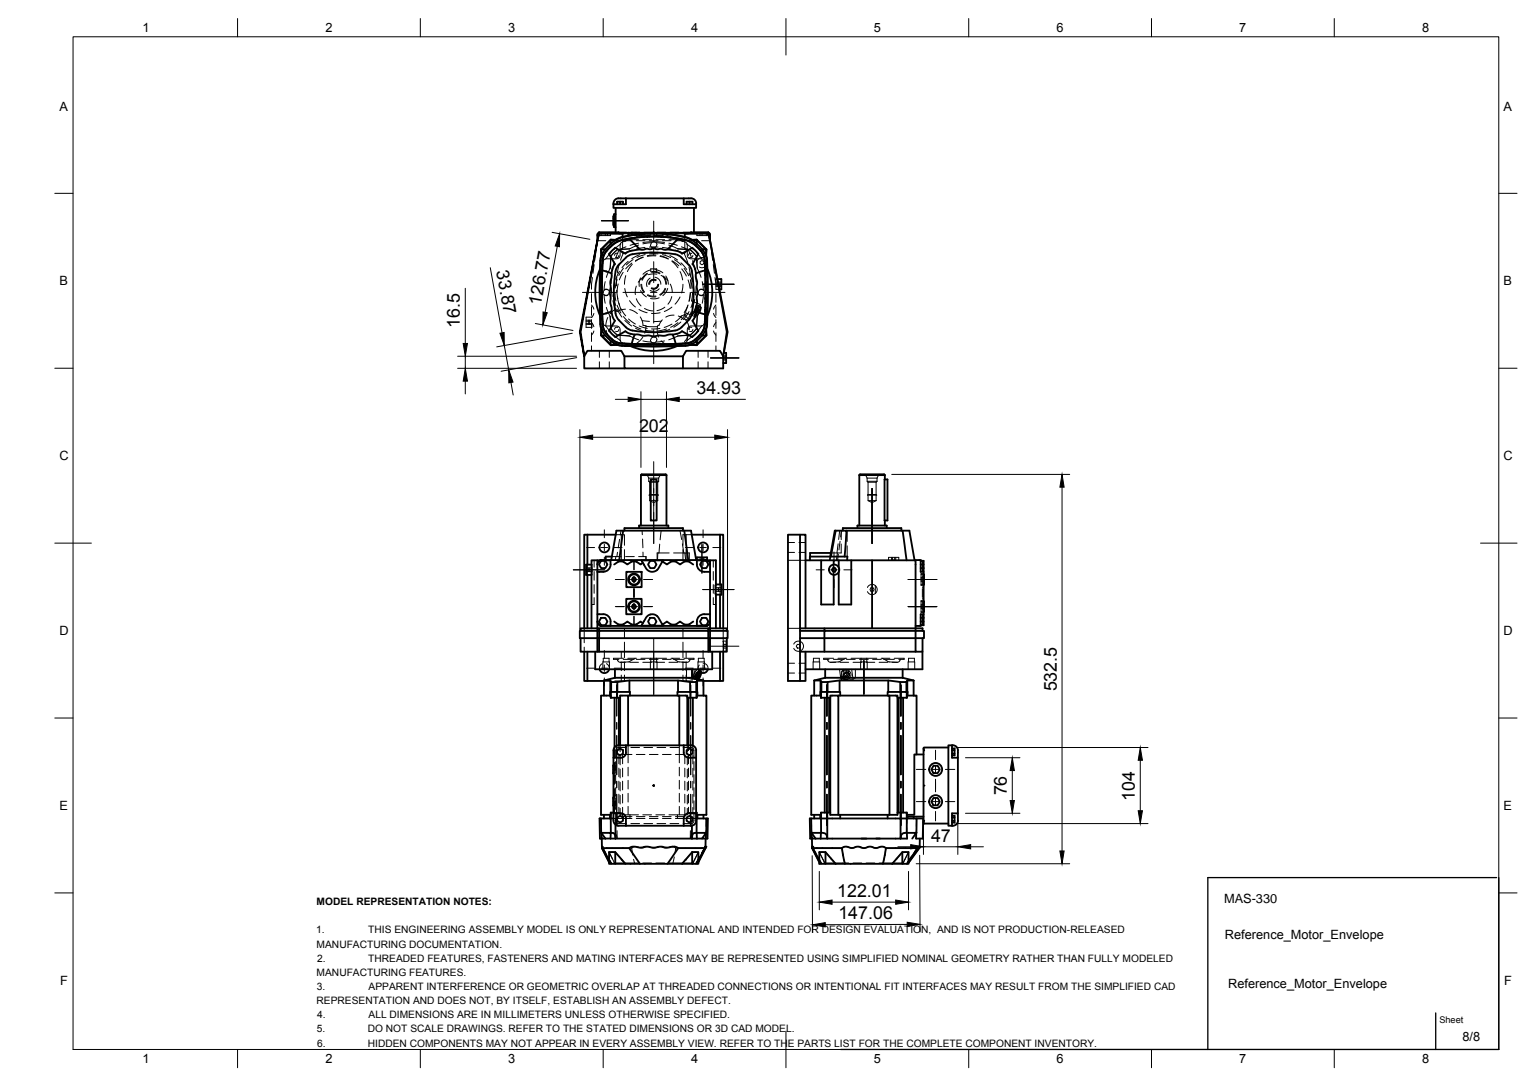
ISO-10303-21;
HEADER;
/* Generated by software containing ST-Developer
 * from STEP Tools, Inc. (www.steptools.com) 
 */

FILE_DESCRIPTION(
/* description */ ('STEP AP214'),
/* implementation_level */ '2;1');

FILE_NAME(
/* name */ 'Reference_Motor_Envelope.step',
/* time_stamp */ '2026-10-12T14:05:15-07:00',
/* author */ (''),
/* organization */ (''),
/* preprocessor_version */ 'ST-DEVELOPER v20.2',
/* originating_system */ 'Autodesk Translation Framework v15.15.0.0',
/* authorisation */ '');

FILE_SCHEMA (('AUTOMOTIVE_DESIGN { 1 0 10303 214 3 1 1 }'));
ENDSEC;

DATA;
#10=MECHANICAL_DESIGN_GEOMETRIC_PRESENTATION_REPRESENTATION('',(#288),#39959);
#95=SPHERICAL_SURFACE('',#19264,20.3600000000001);
#96=SPHERICAL_SURFACE('',#19265,20.3600000000002);
#97=(
BOUNDED_CURVE()
B_SPLINE_CURVE(3,(#30732,#30733,#30734,#30735),.UNSPECIFIED.,.F.,.F.)
B_SPLINE_CURVE_WITH_KNOTS((4,4),(-1.,-3.7852598383457E-5),.UNSPECIFIED.)
CURVE()
GEOMETRIC_REPRESENTATION_ITEM()
RATIONAL_B_SPLINE_CURVE((1.,0.978516928803385,0.978516115613319,0.999997560429802))
REPRESENTATION_ITEM('')
);
#98=(
BOUNDED_CURVE()
B_SPLINE_CURVE(3,(#30762,#30763,#30764,#30765),.UNSPECIFIED.,.F.,.F.)
B_SPLINE_CURVE_WITH_KNOTS((4,4),(-1.,0.),.UNSPECIFIED.)
CURVE()
GEOMETRIC_REPRESENTATION_ITEM()
RATIONAL_B_SPLINE_CURVE((1.,0.998672257010864,0.998672257010864,1.))
REPRESENTATION_ITEM('')
);
#99=(
BOUNDED_CURVE()
B_SPLINE_CURVE(2,(#31270,#31271,#31272),.UNSPECIFIED.,.F.,.F.)
B_SPLINE_CURVE_WITH_KNOTS((3,3),(-7.67019091974518,-5.57466309126419),
 .UNSPECIFIED.)
CURVE()
GEOMETRIC_REPRESENTATION_ITEM()
RATIONAL_B_SPLINE_CURVE((1.51474535125471,1.4769886104751,1.42144161629559))
REPRESENTATION_ITEM('')
);
#100=(
BOUNDED_CURVE()
B_SPLINE_CURVE(2,(#31276,#31277,#31278),.UNSPECIFIED.,.F.,.F.)
B_SPLINE_CURVE_WITH_KNOTS((3,3),(-18.6605106590412,-16.5649828305604),
 .UNSPECIFIED.)
CURVE()
GEOMETRIC_REPRESENTATION_ITEM()
RATIONAL_B_SPLINE_CURVE((1.4214416162955,1.476988610475,1.51474535125461))
REPRESENTATION_ITEM('')
);
#101=(
BOUNDED_CURVE()
B_SPLINE_CURVE(2,(#31282,#31283,#31284),.UNSPECIFIED.,.F.,.F.)
B_SPLINE_CURVE_WITH_KNOTS((3,3),(-7.6701909197441,-5.57466309126325),
 .UNSPECIFIED.)
CURVE()
GEOMETRIC_REPRESENTATION_ITEM()
RATIONAL_B_SPLINE_CURVE((1.51474535125461,1.47698861047501,1.4214416162955))
REPRESENTATION_ITEM('')
);
#102=(
BOUNDED_CURVE()
B_SPLINE_CURVE(2,(#31288,#31289,#31290),.UNSPECIFIED.,.F.,.F.)
B_SPLINE_CURVE_WITH_KNOTS((3,3),(-18.660510659043,-16.564982830562),
 .UNSPECIFIED.)
CURVE()
GEOMETRIC_REPRESENTATION_ITEM()
RATIONAL_B_SPLINE_CURVE((1.42144161629558,1.47698861047509,1.5147453512547))
REPRESENTATION_ITEM('')
);
#103=(
BOUNDED_CURVE()
B_SPLINE_CURVE(2,(#31295,#31296,#31297),.UNSPECIFIED.,.F.,.F.)
B_SPLINE_CURVE_WITH_KNOTS((3,3),(0.289788647925159,0.47130189078059),
 .UNSPECIFIED.)
CURVE()
GEOMETRIC_REPRESENTATION_ITEM()
RATIONAL_B_SPLINE_CURVE((1.27594103621743,1.36080572125034,1.44372227312264))
REPRESENTATION_ITEM('')
);
#104=(
BOUNDED_CURVE()
B_SPLINE_CURVE(2,(#31299,#31300,#31301),.UNSPECIFIED.,.F.,.F.)
B_SPLINE_CURVE_WITH_KNOTS((3,3),(4.49748593074956,6.56746087072966),
 .UNSPECIFIED.)
CURVE()
GEOMETRIC_REPRESENTATION_ITEM()
RATIONAL_B_SPLINE_CURVE((1.14470058445899,1.15519608505713,1.14470058445899))
REPRESENTATION_ITEM('')
);
#105=(
BOUNDED_CURVE()
B_SPLINE_CURVE(2,(#31302,#31303,#31304),.UNSPECIFIED.,.F.,.F.)
B_SPLINE_CURVE_WITH_KNOTS((3,3),(0.289788647925165,0.4713018907806),
 .UNSPECIFIED.)
CURVE()
GEOMETRIC_REPRESENTATION_ITEM()
RATIONAL_B_SPLINE_CURVE((1.27594103621742,1.36080572125034,1.44372227312264))
REPRESENTATION_ITEM('')
);
#106=(
BOUNDED_CURVE()
B_SPLINE_CURVE(2,(#31308,#31309,#31310),.UNSPECIFIED.,.F.,.F.)
B_SPLINE_CURVE_WITH_KNOTS((3,3),(16.5649828305673,18.6605106590487),
 .UNSPECIFIED.)
CURVE()
GEOMETRIC_REPRESENTATION_ITEM()
RATIONAL_B_SPLINE_CURVE((1.514745351255,1.47698861047538,1.42144161629586))
REPRESENTATION_ITEM('')
);
#107=(
BOUNDED_CURVE()
B_SPLINE_CURVE(2,(#31314,#31315,#31316),.UNSPECIFIED.,.F.,.F.)
B_SPLINE_CURVE_WITH_KNOTS((3,3),(5.57466309126757,7.67019091974901),
 .UNSPECIFIED.)
CURVE()
GEOMETRIC_REPRESENTATION_ITEM()
RATIONAL_B_SPLINE_CURVE((1.4214416162959,1.47698861047542,1.51474535125504))
REPRESENTATION_ITEM('')
);
#108=(
BOUNDED_CURVE()
B_SPLINE_CURVE(2,(#31320,#31321,#31322),.UNSPECIFIED.,.F.,.F.)
B_SPLINE_CURVE_WITH_KNOTS((3,3),(16.5649828305679,18.6605106590493),
 .UNSPECIFIED.)
CURVE()
GEOMETRIC_REPRESENTATION_ITEM()
RATIONAL_B_SPLINE_CURVE((1.51474535125504,1.47698861047542,1.4214416162959))
REPRESENTATION_ITEM('')
);
#109=(
BOUNDED_CURVE()
B_SPLINE_CURVE(2,(#31325,#31326,#31327),.UNSPECIFIED.,.F.,.F.)
B_SPLINE_CURVE_WITH_KNOTS((3,3),(5.5746630912673,7.67019091974871),
 .UNSPECIFIED.)
CURVE()
GEOMETRIC_REPRESENTATION_ITEM()
RATIONAL_B_SPLINE_CURVE((1.42144161629587,1.47698861047539,1.514745351255))
REPRESENTATION_ITEM('')
);
#110=(
BOUNDED_CURVE()
B_SPLINE_CURVE(2,(#32616,#32617,#32618),.UNSPECIFIED.,.F.,.F.)
B_SPLINE_CURVE_WITH_KNOTS((3,3),(-33.3299544599618,-31.4526565385171),
 .UNSPECIFIED.)
CURVE()
GEOMETRIC_REPRESENTATION_ITEM()
RATIONAL_B_SPLINE_CURVE((1.20098306198357,1.20314118954088,1.20441859364838))
REPRESENTATION_ITEM('')
);
#111=(
BOUNDED_CURVE()
B_SPLINE_CURVE(3,(#32734,#32735,#32736,#32737),.UNSPECIFIED.,.F.,.F.)
B_SPLINE_CURVE_WITH_KNOTS((4,4),(0.,1.),.UNSPECIFIED.)
CURVE()
GEOMETRIC_REPRESENTATION_ITEM()
RATIONAL_B_SPLINE_CURVE((0.996955268533354,0.975234645152216,0.976249555641098,
1.))
REPRESENTATION_ITEM('')
);
#112=(
BOUNDED_CURVE()
B_SPLINE_CURVE(3,(#32739,#32740,#32741,#32742),.UNSPECIFIED.,.F.,.F.)
B_SPLINE_CURVE_WITH_KNOTS((4,4),(0.,1.),.UNSPECIFIED.)
CURVE()
GEOMETRIC_REPRESENTATION_ITEM()
RATIONAL_B_SPLINE_CURVE((1.,0.976245441159908,0.975234294192269,0.996966559097083))
REPRESENTATION_ITEM('')
);
#125=ORIENTED_CLOSED_SHELL('',*,#18265,.F.);
#126=ORIENTED_CLOSED_SHELL('',*,#18266,.F.);
#127=ORIENTED_CLOSED_SHELL('',*,#18267,.F.);
#128=ORIENTED_CLOSED_SHELL('',*,#18268,.F.);
#129=CONICAL_SURFACE('',#18879,28.6682517601201,1.23062314824616);
#130=CONICAL_SURFACE('',#18880,50.,0.475882249660419);
#131=CONICAL_SURFACE('',#18882,32.793965079916,0.986624506004945);
#132=CONICAL_SURFACE('',#18883,45.3097394023382,1.52321322351791);
#133=CONICAL_SURFACE('',#18886,0.857142857149273,0.197395559849881);
#134=CONICAL_SURFACE('',#18890,0.999999999925894,0.463647609000806);
#135=CONICAL_SURFACE('',#18893,0.499999999966139,0.463647608692697);
#136=CONICAL_SURFACE('',#18930,107.1412427187,0.174532925199605);
#137=CONICAL_SURFACE('',#18993,76.5,1.3264502315157);
#138=CONICAL_SURFACE('',#19016,6.99999999990287,0.785398163411024);
#139=CONICAL_SURFACE('',#19043,17.4625,0.785398163397448);
#140=CONICAL_SURFACE('',#19069,945.,0.0174532925199452);
#141=CONICAL_SURFACE('',#19072,6.75000000001091,0.785398163397448);
#142=CONICAL_SURFACE('',#19078,942.,0.0174532925199432);
#143=CONICAL_SURFACE('',#19090,6.34999999994079,0.785398163364011);
#144=CONICAL_SURFACE('',#19099,5.4999999998131,1.10714871774448);
#145=CONICAL_SURFACE('',#19291,96.9819619535671,1.14717901504738);
#146=CONICAL_SURFACE('',#19315,22.3000008196592,0.0174532925199444);
#147=CONICAL_SURFACE('',#19317,86.00000081803,0.0174532925199416);
#148=CONICAL_SURFACE('',#19319,22.3000010500621,0.0174532925199414);
#149=CONICAL_SURFACE('',#19321,942.000001054498,0.0174532925199525);
#150=CONICAL_SURFACE('',#19323,22.3000013536827,0.0174532925199416);
#151=CONICAL_SURFACE('',#19325,86.0000013640202,0.0174532925199415);
#152=CONICAL_SURFACE('',#19327,22.3000017511903,0.0174532925199381);
#153=CONICAL_SURFACE('',#19329,22.3000017511903,0.0174532925199378);
#154=CONICAL_SURFACE('',#19331,86.0000013640202,0.0174532925199428);
#155=CONICAL_SURFACE('',#19333,32.8000013531573,0.0174532925199434);
#156=CONICAL_SURFACE('',#19335,200.000000812291,0.0174532925199407);
#157=CONICAL_SURFACE('',#19337,32.8000008122913,0.0174532925199388);
#158=CONICAL_SURFACE('',#19339,86.0000008122913,0.0174532925199416);
#159=CONICAL_SURFACE('',#19341,22.3000008122913,0.0174532925199454);
#160=CONICAL_SURFACE('',#19343,941.999999061101,0.017453292519947);
#161=CONICAL_SURFACE('',#19389,25.2657032643209,0.0174532925199449);
#162=CONICAL_SURFACE('',#19394,25.2657032643207,0.0174532925199417);
#163=CONICAL_SURFACE('',#19396,945.,0.0174532925199452);
#164=CONICAL_SURFACE('',#19398,25.2657032643207,0.0174532925199417);
#165=CONICAL_SURFACE('',#19403,25.2657032643145,0.0174532925199406);
#166=CONICAL_SURFACE('',#19405,25.2657032643204,0.0174532925199395);
#167=CONICAL_SURFACE('',#19410,34.9999999991313,0.0174532925199434);
#168=CONICAL_SURFACE('',#19412,180.,0.017453292519941);
#169=CONICAL_SURFACE('',#19414,34.9999999991315,0.0174532925199386);
#170=CONICAL_SURFACE('',#19419,25.2657032643206,0.0174532925199426);
#171=CONICAL_SURFACE('',#19421,945.,0.0174532925199372);
#172=CONICAL_SURFACE('',#19904,107.1412427187,0.174532925199605);
#173=CONICAL_SURFACE('',#19906,107.1412427187,0.174532925199605);
#174=CONICAL_SURFACE('',#19908,107.1412427187,0.174532925199605);
#175=CONICAL_SURFACE('',#19910,107.1412427187,0.174532925199605);
#183=BREP_WITH_VOIDS('Body1',#18269,(#125,#126,#127,#128));
#188=(
BOUNDED_SURFACE()
B_SPLINE_SURFACE(3,1,((#30722,#30723),(#30724,#30725),(#30726,#30727),(#30728,
#30729)),.UNSPECIFIED.,.F.,.F.,.F.)
B_SPLINE_SURFACE_WITH_KNOTS((4,4),(2,2),(0.,1.),(0.,1.),.UNSPECIFIED.)
GEOMETRIC_REPRESENTATION_ITEM()
RATIONAL_B_SPLINE_SURFACE(((1.,1.),(0.978516115582536,0.975189339715083),
(0.978516115582536,0.975189339715083),(1.,1.)))
REPRESENTATION_ITEM('')
SURFACE()
);
#189=(
BOUNDED_SURFACE()
B_SPLINE_SURFACE(3,1,((#30753,#30754),(#30755,#30756),(#30757,#30758),(#30759,
#30760)),.UNSPECIFIED.,.F.,.F.,.F.)
B_SPLINE_SURFACE_WITH_KNOTS((4,4),(2,2),(0.,1.),(0.,0.740226077012362),
 .UNSPECIFIED.)
GEOMETRIC_REPRESENTATION_ITEM()
RATIONAL_B_SPLINE_SURFACE(((1.,1.),(0.998672257010864,0.999507458473034),
(0.998672257010864,0.999507458473034),(1.,1.)))
REPRESENTATION_ITEM('')
SURFACE()
);
#190=(
BOUNDED_SURFACE()
B_SPLINE_SURFACE(3,1,((#31681,#31682),(#31683,#31684),(#31685,#31686),(#31687,
#31688)),.UNSPECIFIED.,.F.,.F.,.F.)
B_SPLINE_SURFACE_WITH_KNOTS((4,4),(2,2),(0.,1.),(-0.000822310060064629,
0.),.UNSPECIFIED.)
GEOMETRIC_REPRESENTATION_ITEM()
RATIONAL_B_SPLINE_SURFACE(((1.,1.),(0.962057791684876,0.962057791684876),
(0.962057791684876,0.962057791684876),(1.,1.)))
REPRESENTATION_ITEM('')
SURFACE()
);
#191=(
BOUNDED_SURFACE()
B_SPLINE_SURFACE(3,1,((#31700,#31701),(#31702,#31703),(#31704,#31705),(#31706,
#31707)),.UNSPECIFIED.,.F.,.F.,.F.)
B_SPLINE_SURFACE_WITH_KNOTS((4,4),(2,2),(0.,1.),(-0.000910780085741153,
0.),.UNSPECIFIED.)
GEOMETRIC_REPRESENTATION_ITEM()
RATIONAL_B_SPLINE_SURFACE(((1.,1.),(0.962057791684877,0.962057791684877),
(0.962057791684877,0.962057791684877),(1.,1.)))
REPRESENTATION_ITEM('')
SURFACE()
);
#192=(
BOUNDED_SURFACE()
B_SPLINE_SURFACE(3,1,((#31721,#31722),(#31723,#31724),(#31725,#31726),(#31727,
#31728)),.UNSPECIFIED.,.F.,.F.,.F.)
B_SPLINE_SURFACE_WITH_KNOTS((4,4),(2,2),(0.,1.),(0.,1.),.UNSPECIFIED.)
GEOMETRIC_REPRESENTATION_ITEM()
RATIONAL_B_SPLINE_SURFACE(((1.,1.),(0.962057791684877,0.975189339715083),
(0.962057791684877,0.975189339715083),(1.,1.)))
REPRESENTATION_ITEM('')
SURFACE()
);
#193=(
BOUNDED_SURFACE()
B_SPLINE_SURFACE(3,1,((#31772,#31773,#31774),(#31775,#31776,#31777),(#31778,
#31779,#31780),(#31781,#31782,#31783)),.UNSPECIFIED.,.F.,.F.,.F.)
B_SPLINE_SURFACE_WITH_KNOTS((4,4),(2,1,2),(0.633064943864098,0.634076354292062),
(-0.000184246289843766,0.,1.),.UNSPECIFIED.)
GEOMETRIC_REPRESENTATION_ITEM()
RATIONAL_B_SPLINE_SURFACE(((0.791557642220831,0.791557642220831,0.816814678743125),
(0.791557642220831,0.791557642220831,0.816814678743125),(0.791557642220831,
0.791557642220831,0.816814678743125),(0.791557642220831,0.791557642220831,
0.816814678743125)))
REPRESENTATION_ITEM('')
SURFACE()
);
#194=(
BOUNDED_SURFACE()
B_SPLINE_SURFACE(3,1,((#31793,#31794),(#31795,#31796),(#31797,#31798),(#31799,
#31800)),.UNSPECIFIED.,.F.,.F.,.F.)
B_SPLINE_SURFACE_WITH_KNOTS((4,4),(2,2),(0.,0.365923647633872),(0.,1.),
 .UNSPECIFIED.)
GEOMETRIC_REPRESENTATION_ITEM()
RATIONAL_B_SPLINE_SURFACE(((1.,1.),(0.89042205119026,0.903699651216535),
(0.820941265109217,0.84263787732833),(0.791557641756873,0.816814678335385)))
REPRESENTATION_ITEM('')
SURFACE()
);
#195=(
BOUNDED_SURFACE()
B_SPLINE_SURFACE(3,1,((#31831,#31832),(#31833,#31834),(#31835,#31836),(#31837,
#31838)),.UNSPECIFIED.,.F.,.F.,.F.)
B_SPLINE_SURFACE_WITH_KNOTS((4,4),(2,2),(0.,1.),(-0.000981925268428012,
0.),.UNSPECIFIED.)
GEOMETRIC_REPRESENTATION_ITEM()
RATIONAL_B_SPLINE_SURFACE(((1.,1.),(0.96205779168488,0.96205779168488),
(0.96205779168488,0.96205779168488),(1.,1.)))
REPRESENTATION_ITEM('')
SURFACE()
);
#196=(
BOUNDED_SURFACE()
B_SPLINE_SURFACE(3,1,((#31853,#31854),(#31855,#31856),(#31857,#31858),(#31859,
#31860)),.UNSPECIFIED.,.F.,.F.,.F.)
B_SPLINE_SURFACE_WITH_KNOTS((4,4),(2,2),(0.,1.),(0.,1.),.UNSPECIFIED.)
GEOMETRIC_REPRESENTATION_ITEM()
RATIONAL_B_SPLINE_SURFACE(((1.,1.),(0.96205779168488,0.975189339715083),
(0.96205779168488,0.975189339715083),(1.,1.)))
REPRESENTATION_ITEM('')
SURFACE()
);
#197=(
BOUNDED_SURFACE()
B_SPLINE_SURFACE(3,1,((#31906,#31907),(#31908,#31909),(#31910,#31911),(#31912,
#31913)),.UNSPECIFIED.,.F.,.F.,.F.)
B_SPLINE_SURFACE_WITH_KNOTS((4,4),(2,2),(0.,1.),(-0.000863309921543448,
0.),.UNSPECIFIED.)
GEOMETRIC_REPRESENTATION_ITEM()
RATIONAL_B_SPLINE_SURFACE(((1.,1.),(0.96207291357299,0.96207291357299),
(0.96207291357299,0.96207291357299),(1.,1.)))
REPRESENTATION_ITEM('')
SURFACE()
);
#198=(
BOUNDED_SURFACE()
B_SPLINE_SURFACE(3,1,((#31927,#31928),(#31929,#31930),(#31931,#31932),(#31933,
#31934)),.UNSPECIFIED.,.F.,.F.,.F.)
B_SPLINE_SURFACE_WITH_KNOTS((4,4),(2,2),(0.,1.),(0.,1.),.UNSPECIFIED.)
GEOMETRIC_REPRESENTATION_ITEM()
RATIONAL_B_SPLINE_SURFACE(((1.,1.),(0.96207291357299,0.975189339715083),
(0.96207291357299,0.975189339715083),(1.,1.)))
REPRESENTATION_ITEM('')
SURFACE()
);
#199=(
BOUNDED_SURFACE()
B_SPLINE_SURFACE(3,1,((#31980,#31981),(#31982,#31983),(#31984,#31985),(#31986,
#31987)),.UNSPECIFIED.,.F.,.F.,.F.)
B_SPLINE_SURFACE_WITH_KNOTS((4,4),(2,2),(0.,1.),(-0.000880114866331669,
0.),.UNSPECIFIED.)
GEOMETRIC_REPRESENTATION_ITEM()
RATIONAL_B_SPLINE_SURFACE(((1.,1.),(0.962072913572991,0.962072913572991),
(0.962072913572991,0.962072913572991),(1.,1.)))
REPRESENTATION_ITEM('')
SURFACE()
);
#200=(
BOUNDED_SURFACE()
B_SPLINE_SURFACE(3,1,((#32001,#32002),(#32003,#32004),(#32005,#32006),(#32007,
#32008)),.UNSPECIFIED.,.F.,.F.,.F.)
B_SPLINE_SURFACE_WITH_KNOTS((4,4),(2,2),(0.,1.),(-0.000751572727532702,
0.),.UNSPECIFIED.)
GEOMETRIC_REPRESENTATION_ITEM()
RATIONAL_B_SPLINE_SURFACE(((1.,1.),(0.962057791684879,0.962057791684879),
(0.962057791684879,0.962057791684879),(1.,1.)))
REPRESENTATION_ITEM('')
SURFACE()
);
#201=(
BOUNDED_SURFACE()
B_SPLINE_SURFACE(3,1,((#32916,#32917),(#32918,#32919),(#32920,#32921),(#32922,
#32923)),.UNSPECIFIED.,.F.,.F.,.F.)
B_SPLINE_SURFACE_WITH_KNOTS((4,4),(2,2),(0.,1.),(0.,1.),.UNSPECIFIED.)
GEOMETRIC_REPRESENTATION_ITEM()
RATIONAL_B_SPLINE_SURFACE(((1.,1.),(0.962057791684879,0.975189339715082),
(0.962057791684879,0.975189339715082),(1.,1.)))
REPRESENTATION_ITEM('')
SURFACE()
);
#202=(
BOUNDED_SURFACE()
B_SPLINE_SURFACE(3,1,((#32926,#32927,#32928,#32929),(#32930,#32931,#32932,
#32933),(#32934,#32935,#32936,#32937),(#32938,#32939,#32940,#32941),(#32942,
#32943,#32944,#32945),(#32946,#32947,#32948,#32949),(#32950,#32951,#32952,
#32953),(#32954,#32955,#32956,#32957),(#32958,#32959,#32960,#32961),(#32962,
#32963,#32964,#32965)),.UNSPECIFIED.,.F.,.F.,.F.)
B_SPLINE_SURFACE_WITH_KNOTS((4,3,3,4),(2,1,1,2),(-0.000662388520973799,
0.,1.,1.00066238358002),(-0.00076018000588443,0.,0.676109671237994,0.676144257435705),
 .UNSPECIFIED.)
GEOMETRIC_REPRESENTATION_ITEM()
RATIONAL_B_SPLINE_SURFACE(((1.,1.,1.,1.),(1.,1.,1.,1.),(1.,1.,1.,1.),(1.,
1.,1.,1.),(0.998736553042339,0.998736553042339,0.999455940415833,0.999455940415833),
(0.998736553042339,0.998736553042339,0.999455940415833,0.999455940415833),
(1.,1.,1.,1.),(1.,1.,1.,1.),(1.,1.,1.,1.),(1.,1.,1.,1.)))
REPRESENTATION_ITEM('')
SURFACE()
);
#203=(
BOUNDED_SURFACE()
B_SPLINE_SURFACE(3,1,((#32993,#32994),(#32995,#32996),(#32997,#32998),(#32999,
#33000)),.UNSPECIFIED.,.F.,.F.,.F.)
B_SPLINE_SURFACE_WITH_KNOTS((4,4),(2,2),(0.,1.),(0.,1.),.UNSPECIFIED.)
GEOMETRIC_REPRESENTATION_ITEM()
RATIONAL_B_SPLINE_SURFACE(((1.,1.),(0.962072913572991,0.975189339715083),
(0.962072913572991,0.975189339715083),(1.,1.)))
REPRESENTATION_ITEM('')
SURFACE()
);
#204=(
BOUNDED_SURFACE()
B_SPLINE_SURFACE(3,1,((#33002,#33003,#33004,#33005),(#33006,#33007,#33008,
#33009),(#33010,#33011,#33012,#33013),(#33014,#33015,#33016,#33017)),
 .UNSPECIFIED.,.F.,.F.,.F.)
B_SPLINE_SURFACE_WITH_KNOTS((4,4),(2,1,1,2),(0.847974360952231,1.),(-0.000384803530329693,
0.,1.,1.001),.UNSPECIFIED.)
GEOMETRIC_REPRESENTATION_ITEM()
RATIONAL_B_SPLINE_SURFACE(((0.9997286731407,0.9997286731407,0.99414139959028,
0.99414139959028),(0.999802900849163,0.999802900849163,0.995744154600748,
0.995744154600748),(0.999893343135597,0.999893343135597,0.997697021403988,
0.997697021403988),(1.,1.,1.,1.)))
REPRESENTATION_ITEM('')
SURFACE()
);
#205=(
BOUNDED_SURFACE()
B_SPLINE_SURFACE(3,1,((#33043,#33044),(#33045,#33046),(#33047,#33048),(#33049,
#33050)),.UNSPECIFIED.,.F.,.F.,.F.)
B_SPLINE_SURFACE_WITH_KNOTS((4,4),(2,2),(0.,0.366201644461032),(0.,1.),
 .UNSPECIFIED.)
GEOMETRIC_REPRESENTATION_ITEM()
RATIONAL_B_SPLINE_SURFACE(((1.,1.),(0.890338803435454,0.903626490622545),
(0.820835717386409,0.842545118861594),(0.791490741852866,0.816755884717148)))
REPRESENTATION_ITEM('')
SURFACE()
);
#206=(
BOUNDED_SURFACE()
B_SPLINE_SURFACE(3,1,((#33065,#33066),(#33067,#33068),(#33069,#33070),(#33071,
#33072)),.UNSPECIFIED.,.F.,.F.,.F.)
B_SPLINE_SURFACE_WITH_KNOTS((4,4),(2,2),(0.,1.),(0.,0.966511290545803),
 .UNSPECIFIED.)
GEOMETRIC_REPRESENTATION_ITEM()
RATIONAL_B_SPLINE_SURFACE(((1.,1.),(0.969175395688119,0.979164837438946),
(0.969175395688119,0.979164837438946),(1.,1.)))
REPRESENTATION_ITEM('')
SURFACE()
);
#207=(
BOUNDED_SURFACE()
B_SPLINE_SURFACE(3,1,((#33093,#33094),(#33095,#33096),(#33097,#33098),(#33099,
#33100)),.UNSPECIFIED.,.F.,.F.,.F.)
B_SPLINE_SURFACE_WITH_KNOTS((4,4),(2,2),(0.,1.),(0.,1.),.UNSPECIFIED.)
GEOMETRIC_REPRESENTATION_ITEM()
RATIONAL_B_SPLINE_SURFACE(((1.,1.),(0.97852393395982,0.98163056167315),
(0.97852393395982,0.98163056167315),(1.,1.)))
REPRESENTATION_ITEM('')
SURFACE()
);
#208=(
BOUNDED_SURFACE()
B_SPLINE_SURFACE(3,1,((#33115,#33116),(#33117,#33118),(#33119,#33120),(#33121,
#33122)),.UNSPECIFIED.,.F.,.F.,.F.)
B_SPLINE_SURFACE_WITH_KNOTS((4,4),(2,2),(0.,1.),(0.,0.960625757105633),
 .UNSPECIFIED.)
GEOMETRIC_REPRESENTATION_ITEM()
RATIONAL_B_SPLINE_SURFACE(((1.,1.),(0.969713710620478,0.979821031654969),
(0.969713710620478,0.979821031654969),(1.,1.)))
REPRESENTATION_ITEM('')
SURFACE()
);
#209=(
BOUNDED_SURFACE()
B_SPLINE_SURFACE(3,1,((#33145,#33146),(#33147,#33148),(#33149,#33150),(#33151,
#33152)),.UNSPECIFIED.,.F.,.F.,.F.)
B_SPLINE_SURFACE_WITH_KNOTS((4,4),(2,2),(0.,1.),(0.,1.),.UNSPECIFIED.)
GEOMETRIC_REPRESENTATION_ITEM()
RATIONAL_B_SPLINE_SURFACE(((1.,1.),(0.978523933959819,0.981630561673153),
(0.978523933959819,0.981630561673153),(1.,1.)))
REPRESENTATION_ITEM('')
SURFACE()
);
#210=(
BOUNDED_SURFACE()
B_SPLINE_SURFACE(3,1,((#33167,#33168),(#33169,#33170),(#33171,#33172),(#33173,
#33174)),.UNSPECIFIED.,.F.,.F.,.F.)
B_SPLINE_SURFACE_WITH_KNOTS((4,4),(2,2),(0.,1.),(0.,0.966511290545776),
 .UNSPECIFIED.)
GEOMETRIC_REPRESENTATION_ITEM()
RATIONAL_B_SPLINE_SURFACE(((1.,1.),(0.969175395688119,0.979164837438949),
(0.969175395688119,0.979164837438949),(1.,1.)))
REPRESENTATION_ITEM('')
SURFACE()
);
#211=(
BOUNDED_SURFACE()
B_SPLINE_SURFACE(3,1,((#33197,#33198),(#33199,#33200),(#33201,#33202),(#33203,
#33204)),.UNSPECIFIED.,.F.,.F.,.F.)
B_SPLINE_SURFACE_WITH_KNOTS((4,4),(2,2),(0.633798356768784,1.),(0.,1.),
 .UNSPECIFIED.)
GEOMETRIC_REPRESENTATION_ITEM()
RATIONAL_B_SPLINE_SURFACE(((0.791490742148516,0.816755884976974),(0.820835717853236,
0.842545119271855),(0.890338803803731,0.903626490946197),(1.,1.)))
REPRESENTATION_ITEM('')
SURFACE()
);
#212=(
BOUNDED_SURFACE()
B_SPLINE_SURFACE(3,1,((#33226,#33227,#33228,#33229),(#33230,#33231,#33232,
#33233),(#33234,#33235,#33236,#33237),(#33238,#33239,#33240,#33241)),
 .UNSPECIFIED.,.F.,.F.,.F.)
B_SPLINE_SURFACE_WITH_KNOTS((4,4),(2,1,1,2),(0.,0.152025639047805),(-0.000385633117440705,
0.,1.,1.001),.UNSPECIFIED.)
GEOMETRIC_REPRESENTATION_ITEM()
RATIONAL_B_SPLINE_SURFACE(((1.,1.,1.,1.),(0.999893343135597,0.999893343135597,
0.997697021403987,0.997697021403987),(0.999802900849163,0.999802900849163,
0.995744154600747,0.995744154600747),(0.9997286731407,0.9997286731407,0.994141399590279,
0.994141399590279)))
REPRESENTATION_ITEM('')
SURFACE()
);
#213=(
BOUNDED_SURFACE()
B_SPLINE_SURFACE(3,1,((#33248,#33249),(#33250,#33251),(#33252,#33253),(#33254,
#33255)),.UNSPECIFIED.,.F.,.F.,.F.)
B_SPLINE_SURFACE_WITH_KNOTS((4,4),(2,2),(0.,1.),(1.,1.00115361672614),
 .UNSPECIFIED.)
GEOMETRIC_REPRESENTATION_ITEM()
RATIONAL_B_SPLINE_SURFACE(((1.,1.),(0.975189339715083,0.975189339715083),
(0.975189339715083,0.975189339715083),(1.,1.)))
REPRESENTATION_ITEM('')
SURFACE()
);
#214=(
BOUNDED_SURFACE()
B_SPLINE_SURFACE(3,1,((#33256,#33257,#33258,#33259),(#33260,#33261,#33262,
#33263),(#33264,#33265,#33266,#33267),(#33268,#33269,#33270,#33271),(#33272,
#33273,#33274,#33275),(#33276,#33277,#33278,#33279),(#33280,#33281,#33282,
#33283),(#33284,#33285,#33286,#33287),(#33288,#33289,#33290,#33291),(#33292,
#33293,#33294,#33295)),.UNSPECIFIED.,.F.,.F.,.F.)
B_SPLINE_SURFACE_WITH_KNOTS((4,3,3,4),(2,1,1,2),(-0.000651766775030853,
0.,1.,1.00065175575688),(-0.000817120226221179,0.,0.676109671237986,0.676119671237986),
 .UNSPECIFIED.)
GEOMETRIC_REPRESENTATION_ITEM()
RATIONAL_B_SPLINE_SURFACE(((1.,1.,1.,1.),(1.,1.,1.,1.),(1.,1.,1.,1.),(1.,
1.,1.,1.),(0.998736553042339,0.998736553042339,0.999455940415833,0.999455940415833),
(0.998736553042339,0.998736553042339,0.999455940415833,0.999455940415833),
(1.,1.,1.,1.),(1.,1.,1.,1.),(1.,1.,1.,1.),(1.,1.,1.,1.)))
REPRESENTATION_ITEM('')
SURFACE()
);
#215=(
BOUNDED_SURFACE()
B_SPLINE_SURFACE(3,1,((#33318,#33319),(#33320,#33321),(#33322,#33323),(#33324,
#33325)),.UNSPECIFIED.,.F.,.F.,.F.)
B_SPLINE_SURFACE_WITH_KNOTS((4,4),(2,2),(0.,1.),(1.,1.00127139915746),
 .UNSPECIFIED.)
GEOMETRIC_REPRESENTATION_ITEM()
RATIONAL_B_SPLINE_SURFACE(((1.,1.),(0.975189339715083,0.975189339715083),
(0.975189339715083,0.975189339715083),(1.,1.)))
REPRESENTATION_ITEM('')
SURFACE()
);
#216=(
BOUNDED_SURFACE()
B_SPLINE_SURFACE(3,1,((#33333,#33334,#33335,#33336),(#33337,#33338,#33339,
#33340),(#33341,#33342,#33343,#33344),(#33345,#33346,#33347,#33348),(#33349,
#33350,#33351,#33352),(#33353,#33354,#33355,#33356),(#33357,#33358,#33359,
#33360)),.UNSPECIFIED.,.F.,.F.,.F.)
B_SPLINE_SURFACE_WITH_KNOTS((4,3,4),(2,1,1,2),(0.,0.15224442477612,0.152293862972879),
(-0.000531337228447352,0.,1.,1.001),.UNSPECIFIED.)
GEOMETRIC_REPRESENTATION_ITEM()
RATIONAL_B_SPLINE_SURFACE(((1.,1.,1.,1.),(0.999893154836255,0.999893154836255,
0.997693707102185,0.997693707102186),(0.999802576253004,0.999802576253004,
0.995738534439964,0.995738534439964),(0.999728264250248,0.999728264250248,
0.994134482013335,0.994134482013335),(0.999728264250248,0.999728264250248,
0.994134482013335,0.994134482013335),(0.999728264250248,0.999728264250248,
0.994134482013335,0.994134482013335),(0.999728264250248,0.999728264250248,
0.994134482013335,0.994134482013335)))
REPRESENTATION_ITEM('')
SURFACE()
);
#217=(
BOUNDED_SURFACE()
B_SPLINE_SURFACE(3,1,((#33373,#33374,#33375,#33376),(#33377,#33378,#33379,
#33380),(#33381,#33382,#33383,#33384),(#33385,#33386,#33387,#33388)),
 .UNSPECIFIED.,.F.,.F.,.F.)
B_SPLINE_SURFACE_WITH_KNOTS((4,4),(2,1,1,2),(0.847755575223898,1.),(-0.000531332476382396,
0.,1.,1.001),.UNSPECIFIED.)
GEOMETRIC_REPRESENTATION_ITEM()
RATIONAL_B_SPLINE_SURFACE(((0.999728264250248,0.999728264250248,0.994134482013336,
0.994134482013336),(0.999802576253004,0.999802576253004,0.995738534439964,
0.995738534439964),(0.999893154836255,0.999893154836255,0.997693707102186,
0.997693707102186),(1.,1.,1.,1.)))
REPRESENTATION_ITEM('')
SURFACE()
);
#218=(
BOUNDED_SURFACE()
B_SPLINE_SURFACE(3,1,((#33391,#33392,#33393,#33394),(#33395,#33396,#33397,
#33398),(#33399,#33400,#33401,#33402),(#33403,#33404,#33405,#33406)),
 .UNSPECIFIED.,.F.,.F.,.F.)
B_SPLINE_SURFACE_WITH_KNOTS((4,4),(2,1,1,2),(0.365923647633872,0.36753176510902),
(-0.000355481502485282,0.,1.,1.0002958898079),.UNSPECIFIED.)
GEOMETRIC_REPRESENTATION_ITEM()
RATIONAL_B_SPLINE_SURFACE(((0.791557641756873,0.791557641756873,0.816814678335385,
0.816814678335385),(0.791557641756873,0.791557641756873,0.816814678335385,
0.816814678335385),(0.791557641756873,0.791557641756873,0.816814678335385,
0.816814678335385),(0.791557641756873,0.791557641756873,0.816814678335385,
0.816814678335385)))
REPRESENTATION_ITEM('')
SURFACE()
);
#219=(
BOUNDED_SURFACE()
B_SPLINE_SURFACE(3,1,((#33407,#33408),(#33409,#33410),(#33411,#33412),(#33413,
#33414)),.UNSPECIFIED.,.F.,.F.,.F.)
B_SPLINE_SURFACE_WITH_KNOTS((4,4),(2,2),(0.,1.),(0.,0.966044174191949),
 .UNSPECIFIED.)
GEOMETRIC_REPRESENTATION_ITEM()
RATIONAL_B_SPLINE_SURFACE(((1.,1.),(0.969175395688119,0.979160009526791),
(0.969175395688119,0.979160009526791),(1.,1.)))
REPRESENTATION_ITEM('')
SURFACE()
);
#220=(
BOUNDED_SURFACE()
B_SPLINE_SURFACE(3,1,((#33423,#33424),(#33425,#33426),(#33427,#33428),(#33429,
#33430)),.UNSPECIFIED.,.F.,.F.,.F.)
B_SPLINE_SURFACE_WITH_KNOTS((4,4),(2,2),(0.,1.),(0.,1.),.UNSPECIFIED.)
GEOMETRIC_REPRESENTATION_ITEM()
RATIONAL_B_SPLINE_SURFACE(((1.,1.),(0.97852393395982,0.98163056167315),
(0.97852393395982,0.98163056167315),(1.,1.)))
REPRESENTATION_ITEM('')
SURFACE()
);
#221=(
BOUNDED_SURFACE()
B_SPLINE_SURFACE(3,1,((#33432,#33433),(#33434,#33435),(#33436,#33437),(#33438,
#33439)),.UNSPECIFIED.,.F.,.F.,.F.)
B_SPLINE_SURFACE_WITH_KNOTS((4,4),(2,2),(0.,1.),(0.,0.960122375136112),
 .UNSPECIFIED.)
GEOMETRIC_REPRESENTATION_ITEM()
RATIONAL_B_SPLINE_SURFACE(((1.,1.),(0.969713710620478,0.979815735270679),
(0.969713710620478,0.979815735270679),(1.,1.)))
REPRESENTATION_ITEM('')
SURFACE()
);
#222=(
BOUNDED_SURFACE()
B_SPLINE_SURFACE(3,1,((#33448,#33449),(#33450,#33451),(#33452,#33453),(#33454,
#33455)),.UNSPECIFIED.,.F.,.F.,.F.)
B_SPLINE_SURFACE_WITH_KNOTS((4,4),(2,2),(0.,1.),(0.,1.),.UNSPECIFIED.)
GEOMETRIC_REPRESENTATION_ITEM()
RATIONAL_B_SPLINE_SURFACE(((1.,1.),(0.978523933959819,0.981630561673153),
(0.978523933959819,0.981630561673153),(1.,1.)))
REPRESENTATION_ITEM('')
SURFACE()
);
#223=(
BOUNDED_SURFACE()
B_SPLINE_SURFACE(3,1,((#33457,#33458),(#33459,#33460),(#33461,#33462),(#33463,
#33464)),.UNSPECIFIED.,.F.,.F.,.F.)
B_SPLINE_SURFACE_WITH_KNOTS((4,4),(2,2),(0.,1.),(0.,0.966044174191933),
 .UNSPECIFIED.)
GEOMETRIC_REPRESENTATION_ITEM()
RATIONAL_B_SPLINE_SURFACE(((1.,1.),(0.969175395688119,0.979160009526794),
(0.969175395688119,0.979160009526794),(1.,1.)))
REPRESENTATION_ITEM('')
SURFACE()
);
#224=(
BOUNDED_SURFACE()
B_SPLINE_SURFACE(3,1,((#33466,#33467),(#33468,#33469),(#33470,#33471),(#33472,
#33473)),.UNSPECIFIED.,.F.,.F.,.F.)
B_SPLINE_SURFACE_WITH_KNOTS((4,4),(2,2),(0.634076354292062,1.),(0.,1.),
 .UNSPECIFIED.)
GEOMETRIC_REPRESENTATION_ITEM()
RATIONAL_B_SPLINE_SURFACE(((0.791557642220831,0.816814678743125),(0.820941265840603,
0.842637877971094),(0.890422051766993,0.903699651723386),(1.,1.)))
REPRESENTATION_ITEM('')
SURFACE()
);
#225=(
BOUNDED_SURFACE()
B_SPLINE_SURFACE(3,1,((#33474,#33475),(#33476,#33477),(#33478,#33479),(#33480,
#33481)),.UNSPECIFIED.,.F.,.F.,.F.)
B_SPLINE_SURFACE_WITH_KNOTS((4,4),(2,2),(0.,1.),(1.,1.00115971095081),
 .UNSPECIFIED.)
GEOMETRIC_REPRESENTATION_ITEM()
RATIONAL_B_SPLINE_SURFACE(((1.,1.),(0.975189339715083,0.975189339715083),
(0.975189339715083,0.975189339715083),(1.,1.)))
REPRESENTATION_ITEM('')
SURFACE()
);
#226=(
BOUNDED_SURFACE()
B_SPLINE_SURFACE(3,1,((#33482,#33483),(#33484,#33485),(#33486,#33487),(#33488,
#33489),(#33490,#33491),(#33492,#33493),(#33494,#33495),(#33496,#33497),
(#33498,#33499),(#33500,#33501)),.UNSPECIFIED.,.F.,.F.,.F.)
B_SPLINE_SURFACE_WITH_KNOTS((4,3,3,4),(2,2),(-0.000658266375657395,0.,1.,
1.00065830337858),(-0.000823662838273568,0.),.UNSPECIFIED.)
GEOMETRIC_REPRESENTATION_ITEM()
RATIONAL_B_SPLINE_SURFACE(((1.,1.),(1.,1.),(1.,1.),(1.,1.),(0.998672257010864,
0.998672257010864),(0.998672257010864,0.998672257010864),(1.,1.),(1.,1.),
(1.,1.),(1.,1.)))
REPRESENTATION_ITEM('')
SURFACE()
);
#227=(
BOUNDED_SURFACE()
B_SPLINE_SURFACE(3,1,((#33526,#33527),(#33528,#33529),(#33530,#33531),(#33532,
#33533)),.UNSPECIFIED.,.F.,.F.,.F.)
B_SPLINE_SURFACE_WITH_KNOTS((4,4),(2,2),(0.,1.),(-0.000998381213712629,
0.),.UNSPECIFIED.)
GEOMETRIC_REPRESENTATION_ITEM()
RATIONAL_B_SPLINE_SURFACE(((1.,1.),(0.978516115582536,0.978516115582536),
(0.978516115582536,0.978516115582536),(1.,1.)))
REPRESENTATION_ITEM('')
SURFACE()
);
#228=(
BOUNDED_SURFACE()
B_SPLINE_SURFACE(3,1,((#34127,#34128,#34129,#34130),(#34131,#34132,#34133,
#34134),(#34135,#34136,#34137,#34138),(#34139,#34140,#34141,#34142),(#34143,
#34144,#34145,#34146),(#34147,#34148,#34149,#34150),(#34151,#34152,#34153,
#34154),(#34155,#34156,#34157,#34158),(#34159,#34160,#34161,#34162),(#34163,
#34164,#34165,#34166)),.UNSPECIFIED.,.F.,.F.,.F.)
B_SPLINE_SURFACE_WITH_KNOTS((4,3,3,4),(2,1,1,2),(-0.001,0.,0.205321724422313,
0.206321724412313),(-0.000396813100233054,0.,1.,1.001),.UNSPECIFIED.)
GEOMETRIC_REPRESENTATION_ITEM()
RATIONAL_B_SPLINE_SURFACE(((1.,1.,1.,1.),(1.,1.,1.,1.),(1.,1.,1.,1.),(1.,
1.,1.,1.),(0.996948890458759,0.996948890458759,0.996889659273247,0.996889659273247),
(0.994524239989928,0.994524239989928,0.994417939068052,0.994417939068052),
(0.992726048593505,0.992726048593505,0.992584839384415,0.992584839384415),
(0.992726048593505,0.992726048593505,0.992584839384415,0.992584839384415),
(0.992726048593505,0.992726048593505,0.992584839384415,0.992584839384415),
(0.992726048593505,0.992726048593505,0.992584839384415,0.992584839384415)))
REPRESENTATION_ITEM('')
SURFACE()
);
#229=(
BOUNDED_SURFACE()
B_SPLINE_SURFACE(3,1,((#35952,#35953),(#35954,#35955),(#35956,#35957),(#35958,
#35959),(#35960,#35961),(#35962,#35963),(#35964,#35965)),.UNSPECIFIED.,
 .F.,.F.,.F.)
B_SPLINE_SURFACE_WITH_KNOTS((4,3,4),(2,2),(0.,1.,1.00008671004856),(0.,
0.740226077012249),.UNSPECIFIED.)
GEOMETRIC_REPRESENTATION_ITEM()
RATIONAL_B_SPLINE_SURFACE(((1.,1.),(0.998672257010864,0.999507458473034),
(0.998672257010864,0.999507458473034),(1.,1.),(1.,1.),(1.,1.),(1.,1.)))
REPRESENTATION_ITEM('')
SURFACE()
);
#230=(
BOUNDED_SURFACE()
B_SPLINE_SURFACE(3,1,((#35978,#35979),(#35980,#35981),(#35982,#35983),(#35984,
#35985)),.UNSPECIFIED.,.F.,.F.,.F.)
B_SPLINE_SURFACE_WITH_KNOTS((4,4),(2,2),(0.,1.),(0.,1.),.UNSPECIFIED.)
GEOMETRIC_REPRESENTATION_ITEM()
RATIONAL_B_SPLINE_SURFACE(((1.,1.),(0.962057791684876,0.975189339715083),
(0.962057791684876,0.975189339715083),(1.,1.)))
REPRESENTATION_ITEM('')
SURFACE()
);
#231=(
BOUNDED_SURFACE()
B_SPLINE_SURFACE(3,1,((#35998,#35999,#36000,#36001),(#36002,#36003,#36004,
#36005),(#36006,#36007,#36008,#36009),(#36010,#36011,#36012,#36013)),
 .UNSPECIFIED.,.F.,.F.,.F.)
B_SPLINE_SURFACE_WITH_KNOTS((4,4),(2,1,1,2),(0.,0.152244424776119),(-0.000281365801619608,
0.,1.,1.001),.UNSPECIFIED.)
GEOMETRIC_REPRESENTATION_ITEM()
RATIONAL_B_SPLINE_SURFACE(((1.,1.,1.,1.),(0.999893154836255,0.999893154836255,
0.997693707102186,0.997693707102186),(0.999802576253004,0.999802576253004,
0.995738534439964,0.995738534439964),(0.999728264250248,0.999728264250248,
0.994134482013336,0.994134482013336)))
REPRESENTATION_ITEM('')
SURFACE()
);
#232=(
BOUNDED_SURFACE()
B_SPLINE_SURFACE(3,1,((#36027,#36028,#36029,#36030),(#36031,#36032,#36033,
#36034),(#36035,#36036,#36037,#36038),(#36039,#36040,#36041,#36042)),
 .UNSPECIFIED.,.F.,.F.,.F.)
B_SPLINE_SURFACE_WITH_KNOTS((4,4),(2,1,1,2),(0.847755575223896,1.),(-0.000269810410367957,
0.,1.,1.001),.UNSPECIFIED.)
GEOMETRIC_REPRESENTATION_ITEM()
RATIONAL_B_SPLINE_SURFACE(((0.999728264250248,0.999728264250248,0.994134482013336,
0.994134482013336),(0.999802576253004,0.999802576253004,0.995738534439964,
0.995738534439964),(0.999893154836255,0.999893154836255,0.997693707102186,
0.997693707102186),(1.,1.,1.,1.)))
REPRESENTATION_ITEM('')
SURFACE()
);
#233=(
BOUNDED_SURFACE()
B_SPLINE_SURFACE(3,1,((#36063,#36064),(#36065,#36066),(#36067,#36068),(#36069,
#36070)),.UNSPECIFIED.,.F.,.F.,.F.)
B_SPLINE_SURFACE_WITH_KNOTS((4,4),(2,2),(0.,0.365923648059291),(0.,1.),
 .UNSPECIFIED.)
GEOMETRIC_REPRESENTATION_ITEM()
RATIONAL_B_SPLINE_SURFACE(((1.,1.),(0.890422051062866,0.903699651104578),
(0.820941264947662,0.842637877186351),(0.79155764165439,0.816814678245319)))
REPRESENTATION_ITEM('')
SURFACE()
);
#234=(
BOUNDED_SURFACE()
B_SPLINE_SURFACE(3,1,((#36085,#36086),(#36087,#36088),(#36089,#36090),(#36091,
#36092)),.UNSPECIFIED.,.F.,.F.,.F.)
B_SPLINE_SURFACE_WITH_KNOTS((4,4),(2,2),(0.,1.),(0.,0.966044174191948),
 .UNSPECIFIED.)
GEOMETRIC_REPRESENTATION_ITEM()
RATIONAL_B_SPLINE_SURFACE(((1.,1.),(0.969175395688119,0.979160009526791),
(0.969175395688119,0.979160009526791),(1.,1.)))
REPRESENTATION_ITEM('')
SURFACE()
);
#235=(
BOUNDED_SURFACE()
B_SPLINE_SURFACE(3,1,((#36115,#36116),(#36117,#36118),(#36119,#36120),(#36121,
#36122)),.UNSPECIFIED.,.F.,.F.,.F.)
B_SPLINE_SURFACE_WITH_KNOTS((4,4),(2,2),(0.,1.),(0.,1.),.UNSPECIFIED.)
GEOMETRIC_REPRESENTATION_ITEM()
RATIONAL_B_SPLINE_SURFACE(((1.,1.),(0.97852393395982,0.98163056167315),
(0.97852393395982,0.98163056167315),(1.,1.)))
REPRESENTATION_ITEM('')
SURFACE()
);
#236=(
BOUNDED_SURFACE()
B_SPLINE_SURFACE(3,1,((#36137,#36138),(#36139,#36140),(#36141,#36142),(#36143,
#36144)),.UNSPECIFIED.,.F.,.F.,.F.)
B_SPLINE_SURFACE_WITH_KNOTS((4,4),(2,2),(0.,1.),(0.,0.960122375136112),
 .UNSPECIFIED.)
GEOMETRIC_REPRESENTATION_ITEM()
RATIONAL_B_SPLINE_SURFACE(((1.,1.),(0.969713710620478,0.979815735270679),
(0.969713710620478,0.979815735270679),(1.,1.)))
REPRESENTATION_ITEM('')
SURFACE()
);
#237=(
BOUNDED_SURFACE()
B_SPLINE_SURFACE(3,1,((#36167,#36168),(#36169,#36170),(#36171,#36172),(#36173,
#36174)),.UNSPECIFIED.,.F.,.F.,.F.)
B_SPLINE_SURFACE_WITH_KNOTS((4,4),(2,2),(0.,1.),(0.,1.),.UNSPECIFIED.)
GEOMETRIC_REPRESENTATION_ITEM()
RATIONAL_B_SPLINE_SURFACE(((1.,1.),(0.978523933959819,0.981630561673153),
(0.978523933959819,0.981630561673153),(1.,1.)))
REPRESENTATION_ITEM('')
SURFACE()
);
#238=(
BOUNDED_SURFACE()
B_SPLINE_SURFACE(3,1,((#36189,#36190),(#36191,#36192),(#36193,#36194),(#36195,
#36196)),.UNSPECIFIED.,.F.,.F.,.F.)
B_SPLINE_SURFACE_WITH_KNOTS((4,4),(2,2),(0.,1.),(0.,0.966044174191938),
 .UNSPECIFIED.)
GEOMETRIC_REPRESENTATION_ITEM()
RATIONAL_B_SPLINE_SURFACE(((1.,1.),(0.969175395688119,0.979160009526794),
(0.969175395688119,0.979160009526794),(1.,1.)))
REPRESENTATION_ITEM('')
SURFACE()
);
#239=(
BOUNDED_SURFACE()
B_SPLINE_SURFACE(3,1,((#36209,#36210),(#36211,#36212),(#36213,#36214),(#36215,
#36216)),.UNSPECIFIED.,.F.,.F.,.F.)
B_SPLINE_SURFACE_WITH_KNOTS((4,4),(2,2),(0.634076354292045,1.),(0.,1.),
 .UNSPECIFIED.)
GEOMETRIC_REPRESENTATION_ITEM()
RATIONAL_B_SPLINE_SURFACE(((0.791557642220827,0.816814678743122),(0.820941265840597,
0.842637877971089),(0.890422051766988,0.903699651723381),(1.,1.)))
REPRESENTATION_ITEM('')
SURFACE()
);
#240=(
BOUNDED_SURFACE()
B_SPLINE_SURFACE(3,2,((#38724,#38725,#38726),(#38727,#38728,#38729),(#38730,
#38731,#38732),(#38733,#38734,#38735),(#38736,#38737,#38738),(#38739,#38740,
#38741)),.UNSPECIFIED.,.F.,.F.,.F.)
B_SPLINE_SURFACE_WITH_KNOTS((4,2,4),(3,3),(7.24208658159082,7.54803410778265,
7.85398163397448),(0.,1.),.UNSPECIFIED.)
GEOMETRIC_REPRESENTATION_ITEM()
RATIONAL_B_SPLINE_SURFACE(((1.,0.913794834970588,1.),(1.,0.940095751976153,
1.),(1.,0.962067838102692,1.),(1.,0.992046010392396,1.),(1.,1.00005792034581,
1.),(1.,1.,1.)))
REPRESENTATION_ITEM('')
SURFACE()
);
#241=(
BOUNDED_SURFACE()
B_SPLINE_SURFACE(3,2,((#38904,#38905,#38906),(#38907,#38908,#38909),(#38910,
#38911,#38912),(#38913,#38914,#38915),(#38916,#38917,#38918),(#38919,#38920,
#38921)),.UNSPECIFIED.,.F.,.F.,.F.)
B_SPLINE_SURFACE_WITH_KNOTS((4,2,4),(3,3),(7.2420865815908,7.54803410778264,
7.85398163397448),(0.,1.),.UNSPECIFIED.)
GEOMETRIC_REPRESENTATION_ITEM()
RATIONAL_B_SPLINE_SURFACE(((1.,0.913794834970583,1.),(1.,0.94009575197619,
1.),(1.,0.962067838102636,1.),(1.,0.99204601039245,1.),(1.,1.00005792034577,
1.),(1.,1.,1.)))
REPRESENTATION_ITEM('')
SURFACE()
);
#242=(
BOUNDED_SURFACE()
B_SPLINE_SURFACE(3,2,((#39155,#39156,#39157),(#39158,#39159,#39160),(#39161,
#39162,#39163),(#39164,#39165,#39166),(#39167,#39168,#39169),(#39170,#39171,
#39172)),.UNSPECIFIED.,.F.,.F.,.F.)
B_SPLINE_SURFACE_WITH_KNOTS((4,2,4),(3,3),(7.24208658159082,7.54803410778265,
7.85398163397448),(0.,1.),.UNSPECIFIED.)
GEOMETRIC_REPRESENTATION_ITEM()
RATIONAL_B_SPLINE_SURFACE(((1.,0.913794834970588,1.),(1.,0.940095751976173,
1.),(1.,0.962067838102665,1.),(1.,0.992046010392423,1.),(1.,1.00005792034579,
1.),(1.,1.,1.)))
REPRESENTATION_ITEM('')
SURFACE()
);
#243=(
BOUNDED_SURFACE()
B_SPLINE_SURFACE(3,2,((#39243,#39244,#39245),(#39246,#39247,#39248),(#39249,
#39250,#39251),(#39252,#39253,#39254),(#39255,#39256,#39257),(#39258,#39259,
#39260)),.UNSPECIFIED.,.F.,.F.,.F.)
B_SPLINE_SURFACE_WITH_KNOTS((4,2,4),(3,3),(7.2420865815908,7.54803410778264,
7.85398163397448),(0.,1.),.UNSPECIFIED.)
GEOMETRIC_REPRESENTATION_ITEM()
RATIONAL_B_SPLINE_SURFACE(((1.,0.913794834970582,1.),(1.,0.94009575197617,
1.),(1.,0.962067838102664,1.),(1.,0.992046010392423,1.),(1.,1.00005792034579,
1.),(1.,1.,1.)))
REPRESENTATION_ITEM('')
SURFACE()
);
#248=B_SPLINE_SURFACE_WITH_KNOTS('',3,1,((#33564,#33565,#33566,#33567),
(#33568,#33569,#33570,#33571),(#33572,#33573,#33574,#33575),(#33576,#33577,
#33578,#33579),(#33580,#33581,#33582,#33583),(#33584,#33585,#33586,#33587),
(#33588,#33589,#33590,#33591),(#33592,#33593,#33594,#33595),(#33596,#33597,
#33598,#33599),(#33600,#33601,#33602,#33603),(#33604,#33605,#33606,#33607),
(#33608,#33609,#33610,#33611),(#33612,#33613,#33614,#33615),(#33616,#33617,
#33618,#33619),(#33620,#33621,#33622,#33623),(#33624,#33625,#33626,#33627)),
 .UNSPECIFIED.,.F.,.F.,.F.,(4,3,2,2,2,3,4),(2,1,1,2),(-0.00031432553449176,
0.,0.125,0.25,0.375,0.418191871014293,0.418392704999572),(-0.000189913748737528,
0.,1.,1.00033781779361),.UNSPECIFIED.);
#249=B_SPLINE_SURFACE_WITH_KNOTS('',3,1,((#33642,#33643,#33644,#33645),
(#33646,#33647,#33648,#33649),(#33650,#33651,#33652,#33653),(#33654,#33655,
#33656,#33657),(#33658,#33659,#33660,#33661),(#33662,#33663,#33664,#33665),
(#33666,#33667,#33668,#33669),(#33670,#33671,#33672,#33673),(#33674,#33675,
#33676,#33677),(#33678,#33679,#33680,#33681),(#33682,#33683,#33684,#33685),
(#33686,#33687,#33688,#33689),(#33690,#33691,#33692,#33693),(#33694,#33695,
#33696,#33697),(#33698,#33699,#33700,#33701),(#33702,#33703,#33704,#33705)),
 .UNSPECIFIED.,.F.,.F.,.F.,(4,3,2,2,2,3,4),(2,1,1,2),(-0.00221274313418469,
0.,0.25,0.5,0.75,1.,1.00210632487476),(-0.00205770015535969,0.,0.975652891172124,
0.976690614800578),.UNSPECIFIED.);
#250=B_SPLINE_SURFACE_WITH_KNOTS('',3,1,((#33724,#33725,#33726,#33727),
(#33728,#33729,#33730,#33731),(#33732,#33733,#33734,#33735),(#33736,#33737,
#33738,#33739),(#33740,#33741,#33742,#33743),(#33744,#33745,#33746,#33747),
(#33748,#33749,#33750,#33751),(#33752,#33753,#33754,#33755),(#33756,#33757,
#33758,#33759),(#33760,#33761,#33762,#33763),(#33764,#33765,#33766,#33767),
(#33768,#33769,#33770,#33771),(#33772,#33773,#33774,#33775),(#33776,#33777,
#33778,#33779),(#33780,#33781,#33782,#33783),(#33784,#33785,#33786,#33787)),
 .UNSPECIFIED.,.F.,.F.,.F.,(4,3,2,2,2,3,4),(2,1,1,2),(-0.00236149222569652,
0.,0.25,0.5,0.75,1.,1.00236149222657),(-0.00220329632355928,0.,1.,1.00136244470998),
 .UNSPECIFIED.);
#251=B_SPLINE_SURFACE_WITH_KNOTS('',3,1,((#33802,#33803,#33804,#33805),
(#33806,#33807,#33808,#33809),(#33810,#33811,#33812,#33813),(#33814,#33815,
#33816,#33817),(#33818,#33819,#33820,#33821),(#33822,#33823,#33824,#33825),
(#33826,#33827,#33828,#33829),(#33830,#33831,#33832,#33833),(#33834,#33835,
#33836,#33837),(#33838,#33839,#33840,#33841),(#33842,#33843,#33844,#33845),
(#33846,#33847,#33848,#33849),(#33850,#33851,#33852,#33853),(#33854,#33855,
#33856,#33857),(#33858,#33859,#33860,#33861),(#33862,#33863,#33864,#33865)),
 .UNSPECIFIED.,.F.,.F.,.F.,(4,3,2,2,2,3,4),(2,1,1,2),(-0.00193140008151945,
0.,0.25,0.5,0.75,1.,1.00183441898671),(-0.00178369340673476,0.,0.978636855822753,
0.979556967191144),.UNSPECIFIED.);
#252=B_SPLINE_SURFACE_WITH_KNOTS('',3,1,((#33884,#33885,#33886,#33887),
(#33888,#33889,#33890,#33891),(#33892,#33893,#33894,#33895),(#33896,#33897,
#33898,#33899),(#33900,#33901,#33902,#33903),(#33904,#33905,#33906,#33907),
(#33908,#33909,#33910,#33911),(#33912,#33913,#33914,#33915),(#33916,#33917,
#33918,#33919),(#33920,#33921,#33922,#33923),(#33924,#33925,#33926,#33927),
(#33928,#33929,#33930,#33931),(#33932,#33933,#33934,#33935),(#33936,#33937,
#33938,#33939),(#33940,#33941,#33942,#33943),(#33944,#33945,#33946,#33947)),
 .UNSPECIFIED.,.F.,.F.,.F.,(4,3,2,2,2,3,4),(2,1,1,2),(-0.00236149222579484,
0.,0.25,0.5,0.75,1.,1.00236149222666),(-0.00220329632365572,0.,1.,1.00131125111415),
 .UNSPECIFIED.);
#253=B_SPLINE_SURFACE_WITH_KNOTS('',3,1,((#33962,#33963,#33964,#33965),
(#33966,#33967,#33968,#33969),(#33970,#33971,#33972,#33973),(#33974,#33975,
#33976,#33977),(#33978,#33979,#33980,#33981),(#33982,#33983,#33984,#33985),
(#33986,#33987,#33988,#33989),(#33990,#33991,#33992,#33993),(#33994,#33995,
#33996,#33997),(#33998,#33999,#34000,#34001),(#34002,#34003,#34004,#34005),
(#34006,#34007,#34008,#34009),(#34010,#34011,#34012,#34013),(#34014,#34015,
#34016,#34017),(#34018,#34019,#34020,#34021),(#34022,#34023,#34024,#34025)),
 .UNSPECIFIED.,.F.,.F.,.F.,(4,3,2,2,2,3,4),(2,1,1,2),(-0.00224555441012961,
0.,0.25,0.5,0.75,1.,1.00213171827197),(-0.00209030173265073,0.,0.975652891172124,
0.97673425926222),.UNSPECIFIED.);
#254=B_SPLINE_SURFACE_WITH_KNOTS('',3,1,((#34044,#34045,#34046,#34047),
(#34048,#34049,#34050,#34051),(#34052,#34053,#34054,#34055),(#34056,#34057,
#34058,#34059),(#34060,#34061,#34062,#34063),(#34064,#34065,#34066,#34067),
(#34068,#34069,#34070,#34071),(#34072,#34073,#34074,#34075),(#34076,#34077,
#34078,#34079),(#34080,#34081,#34082,#34083),(#34084,#34085,#34086,#34087),
(#34088,#34089,#34090,#34091),(#34092,#34093,#34094,#34095),(#34096,#34097,
#34098,#34099),(#34100,#34101,#34102,#34103),(#34104,#34105,#34106,#34107)),
 .UNSPECIFIED.,.F.,.F.,.F.,(4,3,2,2,2,3,4),(2,1,1,2),(0.581437458849578,
0.581806922548263,0.625,0.75,0.875,1.,1.00037830613069),(-0.000375883807932015,
0.,1.,1.00034850475001),.UNSPECIFIED.);
#255=B_SPLINE_SURFACE_WITH_KNOTS('',3,3,((#34263,#34264,#34265,#34266,#34267,
#34268,#34269,#34270,#34271,#34272,#34273,#34274,#34275,#34276,#34277,#34278,
#34279,#34280,#34281,#34282,#34283,#34284,#34285,#34286,#34287,#34288,#34289,
#34290,#34291,#34292,#34293,#34294,#34295,#34296,#34297,#34298,#34299,#34300,
#34301,#34302,#34303,#34304,#34305,#34306,#34307,#34308,#34309,#34310,#34311,
#34312,#34313,#34314,#34315,#34316),(#34317,#34318,#34319,#34320,#34321,
#34322,#34323,#34324,#34325,#34326,#34327,#34328,#34329,#34330,#34331,#34332,
#34333,#34334,#34335,#34336,#34337,#34338,#34339,#34340,#34341,#34342,#34343,
#34344,#34345,#34346,#34347,#34348,#34349,#34350,#34351,#34352,#34353,#34354,
#34355,#34356,#34357,#34358,#34359,#34360,#34361,#34362,#34363,#34364,#34365,
#34366,#34367,#34368,#34369,#34370),(#34371,#34372,#34373,#34374,#34375,
#34376,#34377,#34378,#34379,#34380,#34381,#34382,#34383,#34384,#34385,#34386,
#34387,#34388,#34389,#34390,#34391,#34392,#34393,#34394,#34395,#34396,#34397,
#34398,#34399,#34400,#34401,#34402,#34403,#34404,#34405,#34406,#34407,#34408,
#34409,#34410,#34411,#34412,#34413,#34414,#34415,#34416,#34417,#34418,#34419,
#34420,#34421,#34422,#34423,#34424),(#34425,#34426,#34427,#34428,#34429,
#34430,#34431,#34432,#34433,#34434,#34435,#34436,#34437,#34438,#34439,#34440,
#34441,#34442,#34443,#34444,#34445,#34446,#34447,#34448,#34449,#34450,#34451,
#34452,#34453,#34454,#34455,#34456,#34457,#34458,#34459,#34460,#34461,#34462,
#34463,#34464,#34465,#34466,#34467,#34468,#34469,#34470,#34471,#34472,#34473,
#34474,#34475,#34476,#34477,#34478),(#34479,#34480,#34481,#34482,#34483,
#34484,#34485,#34486,#34487,#34488,#34489,#34490,#34491,#34492,#34493,#34494,
#34495,#34496,#34497,#34498,#34499,#34500,#34501,#34502,#34503,#34504,#34505,
#34506,#34507,#34508,#34509,#34510,#34511,#34512,#34513,#34514,#34515,#34516,
#34517,#34518,#34519,#34520,#34521,#34522,#34523,#34524,#34525,#34526,#34527,
#34528,#34529,#34530,#34531,#34532),(#34533,#34534,#34535,#34536,#34537,
#34538,#34539,#34540,#34541,#34542,#34543,#34544,#34545,#34546,#34547,#34548,
#34549,#34550,#34551,#34552,#34553,#34554,#34555,#34556,#34557,#34558,#34559,
#34560,#34561,#34562,#34563,#34564,#34565,#34566,#34567,#34568,#34569,#34570,
#34571,#34572,#34573,#34574,#34575,#34576,#34577,#34578,#34579,#34580,#34581,
#34582,#34583,#34584,#34585,#34586),(#34587,#34588,#34589,#34590,#34591,
#34592,#34593,#34594,#34595,#34596,#34597,#34598,#34599,#34600,#34601,#34602,
#34603,#34604,#34605,#34606,#34607,#34608,#34609,#34610,#34611,#34612,#34613,
#34614,#34615,#34616,#34617,#34618,#34619,#34620,#34621,#34622,#34623,#34624,
#34625,#34626,#34627,#34628,#34629,#34630,#34631,#34632,#34633,#34634,#34635,
#34636,#34637,#34638,#34639,#34640),(#34641,#34642,#34643,#34644,#34645,
#34646,#34647,#34648,#34649,#34650,#34651,#34652,#34653,#34654,#34655,#34656,
#34657,#34658,#34659,#34660,#34661,#34662,#34663,#34664,#34665,#34666,#34667,
#34668,#34669,#34670,#34671,#34672,#34673,#34674,#34675,#34676,#34677,#34678,
#34679,#34680,#34681,#34682,#34683,#34684,#34685,#34686,#34687,#34688,#34689,
#34690,#34691,#34692,#34693,#34694),(#34695,#34696,#34697,#34698,#34699,
#34700,#34701,#34702,#34703,#34704,#34705,#34706,#34707,#34708,#34709,#34710,
#34711,#34712,#34713,#34714,#34715,#34716,#34717,#34718,#34719,#34720,#34721,
#34722,#34723,#34724,#34725,#34726,#34727,#34728,#34729,#34730,#34731,#34732,
#34733,#34734,#34735,#34736,#34737,#34738,#34739,#34740,#34741,#34742,#34743,
#34744,#34745,#34746,#34747,#34748),(#34749,#34750,#34751,#34752,#34753,
#34754,#34755,#34756,#34757,#34758,#34759,#34760,#34761,#34762,#34763,#34764,
#34765,#34766,#34767,#34768,#34769,#34770,#34771,#34772,#34773,#34774,#34775,
#34776,#34777,#34778,#34779,#34780,#34781,#34782,#34783,#34784,#34785,#34786,
#34787,#34788,#34789,#34790,#34791,#34792,#34793,#34794,#34795,#34796,#34797,
#34798,#34799,#34800,#34801,#34802),(#34803,#34804,#34805,#34806,#34807,
#34808,#34809,#34810,#34811,#34812,#34813,#34814,#34815,#34816,#34817,#34818,
#34819,#34820,#34821,#34822,#34823,#34824,#34825,#34826,#34827,#34828,#34829,
#34830,#34831,#34832,#34833,#34834,#34835,#34836,#34837,#34838,#34839,#34840,
#34841,#34842,#34843,#34844,#34845,#34846,#34847,#34848,#34849,#34850,#34851,
#34852,#34853,#34854,#34855,#34856),(#34857,#34858,#34859,#34860,#34861,
#34862,#34863,#34864,#34865,#34866,#34867,#34868,#34869,#34870,#34871,#34872,
#34873,#34874,#34875,#34876,#34877,#34878,#34879,#34880,#34881,#34882,#34883,
#34884,#34885,#34886,#34887,#34888,#34889,#34890,#34891,#34892,#34893,#34894,
#34895,#34896,#34897,#34898,#34899,#34900,#34901,#34902,#34903,#34904,#34905,
#34906,#34907,#34908,#34909,#34910),(#34911,#34912,#34913,#34914,#34915,
#34916,#34917,#34918,#34919,#34920,#34921,#34922,#34923,#34924,#34925,#34926,
#34927,#34928,#34929,#34930,#34931,#34932,#34933,#34934,#34935,#34936,#34937,
#34938,#34939,#34940,#34941,#34942,#34943,#34944,#34945,#34946,#34947,#34948,
#34949,#34950,#34951,#34952,#34953,#34954,#34955,#34956,#34957,#34958,#34959,
#34960,#34961,#34962,#34963,#34964),(#34965,#34966,#34967,#34968,#34969,
#34970,#34971,#34972,#34973,#34974,#34975,#34976,#34977,#34978,#34979,#34980,
#34981,#34982,#34983,#34984,#34985,#34986,#34987,#34988,#34989,#34990,#34991,
#34992,#34993,#34994,#34995,#34996,#34997,#34998,#34999,#35000,#35001,#35002,
#35003,#35004,#35005,#35006,#35007,#35008,#35009,#35010,#35011,#35012,#35013,
#35014,#35015,#35016,#35017,#35018),(#35019,#35020,#35021,#35022,#35023,
#35024,#35025,#35026,#35027,#35028,#35029,#35030,#35031,#35032,#35033,#35034,
#35035,#35036,#35037,#35038,#35039,#35040,#35041,#35042,#35043,#35044,#35045,
#35046,#35047,#35048,#35049,#35050,#35051,#35052,#35053,#35054,#35055,#35056,
#35057,#35058,#35059,#35060,#35061,#35062,#35063,#35064,#35065,#35066,#35067,
#35068,#35069,#35070,#35071,#35072),(#35073,#35074,#35075,#35076,#35077,
#35078,#35079,#35080,#35081,#35082,#35083,#35084,#35085,#35086,#35087,#35088,
#35089,#35090,#35091,#35092,#35093,#35094,#35095,#35096,#35097,#35098,#35099,
#35100,#35101,#35102,#35103,#35104,#35105,#35106,#35107,#35108,#35109,#35110,
#35111,#35112,#35113,#35114,#35115,#35116,#35117,#35118,#35119,#35120,#35121,
#35122,#35123,#35124,#35125,#35126),(#35127,#35128,#35129,#35130,#35131,
#35132,#35133,#35134,#35135,#35136,#35137,#35138,#35139,#35140,#35141,#35142,
#35143,#35144,#35145,#35146,#35147,#35148,#35149,#35150,#35151,#35152,#35153,
#35154,#35155,#35156,#35157,#35158,#35159,#35160,#35161,#35162,#35163,#35164,
#35165,#35166,#35167,#35168,#35169,#35170,#35171,#35172,#35173,#35174,#35175,
#35176,#35177,#35178,#35179,#35180),(#35181,#35182,#35183,#35184,#35185,
#35186,#35187,#35188,#35189,#35190,#35191,#35192,#35193,#35194,#35195,#35196,
#35197,#35198,#35199,#35200,#35201,#35202,#35203,#35204,#35205,#35206,#35207,
#35208,#35209,#35210,#35211,#35212,#35213,#35214,#35215,#35216,#35217,#35218,
#35219,#35220,#35221,#35222,#35223,#35224,#35225,#35226,#35227,#35228,#35229,
#35230,#35231,#35232,#35233,#35234),(#35235,#35236,#35237,#35238,#35239,
#35240,#35241,#35242,#35243,#35244,#35245,#35246,#35247,#35248,#35249,#35250,
#35251,#35252,#35253,#35254,#35255,#35256,#35257,#35258,#35259,#35260,#35261,
#35262,#35263,#35264,#35265,#35266,#35267,#35268,#35269,#35270,#35271,#35272,
#35273,#35274,#35275,#35276,#35277,#35278,#35279,#35280,#35281,#35282,#35283,
#35284,#35285,#35286,#35287,#35288),(#35289,#35290,#35291,#35292,#35293,
#35294,#35295,#35296,#35297,#35298,#35299,#35300,#35301,#35302,#35303,#35304,
#35305,#35306,#35307,#35308,#35309,#35310,#35311,#35312,#35313,#35314,#35315,
#35316,#35317,#35318,#35319,#35320,#35321,#35322,#35323,#35324,#35325,#35326,
#35327,#35328,#35329,#35330,#35331,#35332,#35333,#35334,#35335,#35336,#35337,
#35338,#35339,#35340,#35341,#35342),(#35343,#35344,#35345,#35346,#35347,
#35348,#35349,#35350,#35351,#35352,#35353,#35354,#35355,#35356,#35357,#35358,
#35359,#35360,#35361,#35362,#35363,#35364,#35365,#35366,#35367,#35368,#35369,
#35370,#35371,#35372,#35373,#35374,#35375,#35376,#35377,#35378,#35379,#35380,
#35381,#35382,#35383,#35384,#35385,#35386,#35387,#35388,#35389,#35390,#35391,
#35392,#35393,#35394,#35395,#35396),(#35397,#35398,#35399,#35400,#35401,
#35402,#35403,#35404,#35405,#35406,#35407,#35408,#35409,#35410,#35411,#35412,
#35413,#35414,#35415,#35416,#35417,#35418,#35419,#35420,#35421,#35422,#35423,
#35424,#35425,#35426,#35427,#35428,#35429,#35430,#35431,#35432,#35433,#35434,
#35435,#35436,#35437,#35438,#35439,#35440,#35441,#35442,#35443,#35444,#35445,
#35446,#35447,#35448,#35449,#35450),(#35451,#35452,#35453,#35454,#35455,
#35456,#35457,#35458,#35459,#35460,#35461,#35462,#35463,#35464,#35465,#35466,
#35467,#35468,#35469,#35470,#35471,#35472,#35473,#35474,#35475,#35476,#35477,
#35478,#35479,#35480,#35481,#35482,#35483,#35484,#35485,#35486,#35487,#35488,
#35489,#35490,#35491,#35492,#35493,#35494,#35495,#35496,#35497,#35498,#35499,
#35500,#35501,#35502,#35503,#35504),(#35505,#35506,#35507,#35508,#35509,
#35510,#35511,#35512,#35513,#35514,#35515,#35516,#35517,#35518,#35519,#35520,
#35521,#35522,#35523,#35524,#35525,#35526,#35527,#35528,#35529,#35530,#35531,
#35532,#35533,#35534,#35535,#35536,#35537,#35538,#35539,#35540,#35541,#35542,
#35543,#35544,#35545,#35546,#35547,#35548,#35549,#35550,#35551,#35552,#35553,
#35554,#35555,#35556,#35557,#35558),(#35559,#35560,#35561,#35562,#35563,
#35564,#35565,#35566,#35567,#35568,#35569,#35570,#35571,#35572,#35573,#35574,
#35575,#35576,#35577,#35578,#35579,#35580,#35581,#35582,#35583,#35584,#35585,
#35586,#35587,#35588,#35589,#35590,#35591,#35592,#35593,#35594,#35595,#35596,
#35597,#35598,#35599,#35600,#35601,#35602,#35603,#35604,#35605,#35606,#35607,
#35608,#35609,#35610,#35611,#35612),(#35613,#35614,#35615,#35616,#35617,
#35618,#35619,#35620,#35621,#35622,#35623,#35624,#35625,#35626,#35627,#35628,
#35629,#35630,#35631,#35632,#35633,#35634,#35635,#35636,#35637,#35638,#35639,
#35640,#35641,#35642,#35643,#35644,#35645,#35646,#35647,#35648,#35649,#35650,
#35651,#35652,#35653,#35654,#35655,#35656,#35657,#35658,#35659,#35660,#35661,
#35662,#35663,#35664,#35665,#35666),(#35667,#35668,#35669,#35670,#35671,
#35672,#35673,#35674,#35675,#35676,#35677,#35678,#35679,#35680,#35681,#35682,
#35683,#35684,#35685,#35686,#35687,#35688,#35689,#35690,#35691,#35692,#35693,
#35694,#35695,#35696,#35697,#35698,#35699,#35700,#35701,#35702,#35703,#35704,
#35705,#35706,#35707,#35708,#35709,#35710,#35711,#35712,#35713,#35714,#35715,
#35716,#35717,#35718,#35719,#35720),(#35721,#35722,#35723,#35724,#35725,
#35726,#35727,#35728,#35729,#35730,#35731,#35732,#35733,#35734,#35735,#35736,
#35737,#35738,#35739,#35740,#35741,#35742,#35743,#35744,#35745,#35746,#35747,
#35748,#35749,#35750,#35751,#35752,#35753,#35754,#35755,#35756,#35757,#35758,
#35759,#35760,#35761,#35762,#35763,#35764,#35765,#35766,#35767,#35768,#35769,
#35770,#35771,#35772,#35773,#35774),(#35775,#35776,#35777,#35778,#35779,
#35780,#35781,#35782,#35783,#35784,#35785,#35786,#35787,#35788,#35789,#35790,
#35791,#35792,#35793,#35794,#35795,#35796,#35797,#35798,#35799,#35800,#35801,
#35802,#35803,#35804,#35805,#35806,#35807,#35808,#35809,#35810,#35811,#35812,
#35813,#35814,#35815,#35816,#35817,#35818,#35819,#35820,#35821,#35822,#35823,
#35824,#35825,#35826,#35827,#35828),(#35829,#35830,#35831,#35832,#35833,
#35834,#35835,#35836,#35837,#35838,#35839,#35840,#35841,#35842,#35843,#35844,
#35845,#35846,#35847,#35848,#35849,#35850,#35851,#35852,#35853,#35854,#35855,
#35856,#35857,#35858,#35859,#35860,#35861,#35862,#35863,#35864,#35865,#35866,
#35867,#35868,#35869,#35870,#35871,#35872,#35873,#35874,#35875,#35876,#35877,
#35878,#35879,#35880,#35881,#35882)),.UNSPECIFIED.,.F.,.F.,.F.,(4,3,3,3,
3,3,3,2,2,2,2,4),(4,3,3,3,3,3,3,3,3,3,3,3,3,3,3,2,2,2,2,4),(-0.01,0.,0.166384002763973,
0.200043514355487,0.333101812640448,0.400072323934008,0.500472422318454,
0.667828884642908,0.667927982169589,0.834482890734559,0.834643736071572,
0.99999999990215),(0.,0.167157083656276,0.174191460919259,0.25514637702534,
0.29512942780803,0.334147528089117,0.384392237472365,0.500992769272865,
0.571140699239784,0.667418852842405,0.667511712013671,0.671156010454595,
0.675688248486018,0.832859978993389,0.833653335891096,0.833768414018777,
0.833810652851698,0.999546262459356,0.999999999996918,1.00999999999673),
 .UNSPECIFIED.);
#256=B_SPLINE_SURFACE_WITH_KNOTS('',3,1,((#36395,#36396,#36397,#36398),
(#36399,#36400,#36401,#36402),(#36403,#36404,#36405,#36406),(#36407,#36408,
#36409,#36410),(#36411,#36412,#36413,#36414),(#36415,#36416,#36417,#36418),
(#36419,#36420,#36421,#36422),(#36423,#36424,#36425,#36426),(#36427,#36428,
#36429,#36430),(#36431,#36432,#36433,#36434),(#36435,#36436,#36437,#36438),
(#36439,#36440,#36441,#36442)),.UNSPECIFIED.,.F.,.F.,.F.,(4,3,2,3,4),(2,
1,1,2),(-0.00114028998203398,0.,0.5,1.,1.00102384459753),(0.0558751001225879,
0.0570163348599441,1.,1.00114002661809),.UNSPECIFIED.);
#257=B_SPLINE_SURFACE_WITH_KNOTS('',3,1,((#36469,#36470,#36471,#36472),
(#36473,#36474,#36475,#36476),(#36477,#36478,#36479,#36480),(#36481,#36482,
#36483,#36484),(#36485,#36486,#36487,#36488),(#36489,#36490,#36491,#36492),
(#36493,#36494,#36495,#36496),(#36497,#36498,#36499,#36500),(#36501,#36502,
#36503,#36504),(#36505,#36506,#36507,#36508),(#36509,#36510,#36511,#36512),
(#36513,#36514,#36515,#36516)),.UNSPECIFIED.,.F.,.F.,.F.,(4,3,2,3,4),(2,
1,1,2),(-0.00042130059479378,0.,0.5,1.,1.00042130059344),(0.0848938236597501,
0.0852822930529455,1.,1.00042026460836),.UNSPECIFIED.);
#258=B_SPLINE_SURFACE_WITH_KNOTS('',3,1,((#36543,#36544,#36545,#36546),
(#36547,#36548,#36549,#36550),(#36551,#36552,#36553,#36554),(#36555,#36556,
#36557,#36558),(#36559,#36560,#36561,#36562),(#36563,#36564,#36565,#36566),
(#36567,#36568,#36569,#36570),(#36571,#36572,#36573,#36574),(#36575,#36576,
#36577,#36578),(#36579,#36580,#36581,#36582),(#36583,#36584,#36585,#36586),
(#36587,#36588,#36589,#36590)),.UNSPECIFIED.,.F.,.F.,.F.,(4,3,2,3,4),(2,
1,1,2),(-0.00102384459755735,0.,0.5,1.,1.00110988099093),(0.0559048734390992,
0.0570163348598889,1.,1.00110970363768),.UNSPECIFIED.);
#259=B_SPLINE_SURFACE_WITH_KNOTS('',3,1,((#36614,#36615,#36616,#36617),
(#36618,#36619,#36620,#36621),(#36622,#36623,#36624,#36625),(#36626,#36627,
#36628,#36629),(#36630,#36631,#36632,#36633),(#36634,#36635,#36636,#36637),
(#36638,#36639,#36640,#36641),(#36642,#36643,#36644,#36645),(#36646,#36647,
#36648,#36649),(#36650,#36651,#36652,#36653),(#36654,#36655,#36656,#36657),
(#36658,#36659,#36660,#36661)),.UNSPECIFIED.,.F.,.F.,.F.,(4,3,2,3,4),(2,
1,1,2),(-0.00102384459755,0.,0.5,1.,1.00110774805047),(0.0559075428418175,
0.0570163348598913,1.,1.00110748137492),.UNSPECIFIED.);
#260=B_SPLINE_SURFACE_WITH_KNOTS('',3,1,((#36688,#36689,#36690,#36691),
(#36692,#36693,#36694,#36695),(#36696,#36697,#36698,#36699),(#36700,#36701,
#36702,#36703),(#36704,#36705,#36706,#36707),(#36708,#36709,#36710,#36711),
(#36712,#36713,#36714,#36715),(#36716,#36717,#36718,#36719),(#36720,#36721,
#36722,#36723),(#36724,#36725,#36726,#36727),(#36728,#36729,#36730,#36731),
(#36732,#36733,#36734,#36735)),.UNSPECIFIED.,.F.,.F.,.F.,(4,3,2,3,4),(2,
1,1,2),(-0.000421300593474756,0.,0.5,1.,1.00042130059483),(0.0848938236597613,
0.0852822930529412,1.,1.00042026460839),.UNSPECIFIED.);
#261=B_SPLINE_SURFACE_WITH_KNOTS('',3,1,((#36762,#36763,#36764,#36765),
(#36766,#36767,#36768,#36769),(#36770,#36771,#36772,#36773),(#36774,#36775,
#36776,#36777),(#36778,#36779,#36780,#36781),(#36782,#36783,#36784,#36785),
(#36786,#36787,#36788,#36789),(#36790,#36791,#36792,#36793),(#36794,#36795,
#36796,#36797),(#36798,#36799,#36800,#36801),(#36802,#36803,#36804,#36805),
(#36806,#36807,#36808,#36809)),.UNSPECIFIED.,.F.,.F.,.F.,(4,3,2,3,4),(2,
1,1,2),(-0.00114028998205408,0.,0.5,1.,1.00102384459758),(0.0558751001225738,
0.0570163348599441,1.,1.00114002661814),.UNSPECIFIED.);
#262=B_SPLINE_SURFACE_WITH_KNOTS('',3,1,((#36833,#36834,#36835,#36836),
(#36837,#36838,#36839,#36840),(#36841,#36842,#36843,#36844),(#36845,#36846,
#36847,#36848),(#36849,#36850,#36851,#36852),(#36853,#36854,#36855,#36856),
(#36857,#36858,#36859,#36860),(#36861,#36862,#36863,#36864),(#36865,#36866,
#36867,#36868),(#36869,#36870,#36871,#36872),(#36873,#36874,#36875,#36876),
(#36877,#36878,#36879,#36880)),.UNSPECIFIED.,.F.,.F.,.F.,(4,3,2,3,4),(2,
1,1,2),(-0.00102363639854971,0.,0.5,1.,1.00044073822443),(0.0558990032510512,
0.0570163348599174,1.,1.00110652324197),.UNSPECIFIED.);
#263=B_SPLINE_SURFACE_WITH_KNOTS('',3,1,((#36908,#36909,#36910,#36911),
(#36912,#36913,#36914,#36915),(#36916,#36917,#36918,#36919),(#36920,#36921,
#36922,#36923),(#36924,#36925,#36926,#36927),(#36928,#36929,#36930,#36931),
(#36932,#36933,#36934,#36935),(#36936,#36937,#36938,#36939),(#36940,#36941,
#36942,#36943),(#36944,#36945,#36946,#36947),(#36948,#36949,#36950,#36951),
(#36952,#36953,#36954,#36955)),.UNSPECIFIED.,.F.,.F.,.F.,(4,3,2,3,4),(2,
1,1,2),(-0.000421300593445888,0.,0.5,1.,1.0004213005948),(0.0848938236598966,
0.0852822930529578,1.,1.00042026460836),.UNSPECIFIED.);
#264=B_SPLINE_SURFACE_WITH_KNOTS('',3,1,((#36982,#36983,#36984,#36985),
(#36986,#36987,#36988,#36989),(#36990,#36991,#36992,#36993),(#36994,#36995,
#36996,#36997),(#36998,#36999,#37000,#37001),(#37002,#37003,#37004,#37005),
(#37006,#37007,#37008,#37009),(#37010,#37011,#37012,#37013),(#37014,#37015,
#37016,#37017),(#37018,#37019,#37020,#37021),(#37022,#37023,#37024,#37025),
(#37026,#37027,#37028,#37029)),.UNSPECIFIED.,.F.,.F.,.F.,(4,3,2,3,4),(2,
1,1,2),(-0.000391510227323989,0.,0.5,1.,1.00030873205263),(0.0567815833000114,
0.0571716035704101,1.,1.00039130192454),.UNSPECIFIED.);
#265=B_SPLINE_SURFACE_WITH_KNOTS('',3,1,((#37048,#37049,#37050,#37051),
(#37052,#37053,#37054,#37055),(#37056,#37057,#37058,#37059),(#37060,#37061,
#37062,#37063),(#37064,#37065,#37066,#37067),(#37068,#37069,#37070,#37071),
(#37072,#37073,#37074,#37075),(#37076,#37077,#37078,#37079),(#37080,#37081,
#37082,#37083),(#37084,#37085,#37086,#37087),(#37088,#37089,#37090,#37091),
(#37092,#37093,#37094,#37095)),.UNSPECIFIED.,.F.,.F.,.F.,(4,3,2,3,4),(2,
1,1,2),(-0.000391510227317498,0.,0.5,1.,1.00030873205267),(0.056781583300018,
0.0571716035704015,1.,1.00039130192453),.UNSPECIFIED.);
#266=B_SPLINE_SURFACE_WITH_KNOTS('',3,1,((#37117,#37118,#37119,#37120),
(#37121,#37122,#37123,#37124),(#37125,#37126,#37127,#37128),(#37129,#37130,
#37131,#37132),(#37133,#37134,#37135,#37136),(#37137,#37138,#37139,#37140),
(#37141,#37142,#37143,#37144),(#37145,#37146,#37147,#37148),(#37149,#37150,
#37151,#37152),(#37153,#37154,#37155,#37156),(#37157,#37158,#37159,#37160),
(#37161,#37162,#37163,#37164)),.UNSPECIFIED.,.F.,.F.,.F.,(4,3,2,3,4),(2,
1,1,2),(-0.000421300594797483,0.,0.5,1.,1.00042130059344),(0.0848938236598713,
0.08528229305296,1.,1.00042026460836),.UNSPECIFIED.);
#267=B_SPLINE_SURFACE_WITH_KNOTS('',3,1,((#37191,#37192,#37193,#37194),
(#37195,#37196,#37197,#37198),(#37199,#37200,#37201,#37202),(#37203,#37204,
#37205,#37206),(#37207,#37208,#37209,#37210),(#37211,#37212,#37213,#37214),
(#37215,#37216,#37217,#37218),(#37219,#37220,#37221,#37222),(#37223,#37224,
#37225,#37226),(#37227,#37228,#37229,#37230),(#37231,#37232,#37233,#37234),
(#37235,#37236,#37237,#37238)),.UNSPECIFIED.,.F.,.F.,.F.,(4,3,2,3,4),(2,
1,1,2),(-0.00102384459763704,0.,0.5,1.,1.00110774805053),(0.0559075428417994,
0.0570163348599251,1.,1.00110748137497),.UNSPECIFIED.);
#273=SHAPE_REPRESENTATION_RELATIONSHIP('SRR','None',#40007,#280);
#280=ADVANCED_BREP_SHAPE_REPRESENTATION('',(#183),#39957);
#288=STYLED_ITEM('',(#40046),#183);
#423=PLANE('',#18884);
#424=PLANE('',#18885);
#425=PLANE('',#18892);
#426=PLANE('',#18895);
#427=PLANE('',#18896);
#428=PLANE('',#18897);
#429=PLANE('',#18898);
#430=PLANE('',#18899);
#431=PLANE('',#18900);
#432=PLANE('',#18901);
#433=PLANE('',#18902);
#434=PLANE('',#18903);
#435=PLANE('',#18904);
#436=PLANE('',#19106);
#437=PLANE('',#19107);
#438=PLANE('',#19108);
#439=PLANE('',#19109);
#440=PLANE('',#19110);
#441=PLANE('',#19122);
#442=PLANE('',#19123);
#443=PLANE('',#19124);
#444=PLANE('',#19125);
#445=PLANE('',#19126);
#446=PLANE('',#19127);
#447=PLANE('',#19128);
#448=PLANE('',#19129);
#449=PLANE('',#19130);
#450=PLANE('',#19135);
#451=PLANE('',#19137);
#452=PLANE('',#19138);
#453=PLANE('',#19139);
#454=PLANE('',#19140);
#455=PLANE('',#19141);
#456=PLANE('',#19142);
#457=PLANE('',#19143);
#458=PLANE('',#19148);
#459=PLANE('',#19150);
#460=PLANE('',#19151);
#461=PLANE('',#19152);
#462=PLANE('',#19153);
#463=PLANE('',#19154);
#464=PLANE('',#19155);
#465=PLANE('',#19156);
#466=PLANE('',#19161);
#467=PLANE('',#19163);
#468=PLANE('',#19165);
#469=PLANE('',#19166);
#470=PLANE('',#19167);
#471=PLANE('',#19168);
#472=PLANE('',#19169);
#473=PLANE('',#19170);
#474=PLANE('',#19171);
#475=PLANE('',#19175);
#476=PLANE('',#19179);
#477=PLANE('',#19186);
#478=PLANE('',#19193);
#479=PLANE('',#19198);
#480=PLANE('',#19203);
#481=PLANE('',#19205);
#482=PLANE('',#19207);
#483=PLANE('',#19209);
#484=PLANE('',#19211);
#485=PLANE('',#19213);
#486=PLANE('',#19215);
#487=PLANE('',#19217);
#488=PLANE('',#19219);
#489=PLANE('',#19221);
#490=PLANE('',#19223);
#491=PLANE('',#19225);
#492=PLANE('',#19229);
#493=PLANE('',#19232);
#494=PLANE('',#19234);
#495=PLANE('',#19237);
#496=PLANE('',#19239);
#497=PLANE('',#19242);
#498=PLANE('',#19243);
#499=PLANE('',#19246);
#500=PLANE('',#19247);
#501=PLANE('',#19250);
#502=PLANE('',#19251);
#503=PLANE('',#19254);
#504=PLANE('',#19255);
#505=PLANE('',#19263);
#506=PLANE('',#19268);
#507=PLANE('',#19271);
#508=PLANE('',#19274);
#509=PLANE('',#19277);
#510=PLANE('',#19278);
#511=PLANE('',#19280);
#512=PLANE('',#19282);
#513=PLANE('',#19284);
#514=PLANE('',#19286);
#515=PLANE('',#19288);
#516=PLANE('',#19289);
#517=PLANE('',#19290);
#518=PLANE('',#19292);
#519=PLANE('',#19294);
#520=PLANE('',#19296);
#521=PLANE('',#19298);
#522=PLANE('',#19301);
#523=PLANE('',#19303);
#524=PLANE('',#19306);
#525=PLANE('',#19308);
#526=PLANE('',#19310);
#527=PLANE('',#19345);
#528=PLANE('',#19346);
#529=PLANE('',#19349);
#530=PLANE('',#19356);
#531=PLANE('',#19371);
#532=PLANE('',#19383);
#533=PLANE('',#19384);
#534=PLANE('',#19391);
#535=PLANE('',#19392);
#536=PLANE('',#19393);
#537=PLANE('',#19400);
#538=PLANE('',#19401);
#539=PLANE('',#19402);
#540=PLANE('',#19407);
#541=PLANE('',#19408);
#542=PLANE('',#19409);
#543=PLANE('',#19416);
#544=PLANE('',#19417);
#545=PLANE('',#19418);
#546=PLANE('',#19423);
#547=PLANE('',#19424);
#548=PLANE('',#19425);
#549=PLANE('',#19426);
#550=PLANE('',#19427);
#551=PLANE('',#19428);
#552=PLANE('',#19429);
#553=PLANE('',#19430);
#554=PLANE('',#19431);
#555=PLANE('',#19432);
#556=PLANE('',#19433);
#557=PLANE('',#19434);
#558=PLANE('',#19441);
#559=PLANE('',#19442);
#560=PLANE('',#19455);
#561=PLANE('',#19459);
#562=PLANE('',#19460);
#563=PLANE('',#19461);
#564=PLANE('',#19462);
#565=PLANE('',#19463);
#566=PLANE('',#19469);
#567=PLANE('',#19470);
#568=PLANE('',#19471);
#569=PLANE('',#19473);
#570=PLANE('',#19474);
#571=PLANE('',#19475);
#572=PLANE('',#19476);
#573=PLANE('',#19477);
#574=PLANE('',#19482);
#575=PLANE('',#19483);
#576=PLANE('',#19484);
#577=PLANE('',#19485);
#578=PLANE('',#19491);
#579=PLANE('',#19492);
#580=PLANE('',#19496);
#581=PLANE('',#19497);
#582=PLANE('',#19498);
#583=PLANE('',#19501);
#584=PLANE('',#19502);
#585=PLANE('',#19503);
#586=PLANE('',#19504);
#587=PLANE('',#19508);
#588=PLANE('',#19511);
#589=PLANE('',#19512);
#590=PLANE('',#19513);
#591=PLANE('',#19516);
#592=PLANE('',#19517);
#593=PLANE('',#19521);
#594=PLANE('',#19524);
#595=PLANE('',#19525);
#596=PLANE('',#19526);
#597=PLANE('',#19529);
#598=PLANE('',#19530);
#599=PLANE('',#19534);
#600=PLANE('',#19537);
#601=PLANE('',#19538);
#602=PLANE('',#19539);
#603=PLANE('',#19542);
#604=PLANE('',#19543);
#605=PLANE('',#19547);
#606=PLANE('',#19550);
#607=PLANE('',#19551);
#608=PLANE('',#19552);
#609=PLANE('',#19555);
#610=PLANE('',#19556);
#611=PLANE('',#19557);
#612=PLANE('',#19558);
#613=PLANE('',#19559);
#614=PLANE('',#19560);
#615=PLANE('',#19561);
#616=PLANE('',#19562);
#617=PLANE('',#19563);
#618=PLANE('',#19564);
#619=PLANE('',#19565);
#620=PLANE('',#19566);
#621=PLANE('',#19567);
#622=PLANE('',#19568);
#623=PLANE('',#19569);
#624=PLANE('',#19570);
#625=PLANE('',#19571);
#626=PLANE('',#19572);
#627=PLANE('',#19573);
#628=PLANE('',#19577);
#629=PLANE('',#19578);
#630=PLANE('',#19580);
#631=PLANE('',#19581);
#632=PLANE('',#19584);
#633=PLANE('',#19585);
#634=PLANE('',#19586);
#635=PLANE('',#19587);
#636=PLANE('',#19590);
#637=PLANE('',#19591);
#638=PLANE('',#19593);
#639=PLANE('',#19594);
#640=PLANE('',#19598);
#641=PLANE('',#19599);
#642=PLANE('',#19601);
#643=PLANE('',#19602);
#644=PLANE('',#19603);
#645=PLANE('',#19605);
#646=PLANE('',#19607);
#647=PLANE('',#19609);
#648=PLANE('',#19610);
#649=PLANE('',#19612);
#650=PLANE('',#19614);
#651=PLANE('',#19616);
#652=PLANE('',#19618);
#653=PLANE('',#19619);
#654=PLANE('',#19622);
#655=PLANE('',#19625);
#656=PLANE('',#19626);
#657=PLANE('',#19628);
#658=PLANE('',#19629);
#659=PLANE('',#19630);
#660=PLANE('',#19631);
#661=PLANE('',#19632);
#662=PLANE('',#19633);
#663=PLANE('',#19636);
#664=PLANE('',#19639);
#665=PLANE('',#19640);
#666=PLANE('',#19641);
#667=PLANE('',#19642);
#668=PLANE('',#19643);
#669=PLANE('',#19647);
#670=PLANE('',#19648);
#671=PLANE('',#19649);
#672=PLANE('',#19650);
#673=PLANE('',#19651);
#674=PLANE('',#19653);
#675=PLANE('',#19654);
#676=PLANE('',#19656);
#677=PLANE('',#19658);
#678=PLANE('',#19659);
#679=PLANE('',#19661);
#680=PLANE('',#19664);
#681=PLANE('',#19666);
#682=PLANE('',#19667);
#683=PLANE('',#19669);
#684=PLANE('',#19671);
#685=PLANE('',#19672);
#686=PLANE('',#19674);
#687=PLANE('',#19675);
#688=PLANE('',#19676);
#689=PLANE('',#19677);
#690=PLANE('',#19678);
#691=PLANE('',#19679);
#692=PLANE('',#19680);
#693=PLANE('',#19684);
#694=PLANE('',#19687);
#695=PLANE('',#19690);
#696=PLANE('',#19691);
#697=PLANE('',#19692);
#698=PLANE('',#19693);
#699=PLANE('',#19694);
#700=PLANE('',#19695);
#701=PLANE('',#19696);
#702=PLANE('',#19697);
#703=PLANE('',#19698);
#704=PLANE('',#19699);
#705=PLANE('',#19700);
#706=PLANE('',#19701);
#707=PLANE('',#19702);
#708=PLANE('',#19703);
#709=PLANE('',#19704);
#710=PLANE('',#19709);
#711=PLANE('',#19711);
#712=PLANE('',#19712);
#713=PLANE('',#19713);
#714=PLANE('',#19714);
#715=PLANE('',#19715);
#716=PLANE('',#19716);
#717=PLANE('',#19720);
#718=PLANE('',#19722);
#719=PLANE('',#19723);
#720=PLANE('',#19724);
#721=PLANE('',#19725);
#722=PLANE('',#19726);
#723=PLANE('',#19727);
#724=PLANE('',#19732);
#725=PLANE('',#19736);
#726=PLANE('',#19739);
#727=PLANE('',#19744);
#728=PLANE('',#19745);
#729=PLANE('',#19747);
#730=PLANE('',#19750);
#731=PLANE('',#19754);
#732=PLANE('',#19758);
#733=PLANE('',#19759);
#734=PLANE('',#19760);
#735=PLANE('',#19761);
#736=PLANE('',#19762);
#737=PLANE('',#19763);
#738=PLANE('',#19764);
#739=PLANE('',#19768);
#740=PLANE('',#19770);
#741=PLANE('',#19771);
#742=PLANE('',#19772);
#743=PLANE('',#19773);
#744=PLANE('',#19774);
#745=PLANE('',#19775);
#746=PLANE('',#19776);
#747=PLANE('',#19777);
#748=PLANE('',#19778);
#749=PLANE('',#19779);
#750=PLANE('',#19780);
#751=PLANE('',#19781);
#752=PLANE('',#19782);
#753=PLANE('',#19783);
#754=PLANE('',#19784);
#755=PLANE('',#19785);
#756=PLANE('',#19786);
#757=PLANE('',#19787);
#758=PLANE('',#19788);
#759=PLANE('',#19789);
#760=PLANE('',#19790);
#761=PLANE('',#19791);
#762=PLANE('',#19792);
#763=PLANE('',#19793);
#764=PLANE('',#19794);
#765=PLANE('',#19795);
#766=PLANE('',#19797);
#767=PLANE('',#19798);
#768=PLANE('',#19799);
#769=PLANE('',#19801);
#770=PLANE('',#19802);
#771=PLANE('',#19803);
#772=PLANE('',#19805);
#773=PLANE('',#19808);
#774=PLANE('',#19812);
#775=PLANE('',#19815);
#776=PLANE('',#19817);
#777=PLANE('',#19821);
#778=PLANE('',#19823);
#779=PLANE('',#19824);
#780=PLANE('',#19825);
#781=PLANE('',#19826);
#782=PLANE('',#19827);
#783=PLANE('',#19828);
#784=PLANE('',#19829);
#785=PLANE('',#19830);
#786=PLANE('',#19831);
#787=PLANE('',#19832);
#788=PLANE('',#19833);
#789=PLANE('',#19834);
#790=PLANE('',#19835);
#791=PLANE('',#19836);
#792=PLANE('',#19837);
#793=PLANE('',#19838);
#794=PLANE('',#19839);
#795=PLANE('',#19840);
#796=PLANE('',#19842);
#797=PLANE('',#19844);
#798=PLANE('',#19845);
#799=PLANE('',#19849);
#800=PLANE('',#19853);
#801=PLANE('',#19854);
#802=PLANE('',#19855);
#803=PLANE('',#19857);
#804=PLANE('',#19859);
#805=PLANE('',#19865);
#806=PLANE('',#19872);
#807=PLANE('',#19874);
#808=PLANE('',#19875);
#809=PLANE('',#19876);
#810=PLANE('',#19877);
#811=PLANE('',#19878);
#812=PLANE('',#19879);
#813=PLANE('',#19880);
#814=PLANE('',#19881);
#815=PLANE('',#19882);
#816=PLANE('',#19883);
#817=PLANE('',#19884);
#818=PLANE('',#19885);
#819=PLANE('',#19886);
#820=PLANE('',#19887);
#821=PLANE('',#19888);
#822=PLANE('',#19895);
#823=PLANE('',#19896);
#824=PLANE('',#19897);
#825=PLANE('',#19898);
#826=PLANE('',#19899);
#827=PLANE('',#19900);
#828=PLANE('',#19901);
#829=PLANE('',#19912);
#830=PLANE('',#19913);
#831=PLANE('',#19914);
#832=PLANE('',#19915);
#833=PLANE('',#19916);
#834=PLANE('',#19917);
#835=PLANE('',#19918);
#836=PLANE('',#19919);
#837=PLANE('',#19920);
#838=PLANE('',#19921);
#839=PLANE('',#19922);
#840=PLANE('',#19923);
#841=PLANE('',#19924);
#842=PLANE('',#19925);
#843=PLANE('',#19926);
#844=PLANE('',#19927);
#845=PLANE('',#19928);
#846=PLANE('',#19929);
#847=PLANE('',#19930);
#848=PLANE('',#19931);
#849=PLANE('',#19932);
#850=PLANE('',#19933);
#851=PLANE('',#19934);
#852=PLANE('',#19935);
#853=PLANE('',#19936);
#854=PLANE('',#19937);
#855=PLANE('',#19938);
#856=PLANE('',#19939);
#857=PLANE('',#19940);
#858=PLANE('',#19941);
#859=PLANE('',#19942);
#860=PLANE('',#19943);
#996=FACE_BOUND('',#6199,.T.);
#997=FACE_BOUND('',#6201,.T.);
#998=FACE_BOUND('',#6205,.T.);
#999=FACE_BOUND('',#6248,.T.);
#1000=FACE_BOUND('',#6364,.T.);
#1001=FACE_BOUND('',#6367,.T.);
#1002=FACE_BOUND('',#6369,.T.);
#1003=FACE_BOUND('',#6372,.T.);
#1004=FACE_BOUND('',#6386,.T.);
#1005=FACE_BOUND('',#6388,.T.);
#1006=FACE_BOUND('',#6390,.T.);
#1007=FACE_BOUND('',#6392,.T.);
#1008=FACE_BOUND('',#6466,.T.);
#1009=FACE_BOUND('',#6484,.T.);
#1010=FACE_BOUND('',#6485,.T.);
#1011=FACE_BOUND('',#6505,.T.);
#1012=FACE_BOUND('',#6550,.T.);
#1013=FACE_BOUND('',#6557,.T.);
#1014=FACE_BOUND('',#6560,.T.);
#1015=FACE_BOUND('',#6562,.T.);
#1016=FACE_BOUND('',#6569,.T.);
#1017=FACE_BOUND('',#6579,.T.);
#1018=FACE_BOUND('',#6585,.T.);
#1019=FACE_BOUND('',#6588,.T.);
#1020=FACE_BOUND('',#6594,.T.);
#1021=FACE_BOUND('',#6596,.T.);
#1022=FACE_BOUND('',#6606,.T.);
#1023=FACE_BOUND('',#6616,.T.);
#1024=FACE_BOUND('',#6626,.T.);
#1025=FACE_BOUND('',#6642,.T.);
#1026=FACE_BOUND('',#6644,.T.);
#1027=FACE_BOUND('',#6670,.T.);
#1028=FACE_BOUND('',#6688,.T.);
#1029=FACE_BOUND('',#6692,.T.);
#1030=FACE_BOUND('',#6704,.T.);
#1031=FACE_BOUND('',#6706,.T.);
#1032=FACE_BOUND('',#6708,.T.);
#1033=FACE_BOUND('',#6710,.T.);
#1034=FACE_BOUND('',#6712,.T.);
#1035=FACE_BOUND('',#6740,.T.);
#1036=FACE_BOUND('',#6748,.T.);
#1037=FACE_BOUND('',#6781,.T.);
#1038=FACE_BOUND('',#6818,.T.);
#1039=FACE_BOUND('',#6821,.T.);
#1040=FACE_BOUND('',#6822,.T.);
#1041=FACE_BOUND('',#6823,.T.);
#1042=FACE_BOUND('',#6824,.T.);
#1043=FACE_BOUND('',#6825,.T.);
#1044=FACE_BOUND('',#6843,.T.);
#1045=FACE_BOUND('',#6846,.T.);
#1046=FACE_BOUND('',#6849,.T.);
#1047=FACE_BOUND('',#6857,.T.);
#1048=FACE_BOUND('',#6860,.T.);
#1049=FACE_BOUND('',#6862,.T.);
#1050=FACE_BOUND('',#6877,.T.);
#1051=FACE_BOUND('',#6894,.T.);
#1052=FACE_BOUND('',#6898,.T.);
#1053=FACE_BOUND('',#6906,.T.);
#1054=FACE_BOUND('',#6930,.T.);
#1055=FACE_BOUND('',#6938,.T.);
#1056=FACE_BOUND('',#6943,.T.);
#1057=FACE_BOUND('',#6949,.T.);
#1058=FACE_BOUND('',#6953,.T.);
#1059=FACE_BOUND('',#6954,.T.);
#1060=FACE_BOUND('',#6967,.T.);
#1061=FACE_BOUND('',#6968,.T.);
#1062=FACE_BOUND('',#6969,.T.);
#1063=FACE_BOUND('',#6970,.T.);
#1118=B_SPLINE_CURVE_WITH_KNOTS('',3,(#30739,#30740,#30741,#30742,#30743,
#30744),.UNSPECIFIED.,.F.,.F.,(4,2,4),(-0.791676148264701,-0.372293977343492,
-9.65154153425599E-5),.UNSPECIFIED.);
#1119=B_SPLINE_CURVE_WITH_KNOTS('',3,(#30746,#30747,#30748,#30749,#30750,
#30751),.UNSPECIFIED.,.F.,.F.,(4,2,4),(1.00000001008845E-6,0.394087848699293,
0.7875399240535),.UNSPECIFIED.);
#1120=B_SPLINE_CURVE_WITH_KNOTS('',3,(#30769,#30770,#30771,#30772,#30773,
#30774),.UNSPECIFIED.,.F.,.F.,(4,2,4),(-1.2607282506686,-0.589657089902255,
-9.99999981265987E-7),.UNSPECIFIED.);
#1121=B_SPLINE_CURVE_WITH_KNOTS('',3,(#30776,#30777,#30778,#30779,#30780,
#30781),.UNSPECIFIED.,.F.,.F.,(4,2,4),(-1.20095340635985,-0.611306024392865,
-9.99999999029555E-7),.UNSPECIFIED.);
#1122=B_SPLINE_CURVE_WITH_KNOTS('',3,(#30782,#30783,#30784,#30785,#30786,
#30787),.UNSPECIFIED.,.F.,.F.,(4,2,4),(-1.38009654873525,-0.740783265368206,
-9.99999862293069E-7),.UNSPECIFIED.);
#1123=B_SPLINE_CURVE_WITH_KNOTS('',3,(#30835,#30836,#30837,#30838),
 .UNSPECIFIED.,.F.,.F.,(4,4),(-1.5577837123075,-1.08255868409364),
 .UNSPECIFIED.);
#1124=B_SPLINE_CURVE_WITH_KNOTS('',3,(#30841,#30842,#30843,#30844),
 .UNSPECIFIED.,.F.,.F.,(4,4),(-4.8771663186696,-4.4074212598598),
 .UNSPECIFIED.);
#1125=B_SPLINE_CURVE_WITH_KNOTS('',3,(#30850,#30851,#30852,#30853,#30854,
#30855,#30856,#30857),.UNSPECIFIED.,.F.,.F.,(4,2,2,4),(1.10266399002091,
1.49973808840737,2.99947617681474,3.96838445098593),.UNSPECIFIED.);
#1126=B_SPLINE_CURVE_WITH_KNOTS('',3,(#30861,#30862,#30863,#30864),
 .UNSPECIFIED.,.F.,.F.,(4,4),(3.95502240653836,4.90059859273432),
 .UNSPECIFIED.);
#1127=B_SPLINE_CURVE_WITH_KNOTS('',3,(#30868,#30869,#30870,#30871,#30872,
#30873),.UNSPECIFIED.,.F.,.F.,(4,2,4),(1.55848971014011,2.98315547534721,
4.87725449444892),.UNSPECIFIED.);
#1128=B_SPLINE_CURVE_WITH_KNOTS('',3,(#30878,#30879,#30880,#30881),
 .UNSPECIFIED.,.F.,.F.,(4,4),(-2.02935178929506,-1.08377694268274),
 .UNSPECIFIED.);
#1129=B_SPLINE_CURVE_WITH_KNOTS('',3,(#30895,#30896,#30897,#30898,#30899,
#30900),.UNSPECIFIED.,.F.,.F.,(4,2,4),(1.27063161726614,1.45139131523522,
1.5474010823708),.UNSPECIFIED.);
#1130=B_SPLINE_CURVE_WITH_KNOTS('',3,(#30904,#30905,#30906,#30907,#30908,
#30909),.UNSPECIFIED.,.F.,.F.,(4,2,4),(2.04697459142689,2.07719778912169,
2.13306764446534),.UNSPECIFIED.);
#1131=B_SPLINE_CURVE_WITH_KNOTS('',3,(#30913,#30914,#30915,#30916,#30917,
#30918),.UNSPECIFIED.,.F.,.F.,(4,2,4),(4.13426269446195,4.1901325498056,
4.22035574750039),.UNSPECIFIED.);
#1132=B_SPLINE_CURVE_WITH_KNOTS('',3,(#30921,#30922,#30923,#30924,#30925,
#30926),.UNSPECIFIED.,.F.,.F.,(4,2,4),(0.993862152161476,1.08987191929705,
1.27063161726614),.UNSPECIFIED.);
#1133=B_SPLINE_CURVE_WITH_KNOTS('',3,(#30956,#30957,#30958,#30959,#30960,
#30961,#30962,#30963,#30964,#30965,#30966,#30967,#30968,#30969,#30970,#30971,
#30972,#30973),.UNSPECIFIED.,.F.,.F.,(4,2,2,2,2,2,2,2,4),(-1.27702533132968,
-1.25572868727499,-1.16995330406695,-0.996929092471484,-0.823904880876014,
-0.650880669280543,-0.477856457685072,-0.392081074477042,-0.370784430421933),
 .UNSPECIFIED.);
#1134=B_SPLINE_CURVE_WITH_KNOTS('',3,(#30977,#30978,#30979,#30980,#30981,
#30982,#30983,#30984,#30985,#30986,#30987,#30988,#30989,#30990,#30991,#30992,
#30993,#30994),.UNSPECIFIED.,.F.,.F.,(4,2,2,2,2,2,2,2,4),(-2.9248350930817,
-2.90353844902701,-2.81776306581898,-2.64473885422351,-2.47171464262804,
-2.29869043103257,-2.1256662194371,-2.03989083622907,-2.01859419217395),
 .UNSPECIFIED.);
#1135=B_SPLINE_CURVE_WITH_KNOTS('',3,(#30999,#31000,#31001,#31002,#31003,
#31004,#31005,#31006,#31007,#31008,#31009,#31010,#31011,#31012,#31013,#31014,
#31015,#31016),.UNSPECIFIED.,.F.,.F.,(4,2,2,2,2,2,2,2,4),(-1.27702533132966,
-1.25572868727497,-1.16995330406694,-0.996929092471472,-0.823904880876004,
-0.650880669280535,-0.477856457685067,-0.392081074477038,-0.370784430421922),
 .UNSPECIFIED.);
#1136=B_SPLINE_CURVE_WITH_KNOTS('',3,(#31020,#31021,#31022,#31023,#31024,
#31025,#31026,#31027,#31028,#31029,#31030,#31031,#31032,#31033,#31034,#31035,
#31036,#31037),.UNSPECIFIED.,.F.,.F.,(4,2,2,2,2,2,2,2,4),(-2.92483509308168,
-2.90353844902699,-2.81776306581896,-2.64473885422349,-2.47171464262802,
-2.29869043103255,-2.12566621943708,-2.03989083622905,-2.01859419217394),
 .UNSPECIFIED.);
#1137=B_SPLINE_CURVE_WITH_KNOTS('',3,(#31044,#31045,#31046,#31047,#31048,
#31049),.UNSPECIFIED.,.F.,.F.,(4,2,4),(1.49165309308059,1.52025985898216,
1.82900497420274),.UNSPECIFIED.);
#1138=B_SPLINE_CURVE_WITH_KNOTS('',3,(#31053,#31054,#31055,#31056,#31057,
#31058),.UNSPECIFIED.,.F.,.F.,(4,2,4),(2.83826458115358,3.14700969637418,
3.17561646227572),.UNSPECIFIED.);
#1139=B_SPLINE_CURVE_WITH_KNOTS('',3,(#31062,#31063,#31064,#31065,#31066,
#31067,#31068,#31069),.UNSPECIFIED.,.F.,.F.,(4,2,2,4),(2.01859419217413,
2.03989083622903,2.12566621943706,2.2046980767185),.UNSPECIFIED.);
#1140=B_SPLINE_CURVE_WITH_KNOTS('',3,(#31072,#31073,#31074,#31075,#31076,
#31077,#31078,#31079),.UNSPECIFIED.,.F.,.F.,(4,2,2,4),(1.09092144678542,
1.16995330406693,1.25572868727496,1.27702533132984),.UNSPECIFIED.);
#1141=B_SPLINE_CURVE_WITH_KNOTS('',3,(#31083,#31084,#31085,#31086,#31087,
#31088,#31089,#31090,#31091,#31092,#31093,#31094,#31095,#31096,#31097,#31098,
#31099,#31100),.UNSPECIFIED.,.F.,.F.,(4,2,2,2,2,2,2,2,4),(-1.27702533132966,
-1.25572868727498,-1.16995330406695,-0.996929092471477,-0.823904880876007,
-0.650880669280538,-0.477856457685069,-0.392081074477039,-0.370784430421927),
 .UNSPECIFIED.);
#1142=B_SPLINE_CURVE_WITH_KNOTS('',3,(#31109,#31110,#31111,#31112,#31113,
#31114,#31115,#31116,#31117,#31118,#31119,#31120,#31121,#31122,#31123,#31124,
#31125,#31126),.UNSPECIFIED.,.F.,.F.,(4,2,2,2,2,2,2,2,4),(-1.27702533132965,
-1.25572868727496,-1.16995330406693,-0.99692909247146,-0.823904880875993,
-0.650880669280526,-0.47785645768506,-0.392081074477032,-0.370784430421916),
 .UNSPECIFIED.);
#1143=B_SPLINE_CURVE_WITH_KNOTS('',3,(#31130,#31131,#31132,#31133,#31134,
#31135,#31136,#31137,#31138,#31139,#31140,#31141,#31142,#31143,#31144,#31145,
#31146,#31147),.UNSPECIFIED.,.F.,.F.,(4,2,2,2,2,2,2,2,4),(-2.92483509308164,
-2.90353844902695,-2.81776306581892,-2.64473885422345,-2.47171464262799,
-2.29869043103252,-2.12566621943705,-2.03989083622902,-2.0185941921739),
 .UNSPECIFIED.);
#1144=B_SPLINE_CURVE_WITH_KNOTS('',3,(#31197,#31198,#31199,#31200,#31201,
#31202,#31203,#31204,#31205,#31206,#31207,#31208,#31209,#31210,#31211,#31212,
#31213,#31214),.UNSPECIFIED.,.F.,.F.,(4,2,2,2,2,2,2,2,4),(-2.92483509308168,
-2.90353844902699,-2.81776306581896,-2.64473885422349,-2.47171464262802,
-2.29869043103255,-2.12566621943708,-2.03989083622905,-2.01859419217394),
 .UNSPECIFIED.);
#1145=B_SPLINE_CURVE_WITH_KNOTS('',3,(#31223,#31224,#31225,#31226,#31227,
#31228,#31229,#31230,#31231,#31232),.UNSPECIFIED.,.F.,.F.,(4,2,2,2,4),(0.500868628985409,
0.735493341191987,0.896904927369324,1.05831651354666,1.26986694206134),
 .UNSPECIFIED.);
#1146=B_SPLINE_CURVE_WITH_KNOTS('',3,(#31233,#31234,#31235,#31236,#31237,
#31238,#31239,#31240,#31241,#31242),.UNSPECIFIED.,.F.,.F.,(4,2,2,2,4),(1.6584322305039,
1.91496011666266,2.10521778038795,2.29547544411323,2.60768377754927),
 .UNSPECIFIED.);
#1147=B_SPLINE_CURVE_WITH_KNOTS('',3,(#31252,#31253,#31254,#31255,#31256,
#31257,#31258,#31259,#31260,#31261,#31262,#31263),.UNSPECIFIED.,.F.,.F.,
(4,2,2,2,2,4),(-2.23899247185989,-2.23353118304087,-1.98720488286121,-1.74087858268154,
-1.48331632361342,-1.47375923154499),.UNSPECIFIED.);
#1148=B_SPLINE_CURVE_WITH_KNOTS('',3,(#31330,#31331,#31332,#31333,#31334,
#31335,#31336,#31337,#31338,#31339,#31340,#31341,#31342,#31343,#31344,#31345,
#31346,#31347,#31348,#31349,#31350,#31351,#31352,#31353),.UNSPECIFIED.,
 .F.,.F.,(4,2,2,2,2,2,2,2,2,2,2,4),(3.54201414503647,3.60917199339226,3.64693471091968,
3.6846974284471,3.70035540208751,3.71601337572793,3.7335287617438,3.75104414775967,
3.78450531236555,3.81796647697143,3.88488880618319,3.9103123168716),
 .UNSPECIFIED.);
#1149=B_SPLINE_CURVE_WITH_KNOTS('',3,(#31354,#31355,#31356,#31357,#31358,
#31359),.UNSPECIFIED.,.F.,.F.,(4,2,4),(-16.2126008937337,-16.1073352653066,
-15.971670557086),.UNSPECIFIED.);
#1150=B_SPLINE_CURVE_WITH_KNOTS('',3,(#31532,#31533,#31534,#31535,#31536,
#31537,#31538,#31539,#31540,#31541),.UNSPECIFIED.,.F.,.F.,(4,2,2,2,4),(0.,
0.223184802145918,0.439747194735359,0.656355638915093,0.879587963358382),
 .UNSPECIFIED.);
#1151=B_SPLINE_CURVE_WITH_KNOTS('',3,(#31543,#31544,#31545,#31546,#31547,
#31548),.UNSPECIFIED.,.F.,.F.,(4,2,4),(0.,0.160388841871916,0.315547520092146),
 .UNSPECIFIED.);
#1152=B_SPLINE_CURVE_WITH_KNOTS('',3,(#31552,#31553,#31554,#31555,#31556,
#31557),.UNSPECIFIED.,.F.,.F.,(4,2,4),(0.,0.151579443123173,0.307260734801231),
 .UNSPECIFIED.);
#1153=B_SPLINE_CURVE_WITH_KNOTS('',3,(#31559,#31560,#31561,#31562,#31563,
#31564,#31565,#31566,#31567,#31568),.UNSPECIFIED.,.F.,.F.,(4,2,2,2,4),(0.,
0.212152978397668,0.422051181763095,0.652730480685441,0.893650672439128),
 .UNSPECIFIED.);
#1154=B_SPLINE_CURVE_WITH_KNOTS('',3,(#31570,#31571,#31572,#31573,#31574,
#31575),.UNSPECIFIED.,.F.,.F.,(4,2,4),(0.,0.143871076035642,0.282736346863713),
 .UNSPECIFIED.);
#1155=B_SPLINE_CURVE_WITH_KNOTS('',3,(#31579,#31580,#31581,#31582,#31583,
#31584),.UNSPECIFIED.,.F.,.F.,(4,2,4),(0.,0.276923219658822,0.495895501945399),
 .UNSPECIFIED.);
#1156=B_SPLINE_CURVE_WITH_KNOTS('',3,(#31586,#31587,#31588,#31589,#31590,
#31591),.UNSPECIFIED.,.F.,.F.,(4,2,4),(-1.31438656188044,-0.675941586797486,
0.),.UNSPECIFIED.);
#1157=B_SPLINE_CURVE_WITH_KNOTS('',3,(#31599,#31600,#31601,#31602,#31603,
#31604),.UNSPECIFIED.,.F.,.F.,(4,2,4),(-1.31452379814346,-0.638512700577341,
-9.87344898062403E-7),.UNSPECIFIED.);
#1158=B_SPLINE_CURVE_WITH_KNOTS('',3,(#31606,#31607,#31608,#31609,#31610,
#31611),.UNSPECIFIED.,.F.,.F.,(4,2,4),(1.00970274276848E-6,0.207625682362454,
0.496418277299487),.UNSPECIFIED.);
#1159=B_SPLINE_CURVE_WITH_KNOTS('',3,(#31615,#31616,#31617,#31618,#31619,
#31620),.UNSPECIFIED.,.F.,.F.,(4,2,4),(1.00000002999262E-6,0.159334194743211,
0.282730318724299),.UNSPECIFIED.);
#1160=B_SPLINE_CURVE_WITH_KNOTS('',3,(#31622,#31623,#31624,#31625,#31626,
#31627,#31628,#31629),.UNSPECIFIED.,.F.,.F.,(4,2,2,4),(0.,0.414719851775387,
0.654098578320246,0.895378619929204),.UNSPECIFIED.);
#1161=B_SPLINE_CURVE_WITH_KNOTS('',3,(#31631,#31632,#31633,#31634,#31635,
#31636),.UNSPECIFIED.,.F.,.F.,(4,2,4),(0.,0.155726590263008,0.307315201685305),
 .UNSPECIFIED.);
#1162=B_SPLINE_CURVE_WITH_KNOTS('',3,(#31639,#31640,#31641,#31642,#31643,
#31644),.UNSPECIFIED.,.F.,.F.,(4,2,4),(0.,0.155122646177725,0.315476068796403),
 .UNSPECIFIED.);
#1163=B_SPLINE_CURVE_WITH_KNOTS('',3,(#31692,#31693,#31694,#31695,#31696,
#31697,#31698,#31699),.UNSPECIFIED.,.F.,.F.,(4,2,2,4),(-1.20146899372566,
-0.600846725288746,-0.240887418321441,0.),.UNSPECIFIED.);
#1164=B_SPLINE_CURVE_WITH_KNOTS('',3,(#31709,#31710,#31711,#31712,#31713,
#31714,#31715,#31716,#31717,#31718,#31719,#31720),.UNSPECIFIED.,.F.,.F.,
(4,2,2,2,2,4),(-1.49738934525104,-1.30249117565947,-1.11538918315606,-0.877104450222815,
-0.53567900892061,0.),.UNSPECIFIED.);
#1165=B_SPLINE_CURVE_WITH_KNOTS('',3,(#31732,#31733,#31734,#31735,#31736,
#31737,#31738,#31739,#31740,#31741,#31742,#31743,#31744,#31745,#31746,#31747,
#31748,#31749,#31750,#31751,#31752,#31753,#31754,#31755,#31756,#31757,#31758,
#31759,#31760,#31761,#31762,#31763,#31764,#31765),.UNSPECIFIED.,.F.,.F.,
(4,3,3,3,3,3,3,3,3,3,3,4),(0.0428656554157575,0.13679913434849,0.230446688335681,
0.326640852293718,0.419914650723107,0.513145592287718,0.606396601892675,
0.699730411778525,0.793321120935319,0.887097673400666,0.981233417826358,
0.999999999999973),.UNSPECIFIED.);
#1166=B_SPLINE_CURVE_WITH_KNOTS('',3,(#31766,#31767,#31768,#31769,#31770,
#31771),.UNSPECIFIED.,.F.,.F.,(4,2,4),(-0.981740143086555,-0.521961463111386,
0.),.UNSPECIFIED.);
#1167=B_SPLINE_CURVE_WITH_KNOTS('',3,(#31787,#31788,#31789,#31790,#31791,
#31792),.UNSPECIFIED.,.F.,.F.,(4,2,4),(-0.133416986009087,-0.0667110879136702,
-5.1910372269785E-6),.UNSPECIFIED.);
#1168=B_SPLINE_CURVE_WITH_KNOTS('',3,(#31805,#31806,#31807,#31808,#31809,
#31810),.UNSPECIFIED.,.F.,.F.,(4,2,4),(9.99999978184638E-7,0.649745648357186,
1.35925358102172),.UNSPECIFIED.);
#1169=B_SPLINE_CURVE_WITH_KNOTS('',3,(#31812,#31813,#31814,#31815,#31816,
#31817),.UNSPECIFIED.,.F.,.F.,(4,2,4),(0.,0.394929358834096,0.789859724379243),
 .UNSPECIFIED.);
#1170=B_SPLINE_CURVE_WITH_KNOTS('',3,(#31819,#31820,#31821,#31822,#31823,
#31824),.UNSPECIFIED.,.F.,.F.,(4,2,4),(-0.203128010071857,-0.10156462327841,
-1.00000000322065E-6),.UNSPECIFIED.);
#1171=B_SPLINE_CURVE_WITH_KNOTS('',3,(#31825,#31826,#31827,#31828,#31829,
#31830),.UNSPECIFIED.,.F.,.F.,(4,2,4),(1.49144212074817,1.98945111447353,
2.50597513326044),.UNSPECIFIED.);
#1172=B_SPLINE_CURVE_WITH_KNOTS('',3,(#31841,#31842,#31843,#31844,#31845,
#31846,#31847,#31848,#31849,#31850,#31851,#31852),.UNSPECIFIED.,.F.,.F.,
(4,2,2,2,2,4),(-1.49732839853819,-0.998653556005853,-0.620289629858932,
-0.365781376210274,-0.185635579466019,0.),.UNSPECIFIED.);
#1173=B_SPLINE_CURVE_WITH_KNOTS('',3,(#31866,#31867,#31868,#31869,#31870,
#31871),.UNSPECIFIED.,.F.,.F.,(4,2,4),(-0.991698835186327,-0.464861205496753,
0.),.UNSPECIFIED.);
#1174=B_SPLINE_CURVE_WITH_KNOTS('',3,(#31872,#31873,#31874,#31875,#31876,
#31877,#31878,#31879,#31880,#31881,#31882,#31883,#31884,#31885,#31886,#31887,
#31888,#31889,#31890,#31891,#31892,#31893,#31894,#31895,#31896,#31897,#31898,
#31899,#31900,#31901,#31902,#31903,#31904,#31905),.UNSPECIFIED.,.F.,.F.,
(4,3,3,3,3,3,3,3,3,3,3,4),(1.80628081936085E-16,0.0941353335519054,0.187946410909733,
0.284092730197232,0.377429083695201,0.470683798845207,0.563919701125802,
0.657199745463011,0.750681328969369,0.844317073902783,0.938269188721954,
0.957116965209728),.UNSPECIFIED.);
#1175=B_SPLINE_CURVE_WITH_KNOTS('',3,(#31917,#31918,#31919,#31920,#31921,
#31922,#31923,#31924,#31925,#31926),.UNSPECIFIED.,.F.,.F.,(4,2,2,2,4),(-1.49714596644318,
-1.13508004089971,-0.778547165757211,-0.375322448427936,0.),
 .UNSPECIFIED.);
#1176=B_SPLINE_CURVE_WITH_KNOTS('',3,(#31940,#31941,#31942,#31943,#31944,
#31945,#31946,#31947,#31948,#31949,#31950,#31951,#31952,#31953,#31954,#31955,
#31956,#31957,#31958,#31959,#31960,#31961,#31962,#31963,#31964,#31965,#31966,
#31967,#31968,#31969,#31970,#31971,#31972,#31973),.UNSPECIFIED.,.F.,.F.,
(4,3,3,3,3,3,3,3,3,3,3,4),(0.0426189802653293,0.136532611271545,0.230169834401958,
0.326398605101725,0.41967855846039,0.512918289440782,0.606178554076897,
0.699519886497026,0.793111915273064,0.886884192924315,0.9810061634702,1.00000000000009),
 .UNSPECIFIED.);
#1177=B_SPLINE_CURVE_WITH_KNOTS('',3,(#31974,#31975,#31976,#31977,#31978,
#31979),.UNSPECIFIED.,.F.,.F.,(4,2,4),(-0.970835171563933,-0.515920953006016,
0.),.UNSPECIFIED.);
#1178=B_SPLINE_CURVE_WITH_KNOTS('',3,(#31991,#31992,#31993,#31994,#31995,
#31996,#31997,#31998,#31999,#32000),.UNSPECIFIED.,.F.,.F.,(4,2,2,2,4),(-1.49810739332486,
-1.34911047074889,-0.620300163072249,-0.284723572909162,0.),
 .UNSPECIFIED.);
#1179=B_SPLINE_CURVE_WITH_KNOTS('',3,(#32012,#32013,#32014,#32015,#32016,
#32017,#32018,#32019,#32020,#32021),.UNSPECIFIED.,.F.,.F.,(4,2,2,2,4),(-1.49747557017719,
-1.09769840149384,-0.714928203148522,-0.377751581416893,0.),
 .UNSPECIFIED.);
#1180=B_SPLINE_CURVE_WITH_KNOTS('',3,(#32472,#32473,#32474,#32475,#32476,
#32477),.UNSPECIFIED.,.F.,.F.,(4,2,4),(-0.981606280218853,-0.521850501049393,
0.),.UNSPECIFIED.);
#1181=B_SPLINE_CURVE_WITH_KNOTS('',3,(#32482,#32483,#32484,#32485,#32486,
#32487),.UNSPECIFIED.,.F.,.F.,(4,2,4),(-1.26025824344159,-0.587863989490026,
-9.99999988926525E-7),.UNSPECIFIED.);
#1182=B_SPLINE_CURVE_WITH_KNOTS('',3,(#32493,#32494,#32495,#32496,#32497,
#32498),.UNSPECIFIED.,.F.,.F.,(4,2,4),(-1.20095164808206,-0.601230313153804,
-9.9999999636502E-7),.UNSPECIFIED.);
#1183=B_SPLINE_CURVE_WITH_KNOTS('',3,(#32503,#32504,#32505,#32506,#32507,
#32508),.UNSPECIFIED.,.F.,.F.,(4,2,4),(-0.979787980011625,-0.459672473975673,
0.),.UNSPECIFIED.);
#1184=B_SPLINE_CURVE_WITH_KNOTS('',3,(#32509,#32510,#32511,#32512,#32513,
#32514),.UNSPECIFIED.,.F.,.F.,(4,2,4),(-1.20447770770638,-0.642888512151301,
-9.99999843598331E-7),.UNSPECIFIED.);
#1185=B_SPLINE_CURVE_WITH_KNOTS('',3,(#32520,#32521,#32522,#32523,#32524,
#32525),.UNSPECIFIED.,.F.,.F.,(4,2,4),(-1.27174362759288,-0.592870374348338,
-9.99999989116678E-7),.UNSPECIFIED.);
#1186=B_SPLINE_CURVE_WITH_KNOTS('',3,(#32531,#32532,#32533,#32534,#32535,
#32536),.UNSPECIFIED.,.F.,.F.,(4,2,4),(-1.20095492134397,-0.600247667823548,
-9.99999999029555E-7),.UNSPECIFIED.);
#1187=B_SPLINE_CURVE_WITH_KNOTS('',3,(#32538,#32539,#32540,#32541,#32542,
#32543),.UNSPECIFIED.,.F.,.F.,(4,2,4),(-1.1923457836634,-0.636112763433397,
-9.9999983627086E-7),.UNSPECIFIED.);
#1188=B_SPLINE_CURVE_WITH_KNOTS('',3,(#32558,#32559,#32560,#32561,#32562,
#32563,#32564,#32565,#32566,#32567),.UNSPECIFIED.,.F.,.F.,(4,2,2,2,4),(-0.811018179914924,
-0.664454692598758,-0.572774590965832,-0.394840790088965,0.),
 .UNSPECIFIED.);
#1189=B_SPLINE_CURVE_WITH_KNOTS('',3,(#32572,#32573,#32574,#32575,#32576,
#32577),.UNSPECIFIED.,.F.,.F.,(4,2,4),(-1.46761581044962,-0.679870711727504,
-9.99999985706879E-7),.UNSPECIFIED.);
#1190=B_SPLINE_CURVE_WITH_KNOTS('',3,(#32583,#32584,#32585,#32586,#32587,
#32588),.UNSPECIFIED.,.F.,.F.,(4,2,4),(-1.20095336165845,-0.589756404209531,
-9.99999999465967E-7),.UNSPECIFIED.);
#1191=B_SPLINE_CURVE_WITH_KNOTS('',3,(#32591,#32592,#32593,#32594,#32595,
#32596),.UNSPECIFIED.,.F.,.F.,(4,2,4),(-1.25535652774483,-0.666244907753614,
-1.33226762955019E-15),.UNSPECIFIED.);
#1192=B_SPLINE_CURVE_WITH_KNOTS('',3,(#32599,#32600,#32601,#32602,#32603,
#32604),.UNSPECIFIED.,.F.,.F.,(4,2,4),(-0.990141997994943,-0.466167882443553,
-9.99999943980542E-7),.UNSPECIFIED.);
#1193=B_SPLINE_CURVE_WITH_KNOTS('',3,(#32608,#32609,#32610,#32611,#32612,
#32613,#32614,#32615),.UNSPECIFIED.,.F.,.F.,(4,2,2,4),(9.99977311176857E-7,
0.108585823432627,0.151061815337212,0.21421875376243),.UNSPECIFIED.);
#1194=B_SPLINE_CURVE_WITH_KNOTS('',3,(#32619,#32620,#32621,#32622,#32623,
#32624),.UNSPECIFIED.,.F.,.F.,(4,2,4),(0.,0.393385683687471,0.787575248868537),
 .UNSPECIFIED.);
#1195=B_SPLINE_CURVE_WITH_KNOTS('',3,(#32628,#32629,#32630,#32631,#32632,
#32633),.UNSPECIFIED.,.F.,.F.,(4,2,4),(1.00000001804486E-6,0.394931365545149,
0.789860724379214),.UNSPECIFIED.);
#1196=B_SPLINE_CURVE_WITH_KNOTS('',3,(#32635,#32636,#32637,#32638,#32639,
#32640),.UNSPECIFIED.,.F.,.F.,(4,2,4),(0.,0.399659978932644,0.799320001325682),
 .UNSPECIFIED.);
#1197=B_SPLINE_CURVE_WITH_KNOTS('',3,(#32642,#32643,#32644,#32645,#32646,
#32647),.UNSPECIFIED.,.F.,.F.,(4,2,4),(0.,0.333003326126868,0.666006652253743),
 .UNSPECIFIED.);
#1198=B_SPLINE_CURVE_WITH_KNOTS('',3,(#32649,#32650,#32651,#32652,#32653,
#32654),.UNSPECIFIED.,.F.,.F.,(4,2,4),(0.,0.396114271378094,0.792228542747862),
 .UNSPECIFIED.);
#1199=B_SPLINE_CURVE_WITH_KNOTS('',3,(#32656,#32657,#32658,#32659,#32660,
#32661),.UNSPECIFIED.,.F.,.F.,(4,2,4),(0.,0.333003326126872,0.666006652253742),
 .UNSPECIFIED.);
#1200=B_SPLINE_CURVE_WITH_KNOTS('',3,(#32662,#32663,#32664,#32665,#32666,
#32667),.UNSPECIFIED.,.F.,.F.,(4,2,4),(0.,0.399660022402238,0.799320001325697),
 .UNSPECIFIED.);
#1201=B_SPLINE_CURVE_WITH_KNOTS('',3,(#32669,#32670,#32671,#32672,#32673,
#32674),.UNSPECIFIED.,.F.,.F.,(4,2,4),(4.61607433837006E-5,0.394237334279624,
0.787624623042523),.UNSPECIFIED.);
#1202=B_SPLINE_CURVE_WITH_KNOTS('',3,(#32675,#32676,#32677,#32678,#32679,
#32680),.UNSPECIFIED.,.F.,.F.,(4,2,4),(0.,0.393451752374059,0.78755756073778),
 .UNSPECIFIED.);
#1203=B_SPLINE_CURVE_WITH_KNOTS('',3,(#32684,#32685,#32686,#32687,#32688,
#32689),.UNSPECIFIED.,.F.,.F.,(4,2,4),(1.0000000167154E-6,0.394931365545151,
0.78986072437921),.UNSPECIFIED.);
#1204=B_SPLINE_CURVE_WITH_KNOTS('',3,(#32691,#32692,#32693,#32694,#32695,
#32696),.UNSPECIFIED.,.F.,.F.,(4,2,4),(0.,0.399659978932271,0.799320001325689),
 .UNSPECIFIED.);
#1205=B_SPLINE_CURVE_WITH_KNOTS('',3,(#32698,#32699,#32700,#32701,#32702,
#32703),.UNSPECIFIED.,.F.,.F.,(4,2,4),(0.,0.333003326126866,0.666006652253748),
 .UNSPECIFIED.);
#1206=B_SPLINE_CURVE_WITH_KNOTS('',3,(#32705,#32706,#32707,#32708,#32709,
#32710),.UNSPECIFIED.,.F.,.F.,(4,2,4),(0.,0.396114271378084,0.79222854274787),
 .UNSPECIFIED.);
#1207=B_SPLINE_CURVE_WITH_KNOTS('',3,(#32712,#32713,#32714,#32715,#32716,
#32717),.UNSPECIFIED.,.F.,.F.,(4,2,4),(0.,0.333003326126869,0.666006652253723),
 .UNSPECIFIED.);
#1208=B_SPLINE_CURVE_WITH_KNOTS('',3,(#32719,#32720,#32721,#32722,#32723,
#32724),.UNSPECIFIED.,.F.,.F.,(4,2,4),(0.,0.399660022402634,0.799320001325709),
 .UNSPECIFIED.);
#1209=B_SPLINE_CURVE_WITH_KNOTS('',3,(#32726,#32727,#32728,#32729,#32730,
#32731),.UNSPECIFIED.,.F.,.F.,(4,2,4),(0.,0.394929358834099,0.789859724379254),
 .UNSPECIFIED.);
#1210=B_SPLINE_CURVE_WITH_KNOTS('',3,(#32746,#32747,#32748,#32749,#32750,
#32751),.UNSPECIFIED.,.F.,.F.,(4,2,4),(1.00000001560095E-6,0.394931365545173,
0.789860724379263),.UNSPECIFIED.);
#1211=B_SPLINE_CURVE_WITH_KNOTS('',3,(#32753,#32754,#32755,#32756,#32757,
#32758),.UNSPECIFIED.,.F.,.F.,(4,2,4),(0.,0.399659978931984,0.799320001325694),
 .UNSPECIFIED.);
#1212=B_SPLINE_CURVE_WITH_KNOTS('',3,(#32760,#32761,#32762,#32763,#32764,
#32765),.UNSPECIFIED.,.F.,.F.,(4,2,4),(0.,0.333003326126855,0.666006652253734),
 .UNSPECIFIED.);
#1213=B_SPLINE_CURVE_WITH_KNOTS('',3,(#32767,#32768,#32769,#32770,#32771,
#32772),.UNSPECIFIED.,.F.,.F.,(4,2,4),(0.,0.396114271378083,0.792228542747862),
 .UNSPECIFIED.);
#1214=B_SPLINE_CURVE_WITH_KNOTS('',3,(#32774,#32775,#32776,#32777,#32778,
#32779),.UNSPECIFIED.,.F.,.F.,(4,2,4),(0.,0.333003326126878,0.666006652253737),
 .UNSPECIFIED.);
#1215=B_SPLINE_CURVE_WITH_KNOTS('',3,(#32781,#32782,#32783,#32784,#32785,
#32786),.UNSPECIFIED.,.F.,.F.,(4,2,4),(0.,0.399660022402913,0.79932000132569),
 .UNSPECIFIED.);
#1216=B_SPLINE_CURVE_WITH_KNOTS('',3,(#32788,#32789,#32790,#32791,#32792,
#32793),.UNSPECIFIED.,.F.,.F.,(4,2,4),(0.,0.394929358834091,0.789859724379262),
 .UNSPECIFIED.);
#1217=B_SPLINE_CURVE_WITH_KNOTS('',3,(#32796,#32797,#32798,#32799,#32800,
#32801),.UNSPECIFIED.,.F.,.F.,(4,2,4),(1.00000001065878E-6,0.393842731522518,
0.787628258068762),.UNSPECIFIED.);
#1218=B_SPLINE_CURVE_WITH_KNOTS('',3,(#32803,#32804,#32805,#32806,#32807,
#32808,#32809,#32810,#32811,#32812,#32813,#32814,#32815,#32816,#32817,#32818,
#32819,#32820,#32821,#32822,#32823,#32824,#32825,#32826,#32827,#32828,#32829),
 .UNSPECIFIED.,.F.,.F.,(4,3,3,3,3,3,2,2,2,2,4),(0.,0.166384002763973,0.200043514355487,
0.333101812640448,0.400072323934008,0.500472422318454,0.667828884642908,
0.667927982169589,0.834482890734559,0.834643736071572,0.99999999990215),
 .UNSPECIFIED.);
#1219=B_SPLINE_CURVE_WITH_KNOTS('',3,(#32833,#32834,#32835,#32836,#32837,
#32838,#32839,#32840),.UNSPECIFIED.,.F.,.F.,(4,2,2,4),(9.99976141228907E-7,
0.105157211260081,0.151172928145465,0.210254656084201),.UNSPECIFIED.);
#1220=B_SPLINE_CURVE_WITH_KNOTS('',3,(#32842,#32843,#32844,#32845,#32846,
#32847,#32848,#32849),.UNSPECIFIED.,.F.,.F.,(4,2,2,4),(9.99965210135567E-7,
0.0633219202251493,0.106228627126563,0.154610242485071),.UNSPECIFIED.);
#1221=B_SPLINE_CURVE_WITH_KNOTS('',3,(#32851,#32852,#32853,#32854,#32855,
#32856),.UNSPECIFIED.,.F.,.F.,(4,2,4),(9.99965276140573E-7,0.0775123835625057,
0.155023767084188),.UNSPECIFIED.);
#1222=B_SPLINE_CURVE_WITH_KNOTS('',3,(#32858,#32859,#32860,#32861,#32862,
#32863,#32864,#32865),.UNSPECIFIED.,.F.,.F.,(4,2,2,4),(9.99966295642252E-7,
0.0658748368226187,0.110565073148263,0.160346982706108),.UNSPECIFIED.);
#1223=B_SPLINE_CURVE_WITH_KNOTS('',3,(#32867,#32868,#32869,#32870,#32871,
#32872),.UNSPECIFIED.,.F.,.F.,(4,2,4),(9.99986040324985E-7,0.164974177883319,
0.361524612017389),.UNSPECIFIED.);
#1224=B_SPLINE_CURVE_WITH_KNOTS('',3,(#32873,#32874,#32875,#32876,#32877,
#32878,#32879,#32880),.UNSPECIFIED.,.F.,.F.,(4,2,2,4),(9.9999999975075E-7,
0.128289718374617,0.220416183775122,0.361296752356353),.UNSPECIFIED.);
#1225=B_SPLINE_CURVE_WITH_KNOTS('',3,(#32967,#32968,#32969,#32970,#32971,
#32972,#32973,#32974,#32975,#32976,#32977,#32978,#32979,#32980,#32981,#32982,
#32983,#32984,#32985,#32986,#32987,#32988,#32989,#32990,#32991,#32992),
 .UNSPECIFIED.,.F.,.F.,(4,2,2,2,2,2,2,2,2,2,2,2,4),(-0.668077385109111,
-0.655486882058708,-0.645122638439435,-0.624392837944345,-0.58292822337847,
-0.499980909052796,-0.334030281527956,-0.168124054836522,-0.0851704516733711,
-0.0436954289381117,-0.0229585825929834,-0.0125903518508265,-9.99972897337794E-7),
 .UNSPECIFIED.);
#1226=B_SPLINE_CURVE_WITH_KNOTS('',3,(#33019,#33020,#33021,#33022,#33023,
#33024,#33025,#33026),.UNSPECIFIED.,.F.,.F.,(4,2,2,4),(9.99999997781767E-7,
1.05861232407444,1.79204764279102,2.50572967370245),.UNSPECIFIED.);
#1227=B_SPLINE_CURVE_WITH_KNOTS('',3,(#33027,#33028,#33029,#33030,#33031,
#33032),.UNSPECIFIED.,.F.,.F.,(4,2,4),(-1.31283511954368,-0.637662453649952,
-9.87368154348189E-7),.UNSPECIFIED.);
#1228=B_SPLINE_CURVE_WITH_KNOTS('',3,(#33037,#33038,#33039,#33040,#33041,
#33042),.UNSPECIFIED.,.F.,.F.,(4,2,4),(-0.219238344309207,-0.109619779347491,
-1.00000000258227E-6),.UNSPECIFIED.);
#1229=B_SPLINE_CURVE_WITH_KNOTS('',3,(#33051,#33052,#33053,#33054,#33055,
#33056),.UNSPECIFIED.,.F.,.F.,(4,2,4),(1.0096733036915E-6,0.204604110997339,
0.489538124307061),.UNSPECIFIED.);
#1230=B_SPLINE_CURVE_WITH_KNOTS('',3,(#33059,#33060,#33061,#33062,#33063,
#33064),.UNSPECIFIED.,.F.,.F.,(4,2,4),(1.00000037364389E-6,0.154897514630139,
0.274475905655399),.UNSPECIFIED.);
#1231=B_SPLINE_CURVE_WITH_KNOTS('',3,(#33075,#33076,#33077,#33078,#33079,
#33080,#33081,#33082),.UNSPECIFIED.,.F.,.F.,(4,2,2,4),(0.,0.414903698568167,
0.654288803333593,0.895643214275791),.UNSPECIFIED.);
#1232=B_SPLINE_CURVE_WITH_KNOTS('',3,(#33087,#33088,#33089,#33090,#33091,
#33092),.UNSPECIFIED.,.F.,.F.,(4,2,4),(-0.236447866929972,-0.118098613922891,
0.),.UNSPECIFIED.);
#1233=B_SPLINE_CURVE_WITH_KNOTS('',3,(#33103,#33104,#33105,#33106,#33107,
#33108),.UNSPECIFIED.,.F.,.F.,(4,2,4),(0.,0.150850161004902,0.306679145643486),
 .UNSPECIFIED.);
#1234=B_SPLINE_CURVE_WITH_KNOTS('',3,(#33109,#33110,#33111,#33112,#33113,
#33114),.UNSPECIFIED.,.F.,.F.,(4,2,4),(0.,0.151283693630131,0.298616647391532),
 .UNSPECIFIED.);
#1235=B_SPLINE_CURVE_WITH_KNOTS('',3,(#33125,#33126,#33127,#33128,#33129,
#33130,#33131,#33132,#33133,#33134),.UNSPECIFIED.,.F.,.F.,(4,2,2,2,4),(-0.879854016291582,
-0.656514046006911,-0.439871468993734,-0.223283558174501,0.),
 .UNSPECIFIED.);
#1236=B_SPLINE_CURVE_WITH_KNOTS('',3,(#33139,#33140,#33141,#33142,#33143,
#33144),.UNSPECIFIED.,.F.,.F.,(4,2,4),(-0.236447869261725,-0.118223934265819,
0.),.UNSPECIFIED.);
#1237=B_SPLINE_CURVE_WITH_KNOTS('',3,(#33155,#33156,#33157,#33158,#33159,
#33160),.UNSPECIFIED.,.F.,.F.,(4,2,4),(0.,0.147316860903661,0.298566671239079),
 .UNSPECIFIED.);
#1238=B_SPLINE_CURVE_WITH_KNOTS('',3,(#33161,#33162,#33163,#33164,#33165,
#33166),.UNSPECIFIED.,.F.,.F.,(4,2,4),(0.,0.155861462063028,0.306744458244242),
 .UNSPECIFIED.);
#1239=B_SPLINE_CURVE_WITH_KNOTS('',3,(#33177,#33178,#33179,#33180,#33181,
#33182,#33183,#33184,#33185,#33186),.UNSPECIFIED.,.F.,.F.,(4,2,2,2,4),(0.,
0.212413059834235,0.422510962127527,0.653050142710767,0.893897606534324),
 .UNSPECIFIED.);
#1240=B_SPLINE_CURVE_WITH_KNOTS('',3,(#33191,#33192,#33193,#33194,#33195,
#33196),.UNSPECIFIED.,.F.,.F.,(4,2,4),(-0.21923729130139,-0.109655629737214,
0.),.UNSPECIFIED.);
#1241=B_SPLINE_CURVE_WITH_KNOTS('',3,(#33206,#33207,#33208,#33209,#33210,
#33211,#33212,#33213),.UNSPECIFIED.,.F.,.F.,(4,2,2,4),(1.00620996162504E-6,
0.71712566206726,1.45409684772959,2.51788337929663),.UNSPECIFIED.);
#1242=B_SPLINE_CURVE_WITH_KNOTS('',3,(#33214,#33215,#33216,#33217,#33218,
#33219),.UNSPECIFIED.,.F.,.F.,(4,2,4),(0.,0.273557576637765,0.489035686879138),
 .UNSPECIFIED.);
#1243=B_SPLINE_CURVE_WITH_KNOTS('',3,(#33220,#33221,#33222,#33223,#33224,
#33225),.UNSPECIFIED.,.F.,.F.,(4,2,4),(0.,0.139626851787869,0.274479307755968),
 .UNSPECIFIED.);
#1244=B_SPLINE_CURVE_WITH_KNOTS('',3,(#33242,#33243,#33244,#33245,#33246,
#33247),.UNSPECIFIED.,.F.,.F.,(4,2,4),(-1.31305950518371,-0.674802781976278,
0.),.UNSPECIFIED.);
#1245=B_SPLINE_CURVE_WITH_KNOTS('',3,(#33296,#33297,#33298,#33299,#33300,
#33301,#33302,#33303,#33304,#33305,#33306,#33307,#33308,#33309,#33310,#33311,
#33312,#33313,#33314,#33315,#33316,#33317),.UNSPECIFIED.,.F.,.F.,(4,2,2,
2,2,2,2,2,2,2,4),(-0.67702556757787,-0.651718544287976,-0.630843443379476,
-0.58908983016846,-0.505569216727294,-0.338477588334701,-0.171470508905719,
-0.087950579362434,-0.04618670809926,-0.0253037910690105,-9.99986766170302E-7),
 .UNSPECIFIED.);
#1246=B_SPLINE_CURVE_WITH_KNOTS('',3,(#33327,#33328,#33329,#33330,#33331,
#33332),.UNSPECIFIED.,.F.,.F.,(4,2,4),(-0.20312688170718,-0.101605684816453,
0.),.UNSPECIFIED.);
#1247=B_SPLINE_CURVE_WITH_KNOTS('',3,(#33361,#33362,#33363,#33364,#33365,
#33366),.UNSPECIFIED.,.F.,.F.,(4,2,4),(1.00620234016808E-6,0.51961835527925,
1.02113839753968),.UNSPECIFIED.);
#1248=B_SPLINE_CURVE_WITH_KNOTS('',3,(#33367,#33368,#33369,#33370,#33371,
#33372),.UNSPECIFIED.,.F.,.F.,(4,2,4),(1.15442842194411,1.861681583331,
2.51727485684938),.UNSPECIFIED.);
#1249=B_SPLINE_CURVE_WITH_KNOTS('',3,(#33417,#33418,#33419,#33420,#33421,
#33422),.UNSPECIFIED.,.F.,.F.,(4,2,4),(-0.219070150136512,-0.109422426323688,
0.),.UNSPECIFIED.);
#1250=B_SPLINE_CURVE_WITH_KNOTS('',3,(#33442,#33443,#33444,#33445,#33446,
#33447),.UNSPECIFIED.,.F.,.F.,(4,2,4),(-0.219070150454542,-0.10976760949543,
0.),.UNSPECIFIED.);
#1251=B_SPLINE_CURVE_WITH_KNOTS('',3,(#33502,#33503,#33504,#33505,#33506,
#33507,#33508,#33509,#33510,#33511,#33512,#33513,#33514,#33515,#33516,#33517,
#33518,#33519,#33520,#33521,#33522,#33523,#33524,#33525),.UNSPECIFIED.,
 .F.,.F.,(4,2,2,2,2,2,2,2,2,2,2,4),(-0.689781963483316,-0.663919875534272,
-0.64257964545,-0.599900589922741,-0.514548378234951,-0.343871644022324,
-0.173035127373472,-0.0876435221726812,-0.0449550934221477,-0.0236127939716027,
-0.0129421303647674,-9.99973913562435E-7),.UNSPECIFIED.);
#1252=B_SPLINE_CURVE_WITH_KNOTS('',3,(#33534,#33535,#33536,#33537,#33538,
#33539,#33540,#33541),.UNSPECIFIED.,.F.,.F.,(4,2,2,4),(-1.66037250641965,
-0.87290811148185,-0.0419427109352258,0.),.UNSPECIFIED.);
#1253=B_SPLINE_CURVE_WITH_KNOTS('',3,(#33544,#33545,#33546,#33547,#33548,
#33549),.UNSPECIFIED.,.F.,.F.,(4,2,4),(0.,1.22223732175759,2.95853995676252),
 .UNSPECIFIED.);
#1254=B_SPLINE_CURVE_WITH_KNOTS('',3,(#33550,#33551,#33552,#33553),
 .UNSPECIFIED.,.F.,.F.,(4,4),(-23.1972630946761,-22.347414707605),
 .UNSPECIFIED.);
#1255=B_SPLINE_CURVE_WITH_KNOTS('',3,(#33558,#33559,#33560,#33561,#33562,
#33563),.UNSPECIFIED.,.F.,.F.,(4,2,4),(9.99999994860392E-7,0.112313919124985,
0.224652231943206),.UNSPECIFIED.);
#1256=B_SPLINE_CURVE_WITH_KNOTS('',3,(#33628,#33629,#33630,#33631,#33632,
#33633),.UNSPECIFIED.,.F.,.F.,(4,2,4),(0.,0.20854145283333,0.373296784857941),
 .UNSPECIFIED.);
#1257=B_SPLINE_CURVE_WITH_KNOTS('',3,(#33636,#33637,#33638,#33639,#33640,
#33641),.UNSPECIFIED.,.F.,.F.,(4,2,4),(9.99999986949769E-7,0.158932365867243,
0.391091294154302),.UNSPECIFIED.);
#1258=B_SPLINE_CURVE_WITH_KNOTS('',3,(#33708,#33709,#33710,#33711,#33712,
#33713),.UNSPECIFIED.,.F.,.F.,(4,2,4),(1.03330465267236E-6,0.182634881882751,
0.383588358675),.UNSPECIFIED.);
#1259=B_SPLINE_CURVE_WITH_KNOTS('',3,(#33718,#33719,#33720,#33721,#33722,
#33723),.UNSPECIFIED.,.F.,.F.,(4,2,4),(9.999997436785E-7,0.113920800023667,
0.228887545318261),.UNSPECIFIED.);
#1260=B_SPLINE_CURVE_WITH_KNOTS('',3,(#33790,#33791,#33792,#33793,#33794,
#33795),.UNSPECIFIED.,.F.,.F.,(4,2,4),(9.99999083278551E-7,0.12313457024449,
0.288846007336836),.UNSPECIFIED.);
#1261=B_SPLINE_CURVE_WITH_KNOTS('',3,(#33796,#33797,#33798,#33799,#33800,
#33801),.UNSPECIFIED.,.F.,.F.,(4,2,4),(9.99991096902383E-7,0.078379741412785,
0.129432320943639),.UNSPECIFIED.);
#1262=B_SPLINE_CURVE_WITH_KNOTS('',3,(#33868,#33869,#33870,#33871,#33872,
#33873),.UNSPECIFIED.,.F.,.F.,(4,2,4),(9.99989423159434E-7,0.211833339665523,
0.42360307281474),.UNSPECIFIED.);
#1263=B_SPLINE_CURVE_WITH_KNOTS('',3,(#33878,#33879,#33880,#33881,#33882,
#33883),.UNSPECIFIED.,.F.,.F.,(4,2,4),(9.99999996036891E-7,0.11189630300938,
0.221776909200746),.UNSPECIFIED.);
#1264=B_SPLINE_CURVE_WITH_KNOTS('',3,(#33950,#33951,#33952,#33953,#33954,
#33955),.UNSPECIFIED.,.F.,.F.,(4,2,4),(1.00000031278451E-6,0.146046673780185,
0.369899176224888),.UNSPECIFIED.);
#1265=B_SPLINE_CURVE_WITH_KNOTS('',3,(#33956,#33957,#33958,#33959,#33960,
#33961),.UNSPECIFIED.,.F.,.F.,(4,2,4),(9.99963678285791E-7,0.0529579303912984,
0.0924045001196666),.UNSPECIFIED.);
#1266=B_SPLINE_CURVE_WITH_KNOTS('',3,(#34028,#34029,#34030,#34031,#34032,
#34033),.UNSPECIFIED.,.F.,.F.,(4,2,4),(9.99986781446215E-7,0.170524601610324,
0.324175091837708),.UNSPECIFIED.);
#1267=B_SPLINE_CURVE_WITH_KNOTS('',3,(#34038,#34039,#34040,#34041,#34042,
#34043),.UNSPECIFIED.,.F.,.F.,(4,2,4),(1.0000000011459E-6,0.112462083036288,
0.225270672274139),.UNSPECIFIED.);
#1268=B_SPLINE_CURVE_WITH_KNOTS('',3,(#34109,#34110,#34111,#34112,#34113,
#34114),.UNSPECIFIED.,.F.,.F.,(4,2,4),(9.99378738311195E-7,1.48487197654131,
3.23722575134267),.UNSPECIFIED.);
#1269=B_SPLINE_CURVE_WITH_KNOTS('',3,(#34115,#34116,#34117,#34118,#34119,
#34120),.UNSPECIFIED.,.F.,.F.,(4,2,4),(9.99999984664222E-7,0.280996171754984,
0.634468298631835),.UNSPECIFIED.);
#1270=B_SPLINE_CURVE_WITH_KNOTS('',3,(#34121,#34122,#34123,#34124,#34125,
#34126),.UNSPECIFIED.,.F.,.F.,(4,2,4),(9.9997018998747E-7,0.0631262577557768,
0.106314027062238),.UNSPECIFIED.);
#1271=B_SPLINE_CURVE_WITH_KNOTS('',3,(#34168,#34169,#34170,#34171,#34172,
#34173,#34174,#34175,#34176,#34177,#34178,#34179,#34180,#34181,#34182,#34183,
#34184,#34185,#34186,#34187,#34188,#34189,#34190,#34191,#34192,#34193,#34194,
#34195,#34196,#34197,#34198,#34199,#34200,#34201,#34202,#34203,#34204,#34205,
#34206,#34207,#34208,#34209,#34210,#34211,#34212,#34213,#34214,#34215,#34216,
#34217,#34218,#34219,#34220,#34221,#34222,#34223,#34224,#34225,#34226,#34227,
#34228,#34229,#34230,#34231,#34232,#34233,#34234,#34235,#34236,#34237,#34238,
#34239,#34240,#34241,#34242,#34243,#34244,#34245,#34246,#34247,#34248,#34249,
#34250,#34251,#34252,#34253,#34254,#34255),.UNSPECIFIED.,.F.,.F.,(4,3,3,
3,3,3,3,3,3,3,3,3,3,3,3,3,3,3,3,3,3,3,3,3,3,3,3,3,3,4),(0.,0.166675928619695,
0.173691671300186,0.254448942023543,0.294348326144002,0.333295697963079,
0.383467607004402,0.499995091497343,0.500000000000883,0.570172751020376,
0.666571417474997,0.666664431569024,0.670314863554253,0.674854874036545,
0.749023437501325,0.750000000001324,0.812500000001118,0.836217353799779,
0.836971115969276,0.837080348477548,0.837120435215152,0.843750000001017,
0.867187500000943,0.874511718750916,0.875000000000913,0.906458280152192,
0.943531800863156,0.995806241052779,0.999114427440319,1.),.UNSPECIFIED.);
#1272=B_SPLINE_CURVE_WITH_KNOTS('',3,(#34256,#34257,#34258,#34259,#34260,
#34261,#34262),.UNSPECIFIED.,.F.,.F.,(4,3,4),(8.05019156257696E-11,0.00536781103725429,
0.00861833511932773),.UNSPECIFIED.);
#1273=B_SPLINE_CURVE_WITH_KNOTS('',3,(#35884,#35885,#35886,#35887,#35888,
#35889,#35890,#35891,#35892,#35893,#35894,#35895,#35896,#35897,#35898,#35899,
#35900,#35901,#35902,#35903,#35904,#35905,#35906,#35907,#35908,#35909,#35910,
#35911,#35912,#35913,#35914,#35915,#35916,#35917,#35918,#35919,#35920,#35921,
#35922,#35923,#35924,#35925,#35926,#35927),.UNSPECIFIED.,.F.,.F.,(4,2,1,
1,1,1,2,2,2,1,1,1,2,2,2,2,2,1,2,2,2,1,1,1,1,2,2,4),(0.,0.249999999994906,
0.374999999992358,0.437499999991084,0.468749999990448,0.484374999990131,
0.499755859364856,0.499999999989862,0.562499999991161,0.59374999999181,
0.609374999992134,0.617187499992296,0.623046874992423,0.624999999992465,
0.687499999993976,0.695312499994169,0.703124999994362,0.718749999994754,
0.749023437495509,0.74999999999553,0.812499999996658,0.843749999997218,
0.859374999997502,0.867187499997643,0.871093749997717,0.874023437497773,
0.874999999997791,1.),.UNSPECIFIED.);
#1274=B_SPLINE_CURVE_WITH_KNOTS('',3,(#35928,#35929,#35930,#35931,#35932,
#35933,#35934,#35935,#35936,#35937,#35938,#35939,#35940,#35941,#35942,#35943,
#35944,#35945,#35946,#35947,#35948,#35949,#35950,#35951),.UNSPECIFIED.,
 .F.,.F.,(4,2,2,2,2,2,2,2,2,2,2,4),(1.01547833161899E-13,0.15566333494698,
0.311333269417955,0.622613162774609,0.829990346854508,1.24450593125942,
1.45160761783459,1.55514057778074,1.60689756195558,1.63277301939669,1.6457099117961,
1.66147743182145),.UNSPECIFIED.);
#1275=B_SPLINE_CURVE_WITH_KNOTS('',3,(#35968,#35969,#35970,#35971,#35972,
#35973,#35974,#35975,#35976,#35977),.UNSPECIFIED.,.F.,.F.,(4,3,3,4),(0.,
0.00439626310689482,0.00879197415188345,0.0108268048064541),
 .UNSPECIFIED.);
#1276=B_SPLINE_CURVE_WITH_KNOTS('',3,(#35992,#35993,#35994,#35995,#35996,
#35997),.UNSPECIFIED.,.F.,.F.,(4,2,4),(-0.203125620789724,-0.101587706586047,
0.),.UNSPECIFIED.);
#1277=B_SPLINE_CURVE_WITH_KNOTS('',3,(#36015,#36016,#36017,#36018),
 .UNSPECIFIED.,.F.,.F.,(4,4),(6.93889390390723E-18,0.0131542251006493),
 .UNSPECIFIED.);
#1278=B_SPLINE_CURVE_WITH_KNOTS('',3,(#36019,#36020,#36021,#36022,#36023,
#36024,#36025,#36026),.UNSPECIFIED.,.F.,.F.,(4,2,2,4),(1.00147320738661E-6,
0.717114068453892,1.45422582770195,2.51726157849465),.UNSPECIFIED.);
#1279=B_SPLINE_CURVE_WITH_KNOTS('',3,(#36044,#36045,#36046,#36047,#36048,
#36049,#36050,#36051),.UNSPECIFIED.,.F.,.F.,(4,2,2,4),(9.99999983042343E-7,
1.05770788847698,1.79140562198516,2.50518852593767),.UNSPECIFIED.);
#1280=B_SPLINE_CURVE_WITH_KNOTS('',3,(#36052,#36053,#36054,#36055,#36056,
#36057),.UNSPECIFIED.,.F.,.F.,(4,2,4),(-1.31507690872101,-0.657539408413606,
-9.8734492248731E-7),.UNSPECIFIED.);
#1281=B_SPLINE_CURVE_WITH_KNOTS('',3,(#36071,#36072,#36073,#36074,#36075,
#36076),.UNSPECIFIED.,.F.,.F.,(4,2,4),(1.00970492822167E-6,0.246544274330857,
0.495341408835484),.UNSPECIFIED.);
#1282=B_SPLINE_CURVE_WITH_KNOTS('',3,(#36079,#36080,#36081,#36082,#36083,
#36084),.UNSPECIFIED.,.F.,.F.,(4,2,4),(1.00000002958826E-6,0.141407464738658,
0.282694947289526),.UNSPECIFIED.);
#1283=B_SPLINE_CURVE_WITH_KNOTS('',3,(#36095,#36096,#36097,#36098,#36099,
#36100,#36101,#36102,#36103,#36104),.UNSPECIFIED.,.F.,.F.,(4,2,2,2,4),(0.,
0.227646793319022,0.445793915542063,0.66886948512083,0.894190037790346),
 .UNSPECIFIED.);
#1284=B_SPLINE_CURVE_WITH_KNOTS('',3,(#36109,#36110,#36111,#36112,#36113,
#36114),.UNSPECIFIED.,.F.,.F.,(4,2,4),(-0.219067405041613,-0.109420963077563,
0.),.UNSPECIFIED.);
#1285=B_SPLINE_CURVE_WITH_KNOTS('',3,(#36125,#36126,#36127,#36128,#36129,
#36130),.UNSPECIFIED.,.F.,.F.,(4,2,4),(0.,0.157819485234147,0.315476292188043),
 .UNSPECIFIED.);
#1286=B_SPLINE_CURVE_WITH_KNOTS('',3,(#36131,#36132,#36133,#36134,#36135,
#36136),.UNSPECIFIED.,.F.,.F.,(4,2,4),(0.,0.153590633707747,0.307315056675274),
 .UNSPECIFIED.);
#1287=B_SPLINE_CURVE_WITH_KNOTS('',3,(#36147,#36148,#36149,#36150,#36151,
#36152,#36153,#36154,#36155,#36156),.UNSPECIFIED.,.F.,.F.,(4,2,2,2,4),(0.,
0.223290793074201,0.43983513202536,0.656542865977632,0.880002105353678),
 .UNSPECIFIED.);
#1288=B_SPLINE_CURVE_WITH_KNOTS('',3,(#36161,#36162,#36163,#36164,#36165,
#36166),.UNSPECIFIED.,.F.,.F.,(4,2,4),(-0.219067432347822,-0.109533716096716,
0.),.UNSPECIFIED.);
#1289=B_SPLINE_CURVE_WITH_KNOTS('',3,(#36177,#36178,#36179,#36180,#36181,
#36182),.UNSPECIFIED.,.F.,.F.,(4,2,4),(0.,0.153696799307367,0.30725981325678),
 .UNSPECIFIED.);
#1290=B_SPLINE_CURVE_WITH_KNOTS('',3,(#36183,#36184,#36185,#36186,#36187,
#36188),.UNSPECIFIED.,.F.,.F.,(4,2,4),(0.,0.157693074719598,0.315548927891733),
 .UNSPECIFIED.);
#1291=B_SPLINE_CURVE_WITH_KNOTS('',3,(#36199,#36200,#36201,#36202,#36203,
#36204,#36205,#36206,#36207,#36208),.UNSPECIFIED.,.F.,.F.,(4,2,2,2,4),(0.,
0.225387094225478,0.448531943602552,0.66660741501709,0.894174761832726),
 .UNSPECIFIED.);
#1292=B_SPLINE_CURVE_WITH_KNOTS('',3,(#36217,#36218,#36219,#36220,#36221,
#36222),.UNSPECIFIED.,.F.,.F.,(4,2,4),(1.44977320229459E-15,0.24697660625387,
0.494938254641676),.UNSPECIFIED.);
#1293=B_SPLINE_CURVE_WITH_KNOTS('',3,(#36223,#36224,#36225,#36226,#36227,
#36228),.UNSPECIFIED.,.F.,.F.,(4,2,4),(0.,0.141299010574654,0.282729372489341),
 .UNSPECIFIED.);
#1294=B_SPLINE_CURVE_WITH_KNOTS('',3,(#36285,#36286,#36287,#36288),
 .UNSPECIFIED.,.F.,.F.,(4,4),(4.11130213194751E-6,0.999911030802199),
 .UNSPECIFIED.);
#1295=B_SPLINE_CURVE_WITH_KNOTS('',3,(#36321,#36322,#36323,#36324,#36325,
#36326),.UNSPECIFIED.,.F.,.F.,(4,2,4),(-0.291319261775491,-0.159787359154877,
0.),.UNSPECIFIED.);
#1296=B_SPLINE_CURVE_WITH_KNOTS('',3,(#36329,#36330,#36331,#36332,#36333,
#36334),.UNSPECIFIED.,.F.,.F.,(4,2,4),(-0.942062317972325,-0.782274958817505,
-0.650743056196821),.UNSPECIFIED.);
#1297=B_SPLINE_CURVE_WITH_KNOTS('',3,(#36343,#36344,#36345,#36346,#36347,
#36348),.UNSPECIFIED.,.F.,.F.,(4,2,4),(-0.29131926177555,-0.159787359154858,
-3.46389583683049E-14),.UNSPECIFIED.);
#1298=B_SPLINE_CURVE_WITH_KNOTS('',3,(#36351,#36352,#36353,#36354,#36355,
#36356),.UNSPECIFIED.,.F.,.F.,(4,2,4),(-0.94206231797227,-0.782274958817496,
-0.650743056196749),.UNSPECIFIED.);
#1299=B_SPLINE_CURVE_WITH_KNOTS('',3,(#36359,#36360,#36361,#36362,#36363,
#36364),.UNSPECIFIED.,.F.,.F.,(4,2,4),(-0.299277276892238,-0.149638638446119,
0.),.UNSPECIFIED.);
#1300=B_SPLINE_CURVE_WITH_KNOTS('',3,(#36368,#36369,#36370,#36371,#36372,
#36373),.UNSPECIFIED.,.F.,.F.,(4,2,4),(-0.942062317972285,-0.782274958817465,
-0.650743056196774),.UNSPECIFIED.);
#1301=B_SPLINE_CURVE_WITH_KNOTS('',3,(#36379,#36380,#36381,#36382,#36383,
#36384),.UNSPECIFIED.,.F.,.F.,(4,2,4),(-0.291319261775506,-0.15978735915482,
0.),.UNSPECIFIED.);
#1302=B_SPLINE_CURVE_WITH_KNOTS('',3,(#36387,#36388,#36389,#36390,#36391,
#36392),.UNSPECIFIED.,.F.,.F.,(4,2,4),(-0.942062317972366,-0.792423679526272,
-0.642785041080179),.UNSPECIFIED.);
#1303=B_SPLINE_CURVE_WITH_KNOTS('',3,(#36445,#36446,#36447,#36448,#36449,
#36450),.UNSPECIFIED.,.F.,.F.,(4,2,4),(7.05548697529559E-15,0.00523107916144303,
0.010462158322879),.UNSPECIFIED.);
#1304=B_SPLINE_CURVE_WITH_KNOTS('',3,(#36455,#36456,#36457,#36458,#36459,
#36460,#36461,#36462,#36463,#36464,#36465,#36466,#36467,#36468),
 .UNSPECIFIED.,.F.,.F.,(4,2,2,2,2,2,4),(1.00000023840693E-6,0.2965902763434,
0.65268898649409,1.00818635283356,1.36397466372344,1.98488039747023,2.01473577478548),
 .UNSPECIFIED.);
#1305=B_SPLINE_CURVE_WITH_KNOTS('',3,(#36521,#36522,#36523,#36524,#36525,
#36526,#36527,#36528,#36529,#36530,#36531,#36532,#36533,#36534,#36535,#36536,
#36537,#36538,#36539,#36540,#36541,#36542),.UNSPECIFIED.,.F.,.F.,(4,2,2,
2,2,2,2,2,2,2,4),(9.99322294003157E-7,0.011417887542787,0.0222845745097274,
0.0440049682421546,0.0874125886811494,0.174267175958524,0.261121619243541,
0.304529168043487,0.326249525934761,0.337116194970005,0.348534141656),
 .UNSPECIFIED.);
#1306=B_SPLINE_CURVE_WITH_KNOTS('',3,(#36592,#36593,#36594,#36595,#36596,
#36597),.UNSPECIFIED.,.F.,.F.,(4,2,4),(9.13855224931671E-16,0.00523107914708959,
0.0104621582941783),.UNSPECIFIED.);
#1307=B_SPLINE_CURVE_WITH_KNOTS('',3,(#36599,#36600,#36601,#36602,#36603,
#36604,#36605,#36606,#36607,#36608,#36609,#36610,#36611,#36612),
 .UNSPECIFIED.,.F.,.F.,(4,2,2,2,2,2,4),(9.99999960801238E-7,0.0410400374680066,
0.66754883484164,1.04225619039533,1.42067016209639,1.80065436420091,2.13788105830901),
 .UNSPECIFIED.);
#1308=B_SPLINE_CURVE_WITH_KNOTS('',3,(#36668,#36669,#36670,#36671,#36672,
#36673,#36674,#36675,#36676,#36677,#36678,#36679,#36680,#36681),
 .UNSPECIFIED.,.F.,.F.,(4,2,2,2,2,2,4),(-1.99242246967209,-1.69912264605073,
-1.34696492109298,-0.995397472045463,-0.643553467950021,-0.0295448893533265,
-9.99999972400604E-7),.UNSPECIFIED.);
#1309=B_SPLINE_CURVE_WITH_KNOTS('',3,(#36682,#36683,#36684,#36685,#36686,
#36687),.UNSPECIFIED.,.F.,.F.,(4,2,4),(2.97263381041754E-14,0.00523107914593693,
0.0104621582918441),.UNSPECIFIED.);
#1310=B_SPLINE_CURVE_WITH_KNOTS('',3,(#36739,#36740,#36741,#36742,#36743,
#36744,#36745,#36746,#36747,#36748,#36749,#36750,#36751,#36752,#36753,#36754,
#36755,#36756,#36757,#36758,#36759,#36760),.UNSPECIFIED.,.F.,.F.,(4,2,2,
2,2,2,2,2,2,2,4),(-0.34853295910873,-0.337115227653266,-0.32624857232804,
-0.304528241839957,-0.261120747808474,-0.174266413464672,-0.0874122231124873,
-0.0440048007218869,-0.0222845060773082,-0.0114178686877548,-9.99322293774237E-7),
 .UNSPECIFIED.);
#1311=B_SPLINE_CURVE_WITH_KNOTS('',3,(#36811,#36812,#36813,#36814,#36815,
#36816),.UNSPECIFIED.,.F.,.F.,(4,2,4),(1.24917436300588E-15,0.00523107916140929,
0.0104621583229247),.UNSPECIFIED.);
#1312=B_SPLINE_CURVE_WITH_KNOTS('',3,(#36818,#36819,#36820,#36821,#36822,
#36823,#36824,#36825,#36826,#36827,#36828,#36829,#36830,#36831),
 .UNSPECIFIED.,.F.,.F.,(4,2,2,2,2,2,4),(-1.54593699203168,-1.51627628058056,
-1.06322836063848,-0.792267283873332,-0.518634619264518,-0.243863513378528,
-9.99999280715258E-7),.UNSPECIFIED.);
#1313=B_SPLINE_CURVE_WITH_KNOTS('',3,(#36887,#36888,#36889,#36890,#36891,
#36892,#36893,#36894,#36895,#36896,#36897,#36898,#36899,#36900),
 .UNSPECIFIED.,.F.,.F.,(4,2,2,2,2,2,4),(-2.0247534649149,-1.7026576276926,
-1.34880623927078,-0.995849757258031,-0.643258648524814,-0.0288142926510343,
-9.99999972288645E-7),.UNSPECIFIED.);
#1314=B_SPLINE_CURVE_WITH_KNOTS('',3,(#36901,#36902,#36903,#36904,#36905,
#36906,#36907),.UNSPECIFIED.,.F.,.F.,(4,3,4),(1.73056695609661E-14,0.00523109611618601,
0.0104552267462395),.UNSPECIFIED.);
#1315=B_SPLINE_CURVE_WITH_KNOTS('',3,(#36959,#36960,#36961,#36962,#36963,
#36964,#36965,#36966,#36967,#36968,#36969,#36970,#36971,#36972,#36973,#36974,
#36975,#36976,#36977,#36978,#36979,#36980),.UNSPECIFIED.,.F.,.F.,(4,2,2,
2,2,2,2,2,2,2,4),(-0.348530046369699,-0.337112119683411,-0.326245568052259,
-0.304525444827838,-0.261118365012474,-0.174264859478894,-0.0874114979360114,
-0.0440044897577281,-0.0222844023781863,-0.0114178686869934,-9.9932229816912E-7),
 .UNSPECIFIED.);
#1316=B_SPLINE_CURVE_WITH_KNOTS('',3,(#37033,#37034,#37035,#37036,#37037,
#37038,#37039,#37040,#37041,#37042,#37043,#37044,#37045,#37046),
 .UNSPECIFIED.,.F.,.F.,(4,2,2,2,2,2,4),(-1.70662420609644,-1.45502819722534,
-1.20126789349393,-0.996223548128144,-0.767391103085636,-0.365223297458236,
-1.00000010760937E-6),.UNSPECIFIED.);
#1317=B_SPLINE_CURVE_WITH_KNOTS('',3,(#37103,#37104,#37105,#37106,#37107,
#37108,#37109,#37110,#37111,#37112,#37113,#37114,#37115,#37116),
 .UNSPECIFIED.,.F.,.F.,(4,2,2,2,2,2,4),(1.00000005213949E-6,0.373786457125504,
0.781780831542326,1.04178058769923,1.27449283557987,1.5610312787827,1.85194823288523),
 .UNSPECIFIED.);
#1318=B_SPLINE_CURVE_WITH_KNOTS('',3,(#37169,#37170,#37171,#37172,#37173,
#37174,#37175,#37176,#37177,#37178,#37179,#37180,#37181,#37182,#37183,#37184,
#37185,#37186,#37187,#37188,#37189,#37190),.UNSPECIFIED.,.F.,.F.,(4,2,2,
2,2,2,2,2,2,2,4),(9.99322295139288E-7,0.0114188541247426,0.0222854506093803,
0.0440056634961537,0.087412922514029,0.174266786615345,0.26112050672579,
0.30452769410305,0.326247871147981,0.337114449697216,0.348532261911283),
 .UNSPECIFIED.);
#1319=B_SPLINE_CURVE_WITH_KNOTS('',3,(#37240,#37241,#37242,#37243,#37244,
#37245),.UNSPECIFIED.,.F.,.F.,(4,2,4),(4.38854183572088E-17,0.00523107914592229,
0.0104621582918445),.UNSPECIFIED.);
#1320=B_SPLINE_CURVE_WITH_KNOTS('',3,(#37247,#37248,#37249,#37250,#37251,
#37252,#37253,#37254,#37255,#37256,#37257,#37258,#37259,#37260),
 .UNSPECIFIED.,.F.,.F.,(4,2,2,2,2,2,4),(9.99999961583338E-7,0.041041854241271,
0.667547702208066,1.04225347352809,1.42066695540823,1.80065028480642,2.13787646890171),
 .UNSPECIFIED.);
#1321=B_SPLINE_CURVE_WITH_KNOTS('',3,(#37319,#37320,#37321,#37322),
 .UNSPECIFIED.,.F.,.F.,(4,4),(0.,0.0275043317552308),.UNSPECIFIED.);
#1322=B_SPLINE_CURVE_WITH_KNOTS('',3,(#37333,#37334,#37335,#37336),
 .UNSPECIFIED.,.F.,.F.,(4,4),(4.997930709674E-16,0.0275043317552307),
 .UNSPECIFIED.);
#1323=B_SPLINE_CURVE_WITH_KNOTS('',3,(#37349,#37350,#37351,#37352),
 .UNSPECIFIED.,.F.,.F.,(4,4),(4.997930709674E-16,0.0275043317552307),
 .UNSPECIFIED.);
#1324=B_SPLINE_CURVE_WITH_KNOTS('',3,(#37363,#37364,#37365,#37366),
 .UNSPECIFIED.,.F.,.F.,(4,4),(4.997930709674E-16,0.0275043317552318),
 .UNSPECIFIED.);
#1325=B_SPLINE_CURVE_WITH_KNOTS('',3,(#37373,#37374,#37375,#37376),
 .UNSPECIFIED.,.F.,.F.,(4,4),(0.,0.0275043309106357),.UNSPECIFIED.);
#1326=B_SPLINE_CURVE_WITH_KNOTS('',3,(#37387,#37388,#37389,#37390),
 .UNSPECIFIED.,.F.,.F.,(4,4),(0.,0.0275045756311934),.UNSPECIFIED.);
#1327=B_SPLINE_CURVE_WITH_KNOTS('',3,(#37403,#37404,#37405,#37406),
 .UNSPECIFIED.,.F.,.F.,(4,4),(0.,0.0275045756311959),.UNSPECIFIED.);
#1328=B_SPLINE_CURVE_WITH_KNOTS('',3,(#37417,#37418,#37419,#37420),
 .UNSPECIFIED.,.F.,.F.,(4,4),(0.,0.0275043317552308),.UNSPECIFIED.);
#1329=B_SPLINE_CURVE_WITH_KNOTS('',3,(#38165,#38166,#38167,#38168,#38169,
#38170,#38171,#38172,#38173,#38174),.UNSPECIFIED.,.F.,.F.,(4,2,2,2,4),(-5.2918916828979,
-5.03351157658279,-4.84005150769012,-4.64659143879744,-4.34027267238539),
 .UNSPECIFIED.);
#1330=B_SPLINE_CURVE_WITH_KNOTS('',3,(#38336,#38337,#38338,#38339,#38340,
#38341),.UNSPECIFIED.,.F.,.F.,(4,2,4),(-0.371374848070398,-0.285575684483783,
-0.218017291375941),.UNSPECIFIED.);
#1331=B_SPLINE_CURVE_WITH_KNOTS('',3,(#38351,#38352,#38353,#38354,#38355,
#38356),.UNSPECIFIED.,.F.,.F.,(4,2,4),(-1.50046812968576,-1.43290973657793,
-1.34711057299131),.UNSPECIFIED.);
#1332=B_SPLINE_CURVE_WITH_KNOTS('',3,(#38550,#38551,#38552,#38553,#38554,
#38555),.UNSPECIFIED.,.F.,.F.,(4,2,4),(-0.524597258187126,-0.399172888862268,
0.),.UNSPECIFIED.);
#1333=B_SPLINE_CURVE_WITH_KNOTS('',3,(#38556,#38557,#38558,#38559,#38560,
#38561),.UNSPECIFIED.,.F.,.F.,(4,2,4),(-4.54956787028548,-4.15039498142321,
-4.02497061209835),.UNSPECIFIED.);
#1334=B_SPLINE_CURVE_WITH_KNOTS('',3,(#38564,#38565,#38566,#38567,#38568,
#38569),.UNSPECIFIED.,.F.,.F.,(4,2,4),(-4.54956787028547,-4.15039498142321,
-4.02497061209835),.UNSPECIFIED.);
#1335=B_SPLINE_CURVE_WITH_KNOTS('',3,(#38570,#38571,#38572,#38573,#38574,
#38575),.UNSPECIFIED.,.F.,.F.,(4,2,4),(-0.524597258187133,-0.399172888862267,
-1.88737914186277E-15),.UNSPECIFIED.);
#1336=B_SPLINE_CURVE_WITH_KNOTS('',3,(#38577,#38578,#38579,#38580,#38581,
#38582),.UNSPECIFIED.,.F.,.F.,(4,2,4),(-4.54910652185684,-4.14993363299457,
-4.02450926366971),.UNSPECIFIED.);
#1337=B_SPLINE_CURVE_WITH_KNOTS('',3,(#38583,#38584,#38585,#38586,#38587,
#38588),.UNSPECIFIED.,.F.,.F.,(4,2,4),(-0.524597258187127,-0.399172888862266,
0.),.UNSPECIFIED.);
#1338=B_SPLINE_CURVE_WITH_KNOTS('',3,(#38591,#38592,#38593,#38594,#38595,
#38596),.UNSPECIFIED.,.F.,.F.,(4,2,4),(-4.54910652185684,-4.14993363299457,
-4.0245092636697),.UNSPECIFIED.);
#1339=B_SPLINE_CURVE_WITH_KNOTS('',3,(#38597,#38598,#38599,#38600),
 .UNSPECIFIED.,.F.,.F.,(4,4),(-0.370064844470512,0.),.UNSPECIFIED.);
#1340=B_SPLINE_CURVE_WITH_KNOTS('',3,(#38604,#38605,#38606,#38607),
 .UNSPECIFIED.,.F.,.F.,(4,4),(-4.54956787028547,-4.17950302581496),
 .UNSPECIFIED.);
#1341=B_SPLINE_CURVE_WITH_KNOTS('',3,(#38608,#38609,#38610,#38611,#38612,
#38613),.UNSPECIFIED.,.F.,.F.,(4,2,4),(-0.524597258187134,-0.399172888862265,
0.),.UNSPECIFIED.);
#1342=B_SPLINE_CURVE_WITH_KNOTS('',3,(#38623,#38624,#38625,#38626,#38627,
#38628),.UNSPECIFIED.,.F.,.F.,(4,2,4),(-0.371374848070411,-0.285575684483777,
-0.218017291375943),.UNSPECIFIED.);
#1343=B_SPLINE_CURVE_WITH_KNOTS('',3,(#38638,#38639,#38640,#38641,#38642,
#38643),.UNSPECIFIED.,.F.,.F.,(4,2,4),(-1.50046812968577,-1.43290973657793,
-1.3471105729913),.UNSPECIFIED.);
#1344=B_SPLINE_CURVE_WITH_KNOTS('',3,(#38648,#38649,#38650,#38651,#38652,
#38653),.UNSPECIFIED.,.F.,.F.,(4,2,4),(-4.54956787028547,-4.15039498142321,
-4.02497061209834),.UNSPECIFIED.);
#1345=B_SPLINE_CURVE_WITH_KNOTS('',3,(#38654,#38655,#38656,#38657,#38658,
#38659),.UNSPECIFIED.,.F.,.F.,(4,2,4),(-0.524597258187132,-0.399172888862266,
0.),.UNSPECIFIED.);
#1346=B_SPLINE_CURVE_WITH_KNOTS('',3,(#38661,#38662,#38663,#38664,#38665,
#38666),.UNSPECIFIED.,.F.,.F.,(4,2,4),(-4.54910652185684,-4.14993363299457,
-4.02450926366973),.UNSPECIFIED.);
#1347=B_SPLINE_CURVE_WITH_KNOTS('',3,(#38667,#38668,#38669,#38670,#38671,
#38672),.UNSPECIFIED.,.F.,.F.,(4,2,4),(-0.524597258187128,-0.399172888862267,
0.),.UNSPECIFIED.);
#1348=B_SPLINE_CURVE_WITH_KNOTS('',3,(#38675,#38676,#38677,#38678,#38679,
#38680),.UNSPECIFIED.,.F.,.F.,(4,2,4),(-4.54956787028547,-4.15039498142321,
-4.02497061209834),.UNSPECIFIED.);
#1349=B_SPLINE_CURVE_WITH_KNOTS('',3,(#38681,#38682,#38683,#38684,#38685,
#38686),.UNSPECIFIED.,.F.,.F.,(4,2,4),(-0.524597258187134,-0.399172888862263,
0.),.UNSPECIFIED.);
#1350=B_SPLINE_CURVE_WITH_KNOTS('',3,(#38688,#38689,#38690,#38691,#38692,
#38693),.UNSPECIFIED.,.F.,.F.,(4,2,4),(-4.54910652185683,-4.14993363299457,
-4.0245092636697),.UNSPECIFIED.);
#1351=B_SPLINE_CURVE_WITH_KNOTS('',3,(#38694,#38695,#38696,#38697,#38698,
#38699),.UNSPECIFIED.,.F.,.F.,(4,2,4),(-0.524597258187127,-0.399172888862264,
0.),.UNSPECIFIED.);
#1352=B_SPLINE_CURVE_WITH_KNOTS('',3,(#38702,#38703,#38704,#38705,#38706,
#38707),.UNSPECIFIED.,.F.,.F.,(4,2,4),(-4.54910652185684,-4.14993363299457,
-4.02450926366971),.UNSPECIFIED.);
#1353=B_SPLINE_CURVE_WITH_KNOTS('',3,(#38710,#38711,#38712,#38713,#38714,
#38715),.UNSPECIFIED.,.F.,.F.,(4,2,4),(-0.52459725818713,-0.399172888862267,
0.),.UNSPECIFIED.);
#1354=B_SPLINE_CURVE_WITH_KNOTS('',3,(#38744,#38745,#38746,#38747,#38748,
#38749,#38750,#38751,#38752,#38753,#38754,#38755,#38756,#38757,#38758,#38759,
#38760,#38761,#38762,#38763,#38764,#38765,#38766,#38767,#38768,#38769,#38770,
#38771,#38772,#38773,#38774,#38775,#38776,#38777,#38778,#38779,#38780,#38781,
#38782,#38783,#38784,#38785,#38786),.UNSPECIFIED.,.F.,.F.,(4,3,3,3,3,3,
3,3,3,3,3,3,3,3,4),(0.,0.0872544796701012,0.179967974567206,0.275362932442676,
0.370587215980396,0.437499999999772,0.468749999999765,0.484374999999753,
0.49218749999974,0.496093749999741,0.499999999999741,0.638357505841048,
0.781776182157294,0.891012188806263,0.999999999999994),.UNSPECIFIED.);
#1355=B_SPLINE_CURVE_WITH_KNOTS('',3,(#38788,#38789,#38790,#38791,#38792,
#38793,#38794,#38795,#38796,#38797,#38798,#38799,#38800,#38801,#38802,#38803,
#38804,#38805,#38806,#38807,#38808,#38809,#38810,#38811,#38812,#38813,#38814,
#38815,#38816,#38817,#38818,#38819,#38820,#38821,#38822,#38823,#38824,#38825,
#38826,#38827,#38828,#38829,#38830,#38831,#38832,#38833,#38834,#38835,#38836),
 .UNSPECIFIED.,.F.,.F.,(4,3,3,3,3,3,3,3,3,3,3,3,3,3,3,3,4),(0.,0.09989275696205,
0.197149256723823,0.250000000001032,0.343701993891013,0.443601545051249,
0.497279897256218,0.498046875002055,0.500000000002058,0.571177947453751,
0.641445155754051,0.70984637527501,0.750000000001029,0.813786943013992,
0.876119581926588,0.938059790963294,1.),.UNSPECIFIED.);
#1356=B_SPLINE_CURVE_WITH_KNOTS('',3,(#38837,#38838,#38839,#38840,#38841,
#38842),.UNSPECIFIED.,.F.,.F.,(4,2,4),(-0.241266937338003,-0.121297446584125,
0.),.UNSPECIFIED.);
#1357=B_SPLINE_CURVE_WITH_KNOTS('',3,(#38923,#38924,#38925,#38926,#38927,
#38928),.UNSPECIFIED.,.F.,.F.,(4,2,4),(-0.241267240141802,-0.121297491113608,
0.),.UNSPECIFIED.);
#1358=B_SPLINE_CURVE_WITH_KNOTS('',3,(#38929,#38930,#38931,#38932,#38933,
#38934,#38935,#38936,#38937,#38938,#38939,#38940,#38941,#38942,#38943,#38944,
#38945,#38946,#38947,#38948,#38949,#38950,#38951,#38952,#38953,#38954,#38955,
#38956,#38957,#38958,#38959,#38960,#38961,#38962,#38963,#38964,#38965,#38966,
#38967,#38968,#38969,#38970,#38971,#38972,#38973,#38974,#38975,#38976,#38977),
 .UNSPECIFIED.,.F.,.F.,(4,3,3,3,3,3,3,3,3,3,3,3,3,3,3,3,4),(0.,0.0590959733778193,
0.12064791084943,0.183845110418003,0.245892786158591,0.299888306122572,
0.371749913788964,0.443192297459707,0.498046874999004,0.499999999999002,
0.502720163109487,0.593864795540943,0.686682262709001,0.782202229346505,
0.879448387345353,0.979332662309031,1.),.UNSPECIFIED.);
#1359=B_SPLINE_CURVE_WITH_KNOTS('',3,(#39175,#39176,#39177,#39178,#39179,
#39180),.UNSPECIFIED.,.F.,.F.,(4,2,4),(-0.241267240141382,-0.121297491113753,
0.),.UNSPECIFIED.);
#1360=B_SPLINE_CURVE_WITH_KNOTS('',3,(#39182,#39183,#39184,#39185,#39186,
#39187,#39188,#39189,#39190,#39191,#39192,#39193,#39194,#39195,#39196,#39197,
#39198,#39199,#39200,#39201,#39202,#39203,#39204,#39205,#39206,#39207,#39208,
#39209,#39210,#39211,#39212,#39213,#39214,#39215,#39216,#39217,#39218,#39219,
#39220,#39221,#39222,#39223,#39224,#39225,#39226,#39227,#39228,#39229,#39230),
 .UNSPECIFIED.,.F.,.F.,(4,3,3,3,3,3,3,3,3,3,3,3,3,3,3,3,4),(0.,0.0590959737305276,
0.120647911557508,0.183845111495701,0.245892787653034,0.299888306754146,
0.371749914989915,0.443192319371491,0.498046874999129,0.499999999999131,
0.502720163116374,0.593864796197773,0.686682264014154,0.78220223130903,
0.879448389968442,0.979332665575473,1.),.UNSPECIFIED.);
#1361=B_SPLINE_CURVE_WITH_KNOTS('',3,(#39262,#39263,#39264,#39265,#39266,
#39267,#39268,#39269,#39270,#39271,#39272,#39273,#39274,#39275,#39276,#39277,
#39278,#39279,#39280,#39281,#39282,#39283,#39284,#39285,#39286,#39287,#39288,
#39289,#39290,#39291,#39292,#39293,#39294,#39295,#39296,#39297,#39298,#39299,
#39300,#39301,#39302,#39303,#39304,#39305,#39306,#39307,#39308,#39309,#39310),
 .UNSPECIFIED.,.F.,.F.,(4,3,3,3,3,3,3,3,3,3,3,3,3,3,3,3,4),(0.,0.0998927578409832,
0.197149258553956,0.249999999999427,0.343701994843245,0.443601545265527,
0.497279897243239,0.498046874998851,0.499999999998844,0.571177948292924,
0.64144515738966,0.709846377640365,0.749999999999422,0.813786943534484,
0.876119582949847,0.938059791474924,1.),.UNSPECIFIED.);
#1362=B_SPLINE_CURVE_WITH_KNOTS('',3,(#39311,#39312,#39313,#39314,#39315,
#39316),.UNSPECIFIED.,.F.,.F.,(4,2,4),(-0.24126693733769,-0.121297446583894,
0.),.UNSPECIFIED.);
#1363=B_SPLINE_CURVE_WITH_KNOTS('',3,(#39456,#39457,#39458,#39459,#39460,
#39461,#39462,#39463),.UNSPECIFIED.,.F.,.F.,(4,2,2,4),(1.0455577725842,
1.95553903235196,3.95431621571259,4.41434897542879),.UNSPECIFIED.);
#1364=B_SPLINE_CURVE_WITH_KNOTS('',3,(#39475,#39476,#39477,#39478,#39479,
#39480,#39481,#39482),.UNSPECIFIED.,.F.,.F.,(4,2,2,4),(2.03056498878569,
2.99956672815959,4.49935009223939,4.8962823044381),.UNSPECIFIED.);
#1365=B_SPLINE_CURVE_WITH_KNOTS('',3,(#39636,#39637,#39638,#39639),
 .UNSPECIFIED.,.F.,.F.,(4,4),(-4.87675282368594,-1.08452914514666),
 .UNSPECIFIED.);
#1366=B_SPLINE_CURVE_WITH_KNOTS('',3,(#39644,#39645,#39646,#39647),
 .UNSPECIFIED.,.F.,.F.,(4,4),(-4.87667483628068,-1.08444993827179),
 .UNSPECIFIED.);
#1367=B_SPLINE_CURVE_WITH_KNOTS('',3,(#39650,#39651,#39652,#39653),
 .UNSPECIFIED.,.F.,.F.,(4,4),(-4.87674823462075,-1.08452453146112),
 .UNSPECIFIED.);
#1377=ELLIPSE('',#18924,7.07832284981318,6.99999999999854);
#1378=ELLIPSE('',#18926,7.07832284981318,6.99999999999854);
#1379=ELLIPSE('',#18948,7.0629889670351,6.99999999995947);
#1380=ELLIPSE('',#18952,7.06298896705052,6.9999999999871);
#1381=ELLIPSE('',#18962,23.999999999378,11.9999999993886);
#1382=ELLIPSE('',#18963,23.9999999977437,11.9999999977833);
#1383=ELLIPSE('',#18991,23.9999999996724,11.9999999997014);
#1384=ELLIPSE('',#18992,24.0000000005569,12.0000000005208);
#1385=ELLIPSE('',#19004,7.00423907309944,7.00000000002481);
#1386=ELLIPSE('',#19100,22.0866861336612,22.0548621009617);
#1387=ELLIPSE('',#19101,22.0591508859082,21.9667873157955);
#1388=ELLIPSE('',#19102,22.05915088596,21.9667873158956);
#1389=ELLIPSE('',#19103,22.0711672770103,22.010135576304);
#1390=ELLIPSE('',#19104,22.0646581901642,22.0091682784596);
#1391=ELLIPSE('',#19105,22.0748759515261,22.039900950448);
#1392=ELLIPSE('',#19358,62.7132858513459,44.3213853810186);
#1393=ELLIPSE('',#19361,62.713288482779,44.3213890977139);
#1394=ELLIPSE('',#19364,62.7132852238632,44.321384494158);
#1395=ELLIPSE('',#19365,44.5345980614777,31.4244600121006);
#1396=ELLIPSE('',#19367,44.5346010360152,31.424464205272);
#1397=ELLIPSE('',#19369,62.7132944274914,44.3213974951955);
#1398=ELLIPSE('',#19645,4.50272511841123,4.49999999999998);
#1399=ELLIPSE('',#19681,6.92820323083716,6.00000000034999);
#1400=ELLIPSE('',#19688,23.9999999687057,11.9999999731157);
#1401=ELLIPSE('',#19689,6.92820323020547,5.99999999993053);
#1402=ELLIPSE('',#19731,23.9999999658975,11.9999999709002);
#1403=ELLIPSE('',#19733,6.92820323026176,5.99999999998559);
#1404=ELLIPSE('',#19740,6.92820323018877,6.00000000002855);
#1405=ELLIPSE('',#19757,6.08833509735678,4.61528466193146);
#1406=ELLIPSE('',#19807,6.08086351685543,4.60377817015316);
#1407=ELLIPSE('',#19811,6.08735970830141,4.61379430849458);
#1790=LINE('',#30645,#3363);
#1791=LINE('',#30648,#3364);
#1792=LINE('',#30651,#3365);
#1793=LINE('',#30654,#3366);
#1794=LINE('',#30656,#3367);
#1795=LINE('',#30665,#3368);
#1796=LINE('',#30669,#3369);
#1797=LINE('',#30675,#3370);
#1798=LINE('',#30681,#3371);
#1799=LINE('',#30683,#3372);
#1800=LINE('',#30685,#3373);
#1801=LINE('',#30687,#3374);
#1802=LINE('',#30689,#3375);
#1803=LINE('',#30690,#3376);
#1804=LINE('',#30693,#3377);
#1805=LINE('',#30695,#3378);
#1806=LINE('',#30696,#3379);
#1807=LINE('',#30699,#3380);
#1808=LINE('',#30700,#3381);
#1809=LINE('',#30703,#3382);
#1810=LINE('',#30705,#3383);
#1811=LINE('',#30706,#3384);
#1812=LINE('',#30709,#3385);
#1813=LINE('',#30710,#3386);
#1814=LINE('',#30713,#3387);
#1815=LINE('',#30714,#3388);
#1816=LINE('',#30717,#3389);
#1817=LINE('',#30718,#3390);
#1818=LINE('',#30720,#3391);
#1819=LINE('',#30737,#3392);
#1820=LINE('',#30752,#3393);
#1821=LINE('',#30767,#3394);
#1822=LINE('',#30800,#3395);
#1823=LINE('',#30806,#3396);
#1824=LINE('',#30812,#3397);
#1825=LINE('',#30818,#3398);
#1826=LINE('',#30827,#3399);
#1827=LINE('',#30887,#3400);
#1828=LINE('',#30893,#3401);
#1829=LINE('',#30936,#3402);
#1830=LINE('',#30945,#3403);
#1831=LINE('',#30951,#3404);
#1832=LINE('',#30975,#3405);
#1833=LINE('',#30995,#3406);
#1834=LINE('',#31018,#3407);
#1835=LINE('',#31038,#3408);
#1836=LINE('',#31051,#3409);
#1837=LINE('',#31071,#3410);
#1838=LINE('',#31102,#3411);
#1839=LINE('',#31105,#3412);
#1840=LINE('',#31128,#3413);
#1841=LINE('',#31148,#3414);
#1842=LINE('',#31156,#3415);
#1843=LINE('',#31159,#3416);
#1844=LINE('',#31164,#3417);
#1845=LINE('',#31170,#3418);
#1846=LINE('',#31176,#3419);
#1847=LINE('',#31182,#3420);
#1848=LINE('',#31188,#3421);
#1849=LINE('',#31195,#3422);
#1850=LINE('',#31215,#3423);
#1851=LINE('',#31221,#3424);
#1852=LINE('',#31243,#3425);
#1853=LINE('',#31248,#3426);
#1854=LINE('',#31264,#3427);
#1855=LINE('',#31293,#3428);
#1856=LINE('',#31367,#3429);
#1857=LINE('',#31376,#3430);
#1858=LINE('',#31379,#3431);
#1859=LINE('',#31385,#3432);
#1860=LINE('',#31388,#3433);
#1861=LINE('',#31390,#3434);
#1862=LINE('',#31393,#3435);
#1863=LINE('',#31396,#3436);
#1864=LINE('',#31402,#3437);
#1865=LINE('',#31408,#3438);
#1866=LINE('',#31414,#3439);
#1867=LINE('',#31420,#3440);
#1868=LINE('',#31426,#3441);
#1869=LINE('',#31430,#3442);
#1870=LINE('',#31434,#3443);
#1871=LINE('',#31439,#3444);
#1872=LINE('',#31445,#3445);
#1873=LINE('',#31451,#3446);
#1874=LINE('',#31455,#3447);
#1875=LINE('',#31461,#3448);
#1876=LINE('',#31467,#3449);
#1877=LINE('',#31473,#3450);
#1878=LINE('',#31479,#3451);
#1879=LINE('',#31485,#3452);
#1880=LINE('',#31491,#3453);
#1881=LINE('',#31498,#3454);
#1882=LINE('',#31501,#3455);
#1883=LINE('',#31504,#3456);
#1884=LINE('',#31513,#3457);
#1885=LINE('',#31516,#3458);
#1886=LINE('',#31522,#3459);
#1887=LINE('',#31528,#3460);
#1888=LINE('',#31593,#3461);
#1889=LINE('',#31597,#3462);
#1890=LINE('',#31649,#3463);
#1891=LINE('',#31655,#3464);
#1892=LINE('',#31659,#3465);
#1893=LINE('',#31665,#3466);
#1894=LINE('',#31674,#3467);
#1895=LINE('',#31677,#3468);
#1896=LINE('',#31680,#3469);
#1897=LINE('',#31730,#3470);
#1898=LINE('',#31786,#3471);
#1899=LINE('',#31803,#3472);
#1900=LINE('',#31818,#3473);
#1901=LINE('',#31862,#3474);
#1902=LINE('',#31864,#3475);
#1903=LINE('',#31936,#3476);
#1904=LINE('',#31938,#3477);
#1905=LINE('',#32025,#3478);
#1906=LINE('',#32027,#3479);
#1907=LINE('',#32029,#3480);
#1908=LINE('',#32031,#3481);
#1909=LINE('',#32033,#3482);
#1910=LINE('',#32034,#3483);
#1911=LINE('',#32038,#3484);
#1912=LINE('',#32040,#3485);
#1913=LINE('',#32042,#3486);
#1914=LINE('',#32044,#3487);
#1915=LINE('',#32046,#3488);
#1916=LINE('',#32047,#3489);
#1917=LINE('',#32051,#3490);
#1918=LINE('',#32053,#3491);
#1919=LINE('',#32055,#3492);
#1920=LINE('',#32057,#3493);
#1921=LINE('',#32059,#3494);
#1922=LINE('',#32060,#3495);
#1923=LINE('',#32064,#3496);
#1924=LINE('',#32066,#3497);
#1925=LINE('',#32068,#3498);
#1926=LINE('',#32070,#3499);
#1927=LINE('',#32072,#3500);
#1928=LINE('',#32073,#3501);
#1929=LINE('',#32079,#3502);
#1930=LINE('',#32087,#3503);
#1931=LINE('',#32092,#3504);
#1932=LINE('',#32100,#3505);
#1933=LINE('',#32107,#3506);
#1934=LINE('',#32109,#3507);
#1935=LINE('',#32111,#3508);
#1936=LINE('',#32113,#3509);
#1937=LINE('',#32115,#3510);
#1938=LINE('',#32116,#3511);
#1939=LINE('',#32120,#3512);
#1940=LINE('',#32122,#3513);
#1941=LINE('',#32124,#3514);
#1942=LINE('',#32126,#3515);
#1943=LINE('',#32128,#3516);
#1944=LINE('',#32129,#3517);
#1945=LINE('',#32133,#3518);
#1946=LINE('',#32134,#3519);
#1947=LINE('',#32135,#3520);
#1948=LINE('',#32138,#3521);
#1949=LINE('',#32139,#3522);
#1950=LINE('',#32142,#3523);
#1951=LINE('',#32143,#3524);
#1952=LINE('',#32146,#3525);
#1953=LINE('',#32147,#3526);
#1954=LINE('',#32150,#3527);
#1955=LINE('',#32151,#3528);
#1956=LINE('',#32153,#3529);
#1957=LINE('',#32157,#3530);
#1958=LINE('',#32159,#3531);
#1959=LINE('',#32161,#3532);
#1960=LINE('',#32163,#3533);
#1961=LINE('',#32168,#3534);
#1962=LINE('',#32173,#3535);
#1963=LINE('',#32175,#3536);
#1964=LINE('',#32177,#3537);
#1965=LINE('',#32182,#3538);
#1966=LINE('',#32183,#3539);
#1967=LINE('',#32184,#3540);
#1968=LINE('',#32187,#3541);
#1969=LINE('',#32188,#3542);
#1970=LINE('',#32191,#3543);
#1971=LINE('',#32192,#3544);
#1972=LINE('',#32195,#3545);
#1973=LINE('',#32196,#3546);
#1974=LINE('',#32199,#3547);
#1975=LINE('',#32200,#3548);
#1976=LINE('',#32202,#3549);
#1977=LINE('',#32206,#3550);
#1978=LINE('',#32208,#3551);
#1979=LINE('',#32210,#3552);
#1980=LINE('',#32212,#3553);
#1981=LINE('',#32217,#3554);
#1982=LINE('',#32223,#3555);
#1983=LINE('',#32224,#3556);
#1984=LINE('',#32226,#3557);
#1985=LINE('',#32231,#3558);
#1986=LINE('',#32232,#3559);
#1987=LINE('',#32233,#3560);
#1988=LINE('',#32236,#3561);
#1989=LINE('',#32237,#3562);
#1990=LINE('',#32240,#3563);
#1991=LINE('',#32241,#3564);
#1992=LINE('',#32244,#3565);
#1993=LINE('',#32245,#3566);
#1994=LINE('',#32248,#3567);
#1995=LINE('',#32249,#3568);
#1996=LINE('',#32251,#3569);
#1997=LINE('',#32255,#3570);
#1998=LINE('',#32257,#3571);
#1999=LINE('',#32259,#3572);
#2000=LINE('',#32261,#3573);
#2001=LINE('',#32266,#3574);
#2002=LINE('',#32272,#3575);
#2003=LINE('',#32273,#3576);
#2004=LINE('',#32275,#3577);
#2005=LINE('',#32278,#3578);
#2006=LINE('',#32280,#3579);
#2007=LINE('',#32282,#3580);
#2008=LINE('',#32286,#3581);
#2009=LINE('',#32287,#3582);
#2010=LINE('',#32288,#3583);
#2011=LINE('',#32292,#3584);
#2012=LINE('',#32293,#3585);
#2013=LINE('',#32294,#3586);
#2014=LINE('',#32297,#3587);
#2015=LINE('',#32298,#3588);
#2016=LINE('',#32301,#3589);
#2017=LINE('',#32302,#3590);
#2018=LINE('',#32305,#3591);
#2019=LINE('',#32306,#3592);
#2020=LINE('',#32309,#3593);
#2021=LINE('',#32310,#3594);
#2022=LINE('',#32312,#3595);
#2023=LINE('',#32315,#3596);
#2024=LINE('',#32317,#3597);
#2025=LINE('',#32319,#3598);
#2026=LINE('',#32323,#3599);
#2027=LINE('',#32328,#3600);
#2028=LINE('',#32329,#3601);
#2029=LINE('',#32333,#3602);
#2030=LINE('',#32335,#3603);
#2031=LINE('',#32339,#3604);
#2032=LINE('',#32340,#3605);
#2033=LINE('',#32343,#3606);
#2034=LINE('',#32347,#3607);
#2035=LINE('',#32351,#3608);
#2036=LINE('',#32355,#3609);
#2037=LINE('',#32356,#3610);
#2038=LINE('',#32359,#3611);
#2039=LINE('',#32363,#3612);
#2040=LINE('',#32367,#3613);
#2041=LINE('',#32371,#3614);
#2042=LINE('',#32372,#3615);
#2043=LINE('',#32377,#3616);
#2044=LINE('',#32381,#3617);
#2045=LINE('',#32382,#3618);
#2046=LINE('',#32385,#3619);
#2047=LINE('',#32391,#3620);
#2048=LINE('',#32393,#3621);
#2049=LINE('',#32397,#3622);
#2050=LINE('',#32401,#3623);
#2051=LINE('',#32405,#3624);
#2052=LINE('',#32409,#3625);
#2053=LINE('',#32415,#3626);
#2054=LINE('',#32417,#3627);
#2055=LINE('',#32421,#3628);
#2056=LINE('',#32425,#3629);
#2057=LINE('',#32429,#3630);
#2058=LINE('',#32433,#3631);
#2059=LINE('',#32438,#3632);
#2060=LINE('',#32440,#3633);
#2061=LINE('',#32445,#3634);
#2062=LINE('',#32446,#3635);
#2063=LINE('',#32448,#3636);
#2064=LINE('',#32451,#3637);
#2065=LINE('',#32454,#3638);
#2066=LINE('',#32457,#3639);
#2067=LINE('',#32460,#3640);
#2068=LINE('',#32462,#3641);
#2069=LINE('',#32465,#3642);
#2070=LINE('',#32468,#3643);
#2071=LINE('',#32479,#3644);
#2072=LINE('',#32481,#3645);
#2073=LINE('',#32492,#3646);
#2074=LINE('',#32501,#3647);
#2075=LINE('',#32517,#3648);
#2076=LINE('',#32519,#3649);
#2077=LINE('',#32530,#3650);
#2078=LINE('',#32544,#3651);
#2079=LINE('',#32547,#3652);
#2080=LINE('',#32548,#3653);
#2081=LINE('',#32552,#3654);
#2082=LINE('',#32554,#3655);
#2083=LINE('',#32569,#3656);
#2084=LINE('',#32571,#3657);
#2085=LINE('',#32582,#3658);
#2086=LINE('',#32598,#3659);
#2087=LINE('',#32888,#3660);
#2088=LINE('',#32889,#3661);
#2089=LINE('',#32892,#3662);
#2090=LINE('',#32893,#3663);
#2091=LINE('',#32897,#3664);
#2092=LINE('',#32900,#3665);
#2093=LINE('',#32901,#3666);
#2094=LINE('',#32905,#3667);
#2095=LINE('',#32908,#3668);
#2096=LINE('',#32909,#3669);
#2097=LINE('',#32913,#3670);
#2098=LINE('',#32915,#3671);
#2099=LINE('',#32924,#3672);
#2100=LINE('',#32925,#3673);
#2101=LINE('',#32966,#3674);
#2102=LINE('',#33001,#3675);
#2103=LINE('',#33058,#3676);
#2104=LINE('',#33074,#3677);
#2105=LINE('',#33102,#3678);
#2106=LINE('',#33124,#3679);
#2107=LINE('',#33154,#3680);
#2108=LINE('',#33176,#3681);
#2109=LINE('',#33415,#3682);
#2110=LINE('',#33431,#3683);
#2111=LINE('',#33440,#3684);
#2112=LINE('',#33456,#3685);
#2113=LINE('',#33465,#3686);
#2114=LINE('',#33635,#3687);
#2115=LINE('',#33707,#3688);
#2116=LINE('',#33789,#3689);
#2117=LINE('',#33867,#3690);
#2118=LINE('',#33949,#3691);
#2119=LINE('',#34027,#3692);
#2120=LINE('',#35967,#3693);
#2121=LINE('',#35986,#3694);
#2122=LINE('',#36078,#3695);
#2123=LINE('',#36094,#3696);
#2124=LINE('',#36124,#3697);
#2125=LINE('',#36146,#3698);
#2126=LINE('',#36176,#3699);
#2127=LINE('',#36198,#3700);
#2128=LINE('',#36232,#3701);
#2129=LINE('',#36236,#3702);
#2130=LINE('',#36240,#3703);
#2131=LINE('',#36244,#3704);
#2132=LINE('',#36250,#3705);
#2133=LINE('',#36251,#3706);
#2134=LINE('',#36255,#3707);
#2135=LINE('',#36259,#3708);
#2136=LINE('',#36262,#3709);
#2137=LINE('',#36267,#3710);
#2138=LINE('',#36271,#3711);
#2139=LINE('',#36277,#3712);
#2140=LINE('',#36281,#3713);
#2141=LINE('',#36291,#3714);
#2142=LINE('',#36296,#3715);
#2143=LINE('',#36300,#3716);
#2144=LINE('',#36304,#3717);
#2145=LINE('',#36309,#3718);
#2146=LINE('',#36311,#3719);
#2147=LINE('',#36312,#3720);
#2148=LINE('',#36315,#3721);
#2149=LINE('',#36317,#3722);
#2150=LINE('',#36318,#3723);
#2151=LINE('',#36337,#3724);
#2152=LINE('',#36339,#3725);
#2153=LINE('',#36340,#3726);
#2154=LINE('',#36374,#3727);
#2155=LINE('',#36377,#3728);
#2156=LINE('',#36394,#3729);
#2157=LINE('',#36452,#3730);
#2158=LINE('',#36520,#3731);
#2159=LINE('',#36664,#3732);
#2160=LINE('',#36738,#3733);
#2161=LINE('',#36883,#3734);
#2162=LINE('',#36958,#3735);
#2163=LINE('',#37100,#3736);
#2164=LINE('',#37168,#3737);
#2165=LINE('',#37283,#3738);
#2166=LINE('',#37285,#3739);
#2167=LINE('',#37287,#3740);
#2168=LINE('',#37289,#3741);
#2169=LINE('',#37291,#3742);
#2170=LINE('',#37292,#3743);
#2171=LINE('',#37296,#3744);
#2172=LINE('',#37298,#3745);
#2173=LINE('',#37300,#3746);
#2174=LINE('',#37302,#3747);
#2175=LINE('',#37304,#3748);
#2176=LINE('',#37305,#3749);
#2177=LINE('',#37307,#3750);
#2178=LINE('',#37309,#3751);
#2179=LINE('',#37311,#3752);
#2180=LINE('',#37313,#3753);
#2181=LINE('',#37318,#3754);
#2182=LINE('',#37325,#3755);
#2183=LINE('',#37326,#3756);
#2184=LINE('',#37329,#3757);
#2185=LINE('',#37330,#3758);
#2186=LINE('',#37337,#3759);
#2187=LINE('',#37341,#3760);
#2188=LINE('',#37344,#3761);
#2189=LINE('',#37355,#3762);
#2190=LINE('',#37356,#3763);
#2191=LINE('',#37359,#3764);
#2192=LINE('',#37360,#3765);
#2193=LINE('',#37367,#3766);
#2194=LINE('',#37379,#3767);
#2195=LINE('',#37380,#3768);
#2196=LINE('',#37383,#3769);
#2197=LINE('',#37384,#3770);
#2198=LINE('',#37391,#3771);
#2199=LINE('',#37395,#3772);
#2200=LINE('',#37398,#3773);
#2201=LINE('',#37409,#3774);
#2202=LINE('',#37410,#3775);
#2203=LINE('',#37413,#3776);
#2204=LINE('',#37414,#3777);
#2205=LINE('',#37421,#3778);
#2206=LINE('',#37425,#3779);
#2207=LINE('',#37430,#3780);
#2208=LINE('',#37432,#3781);
#2209=LINE('',#37433,#3782);
#2210=LINE('',#37436,#3783);
#2211=LINE('',#37437,#3784);
#2212=LINE('',#37440,#3785);
#2213=LINE('',#37441,#3786);
#2214=LINE('',#37444,#3787);
#2215=LINE('',#37445,#3788);
#2216=LINE('',#37448,#3789);
#2217=LINE('',#37449,#3790);
#2218=LINE('',#37451,#3791);
#2219=LINE('',#37454,#3792);
#2220=LINE('',#37456,#3793);
#2221=LINE('',#37457,#3794);
#2222=LINE('',#37460,#3795);
#2223=LINE('',#37461,#3796);
#2224=LINE('',#37464,#3797);
#2225=LINE('',#37465,#3798);
#2226=LINE('',#37468,#3799);
#2227=LINE('',#37469,#3800);
#2228=LINE('',#37472,#3801);
#2229=LINE('',#37473,#3802);
#2230=LINE('',#37475,#3803);
#2231=LINE('',#37481,#3804);
#2232=LINE('',#37484,#3805);
#2233=LINE('',#37490,#3806);
#2234=LINE('',#37493,#3807);
#2235=LINE('',#37497,#3808);
#2236=LINE('',#37499,#3809);
#2237=LINE('',#37501,#3810);
#2238=LINE('',#37502,#3811);
#2239=LINE('',#37506,#3812);
#2240=LINE('',#37510,#3813);
#2241=LINE('',#37511,#3814);
#2242=LINE('',#37512,#3815);
#2243=LINE('',#37515,#3816);
#2244=LINE('',#37517,#3817);
#2245=LINE('',#37524,#3818);
#2246=LINE('',#37527,#3819);
#2247=LINE('',#37533,#3820);
#2248=LINE('',#37536,#3821);
#2249=LINE('',#37542,#3822);
#2250=LINE('',#37545,#3823);
#2251=LINE('',#37547,#3824);
#2252=LINE('',#37548,#3825);
#2253=LINE('',#37549,#3826);
#2254=LINE('',#37550,#3827);
#2255=LINE('',#37551,#3828);
#2256=LINE('',#37553,#3829);
#2257=LINE('',#37556,#3830);
#2258=LINE('',#37557,#3831);
#2259=LINE('',#37562,#3832);
#2260=LINE('',#37563,#3833);
#2261=LINE('',#37568,#3834);
#2262=LINE('',#37570,#3835);
#2263=LINE('',#37571,#3836);
#2264=LINE('',#37574,#3837);
#2265=LINE('',#37576,#3838);
#2266=LINE('',#37577,#3839);
#2267=LINE('',#37580,#3840);
#2268=LINE('',#37584,#3841);
#2269=LINE('',#37586,#3842);
#2270=LINE('',#37588,#3843);
#2271=LINE('',#37591,#3844);
#2272=LINE('',#37595,#3845);
#2273=LINE('',#37599,#3846);
#2274=LINE('',#37603,#3847);
#2275=LINE('',#37605,#3848);
#2276=LINE('',#37607,#3849);
#2277=LINE('',#37608,#3850);
#2278=LINE('',#37610,#3851);
#2279=LINE('',#37611,#3852);
#2280=LINE('',#37615,#3853);
#2281=LINE('',#37618,#3854);
#2282=LINE('',#37619,#3855);
#2283=LINE('',#37622,#3856);
#2284=LINE('',#37623,#3857);
#2285=LINE('',#37627,#3858);
#2286=LINE('',#37628,#3859);
#2287=LINE('',#37630,#3860);
#2288=LINE('',#37631,#3861);
#2289=LINE('',#37634,#3862);
#2290=LINE('',#37636,#3863);
#2291=LINE('',#37637,#3864);
#2292=LINE('',#37641,#3865);
#2293=LINE('',#37642,#3866);
#2294=LINE('',#37643,#3867);
#2295=LINE('',#37646,#3868);
#2296=LINE('',#37649,#3869);
#2297=LINE('',#37653,#3870);
#2298=LINE('',#37657,#3871);
#2299=LINE('',#37661,#3872);
#2300=LINE('',#37663,#3873);
#2301=LINE('',#37664,#3874);
#2302=LINE('',#37666,#3875);
#2303=LINE('',#37667,#3876);
#2304=LINE('',#37670,#3877);
#2305=LINE('',#37672,#3878);
#2306=LINE('',#37673,#3879);
#2307=LINE('',#37676,#3880);
#2308=LINE('',#37680,#3881);
#2309=LINE('',#37682,#3882);
#2310=LINE('',#37684,#3883);
#2311=LINE('',#37687,#3884);
#2312=LINE('',#37691,#3885);
#2313=LINE('',#37695,#3886);
#2314=LINE('',#37699,#3887);
#2315=LINE('',#37701,#3888);
#2316=LINE('',#37702,#3889);
#2317=LINE('',#37704,#3890);
#2318=LINE('',#37705,#3891);
#2319=LINE('',#37709,#3892);
#2320=LINE('',#37713,#3893);
#2321=LINE('',#37716,#3894);
#2322=LINE('',#37718,#3895);
#2323=LINE('',#37719,#3896);
#2324=LINE('',#37722,#3897);
#2325=LINE('',#37723,#3898);
#2326=LINE('',#37726,#3899);
#2327=LINE('',#37730,#3900);
#2328=LINE('',#37732,#3901);
#2329=LINE('',#37734,#3902);
#2330=LINE('',#37737,#3903);
#2331=LINE('',#37741,#3904);
#2332=LINE('',#37743,#3905);
#2333=LINE('',#37745,#3906);
#2334=LINE('',#37747,#3907);
#2335=LINE('',#37749,#3908);
#2336=LINE('',#37750,#3909);
#2337=LINE('',#37754,#3910);
#2338=LINE('',#37756,#3911);
#2339=LINE('',#37758,#3912);
#2340=LINE('',#37759,#3913);
#2341=LINE('',#37764,#3914);
#2342=LINE('',#37765,#3915);
#2343=LINE('',#37767,#3916);
#2344=LINE('',#37769,#3917);
#2345=LINE('',#37773,#3918);
#2346=LINE('',#37776,#3919);
#2347=LINE('',#37779,#3920);
#2348=LINE('',#37781,#3921);
#2349=LINE('',#37782,#3922);
#2350=LINE('',#37785,#3923);
#2351=LINE('',#37789,#3924);
#2352=LINE('',#37790,#3925);
#2353=LINE('',#37793,#3926);
#2354=LINE('',#37794,#3927);
#2355=LINE('',#37797,#3928);
#2356=LINE('',#37798,#3929);
#2357=LINE('',#37801,#3930);
#2358=LINE('',#37805,#3931);
#2359=LINE('',#37807,#3932);
#2360=LINE('',#37808,#3933);
#2361=LINE('',#37811,#3934);
#2362=LINE('',#37813,#3935);
#2363=LINE('',#37815,#3936);
#2364=LINE('',#37819,#3937);
#2365=LINE('',#37822,#3938);
#2366=LINE('',#37825,#3939);
#2367=LINE('',#37827,#3940);
#2368=LINE('',#37828,#3941);
#2369=LINE('',#37831,#3942);
#2370=LINE('',#37835,#3943);
#2371=LINE('',#37836,#3944);
#2372=LINE('',#37839,#3945);
#2373=LINE('',#37840,#3946);
#2374=LINE('',#37843,#3947);
#2375=LINE('',#37844,#3948);
#2376=LINE('',#37847,#3949);
#2377=LINE('',#37851,#3950);
#2378=LINE('',#37853,#3951);
#2379=LINE('',#37854,#3952);
#2380=LINE('',#37857,#3953);
#2381=LINE('',#37859,#3954);
#2382=LINE('',#37861,#3955);
#2383=LINE('',#37865,#3956);
#2384=LINE('',#37868,#3957);
#2385=LINE('',#37871,#3958);
#2386=LINE('',#37873,#3959);
#2387=LINE('',#37874,#3960);
#2388=LINE('',#37877,#3961);
#2389=LINE('',#37881,#3962);
#2390=LINE('',#37882,#3963);
#2391=LINE('',#37885,#3964);
#2392=LINE('',#37886,#3965);
#2393=LINE('',#37889,#3966);
#2394=LINE('',#37890,#3967);
#2395=LINE('',#37893,#3968);
#2396=LINE('',#37897,#3969);
#2397=LINE('',#37899,#3970);
#2398=LINE('',#37900,#3971);
#2399=LINE('',#37903,#3972);
#2400=LINE('',#37905,#3973);
#2401=LINE('',#37907,#3974);
#2402=LINE('',#37911,#3975);
#2403=LINE('',#37914,#3976);
#2404=LINE('',#37917,#3977);
#2405=LINE('',#37919,#3978);
#2406=LINE('',#37920,#3979);
#2407=LINE('',#37923,#3980);
#2408=LINE('',#37927,#3981);
#2409=LINE('',#37928,#3982);
#2410=LINE('',#37931,#3983);
#2411=LINE('',#37932,#3984);
#2412=LINE('',#37935,#3985);
#2413=LINE('',#37936,#3986);
#2414=LINE('',#37939,#3987);
#2415=LINE('',#37943,#3988);
#2416=LINE('',#37944,#3989);
#2417=LINE('',#37947,#3990);
#2418=LINE('',#37949,#3991);
#2419=LINE('',#37950,#3992);
#2420=LINE('',#37953,#3993);
#2421=LINE('',#37954,#3994);
#2422=LINE('',#37957,#3995);
#2423=LINE('',#37958,#3996);
#2424=LINE('',#37961,#3997);
#2425=LINE('',#37962,#3998);
#2426=LINE('',#37965,#3999);
#2427=LINE('',#37966,#4000);
#2428=LINE('',#37968,#4001);
#2429=LINE('',#37972,#4002);
#2430=LINE('',#37973,#4003);
#2431=LINE('',#37975,#4004);
#2432=LINE('',#37977,#4005);
#2433=LINE('',#37985,#4006);
#2434=LINE('',#37987,#4007);
#2435=LINE('',#37988,#4008);
#2436=LINE('',#37992,#4009);
#2437=LINE('',#37996,#4010);
#2438=LINE('',#37999,#4011);
#2439=LINE('',#38003,#4012);
#2440=LINE('',#38004,#4013);
#2441=LINE('',#38007,#4014);
#2442=LINE('',#38011,#4015);
#2443=LINE('',#38012,#4016);
#2444=LINE('',#38015,#4017);
#2445=LINE('',#38019,#4018);
#2446=LINE('',#38021,#4019);
#2447=LINE('',#38023,#4020);
#2448=LINE('',#38025,#4021);
#2449=LINE('',#38027,#4022);
#2450=LINE('',#38030,#4023);
#2451=LINE('',#38034,#4024);
#2452=LINE('',#38037,#4025);
#2453=LINE('',#38040,#4026);
#2454=LINE('',#38041,#4027);
#2455=LINE('',#38044,#4028);
#2456=LINE('',#38048,#4029);
#2457=LINE('',#38049,#4030);
#2458=LINE('',#38052,#4031);
#2459=LINE('',#38056,#4032);
#2460=LINE('',#38060,#4033);
#2461=LINE('',#38064,#4034);
#2462=LINE('',#38065,#4035);
#2463=LINE('',#38072,#4036);
#2464=LINE('',#38074,#4037);
#2465=LINE('',#38076,#4038);
#2466=LINE('',#38078,#4039);
#2467=LINE('',#38080,#4040);
#2468=LINE('',#38081,#4041);
#2469=LINE('',#38083,#4042);
#2470=LINE('',#38084,#4043);
#2471=LINE('',#38086,#4044);
#2472=LINE('',#38088,#4045);
#2473=LINE('',#38090,#4046);
#2474=LINE('',#38092,#4047);
#2475=LINE('',#38094,#4048);
#2476=LINE('',#38097,#4049);
#2477=LINE('',#38099,#4050);
#2478=LINE('',#38101,#4051);
#2479=LINE('',#38103,#4052);
#2480=LINE('',#38105,#4053);
#2481=LINE('',#38107,#4054);
#2482=LINE('',#38109,#4055);
#2483=LINE('',#38114,#4056);
#2484=LINE('',#38116,#4057);
#2485=LINE('',#38118,#4058);
#2486=LINE('',#38120,#4059);
#2487=LINE('',#38122,#4060);
#2488=LINE('',#38124,#4061);
#2489=LINE('',#38126,#4062);
#2490=LINE('',#38127,#4063);
#2491=LINE('',#38135,#4064);
#2492=LINE('',#38140,#4065);
#2493=LINE('',#38142,#4066);
#2494=LINE('',#38144,#4067);
#2495=LINE('',#38146,#4068);
#2496=LINE('',#38148,#4069);
#2497=LINE('',#38149,#4070);
#2498=LINE('',#38150,#4071);
#2499=LINE('',#38154,#4072);
#2500=LINE('',#38156,#4073);
#2501=LINE('',#38158,#4074);
#2502=LINE('',#38160,#4075);
#2503=LINE('',#38162,#4076);
#2504=LINE('',#38163,#4077);
#2505=LINE('',#38177,#4078);
#2506=LINE('',#38179,#4079);
#2507=LINE('',#38180,#4080);
#2508=LINE('',#38183,#4081);
#2509=LINE('',#38184,#4082);
#2510=LINE('',#38187,#4083);
#2511=LINE('',#38188,#4084);
#2512=LINE('',#38191,#4085);
#2513=LINE('',#38192,#4086);
#2514=LINE('',#38195,#4087);
#2515=LINE('',#38196,#4088);
#2516=LINE('',#38198,#4089);
#2517=LINE('',#38201,#4090);
#2518=LINE('',#38204,#4091);
#2519=LINE('',#38219,#4092);
#2520=LINE('',#38220,#4093);
#2521=LINE('',#38224,#4094);
#2522=LINE('',#38226,#4095);
#2523=LINE('',#38228,#4096);
#2524=LINE('',#38230,#4097);
#2525=LINE('',#38232,#4098);
#2526=LINE('',#38233,#4099);
#2527=LINE('',#38237,#4100);
#2528=LINE('',#38239,#4101);
#2529=LINE('',#38241,#4102);
#2530=LINE('',#38243,#4103);
#2531=LINE('',#38245,#4104);
#2532=LINE('',#38246,#4105);
#2533=LINE('',#38250,#4106);
#2534=LINE('',#38252,#4107);
#2535=LINE('',#38254,#4108);
#2536=LINE('',#38256,#4109);
#2537=LINE('',#38258,#4110);
#2538=LINE('',#38259,#4111);
#2539=LINE('',#38263,#4112);
#2540=LINE('',#38266,#4113);
#2541=LINE('',#38267,#4114);
#2542=LINE('',#38273,#4115);
#2543=LINE('',#38276,#4116);
#2544=LINE('',#38277,#4117);
#2545=LINE('',#38286,#4118);
#2546=LINE('',#38289,#4119);
#2547=LINE('',#38290,#4120);
#2548=LINE('',#38296,#4121);
#2549=LINE('',#38299,#4122);
#2550=LINE('',#38300,#4123);
#2551=LINE('',#38305,#4124);
#2552=LINE('',#38307,#4125);
#2553=LINE('',#38308,#4126);
#2554=LINE('',#38311,#4127);
#2555=LINE('',#38312,#4128);
#2556=LINE('',#38315,#4129);
#2557=LINE('',#38316,#4130);
#2558=LINE('',#38319,#4131);
#2559=LINE('',#38320,#4132);
#2560=LINE('',#38323,#4133);
#2561=LINE('',#38324,#4134);
#2562=LINE('',#38326,#4135);
#2563=LINE('',#38331,#4136);
#2564=LINE('',#38332,#4137);
#2565=LINE('',#38344,#4138);
#2566=LINE('',#38347,#4139);
#2567=LINE('',#38350,#4140);
#2568=LINE('',#38364,#4141);
#2569=LINE('',#38366,#4142);
#2570=LINE('',#38368,#4143);
#2571=LINE('',#38370,#4144);
#2572=LINE('',#38372,#4145);
#2573=LINE('',#38373,#4146);
#2574=LINE('',#38377,#4147);
#2575=LINE('',#38379,#4148);
#2576=LINE('',#38381,#4149);
#2577=LINE('',#38383,#4150);
#2578=LINE('',#38385,#4151);
#2579=LINE('',#38386,#4152);
#2580=LINE('',#38390,#4153);
#2581=LINE('',#38392,#4154);
#2582=LINE('',#38394,#4155);
#2583=LINE('',#38396,#4156);
#2584=LINE('',#38398,#4157);
#2585=LINE('',#38399,#4158);
#2586=LINE('',#38402,#4159);
#2587=LINE('',#38403,#4160);
#2588=LINE('',#38406,#4161);
#2589=LINE('',#38407,#4162);
#2590=LINE('',#38409,#4163);
#2591=LINE('',#38413,#4164);
#2592=LINE('',#38415,#4165);
#2593=LINE('',#38417,#4166);
#2594=LINE('',#38419,#4167);
#2595=LINE('',#38421,#4168);
#2596=LINE('',#38422,#4169);
#2597=LINE('',#38426,#4170);
#2598=LINE('',#38428,#4171);
#2599=LINE('',#38430,#4172);
#2600=LINE('',#38432,#4173);
#2601=LINE('',#38434,#4174);
#2602=LINE('',#38435,#4175);
#2603=LINE('',#38438,#4176);
#2604=LINE('',#38440,#4177);
#2605=LINE('',#38441,#4178);
#2606=LINE('',#38444,#4179);
#2607=LINE('',#38445,#4180);
#2608=LINE('',#38448,#4181);
#2609=LINE('',#38449,#4182);
#2610=LINE('',#38452,#4183);
#2611=LINE('',#38453,#4184);
#2612=LINE('',#38456,#4185);
#2613=LINE('',#38457,#4186);
#2614=LINE('',#38459,#4187);
#2615=LINE('',#38463,#4188);
#2616=LINE('',#38466,#4189);
#2617=LINE('',#38470,#4190);
#2618=LINE('',#38475,#4191);
#2619=LINE('',#38477,#4192);
#2620=LINE('',#38480,#4193);
#2621=LINE('',#38483,#4194);
#2622=LINE('',#38485,#4195);
#2623=LINE('',#38486,#4196);
#2624=LINE('',#38489,#4197);
#2625=LINE('',#38490,#4198);
#2626=LINE('',#38493,#4199);
#2627=LINE('',#38494,#4200);
#2628=LINE('',#38497,#4201);
#2629=LINE('',#38498,#4202);
#2630=LINE('',#38501,#4203);
#2631=LINE('',#38502,#4204);
#2632=LINE('',#38504,#4205);
#2633=LINE('',#38508,#4206);
#2634=LINE('',#38512,#4207);
#2635=LINE('',#38516,#4208);
#2636=LINE('',#38520,#4209);
#2637=LINE('',#38521,#4210);
#2638=LINE('',#38524,#4211);
#2639=LINE('',#38526,#4212);
#2640=LINE('',#38527,#4213);
#2641=LINE('',#38530,#4214);
#2642=LINE('',#38531,#4215);
#2643=LINE('',#38534,#4216);
#2644=LINE('',#38535,#4217);
#2645=LINE('',#38538,#4218);
#2646=LINE('',#38539,#4219);
#2647=LINE('',#38542,#4220);
#2648=LINE('',#38543,#4221);
#2649=LINE('',#38545,#4222);
#2650=LINE('',#38549,#4223);
#2651=LINE('',#38617,#4224);
#2652=LINE('',#38619,#4225);
#2653=LINE('',#38633,#4226);
#2654=LINE('',#38634,#4227);
#2655=LINE('',#38637,#4228);
#2656=LINE('',#38709,#4229);
#2657=LINE('',#38717,#4230);
#2658=LINE('',#38718,#4231);
#2659=LINE('',#38719,#4232);
#2660=LINE('',#38722,#4233);
#2661=LINE('',#38846,#4234);
#2662=LINE('',#38848,#4235);
#2663=LINE('',#38850,#4236);
#2664=LINE('',#38853,#4237);
#2665=LINE('',#38855,#4238);
#2666=LINE('',#38860,#4239);
#2667=LINE('',#38862,#4240);
#2668=LINE('',#38865,#4241);
#2669=LINE('',#38871,#4242);
#2670=LINE('',#38872,#4243);
#2671=LINE('',#38875,#4244);
#2672=LINE('',#38878,#4245);
#2673=LINE('',#38879,#4246);
#2674=LINE('',#38882,#4247);
#2675=LINE('',#38884,#4248);
#2676=LINE('',#38885,#4249);
#2677=LINE('',#38888,#4250);
#2678=LINE('',#38889,#4251);
#2679=LINE('',#38892,#4252);
#2680=LINE('',#38893,#4253);
#2681=LINE('',#38896,#4254);
#2682=LINE('',#38897,#4255);
#2683=LINE('',#38900,#4256);
#2684=LINE('',#38901,#4257);
#2685=LINE('',#38903,#4258);
#2686=LINE('',#38980,#4259);
#2687=LINE('',#38983,#4260);
#2688=LINE('',#38986,#4261);
#2689=LINE('',#38990,#4262);
#2690=LINE('',#38992,#4263);
#2691=LINE('',#38996,#4264);
#2692=LINE('',#38998,#4265);
#2693=LINE('',#38999,#4266);
#2694=LINE('',#39002,#4267);
#2695=LINE('',#39003,#4268);
#2696=LINE('',#39006,#4269);
#2697=LINE('',#39007,#4270);
#2698=LINE('',#39010,#4271);
#2699=LINE('',#39011,#4272);
#2700=LINE('',#39014,#4273);
#2701=LINE('',#39015,#4274);
#2702=LINE('',#39017,#4275);
#2703=LINE('',#39020,#4276);
#2704=LINE('',#39022,#4277);
#2705=LINE('',#39023,#4278);
#2706=LINE('',#39026,#4279);
#2707=LINE('',#39027,#4280);
#2708=LINE('',#39030,#4281);
#2709=LINE('',#39031,#4282);
#2710=LINE('',#39034,#4283);
#2711=LINE('',#39035,#4284);
#2712=LINE('',#39038,#4285);
#2713=LINE('',#39039,#4286);
#2714=LINE('',#39041,#4287);
#2715=LINE('',#39046,#4288);
#2716=LINE('',#39048,#4289);
#2717=LINE('',#39050,#4290);
#2718=LINE('',#39052,#4291);
#2719=LINE('',#39054,#4292);
#2720=LINE('',#39055,#4293);
#2721=LINE('',#39060,#4294);
#2722=LINE('',#39062,#4295);
#2723=LINE('',#39064,#4296);
#2724=LINE('',#39066,#4297);
#2725=LINE('',#39068,#4298);
#2726=LINE('',#39069,#4299);
#2727=LINE('',#39073,#4300);
#2728=LINE('',#39074,#4301);
#2729=LINE('',#39075,#4302);
#2730=LINE('',#39078,#4303);
#2731=LINE('',#39080,#4304);
#2732=LINE('',#39082,#4305);
#2733=LINE('',#39084,#4306);
#2734=LINE('',#39085,#4307);
#2735=LINE('',#39089,#4308);
#2736=LINE('',#39090,#4309);
#2737=LINE('',#39091,#4310);
#2738=LINE('',#39094,#4311);
#2739=LINE('',#39096,#4312);
#2740=LINE('',#39097,#4313);
#2741=LINE('',#39100,#4314);
#2742=LINE('',#39101,#4315);
#2743=LINE('',#39104,#4316);
#2744=LINE('',#39105,#4317);
#2745=LINE('',#39108,#4318);
#2746=LINE('',#39109,#4319);
#2747=LINE('',#39112,#4320);
#2748=LINE('',#39113,#4321);
#2749=LINE('',#39115,#4322);
#2750=LINE('',#39121,#4323);
#2751=LINE('',#39122,#4324);
#2752=LINE('',#39124,#4325);
#2753=LINE('',#39125,#4326);
#2754=LINE('',#39128,#4327);
#2755=LINE('',#39129,#4328);
#2756=LINE('',#39132,#4329);
#2757=LINE('',#39133,#4330);
#2758=LINE('',#39136,#4331);
#2759=LINE('',#39138,#4332);
#2760=LINE('',#39141,#4333);
#2761=LINE('',#39144,#4334);
#2762=LINE('',#39145,#4335);
#2763=LINE('',#39147,#4336);
#2764=LINE('',#39150,#4337);
#2765=LINE('',#39154,#4338);
#2766=LINE('',#39233,#4339);
#2767=LINE('',#39235,#4340);
#2768=LINE('',#39239,#4341);
#2769=LINE('',#39242,#4342);
#2770=LINE('',#39319,#4343);
#2771=LINE('',#39321,#4344);
#2772=LINE('',#39322,#4345);
#2773=LINE('',#39327,#4346);
#2774=LINE('',#39328,#4347);
#2775=LINE('',#39331,#4348);
#2776=LINE('',#39332,#4349);
#2777=LINE('',#39334,#4350);
#2778=LINE('',#39337,#4351);
#2779=LINE('',#39342,#4352);
#2780=LINE('',#39346,#4353);
#2781=LINE('',#39350,#4354);
#2782=LINE('',#39352,#4355);
#2783=LINE('',#39353,#4356);
#2784=LINE('',#39356,#4357);
#2785=LINE('',#39357,#4358);
#2786=LINE('',#39360,#4359);
#2787=LINE('',#39361,#4360);
#2788=LINE('',#39364,#4361);
#2789=LINE('',#39365,#4362);
#2790=LINE('',#39368,#4363);
#2791=LINE('',#39369,#4364);
#2792=LINE('',#39371,#4365);
#2793=LINE('',#39373,#4366);
#2794=LINE('',#39375,#4367);
#2795=LINE('',#39379,#4368);
#2796=LINE('',#39380,#4369);
#2797=LINE('',#39381,#4370);
#2798=LINE('',#39384,#4371);
#2799=LINE('',#39385,#4372);
#2800=LINE('',#39388,#4373);
#2801=LINE('',#39389,#4374);
#2802=LINE('',#39391,#4375);
#2803=LINE('',#39393,#4376);
#2804=LINE('',#39396,#4377);
#2805=LINE('',#39398,#4378);
#2806=LINE('',#39399,#4379);
#2807=LINE('',#39403,#4380);
#2808=LINE('',#39408,#4381);
#2809=LINE('',#39411,#4382);
#2810=LINE('',#39414,#4383);
#2811=LINE('',#39415,#4384);
#2812=LINE('',#39420,#4385);
#2813=LINE('',#39424,#4386);
#2814=LINE('',#39425,#4387);
#2815=LINE('',#39430,#4388);
#2816=LINE('',#39433,#4389);
#2817=LINE('',#39434,#4390);
#2818=LINE('',#39436,#4391);
#2819=LINE('',#39440,#4392);
#2820=LINE('',#39445,#4393);
#2821=LINE('',#39489,#4394);
#2822=LINE('',#39490,#4395);
#2823=LINE('',#39492,#4396);
#2824=LINE('',#39494,#4397);
#2825=LINE('',#39496,#4398);
#2826=LINE('',#39497,#4399);
#2827=LINE('',#39500,#4400);
#2828=LINE('',#39501,#4401);
#2829=LINE('',#39504,#4402);
#2830=LINE('',#39506,#4403);
#2831=LINE('',#39507,#4404);
#2832=LINE('',#39510,#4405);
#2833=LINE('',#39511,#4406);
#2834=LINE('',#39514,#4407);
#2835=LINE('',#39516,#4408);
#2836=LINE('',#39517,#4409);
#2837=LINE('',#39520,#4410);
#2838=LINE('',#39521,#4411);
#2839=LINE('',#39525,#4412);
#2840=LINE('',#39527,#4413);
#2841=LINE('',#39529,#4414);
#2842=LINE('',#39531,#4415);
#2843=LINE('',#39533,#4416);
#2844=LINE('',#39534,#4417);
#2845=LINE('',#39536,#4418);
#2846=LINE('',#39538,#4419);
#2847=LINE('',#39540,#4420);
#2848=LINE('',#39541,#4421);
#2849=LINE('',#39544,#4422);
#2850=LINE('',#39545,#4423);
#2851=LINE('',#39549,#4424);
#2852=LINE('',#39550,#4425);
#2853=LINE('',#39551,#4426);
#2854=LINE('',#39554,#4427);
#2855=LINE('',#39555,#4428);
#2856=LINE('',#39559,#4429);
#2857=LINE('',#39560,#4430);
#2858=LINE('',#39561,#4431);
#2859=LINE('',#39564,#4432);
#2860=LINE('',#39565,#4433);
#2861=LINE('',#39569,#4434);
#2862=LINE('',#39570,#4435);
#2863=LINE('',#39572,#4436);
#2864=LINE('',#39574,#4437);
#2865=LINE('',#39575,#4438);
#2866=LINE('',#39579,#4439);
#2867=LINE('',#39580,#4440);
#2868=LINE('',#39581,#4441);
#2869=LINE('',#39585,#4442);
#2870=LINE('',#39586,#4443);
#2871=LINE('',#39591,#4444);
#2872=LINE('',#39592,#4445);
#2873=LINE('',#39597,#4446);
#2874=LINE('',#39598,#4447);
#2875=LINE('',#39601,#4448);
#2876=LINE('',#39602,#4449);
#2877=LINE('',#39603,#4450);
#2878=LINE('',#39605,#4451);
#2879=LINE('',#39606,#4452);
#2880=LINE('',#39607,#4453);
#2881=LINE('',#39610,#4454);
#2882=LINE('',#39611,#4455);
#2883=LINE('',#39613,#4456);
#2884=LINE('',#39615,#4457);
#2885=LINE('',#39618,#4458);
#2886=LINE('',#39619,#4459);
#2887=LINE('',#39622,#4460);
#2888=LINE('',#39623,#4461);
#2889=LINE('',#39625,#4462);
#2890=LINE('',#39627,#4463);
#2891=LINE('',#39628,#4464);
#2892=LINE('',#39630,#4465);
#2893=LINE('',#39631,#4466);
#2894=LINE('',#39660,#4467);
#2895=LINE('',#39662,#4468);
#2896=LINE('',#39663,#4469);
#2897=LINE('',#39664,#4470);
#2898=LINE('',#39667,#4471);
#2899=LINE('',#39669,#4472);
#2900=LINE('',#39670,#4473);
#2901=LINE('',#39673,#4474);
#2902=LINE('',#39674,#4475);
#2903=LINE('',#39676,#4476);
#2904=LINE('',#39678,#4477);
#2905=LINE('',#39680,#4478);
#2906=LINE('',#39681,#4479);
#2907=LINE('',#39685,#4480);
#2908=LINE('',#39686,#4481);
#2909=LINE('',#39687,#4482);
#2910=LINE('',#39690,#4483);
#2911=LINE('',#39691,#4484);
#2912=LINE('',#39694,#4485);
#2913=LINE('',#39695,#4486);
#2914=LINE('',#39698,#4487);
#2915=LINE('',#39700,#4488);
#2916=LINE('',#39701,#4489);
#2917=LINE('',#39705,#4490);
#2918=LINE('',#39706,#4491);
#2919=LINE('',#39707,#4492);
#2920=LINE('',#39710,#4493);
#2921=LINE('',#39711,#4494);
#2922=LINE('',#39714,#4495);
#2923=LINE('',#39715,#4496);
#2924=LINE('',#39717,#4497);
#2925=LINE('',#39719,#4498);
#2926=LINE('',#39721,#4499);
#2927=LINE('',#39725,#4500);
#2928=LINE('',#39726,#4501);
#2929=LINE('',#39728,#4502);
#2930=LINE('',#39729,#4503);
#2931=LINE('',#39732,#4504);
#2932=LINE('',#39733,#4505);
#2933=LINE('',#39736,#4506);
#2934=LINE('',#39738,#4507);
#2935=LINE('',#39739,#4508);
#2936=LINE('',#39742,#4509);
#2937=LINE('',#39744,#4510);
#2938=LINE('',#39745,#4511);
#2939=LINE('',#39748,#4512);
#2940=LINE('',#39749,#4513);
#2941=LINE('',#39752,#4514);
#2942=LINE('',#39753,#4515);
#2943=LINE('',#39756,#4516);
#2944=LINE('',#39757,#4517);
#2945=LINE('',#39760,#4518);
#2946=LINE('',#39761,#4519);
#2947=LINE('',#39764,#4520);
#2948=LINE('',#39765,#4521);
#2949=LINE('',#39768,#4522);
#2950=LINE('',#39769,#4523);
#2951=LINE('',#39772,#4524);
#2952=LINE('',#39773,#4525);
#2953=LINE('',#39776,#4526);
#2954=LINE('',#39777,#4527);
#2955=LINE('',#39780,#4528);
#2956=LINE('',#39781,#4529);
#2957=LINE('',#39784,#4530);
#2958=LINE('',#39785,#4531);
#2959=LINE('',#39787,#4532);
#3363=VECTOR('',#21450,55.);
#3364=VECTOR('',#21455,28.6682517601201);
#3365=VECTOR('',#21458,50.);
#3366=VECTOR('',#21463,32.793965079916);
#3367=VECTOR('',#21466,45.3097394023382);
#3368=VECTOR('',#21477,0.857142857149274);
#3369=VECTOR('',#21482,0.999999999925893);
#3370=VECTOR('',#21489,0.499999999966139);
#3371=VECTOR('',#21496,1000.);
#3372=VECTOR('',#21497,1000.);
#3373=VECTOR('',#21498,1000.);
#3374=VECTOR('',#21499,1000.);
#3375=VECTOR('',#21500,1000.);
#3376=VECTOR('',#21501,1000.);
#3377=VECTOR('',#21504,1000.);
#3378=VECTOR('',#21505,1000.);
#3379=VECTOR('',#21506,1000.);
#3380=VECTOR('',#21509,1000.);
#3381=VECTOR('',#21510,1000.);
#3382=VECTOR('',#21513,1000.);
#3383=VECTOR('',#21514,1000.);
#3384=VECTOR('',#21515,1000.);
#3385=VECTOR('',#21518,1000.);
#3386=VECTOR('',#21519,1000.);
#3387=VECTOR('',#21522,1000.);
#3388=VECTOR('',#21523,1000.);
#3389=VECTOR('',#21526,1000.);
#3390=VECTOR('',#21527,1000.);
#3391=VECTOR('',#21530,1000.);
#3392=VECTOR('',#21533,10.);
#3393=VECTOR('',#21534,10.);
#3394=VECTOR('',#21535,10.);
#3395=VECTOR('',#21550,6.75000000000001);
#3396=VECTOR('',#21557,6.75);
#3397=VECTOR('',#21564,6.75000000000001);
#3398=VECTOR('',#21571,6.75);
#3399=VECTOR('',#21580,7.00000000000001);
#3400=VECTOR('',#21611,7.);
#3401=VECTOR('',#21618,7.);
#3402=VECTOR('',#21633,7.);
#3403=VECTOR('',#21644,80.);
#3404=VECTOR('',#21651,40.);
#3405=VECTOR('',#21656,1000.);
#3406=VECTOR('',#21657,1000.);
#3407=VECTOR('',#21660,1000.);
#3408=VECTOR('',#21661,1000.);
#3409=VECTOR('',#21666,1000.);
#3410=VECTOR('',#21669,1000.);
#3411=VECTOR('',#21672,1000.);
#3412=VECTOR('',#21675,1000.);
#3413=VECTOR('',#21678,1000.);
#3414=VECTOR('',#21679,1000.);
#3415=VECTOR('',#21686,1000.);
#3416=VECTOR('',#21689,1000.);
#3417=VECTOR('',#21694,4.5);
#3418=VECTOR('',#21701,4.5);
#3419=VECTOR('',#21708,4.5);
#3420=VECTOR('',#21715,4.5);
#3421=VECTOR('',#21722,20.);
#3422=VECTOR('',#21729,1000.);
#3423=VECTOR('',#21730,1000.);
#3424=VECTOR('',#21735,1000.);
#3425=VECTOR('',#21736,1000.);
#3426=VECTOR('',#21741,1000.);
#3427=VECTOR('',#21744,1000.);
#3428=VECTOR('',#21757,76.5);
#3429=VECTOR('',#21772,7.00000000000001);
#3430=VECTOR('',#21783,1000.);
#3431=VECTOR('',#21786,1000.);
#3432=VECTOR('',#21791,1000.);
#3433=VECTOR('',#21794,1000.);
#3434=VECTOR('',#21795,1000.);
#3435=VECTOR('',#21798,1000.);
#3436=VECTOR('',#21801,6.99999999990287);
#3437=VECTOR('',#21808,4.);
#3438=VECTOR('',#21815,4.);
#3439=VECTOR('',#21822,4.);
#3440=VECTOR('',#21829,4.);
#3441=VECTOR('',#21836,17.4625);
#3442=VECTOR('',#21839,1000.);
#3443=VECTOR('',#21842,17.4625);
#3444=VECTOR('',#21847,1000.);
#3445=VECTOR('',#21854,7.99999999999999);
#3446=VECTOR('',#21861,8.00000000000001);
#3447=VECTOR('',#21866,17.4625);
#3448=VECTOR('',#21873,7.00000000000001);
#3449=VECTOR('',#21880,7.00000000000001);
#3450=VECTOR('',#21887,3.);
#3451=VECTOR('',#21894,3.00000000000307);
#3452=VECTOR('',#21901,3.0000000000021);
#3453=VECTOR('',#21908,2.99999999999927);
#3454=VECTOR('',#21915,1000.);
#3455=VECTOR('',#21918,1000.);
#3456=VECTOR('',#21921,6.7500000000354);
#3457=VECTOR('',#21930,1000.);
#3458=VECTOR('',#21933,1000.);
#3459=VECTOR('',#21940,6.75000000001091);
#3460=VECTOR('',#21947,5.5);
#3461=VECTOR('',#21954,1000.);
#3462=VECTOR('',#21957,1000.);
#3463=VECTOR('',#21966,8.80000000000425);
#3464=VECTOR('',#21973,8.80000000000425);
#3465=VECTOR('',#21978,6.34999999994079);
#3466=VECTOR('',#21985,5.5);
#3467=VECTOR('',#21994,1000.);
#3468=VECTOR('',#21997,1000.);
#3469=VECTOR('',#22000,5.4999999998131);
#3470=VECTOR('',#22005,10.);
#3471=VECTOR('',#22006,10.);
#3472=VECTOR('',#22007,10.);
#3473=VECTOR('',#22008,10.);
#3474=VECTOR('',#22011,10.);
#3475=VECTOR('',#22012,10.);
#3476=VECTOR('',#22015,10.);
#3477=VECTOR('',#22016,10.);
#3478=VECTOR('',#22023,1000.);
#3479=VECTOR('',#22024,1000.);
#3480=VECTOR('',#22025,1000.);
#3481=VECTOR('',#22026,1000.);
#3482=VECTOR('',#22027,1000.);
#3483=VECTOR('',#22028,1000.);
#3484=VECTOR('',#22031,1000.);
#3485=VECTOR('',#22032,1000.);
#3486=VECTOR('',#22033,1000.);
#3487=VECTOR('',#22034,1000.);
#3488=VECTOR('',#22035,1000.);
#3489=VECTOR('',#22036,1000.);
#3490=VECTOR('',#22039,1000.);
#3491=VECTOR('',#22040,1000.);
#3492=VECTOR('',#22041,1000.);
#3493=VECTOR('',#22042,1000.);
#3494=VECTOR('',#22043,1000.);
#3495=VECTOR('',#22044,1000.);
#3496=VECTOR('',#22047,1000.);
#3497=VECTOR('',#22048,1000.);
#3498=VECTOR('',#22049,1000.);
#3499=VECTOR('',#22050,1000.);
#3500=VECTOR('',#22051,1000.);
#3501=VECTOR('',#22052,1000.);
#3502=VECTOR('',#22057,1000.);
#3503=VECTOR('',#22064,1000.);
#3504=VECTOR('',#22069,1000.);
#3505=VECTOR('',#22076,1000.);
#3506=VECTOR('',#22083,1000.);
#3507=VECTOR('',#22084,1000.);
#3508=VECTOR('',#22085,1000.);
#3509=VECTOR('',#22086,1000.);
#3510=VECTOR('',#22087,1000.);
#3511=VECTOR('',#22088,1000.);
#3512=VECTOR('',#22091,1000.);
#3513=VECTOR('',#22092,1000.);
#3514=VECTOR('',#22093,1000.);
#3515=VECTOR('',#22094,1000.);
#3516=VECTOR('',#22095,1000.);
#3517=VECTOR('',#22096,1000.);
#3518=VECTOR('',#22099,1000.);
#3519=VECTOR('',#22100,1000.);
#3520=VECTOR('',#22101,1000.);
#3521=VECTOR('',#22104,1000.);
#3522=VECTOR('',#22105,1000.);
#3523=VECTOR('',#22108,1000.);
#3524=VECTOR('',#22109,1000.);
#3525=VECTOR('',#22112,1000.);
#3526=VECTOR('',#22113,1000.);
#3527=VECTOR('',#22116,1000.);
#3528=VECTOR('',#22117,1000.);
#3529=VECTOR('',#22120,1000.);
#3530=VECTOR('',#22123,1000.);
#3531=VECTOR('',#22124,1000.);
#3532=VECTOR('',#22125,1000.);
#3533=VECTOR('',#22126,1000.);
#3534=VECTOR('',#22131,1000.);
#3535=VECTOR('',#22138,1000.);
#3536=VECTOR('',#22139,1000.);
#3537=VECTOR('',#22140,1000.);
#3538=VECTOR('',#22145,1000.);
#3539=VECTOR('',#22146,1000.);
#3540=VECTOR('',#22147,1000.);
#3541=VECTOR('',#22150,1000.);
#3542=VECTOR('',#22151,1000.);
#3543=VECTOR('',#22154,1000.);
#3544=VECTOR('',#22155,1000.);
#3545=VECTOR('',#22158,1000.);
#3546=VECTOR('',#22159,1000.);
#3547=VECTOR('',#22162,1000.);
#3548=VECTOR('',#22163,1000.);
#3549=VECTOR('',#22166,1000.);
#3550=VECTOR('',#22169,1000.);
#3551=VECTOR('',#22170,1000.);
#3552=VECTOR('',#22171,1000.);
#3553=VECTOR('',#22172,1000.);
#3554=VECTOR('',#22177,1000.);
#3555=VECTOR('',#22184,1000.);
#3556=VECTOR('',#22185,1000.);
#3557=VECTOR('',#22186,1000.);
#3558=VECTOR('',#22191,1000.);
#3559=VECTOR('',#22192,1000.);
#3560=VECTOR('',#22193,1000.);
#3561=VECTOR('',#22196,1000.);
#3562=VECTOR('',#22197,1000.);
#3563=VECTOR('',#22200,1000.);
#3564=VECTOR('',#22201,1000.);
#3565=VECTOR('',#22204,1000.);
#3566=VECTOR('',#22205,1000.);
#3567=VECTOR('',#22208,1000.);
#3568=VECTOR('',#22209,1000.);
#3569=VECTOR('',#22212,1000.);
#3570=VECTOR('',#22215,1000.);
#3571=VECTOR('',#22216,1000.);
#3572=VECTOR('',#22217,1000.);
#3573=VECTOR('',#22218,1000.);
#3574=VECTOR('',#22223,1000.);
#3575=VECTOR('',#22230,1000.);
#3576=VECTOR('',#22231,1000.);
#3577=VECTOR('',#22232,1000.);
#3578=VECTOR('',#22237,1000.);
#3579=VECTOR('',#22238,1000.);
#3580=VECTOR('',#22239,1000.);
#3581=VECTOR('',#22242,1000.);
#3582=VECTOR('',#22243,1000.);
#3583=VECTOR('',#22244,1000.);
#3584=VECTOR('',#22247,1000.);
#3585=VECTOR('',#22248,1000.);
#3586=VECTOR('',#22249,1000.);
#3587=VECTOR('',#22252,1000.);
#3588=VECTOR('',#22253,1000.);
#3589=VECTOR('',#22256,1000.);
#3590=VECTOR('',#22257,1000.);
#3591=VECTOR('',#22260,1000.);
#3592=VECTOR('',#22261,1000.);
#3593=VECTOR('',#22264,1000.);
#3594=VECTOR('',#22265,1000.);
#3595=VECTOR('',#22268,1000.);
#3596=VECTOR('',#22271,1000.);
#3597=VECTOR('',#22272,1000.);
#3598=VECTOR('',#22273,1000.);
#3599=VECTOR('',#22278,1000.);
#3600=VECTOR('',#22283,1000.);
#3601=VECTOR('',#22284,1000.);
#3602=VECTOR('',#22289,1000.);
#3603=VECTOR('',#22290,1000.);
#3604=VECTOR('',#22295,1000.);
#3605=VECTOR('',#22296,1000.);
#3606=VECTOR('',#22299,1000.);
#3607=VECTOR('',#22304,1000.);
#3608=VECTOR('',#22309,1000.);
#3609=VECTOR('',#22314,1000.);
#3610=VECTOR('',#22315,1000.);
#3611=VECTOR('',#22318,1000.);
#3612=VECTOR('',#22323,1000.);
#3613=VECTOR('',#22328,1000.);
#3614=VECTOR('',#22333,1000.);
#3615=VECTOR('',#22334,1000.);
#3616=VECTOR('',#22341,1000.);
#3617=VECTOR('',#22346,1000.);
#3618=VECTOR('',#22347,1000.);
#3619=VECTOR('',#22350,1000.);
#3620=VECTOR('',#22359,1000.);
#3621=VECTOR('',#22360,1000.);
#3622=VECTOR('',#22365,1000.);
#3623=VECTOR('',#22370,1000.);
#3624=VECTOR('',#22375,1000.);
#3625=VECTOR('',#22380,1000.);
#3626=VECTOR('',#22389,1000.);
#3627=VECTOR('',#22390,1000.);
#3628=VECTOR('',#22395,1000.);
#3629=VECTOR('',#22400,1000.);
#3630=VECTOR('',#22405,1000.);
#3631=VECTOR('',#22410,1000.);
#3632=VECTOR('',#22419,1000.);
#3633=VECTOR('',#22422,1000.);
#3634=VECTOR('',#22427,1000.);
#3635=VECTOR('',#22428,1000.);
#3636=VECTOR('',#22431,1000.);
#3637=VECTOR('',#22434,1000.);
#3638=VECTOR('',#22437,1000.);
#3639=VECTOR('',#22440,1000.);
#3640=VECTOR('',#22443,1000.);
#3641=VECTOR('',#22446,1000.);
#3642=VECTOR('',#22449,1000.);
#3643=VECTOR('',#22452,1000.);
#3644=VECTOR('',#22455,1000.);
#3645=VECTOR('',#22456,1000.);
#3646=VECTOR('',#22461,1000.);
#3647=VECTOR('',#22464,1000.);
#3648=VECTOR('',#22467,1000.);
#3649=VECTOR('',#22468,1000.);
#3650=VECTOR('',#22473,1000.);
#3651=VECTOR('',#22476,1000.);
#3652=VECTOR('',#22479,1000.);
#3653=VECTOR('',#22480,1000.);
#3654=VECTOR('',#22485,1000.);
#3655=VECTOR('',#22488,1000.);
#3656=VECTOR('',#22491,1000.);
#3657=VECTOR('',#22492,1000.);
#3658=VECTOR('',#22497,1000.);
#3659=VECTOR('',#22500,1000.);
#3660=VECTOR('',#22527,1000.);
#3661=VECTOR('',#22528,1000.);
#3662=VECTOR('',#22531,1000.);
#3663=VECTOR('',#22532,1000.);
#3664=VECTOR('',#22537,1000.);
#3665=VECTOR('',#22540,1000.);
#3666=VECTOR('',#22541,1000.);
#3667=VECTOR('',#22546,1000.);
#3668=VECTOR('',#22549,1000.);
#3669=VECTOR('',#22550,1000.);
#3670=VECTOR('',#22555,1000.);
#3671=VECTOR('',#22558,1000.);
#3672=VECTOR('',#22559,10.);
#3673=VECTOR('',#22560,10.);
#3674=VECTOR('',#22561,10.);
#3675=VECTOR('',#22562,10.);
#3676=VECTOR('',#22567,10.);
#3677=VECTOR('',#22568,10.);
#3678=VECTOR('',#22573,10.);
#3679=VECTOR('',#22574,10.);
#3680=VECTOR('',#22579,10.);
#3681=VECTOR('',#22580,10.);
#3682=VECTOR('',#22591,10.);
#3683=VECTOR('',#22594,10.);
#3684=VECTOR('',#22595,10.);
#3685=VECTOR('',#22598,10.);
#3686=VECTOR('',#22599,10.);
#3687=VECTOR('',#22606,1000.);
#3688=VECTOR('',#22607,1000.);
#3689=VECTOR('',#22612,1000.);
#3690=VECTOR('',#22613,1000.);
#3691=VECTOR('',#22618,1000.);
#3692=VECTOR('',#22619,1000.);
#3693=VECTOR('',#22624,10.);
#3694=VECTOR('',#22625,10.);
#3695=VECTOR('',#22638,10.);
#3696=VECTOR('',#22639,10.);
#3697=VECTOR('',#22644,10.);
#3698=VECTOR('',#22645,10.);
#3699=VECTOR('',#22650,10.);
#3700=VECTOR('',#22651,10.);
#3701=VECTOR('',#22654,1000.);
#3702=VECTOR('',#22657,1000.);
#3703=VECTOR('',#22660,1000.);
#3704=VECTOR('',#22663,1000.);
#3705=VECTOR('',#22670,1000.);
#3706=VECTOR('',#22671,1000.);
#3707=VECTOR('',#22676,1000.);
#3708=VECTOR('',#22681,1000.);
#3709=VECTOR('',#22684,1000.);
#3710=VECTOR('',#22691,1000.);
#3711=VECTOR('',#22696,1000.);
#3712=VECTOR('',#22705,1000.);
#3713=VECTOR('',#22710,1000.);
#3714=VECTOR('',#22717,1000.);
#3715=VECTOR('',#22724,1000.);
#3716=VECTOR('',#22729,1000.);
#3717=VECTOR('',#22734,1000.);
#3718=VECTOR('',#22741,1000.);
#3719=VECTOR('',#22742,1000.);
#3720=VECTOR('',#22743,1000.);
#3721=VECTOR('',#22746,1000.);
#3722=VECTOR('',#22747,1000.);
#3723=VECTOR('',#22748,1000.);
#3724=VECTOR('',#22755,1000.);
#3725=VECTOR('',#22756,1000.);
#3726=VECTOR('',#22757,1000.);
#3727=VECTOR('',#22766,1000.);
#3728=VECTOR('',#22769,1000.);
#3729=VECTOR('',#22774,1000.);
#3730=VECTOR('',#22775,1000.);
#3731=VECTOR('',#22780,1000.);
#3732=VECTOR('',#22783,1000.);
#3733=VECTOR('',#22786,1000.);
#3734=VECTOR('',#22791,1000.);
#3735=VECTOR('',#22794,1000.);
#3736=VECTOR('',#22803,1000.);
#3737=VECTOR('',#22808,1000.);
#3738=VECTOR('',#22837,1000.);
#3739=VECTOR('',#22838,1000.);
#3740=VECTOR('',#22839,1000.);
#3741=VECTOR('',#22840,1000.);
#3742=VECTOR('',#22841,1000.);
#3743=VECTOR('',#22842,1000.);
#3744=VECTOR('',#22845,1000.);
#3745=VECTOR('',#22846,1000.);
#3746=VECTOR('',#22847,1000.);
#3747=VECTOR('',#22848,1000.);
#3748=VECTOR('',#22849,1000.);
#3749=VECTOR('',#22850,1000.);
#3750=VECTOR('',#22853,1000.);
#3751=VECTOR('',#22856,1000.);
#3752=VECTOR('',#22859,1000.);
#3753=VECTOR('',#22862,1000.);
#3754=VECTOR('',#22867,1000.);
#3755=VECTOR('',#22870,1000.);
#3756=VECTOR('',#22871,1000.);
#3757=VECTOR('',#22874,1000.);
#3758=VECTOR('',#22875,1000.);
#3759=VECTOR('',#22878,1000.);
#3760=VECTOR('',#22883,1000.);
#3761=VECTOR('',#22886,1000.);
#3762=VECTOR('',#22895,1000.);
#3763=VECTOR('',#22896,1000.);
#3764=VECTOR('',#22899,1000.);
#3765=VECTOR('',#22900,1000.);
#3766=VECTOR('',#22903,1000.);
#3767=VECTOR('',#22914,1000.);
#3768=VECTOR('',#22915,1000.);
#3769=VECTOR('',#22918,1000.);
#3770=VECTOR('',#22919,1000.);
#3771=VECTOR('',#22922,1000.);
#3772=VECTOR('',#22927,1000.);
#3773=VECTOR('',#22930,1000.);
#3774=VECTOR('',#22939,1000.);
#3775=VECTOR('',#22940,1000.);
#3776=VECTOR('',#22943,1000.);
#3777=VECTOR('',#22944,1000.);
#3778=VECTOR('',#22947,1000.);
#3779=VECTOR('',#22952,1000.);
#3780=VECTOR('',#22959,1000.);
#3781=VECTOR('',#22960,1000.);
#3782=VECTOR('',#22961,1000.);
#3783=VECTOR('',#22964,1000.);
#3784=VECTOR('',#22965,1000.);
#3785=VECTOR('',#22968,1000.);
#3786=VECTOR('',#22969,1000.);
#3787=VECTOR('',#22972,1000.);
#3788=VECTOR('',#22973,1000.);
#3789=VECTOR('',#22976,1000.);
#3790=VECTOR('',#22977,1000.);
#3791=VECTOR('',#22980,1000.);
#3792=VECTOR('',#22983,1000.);
#3793=VECTOR('',#22984,1000.);
#3794=VECTOR('',#22985,1000.);
#3795=VECTOR('',#22988,1000.);
#3796=VECTOR('',#22989,1000.);
#3797=VECTOR('',#22992,1000.);
#3798=VECTOR('',#22993,1000.);
#3799=VECTOR('',#22996,1000.);
#3800=VECTOR('',#22997,1000.);
#3801=VECTOR('',#23000,1000.);
#3802=VECTOR('',#23001,1000.);
#3803=VECTOR('',#23004,1000.);
#3804=VECTOR('',#23009,1000.);
#3805=VECTOR('',#23012,1000.);
#3806=VECTOR('',#23017,1000.);
#3807=VECTOR('',#23020,1000.);
#3808=VECTOR('',#23023,1000.);
#3809=VECTOR('',#23024,1000.);
#3810=VECTOR('',#23025,1000.);
#3811=VECTOR('',#23026,1000.);
#3812=VECTOR('',#23029,1000.);
#3813=VECTOR('',#23032,1000.);
#3814=VECTOR('',#23033,1000.);
#3815=VECTOR('',#23034,1000.);
#3816=VECTOR('',#23037,1000.);
#3817=VECTOR('',#23038,1000.);
#3818=VECTOR('',#23045,1000.);
#3819=VECTOR('',#23048,1000.);
#3820=VECTOR('',#23053,1000.);
#3821=VECTOR('',#23056,1000.);
#3822=VECTOR('',#23061,1000.);
#3823=VECTOR('',#23064,1000.);
#3824=VECTOR('',#23067,1000.);
#3825=VECTOR('',#23068,1000.);
#3826=VECTOR('',#23069,1000.);
#3827=VECTOR('',#23070,1000.);
#3828=VECTOR('',#23071,1000.);
#3829=VECTOR('',#23072,1000.);
#3830=VECTOR('',#23075,1000.);
#3831=VECTOR('',#23076,1000.);
#3832=VECTOR('',#23081,1000.);
#3833=VECTOR('',#23082,1000.);
#3834=VECTOR('',#23089,1000.);
#3835=VECTOR('',#23090,1000.);
#3836=VECTOR('',#23091,1000.);
#3837=VECTOR('',#23094,1000.);
#3838=VECTOR('',#23095,1000.);
#3839=VECTOR('',#23096,1000.);
#3840=VECTOR('',#23099,1000.);
#3841=VECTOR('',#23102,1000.);
#3842=VECTOR('',#23103,1000.);
#3843=VECTOR('',#23104,1000.);
#3844=VECTOR('',#23107,1000.);
#3845=VECTOR('',#23110,1000.);
#3846=VECTOR('',#23113,1000.);
#3847=VECTOR('',#23118,1000.);
#3848=VECTOR('',#23119,1000.);
#3849=VECTOR('',#23120,1000.);
#3850=VECTOR('',#23121,1000.);
#3851=VECTOR('',#23124,1000.);
#3852=VECTOR('',#23125,1000.);
#3853=VECTOR('',#23128,1000.);
#3854=VECTOR('',#23131,1000.);
#3855=VECTOR('',#23132,1000.);
#3856=VECTOR('',#23135,1000.);
#3857=VECTOR('',#23136,1000.);
#3858=VECTOR('',#23139,1000.);
#3859=VECTOR('',#23140,1000.);
#3860=VECTOR('',#23141,1000.);
#3861=VECTOR('',#23142,1000.);
#3862=VECTOR('',#23145,1000.);
#3863=VECTOR('',#23146,1000.);
#3864=VECTOR('',#23147,1000.);
#3865=VECTOR('',#23150,1000.);
#3866=VECTOR('',#23151,1000.);
#3867=VECTOR('',#23152,1000.);
#3868=VECTOR('',#23155,1000.);
#3869=VECTOR('',#23158,1000.);
#3870=VECTOR('',#23161,1000.);
#3871=VECTOR('',#23164,1000.);
#3872=VECTOR('',#23169,1000.);
#3873=VECTOR('',#23170,1000.);
#3874=VECTOR('',#23171,1000.);
#3875=VECTOR('',#23174,1000.);
#3876=VECTOR('',#23175,1000.);
#3877=VECTOR('',#23178,1000.);
#3878=VECTOR('',#23179,1000.);
#3879=VECTOR('',#23180,1000.);
#3880=VECTOR('',#23183,1000.);
#3881=VECTOR('',#23186,1000.);
#3882=VECTOR('',#23187,1000.);
#3883=VECTOR('',#23188,1000.);
#3884=VECTOR('',#23191,1000.);
#3885=VECTOR('',#23194,1000.);
#3886=VECTOR('',#23197,1000.);
#3887=VECTOR('',#23202,1000.);
#3888=VECTOR('',#23203,1000.);
#3889=VECTOR('',#23204,1000.);
#3890=VECTOR('',#23207,1000.);
#3891=VECTOR('',#23208,1000.);
#3892=VECTOR('',#23211,1000.);
#3893=VECTOR('',#23214,1000.);
#3894=VECTOR('',#23219,1000.);
#3895=VECTOR('',#23220,1000.);
#3896=VECTOR('',#23221,1000.);
#3897=VECTOR('',#23224,1000.);
#3898=VECTOR('',#23225,1000.);
#3899=VECTOR('',#23228,1000.);
#3900=VECTOR('',#23231,1000.);
#3901=VECTOR('',#23232,1000.);
#3902=VECTOR('',#23233,1000.);
#3903=VECTOR('',#23236,1000.);
#3904=VECTOR('',#23239,1000.);
#3905=VECTOR('',#23240,1000.);
#3906=VECTOR('',#23241,1000.);
#3907=VECTOR('',#23242,1000.);
#3908=VECTOR('',#23243,1000.);
#3909=VECTOR('',#23244,1000.);
#3910=VECTOR('',#23247,1000.);
#3911=VECTOR('',#23248,1000.);
#3912=VECTOR('',#23249,1000.);
#3913=VECTOR('',#23250,1000.);
#3914=VECTOR('',#23255,1000.);
#3915=VECTOR('',#23256,1000.);
#3916=VECTOR('',#23257,1000.);
#3917=VECTOR('',#23258,1000.);
#3918=VECTOR('',#23263,1000.);
#3919=VECTOR('',#23266,1000.);
#3920=VECTOR('',#23269,1000.);
#3921=VECTOR('',#23270,1000.);
#3922=VECTOR('',#23271,1000.);
#3923=VECTOR('',#23274,1000.);
#3924=VECTOR('',#23279,1000.);
#3925=VECTOR('',#23280,1000.);
#3926=VECTOR('',#23283,1000.);
#3927=VECTOR('',#23284,1000.);
#3928=VECTOR('',#23287,1000.);
#3929=VECTOR('',#23288,1000.);
#3930=VECTOR('',#23291,1000.);
#3931=VECTOR('',#23296,1000.);
#3932=VECTOR('',#23297,1000.);
#3933=VECTOR('',#23298,1000.);
#3934=VECTOR('',#23301,1000.);
#3935=VECTOR('',#23302,1000.);
#3936=VECTOR('',#23303,1000.);
#3937=VECTOR('',#23308,1000.);
#3938=VECTOR('',#23311,1000.);
#3939=VECTOR('',#23314,1000.);
#3940=VECTOR('',#23315,1000.);
#3941=VECTOR('',#23316,1000.);
#3942=VECTOR('',#23319,1000.);
#3943=VECTOR('',#23324,1000.);
#3944=VECTOR('',#23325,1000.);
#3945=VECTOR('',#23328,1000.);
#3946=VECTOR('',#23329,1000.);
#3947=VECTOR('',#23332,1000.);
#3948=VECTOR('',#23333,1000.);
#3949=VECTOR('',#23336,1000.);
#3950=VECTOR('',#23341,1000.);
#3951=VECTOR('',#23342,1000.);
#3952=VECTOR('',#23343,1000.);
#3953=VECTOR('',#23346,1000.);
#3954=VECTOR('',#23347,1000.);
#3955=VECTOR('',#23348,1000.);
#3956=VECTOR('',#23353,1000.);
#3957=VECTOR('',#23356,1000.);
#3958=VECTOR('',#23359,1000.);
#3959=VECTOR('',#23360,1000.);
#3960=VECTOR('',#23361,1000.);
#3961=VECTOR('',#23364,1000.);
#3962=VECTOR('',#23369,1000.);
#3963=VECTOR('',#23370,1000.);
#3964=VECTOR('',#23373,1000.);
#3965=VECTOR('',#23374,1000.);
#3966=VECTOR('',#23377,1000.);
#3967=VECTOR('',#23378,1000.);
#3968=VECTOR('',#23381,1000.);
#3969=VECTOR('',#23386,1000.);
#3970=VECTOR('',#23387,1000.);
#3971=VECTOR('',#23388,1000.);
#3972=VECTOR('',#23391,1000.);
#3973=VECTOR('',#23392,1000.);
#3974=VECTOR('',#23393,1000.);
#3975=VECTOR('',#23398,1000.);
#3976=VECTOR('',#23401,1000.);
#3977=VECTOR('',#23404,1000.);
#3978=VECTOR('',#23405,1000.);
#3979=VECTOR('',#23406,1000.);
#3980=VECTOR('',#23409,1000.);
#3981=VECTOR('',#23414,1000.);
#3982=VECTOR('',#23415,1000.);
#3983=VECTOR('',#23418,1000.);
#3984=VECTOR('',#23419,1000.);
#3985=VECTOR('',#23422,1000.);
#3986=VECTOR('',#23423,1000.);
#3987=VECTOR('',#23426,1000.);
#3988=VECTOR('',#23431,1000.);
#3989=VECTOR('',#23432,1000.);
#3990=VECTOR('',#23435,1000.);
#3991=VECTOR('',#23436,1000.);
#3992=VECTOR('',#23437,1000.);
#3993=VECTOR('',#23440,1000.);
#3994=VECTOR('',#23441,1000.);
#3995=VECTOR('',#23444,1000.);
#3996=VECTOR('',#23445,1000.);
#3997=VECTOR('',#23448,1000.);
#3998=VECTOR('',#23449,1000.);
#3999=VECTOR('',#23452,1000.);
#4000=VECTOR('',#23453,1000.);
#4001=VECTOR('',#23456,1000.);
#4002=VECTOR('',#23463,1000.);
#4003=VECTOR('',#23464,1000.);
#4004=VECTOR('',#23467,1000.);
#4005=VECTOR('',#23470,1000.);
#4006=VECTOR('',#23483,1000.);
#4007=VECTOR('',#23484,1000.);
#4008=VECTOR('',#23485,1000.);
#4009=VECTOR('',#23488,1000.);
#4010=VECTOR('',#23491,1000.);
#4011=VECTOR('',#23494,1000.);
#4012=VECTOR('',#23499,1000.);
#4013=VECTOR('',#23500,1000.);
#4014=VECTOR('',#23503,1000.);
#4015=VECTOR('',#23508,1000.);
#4016=VECTOR('',#23509,1000.);
#4017=VECTOR('',#23512,1000.);
#4018=VECTOR('',#23515,1000.);
#4019=VECTOR('',#23518,1000.);
#4020=VECTOR('',#23521,1000.);
#4021=VECTOR('',#23524,1000.);
#4022=VECTOR('',#23527,1000.);
#4023=VECTOR('',#23530,1000.);
#4024=VECTOR('',#23533,1000.);
#4025=VECTOR('',#23536,1000.);
#4026=VECTOR('',#23539,1000.);
#4027=VECTOR('',#23540,1000.);
#4028=VECTOR('',#23543,1000.);
#4029=VECTOR('',#23548,1000.);
#4030=VECTOR('',#23549,1000.);
#4031=VECTOR('',#23552,1000.);
#4032=VECTOR('',#23555,1000.);
#4033=VECTOR('',#23558,1000.);
#4034=VECTOR('',#23563,1000.);
#4035=VECTOR('',#23564,1000.);
#4036=VECTOR('',#23573,1000.);
#4037=VECTOR('',#23574,1000.);
#4038=VECTOR('',#23575,1000.);
#4039=VECTOR('',#23576,1000.);
#4040=VECTOR('',#23577,1000.);
#4041=VECTOR('',#23578,1000.);
#4042=VECTOR('',#23581,1000.);
#4043=VECTOR('',#23582,1000.);
#4044=VECTOR('',#23585,1000.);
#4045=VECTOR('',#23588,1000.);
#4046=VECTOR('',#23591,1000.);
#4047=VECTOR('',#23594,1000.);
#4048=VECTOR('',#23597,1000.);
#4049=VECTOR('',#23602,1000.);
#4050=VECTOR('',#23605,1000.);
#4051=VECTOR('',#23608,1000.);
#4052=VECTOR('',#23611,1000.);
#4053=VECTOR('',#23614,1000.);
#4054=VECTOR('',#23617,1000.);
#4055=VECTOR('',#23620,1000.);
#4056=VECTOR('',#23625,1000.);
#4057=VECTOR('',#23626,1000.);
#4058=VECTOR('',#23627,1000.);
#4059=VECTOR('',#23628,1000.);
#4060=VECTOR('',#23629,1000.);
#4061=VECTOR('',#23630,1000.);
#4062=VECTOR('',#23631,1000.);
#4063=VECTOR('',#23632,1000.);
#4064=VECTOR('',#23643,1000.);
#4065=VECTOR('',#23648,1000.);
#4066=VECTOR('',#23649,1000.);
#4067=VECTOR('',#23650,1000.);
#4068=VECTOR('',#23651,1000.);
#4069=VECTOR('',#23652,1000.);
#4070=VECTOR('',#23653,1000.);
#4071=VECTOR('',#23654,1000.);
#4072=VECTOR('',#23657,1000.);
#4073=VECTOR('',#23658,1000.);
#4074=VECTOR('',#23659,1000.);
#4075=VECTOR('',#23660,1000.);
#4076=VECTOR('',#23661,1000.);
#4077=VECTOR('',#23662,1000.);
#4078=VECTOR('',#23667,1000.);
#4079=VECTOR('',#23668,1000.);
#4080=VECTOR('',#23669,1000.);
#4081=VECTOR('',#23672,1000.);
#4082=VECTOR('',#23673,1000.);
#4083=VECTOR('',#23676,1000.);
#4084=VECTOR('',#23677,1000.);
#4085=VECTOR('',#23680,1000.);
#4086=VECTOR('',#23681,1000.);
#4087=VECTOR('',#23684,1000.);
#4088=VECTOR('',#23685,1000.);
#4089=VECTOR('',#23688,1000.);
#4090=VECTOR('',#23691,1000.);
#4091=VECTOR('',#23694,1000.);
#4092=VECTOR('',#23719,1000.);
#4093=VECTOR('',#23720,1000.);
#4094=VECTOR('',#23723,1000.);
#4095=VECTOR('',#23724,1000.);
#4096=VECTOR('',#23725,1000.);
#4097=VECTOR('',#23726,1000.);
#4098=VECTOR('',#23727,1000.);
#4099=VECTOR('',#23728,1000.);
#4100=VECTOR('',#23731,1000.);
#4101=VECTOR('',#23732,1000.);
#4102=VECTOR('',#23733,1000.);
#4103=VECTOR('',#23734,1000.);
#4104=VECTOR('',#23735,1000.);
#4105=VECTOR('',#23736,1000.);
#4106=VECTOR('',#23739,1000.);
#4107=VECTOR('',#23740,1000.);
#4108=VECTOR('',#23741,1000.);
#4109=VECTOR('',#23742,1000.);
#4110=VECTOR('',#23743,1000.);
#4111=VECTOR('',#23744,1000.);
#4112=VECTOR('',#23749,1000.);
#4113=VECTOR('',#23752,1000.);
#4114=VECTOR('',#23753,1000.);
#4115=VECTOR('',#23762,1000.);
#4116=VECTOR('',#23765,1000.);
#4117=VECTOR('',#23766,1000.);
#4118=VECTOR('',#23781,1000.);
#4119=VECTOR('',#23784,1000.);
#4120=VECTOR('',#23785,1000.);
#4121=VECTOR('',#23794,1000.);
#4122=VECTOR('',#23797,1000.);
#4123=VECTOR('',#23798,1000.);
#4124=VECTOR('',#23805,1000.);
#4125=VECTOR('',#23806,1000.);
#4126=VECTOR('',#23807,1000.);
#4127=VECTOR('',#23810,1000.);
#4128=VECTOR('',#23811,1000.);
#4129=VECTOR('',#23814,1000.);
#4130=VECTOR('',#23815,1000.);
#4131=VECTOR('',#23818,1000.);
#4132=VECTOR('',#23819,1000.);
#4133=VECTOR('',#23822,1000.);
#4134=VECTOR('',#23823,1000.);
#4135=VECTOR('',#23826,1000.);
#4136=VECTOR('',#23831,1000.);
#4137=VECTOR('',#23832,1000.);
#4138=VECTOR('',#23839,1000.);
#4139=VECTOR('',#23842,1000.);
#4140=VECTOR('',#23845,1000.);
#4141=VECTOR('',#23854,1000.);
#4142=VECTOR('',#23855,1000.);
#4143=VECTOR('',#23856,1000.);
#4144=VECTOR('',#23857,1000.);
#4145=VECTOR('',#23858,1000.);
#4146=VECTOR('',#23859,1000.);
#4147=VECTOR('',#23862,1000.);
#4148=VECTOR('',#23863,1000.);
#4149=VECTOR('',#23864,1000.);
#4150=VECTOR('',#23865,1000.);
#4151=VECTOR('',#23866,1000.);
#4152=VECTOR('',#23867,1000.);
#4153=VECTOR('',#23870,1000.);
#4154=VECTOR('',#23871,1000.);
#4155=VECTOR('',#23872,1000.);
#4156=VECTOR('',#23873,1000.);
#4157=VECTOR('',#23874,1000.);
#4158=VECTOR('',#23875,1000.);
#4159=VECTOR('',#23878,1000.);
#4160=VECTOR('',#23879,1000.);
#4161=VECTOR('',#23882,1000.);
#4162=VECTOR('',#23883,1000.);
#4163=VECTOR('',#23886,1000.);
#4164=VECTOR('',#23889,1000.);
#4165=VECTOR('',#23890,1000.);
#4166=VECTOR('',#23891,1000.);
#4167=VECTOR('',#23892,1000.);
#4168=VECTOR('',#23893,1000.);
#4169=VECTOR('',#23894,1000.);
#4170=VECTOR('',#23897,1000.);
#4171=VECTOR('',#23898,1000.);
#4172=VECTOR('',#23899,1000.);
#4173=VECTOR('',#23900,1000.);
#4174=VECTOR('',#23901,1000.);
#4175=VECTOR('',#23902,1000.);
#4176=VECTOR('',#23905,1000.);
#4177=VECTOR('',#23906,1000.);
#4178=VECTOR('',#23907,1000.);
#4179=VECTOR('',#23910,1000.);
#4180=VECTOR('',#23911,1000.);
#4181=VECTOR('',#23914,1000.);
#4182=VECTOR('',#23915,1000.);
#4183=VECTOR('',#23918,1000.);
#4184=VECTOR('',#23919,1000.);
#4185=VECTOR('',#23922,1000.);
#4186=VECTOR('',#23923,1000.);
#4187=VECTOR('',#23926,1000.);
#4188=VECTOR('',#23929,1000.);
#4189=VECTOR('',#23932,1000.);
#4190=VECTOR('',#23935,1000.);
#4191=VECTOR('',#23942,1000.);
#4192=VECTOR('',#23943,1000.);
#4193=VECTOR('',#23946,1000.);
#4194=VECTOR('',#23949,1000.);
#4195=VECTOR('',#23950,1000.);
#4196=VECTOR('',#23951,1000.);
#4197=VECTOR('',#23954,1000.);
#4198=VECTOR('',#23955,1000.);
#4199=VECTOR('',#23958,1000.);
#4200=VECTOR('',#23959,1000.);
#4201=VECTOR('',#23962,1000.);
#4202=VECTOR('',#23963,1000.);
#4203=VECTOR('',#23966,1000.);
#4204=VECTOR('',#23967,1000.);
#4205=VECTOR('',#23970,1000.);
#4206=VECTOR('',#23973,1000.);
#4207=VECTOR('',#23976,1000.);
#4208=VECTOR('',#23981,1000.);
#4209=VECTOR('',#23984,1000.);
#4210=VECTOR('',#23985,1000.);
#4211=VECTOR('',#23988,1000.);
#4212=VECTOR('',#23989,1000.);
#4213=VECTOR('',#23990,1000.);
#4214=VECTOR('',#23993,1000.);
#4215=VECTOR('',#23994,1000.);
#4216=VECTOR('',#23997,1000.);
#4217=VECTOR('',#23998,1000.);
#4218=VECTOR('',#24001,1000.);
#4219=VECTOR('',#24002,1000.);
#4220=VECTOR('',#24005,1000.);
#4221=VECTOR('',#24006,1000.);
#4222=VECTOR('',#24009,1000.);
#4223=VECTOR('',#24012,1000.);
#4224=VECTOR('',#24021,1000.);
#4225=VECTOR('',#24024,1000.);
#4226=VECTOR('',#24033,1000.);
#4227=VECTOR('',#24034,1000.);
#4228=VECTOR('',#24037,1000.);
#4229=VECTOR('',#24048,1000.);
#4230=VECTOR('',#24051,1000.);
#4231=VECTOR('',#24052,1000.);
#4232=VECTOR('',#24053,1000.);
#4233=VECTOR('',#24056,1000.);
#4234=VECTOR('',#24061,1000.);
#4235=VECTOR('',#24062,1000.);
#4236=VECTOR('',#24063,1000.);
#4237=VECTOR('',#24066,1000.);
#4238=VECTOR('',#24067,1000.);
#4239=VECTOR('',#24072,1000.);
#4240=VECTOR('',#24075,1000.);
#4241=VECTOR('',#24078,1000.);
#4242=VECTOR('',#24085,1000.);
#4243=VECTOR('',#24086,1000.);
#4244=VECTOR('',#24089,1000.);
#4245=VECTOR('',#24092,1000.);
#4246=VECTOR('',#24093,1000.);
#4247=VECTOR('',#24096,1000.);
#4248=VECTOR('',#24097,1000.);
#4249=VECTOR('',#24098,1000.);
#4250=VECTOR('',#24101,1000.);
#4251=VECTOR('',#24102,1000.);
#4252=VECTOR('',#24105,1000.);
#4253=VECTOR('',#24106,1000.);
#4254=VECTOR('',#24109,1000.);
#4255=VECTOR('',#24110,1000.);
#4256=VECTOR('',#24113,1000.);
#4257=VECTOR('',#24114,1000.);
#4258=VECTOR('',#24117,1000.);
#4259=VECTOR('',#24120,1000.);
#4260=VECTOR('',#24123,1000.);
#4261=VECTOR('',#24126,1000.);
#4262=VECTOR('',#24131,1000.);
#4263=VECTOR('',#24132,1000.);
#4264=VECTOR('',#24137,1000.);
#4265=VECTOR('',#24138,1000.);
#4266=VECTOR('',#24139,1000.);
#4267=VECTOR('',#24142,1000.);
#4268=VECTOR('',#24143,1000.);
#4269=VECTOR('',#24146,1000.);
#4270=VECTOR('',#24147,1000.);
#4271=VECTOR('',#24150,1000.);
#4272=VECTOR('',#24151,1000.);
#4273=VECTOR('',#24154,1000.);
#4274=VECTOR('',#24155,1000.);
#4275=VECTOR('',#24158,1000.);
#4276=VECTOR('',#24161,1000.);
#4277=VECTOR('',#24162,1000.);
#4278=VECTOR('',#24163,1000.);
#4279=VECTOR('',#24166,1000.);
#4280=VECTOR('',#24167,1000.);
#4281=VECTOR('',#24170,1000.);
#4282=VECTOR('',#24171,1000.);
#4283=VECTOR('',#24174,1000.);
#4284=VECTOR('',#24175,1000.);
#4285=VECTOR('',#24178,1000.);
#4286=VECTOR('',#24179,1000.);
#4287=VECTOR('',#24182,1000.);
#4288=VECTOR('',#24187,1000.);
#4289=VECTOR('',#24188,1000.);
#4290=VECTOR('',#24189,1000.);
#4291=VECTOR('',#24190,1000.);
#4292=VECTOR('',#24191,1000.);
#4293=VECTOR('',#24192,1000.);
#4294=VECTOR('',#24197,1000.);
#4295=VECTOR('',#24198,1000.);
#4296=VECTOR('',#24199,1000.);
#4297=VECTOR('',#24200,1000.);
#4298=VECTOR('',#24201,1000.);
#4299=VECTOR('',#24202,1000.);
#4300=VECTOR('',#24205,1000.);
#4301=VECTOR('',#24206,1000.);
#4302=VECTOR('',#24207,1000.);
#4303=VECTOR('',#24210,1000.);
#4304=VECTOR('',#24211,1000.);
#4305=VECTOR('',#24212,1000.);
#4306=VECTOR('',#24213,1000.);
#4307=VECTOR('',#24214,1000.);
#4308=VECTOR('',#24217,1000.);
#4309=VECTOR('',#24218,1000.);
#4310=VECTOR('',#24219,1000.);
#4311=VECTOR('',#24222,1000.);
#4312=VECTOR('',#24223,1000.);
#4313=VECTOR('',#24224,1000.);
#4314=VECTOR('',#24227,1000.);
#4315=VECTOR('',#24228,1000.);
#4316=VECTOR('',#24231,1000.);
#4317=VECTOR('',#24232,1000.);
#4318=VECTOR('',#24235,1000.);
#4319=VECTOR('',#24236,1000.);
#4320=VECTOR('',#24239,1000.);
#4321=VECTOR('',#24240,1000.);
#4322=VECTOR('',#24243,1000.);
#4323=VECTOR('',#24248,1000.);
#4324=VECTOR('',#24249,1000.);
#4325=VECTOR('',#24250,1000.);
#4326=VECTOR('',#24251,1000.);
#4327=VECTOR('',#24254,1000.);
#4328=VECTOR('',#24255,1000.);
#4329=VECTOR('',#24258,1000.);
#4330=VECTOR('',#24259,1000.);
#4331=VECTOR('',#24262,1000.);
#4332=VECTOR('',#24263,1000.);
#4333=VECTOR('',#24266,1000.);
#4334=VECTOR('',#24269,1000.);
#4335=VECTOR('',#24270,1000.);
#4336=VECTOR('',#24273,1000.);
#4337=VECTOR('',#24278,1000.);
#4338=VECTOR('',#24283,1000.);
#4339=VECTOR('',#24288,1000.);
#4340=VECTOR('',#24289,1000.);
#4341=VECTOR('',#24294,1000.);
#4342=VECTOR('',#24297,1000.);
#4343=VECTOR('',#24300,1000.);
#4344=VECTOR('',#24301,1000.);
#4345=VECTOR('',#24302,1000.);
#4346=VECTOR('',#24307,1000.);
#4347=VECTOR('',#24308,1000.);
#4348=VECTOR('',#24311,1000.);
#4349=VECTOR('',#24312,1000.);
#4350=VECTOR('',#24315,1000.);
#4351=VECTOR('',#24318,1000.);
#4352=VECTOR('',#24325,1000.);
#4353=VECTOR('',#24330,1000.);
#4354=VECTOR('',#24335,1000.);
#4355=VECTOR('',#24336,1000.);
#4356=VECTOR('',#24337,1000.);
#4357=VECTOR('',#24340,1000.);
#4358=VECTOR('',#24341,1000.);
#4359=VECTOR('',#24344,1000.);
#4360=VECTOR('',#24345,1000.);
#4361=VECTOR('',#24348,1000.);
#4362=VECTOR('',#24349,1000.);
#4363=VECTOR('',#24352,1000.);
#4364=VECTOR('',#24353,1000.);
#4365=VECTOR('',#24356,1000.);
#4366=VECTOR('',#24359,1000.);
#4367=VECTOR('',#24362,1000.);
#4368=VECTOR('',#24365,1000.);
#4369=VECTOR('',#24366,1000.);
#4370=VECTOR('',#24367,1000.);
#4371=VECTOR('',#24370,1000.);
#4372=VECTOR('',#24371,1000.);
#4373=VECTOR('',#24374,1000.);
#4374=VECTOR('',#24375,1000.);
#4375=VECTOR('',#24378,1000.);
#4376=VECTOR('',#24381,1000.);
#4377=VECTOR('',#24386,1000.);
#4378=VECTOR('',#24389,1000.);
#4379=VECTOR('',#24390,1000.);
#4380=VECTOR('',#24393,1000.);
#4381=VECTOR('',#24398,1000.);
#4382=VECTOR('',#24403,1000.);
#4383=VECTOR('',#24406,1000.);
#4384=VECTOR('',#24407,1000.);
#4385=VECTOR('',#24412,1000.);
#4386=VECTOR('',#24417,1000.);
#4387=VECTOR('',#24418,1000.);
#4388=VECTOR('',#24423,1000.);
#4389=VECTOR('',#24428,1000.);
#4390=VECTOR('',#24429,1000.);
#4391=VECTOR('',#24432,1000.);
#4392=VECTOR('',#24435,1000.);
#4393=VECTOR('',#24440,1000.);
#4394=VECTOR('',#24477,1000.);
#4395=VECTOR('',#24478,1000.);
#4396=VECTOR('',#24479,1000.);
#4397=VECTOR('',#24480,1000.);
#4398=VECTOR('',#24481,1000.);
#4399=VECTOR('',#24482,1000.);
#4400=VECTOR('',#24485,1000.);
#4401=VECTOR('',#24486,1000.);
#4402=VECTOR('',#24489,1000.);
#4403=VECTOR('',#24490,1000.);
#4404=VECTOR('',#24491,1000.);
#4405=VECTOR('',#24494,1000.);
#4406=VECTOR('',#24495,1000.);
#4407=VECTOR('',#24498,1000.);
#4408=VECTOR('',#24499,1000.);
#4409=VECTOR('',#24500,1000.);
#4410=VECTOR('',#24503,1000.);
#4411=VECTOR('',#24504,1000.);
#4412=VECTOR('',#24507,1000.);
#4413=VECTOR('',#24508,1000.);
#4414=VECTOR('',#24509,1000.);
#4415=VECTOR('',#24510,1000.);
#4416=VECTOR('',#24511,1000.);
#4417=VECTOR('',#24512,1000.);
#4418=VECTOR('',#24513,1000.);
#4419=VECTOR('',#24514,1000.);
#4420=VECTOR('',#24515,1000.);
#4421=VECTOR('',#24516,1000.);
#4422=VECTOR('',#24519,1000.);
#4423=VECTOR('',#24520,1000.);
#4424=VECTOR('',#24523,1000.);
#4425=VECTOR('',#24524,1000.);
#4426=VECTOR('',#24525,1000.);
#4427=VECTOR('',#24528,1000.);
#4428=VECTOR('',#24529,1000.);
#4429=VECTOR('',#24532,1000.);
#4430=VECTOR('',#24533,1000.);
#4431=VECTOR('',#24534,1000.);
#4432=VECTOR('',#24537,1000.);
#4433=VECTOR('',#24538,1000.);
#4434=VECTOR('',#24541,1000.);
#4435=VECTOR('',#24542,1000.);
#4436=VECTOR('',#24543,1000.);
#4437=VECTOR('',#24544,1000.);
#4438=VECTOR('',#24545,1000.);
#4439=VECTOR('',#24548,1000.);
#4440=VECTOR('',#24549,1000.);
#4441=VECTOR('',#24550,1000.);
#4442=VECTOR('',#24555,1000.);
#4443=VECTOR('',#24556,1000.);
#4444=VECTOR('',#24561,1000.);
#4445=VECTOR('',#24562,1000.);
#4446=VECTOR('',#24567,1000.);
#4447=VECTOR('',#24568,1000.);
#4448=VECTOR('',#24571,1000.);
#4449=VECTOR('',#24572,1000.);
#4450=VECTOR('',#24573,1000.);
#4451=VECTOR('',#24574,1000.);
#4452=VECTOR('',#24575,1000.);
#4453=VECTOR('',#24576,1000.);
#4454=VECTOR('',#24579,1000.);
#4455=VECTOR('',#24580,1000.);
#4456=VECTOR('',#24583,1000.);
#4457=VECTOR('',#24586,1000.);
#4458=VECTOR('',#24589,1000.);
#4459=VECTOR('',#24590,1000.);
#4460=VECTOR('',#24593,1000.);
#4461=VECTOR('',#24594,1000.);
#4462=VECTOR('',#24597,1000.);
#4463=VECTOR('',#24598,1000.);
#4464=VECTOR('',#24599,1000.);
#4465=VECTOR('',#24600,1000.);
#4466=VECTOR('',#24601,1000.);
#4467=VECTOR('',#24624,1000.);
#4468=VECTOR('',#24625,1000.);
#4469=VECTOR('',#24626,1000.);
#4470=VECTOR('',#24627,1000.);
#4471=VECTOR('',#24630,1000.);
#4472=VECTOR('',#24631,1000.);
#4473=VECTOR('',#24632,1000.);
#4474=VECTOR('',#24635,1000.);
#4475=VECTOR('',#24636,1000.);
#4476=VECTOR('',#24639,1000.);
#4477=VECTOR('',#24642,1000.);
#4478=VECTOR('',#24645,1000.);
#4479=VECTOR('',#24646,1000.);
#4480=VECTOR('',#24649,1000.);
#4481=VECTOR('',#24650,1000.);
#4482=VECTOR('',#24651,1000.);
#4483=VECTOR('',#24654,1000.);
#4484=VECTOR('',#24655,1000.);
#4485=VECTOR('',#24658,1000.);
#4486=VECTOR('',#24659,1000.);
#4487=VECTOR('',#24662,1000.);
#4488=VECTOR('',#24663,1000.);
#4489=VECTOR('',#24664,1000.);
#4490=VECTOR('',#24667,1000.);
#4491=VECTOR('',#24668,1000.);
#4492=VECTOR('',#24669,1000.);
#4493=VECTOR('',#24672,1000.);
#4494=VECTOR('',#24673,1000.);
#4495=VECTOR('',#24676,1000.);
#4496=VECTOR('',#24677,1000.);
#4497=VECTOR('',#24680,1000.);
#4498=VECTOR('',#24683,1000.);
#4499=VECTOR('',#24686,1000.);
#4500=VECTOR('',#24689,1000.);
#4501=VECTOR('',#24690,1000.);
#4502=VECTOR('',#24691,1000.);
#4503=VECTOR('',#24692,1000.);
#4504=VECTOR('',#24695,1000.);
#4505=VECTOR('',#24696,1000.);
#4506=VECTOR('',#24699,1000.);
#4507=VECTOR('',#24700,1000.);
#4508=VECTOR('',#24701,1000.);
#4509=VECTOR('',#24704,1000.);
#4510=VECTOR('',#24705,1000.);
#4511=VECTOR('',#24706,1000.);
#4512=VECTOR('',#24709,1000.);
#4513=VECTOR('',#24710,1000.);
#4514=VECTOR('',#24713,1000.);
#4515=VECTOR('',#24714,1000.);
#4516=VECTOR('',#24717,1000.);
#4517=VECTOR('',#24718,1000.);
#4518=VECTOR('',#24721,1000.);
#4519=VECTOR('',#24722,1000.);
#4520=VECTOR('',#24725,1000.);
#4521=VECTOR('',#24726,1000.);
#4522=VECTOR('',#24729,1000.);
#4523=VECTOR('',#24730,1000.);
#4524=VECTOR('',#24733,1000.);
#4525=VECTOR('',#24734,1000.);
#4526=VECTOR('',#24737,1000.);
#4527=VECTOR('',#24738,1000.);
#4528=VECTOR('',#24741,1000.);
#4529=VECTOR('',#24742,1000.);
#4530=VECTOR('',#24745,1000.);
#4531=VECTOR('',#24746,1000.);
#4532=VECTOR('',#24749,1000.);
#4674=CYLINDRICAL_SURFACE('',#18876,55.);
#4675=CYLINDRICAL_SURFACE('',#18910,6.75000000000001);
#4676=CYLINDRICAL_SURFACE('',#18913,6.75);
#4677=CYLINDRICAL_SURFACE('',#18916,6.75000000000001);
#4678=CYLINDRICAL_SURFACE('',#18919,6.75);
#4679=CYLINDRICAL_SURFACE('',#18922,7.00000000000001);
#4680=CYLINDRICAL_SURFACE('',#18927,27.5);
#4681=CYLINDRICAL_SURFACE('',#18935,22.);
#4682=CYLINDRICAL_SURFACE('',#18938,7.);
#4683=CYLINDRICAL_SURFACE('',#18941,7.);
#4684=CYLINDRICAL_SURFACE('',#18946,7.);
#4685=CYLINDRICAL_SURFACE('',#18953,80.);
#4686=CYLINDRICAL_SURFACE('',#18956,40.);
#4687=CYLINDRICAL_SURFACE('',#18959,12.);
#4688=CYLINDRICAL_SURFACE('',#18960,12.);
#4689=CYLINDRICAL_SURFACE('',#18961,12.);
#4690=CYLINDRICAL_SURFACE('',#18964,12.);
#4691=CYLINDRICAL_SURFACE('',#18966,12.);
#4692=CYLINDRICAL_SURFACE('',#18967,53.);
#4693=CYLINDRICAL_SURFACE('',#18971,4.5);
#4694=CYLINDRICAL_SURFACE('',#18974,4.5);
#4695=CYLINDRICAL_SURFACE('',#18977,4.5);
#4696=CYLINDRICAL_SURFACE('',#18980,4.5);
#4697=CYLINDRICAL_SURFACE('',#18983,20.);
#4698=CYLINDRICAL_SURFACE('',#18986,12.);
#4699=CYLINDRICAL_SURFACE('',#18988,10.);
#4700=CYLINDRICAL_SURFACE('',#18990,12.);
#4701=CYLINDRICAL_SURFACE('',#19003,7.00000000000001);
#4702=CYLINDRICAL_SURFACE('',#19009,12.);
#4703=CYLINDRICAL_SURFACE('',#19012,68.);
#4704=CYLINDRICAL_SURFACE('',#19018,4.);
#4705=CYLINDRICAL_SURFACE('',#19021,4.);
#4706=CYLINDRICAL_SURFACE('',#19024,4.);
#4707=CYLINDRICAL_SURFACE('',#19027,4.);
#4708=CYLINDRICAL_SURFACE('',#19030,17.4625);
#4709=CYLINDRICAL_SURFACE('',#19037,7.99999999999999);
#4710=CYLINDRICAL_SURFACE('',#19040,8.00000000000001);
#4711=CYLINDRICAL_SURFACE('',#19045,7.00000000000001);
#4712=CYLINDRICAL_SURFACE('',#19048,7.00000000000001);
#4713=CYLINDRICAL_SURFACE('',#19051,3.);
#4714=CYLINDRICAL_SURFACE('',#19054,3.00000000000307);
#4715=CYLINDRICAL_SURFACE('',#19057,3.0000000000021);
#4716=CYLINDRICAL_SURFACE('',#19060,2.99999999999927);
#4717=CYLINDRICAL_SURFACE('',#19063,68.);
#4718=CYLINDRICAL_SURFACE('',#19066,6.7500000000354);
#4719=CYLINDRICAL_SURFACE('',#19075,5.5);
#4720=CYLINDRICAL_SURFACE('',#19084,8.80000000000425);
#4721=CYLINDRICAL_SURFACE('',#19087,8.80000000000425);
#4722=CYLINDRICAL_SURFACE('',#19092,5.5);
#4723=CYLINDRICAL_SURFACE('',#19096,179.5);
#4724=CYLINDRICAL_SURFACE('',#19132,7.00000000000001);
#4725=CYLINDRICAL_SURFACE('',#19145,7.00000000000001);
#4726=CYLINDRICAL_SURFACE('',#19158,7.00000000000001);
#4727=CYLINDRICAL_SURFACE('',#19173,7.00000000000001);
#4728=CYLINDRICAL_SURFACE('',#19177,16.);
#4729=CYLINDRICAL_SURFACE('',#19180,16.);
#4730=CYLINDRICAL_SURFACE('',#19182,179.5);
#4731=CYLINDRICAL_SURFACE('',#19184,16.);
#4732=CYLINDRICAL_SURFACE('',#19187,16.);
#4733=CYLINDRICAL_SURFACE('',#19189,179.5);
#4734=CYLINDRICAL_SURFACE('',#19191,16.);
#4735=CYLINDRICAL_SURFACE('',#19194,16.);
#4736=CYLINDRICAL_SURFACE('',#19196,16.);
#4737=CYLINDRICAL_SURFACE('',#19199,16.);
#4738=CYLINDRICAL_SURFACE('',#19201,179.5);
#4739=CYLINDRICAL_SURFACE('',#19227,7.00000000000001);
#4740=CYLINDRICAL_SURFACE('',#19228,7.00000000000001);
#4741=CYLINDRICAL_SURFACE('',#19231,7.00000000000001);
#4742=CYLINDRICAL_SURFACE('',#19236,7.00000000000001);
#4743=CYLINDRICAL_SURFACE('',#19240,80.5);
#4744=CYLINDRICAL_SURFACE('',#19244,80.5);
#4745=CYLINDRICAL_SURFACE('',#19248,80.5);
#4746=CYLINDRICAL_SURFACE('',#19252,80.5);
#4747=CYLINDRICAL_SURFACE('',#19266,7.00000000000001);
#4748=CYLINDRICAL_SURFACE('',#19269,7.00000000000001);
#4749=CYLINDRICAL_SURFACE('',#19272,7.00000000000001);
#4750=CYLINDRICAL_SURFACE('',#19275,7.00000000000001);
#4751=CYLINDRICAL_SURFACE('',#19347,4.);
#4752=CYLINDRICAL_SURFACE('',#19350,4.);
#4753=CYLINDRICAL_SURFACE('',#19352,4.);
#4754=CYLINDRICAL_SURFACE('',#19354,4.);
#4755=CYLINDRICAL_SURFACE('',#19385,1.);
#4756=CYLINDRICAL_SURFACE('',#19386,1.);
#4757=CYLINDRICAL_SURFACE('',#19387,1.);
#4758=CYLINDRICAL_SURFACE('',#19388,1.);
#4759=CYLINDRICAL_SURFACE('',#19435,68.);
#4760=CYLINDRICAL_SURFACE('',#19438,77.);
#4761=CYLINDRICAL_SURFACE('',#19444,68.);
#4762=CYLINDRICAL_SURFACE('',#19446,77.);
#4763=CYLINDRICAL_SURFACE('',#19449,68.);
#4764=CYLINDRICAL_SURFACE('',#19452,77.);
#4765=CYLINDRICAL_SURFACE('',#19457,77.);
#4766=CYLINDRICAL_SURFACE('',#19466,5.);
#4767=CYLINDRICAL_SURFACE('',#19479,5.);
#4768=CYLINDRICAL_SURFACE('',#19488,5.);
#4769=CYLINDRICAL_SURFACE('',#19493,5.);
#4770=CYLINDRICAL_SURFACE('',#19506,77.);
#4771=CYLINDRICAL_SURFACE('',#19509,4.);
#4772=CYLINDRICAL_SURFACE('',#19514,4.);
#4773=CYLINDRICAL_SURFACE('',#19519,77.);
#4774=CYLINDRICAL_SURFACE('',#19522,4.);
#4775=CYLINDRICAL_SURFACE('',#19527,4.);
#4776=CYLINDRICAL_SURFACE('',#19532,77.);
#4777=CYLINDRICAL_SURFACE('',#19535,4.);
#4778=CYLINDRICAL_SURFACE('',#19540,4.);
#4779=CYLINDRICAL_SURFACE('',#19545,77.);
#4780=CYLINDRICAL_SURFACE('',#19548,4.);
#4781=CYLINDRICAL_SURFACE('',#19553,4.);
#4782=CYLINDRICAL_SURFACE('',#19604,76.5);
#4783=CYLINDRICAL_SURFACE('',#19606,68.);
#4784=CYLINDRICAL_SURFACE('',#19608,76.5);
#4785=CYLINDRICAL_SURFACE('',#19611,76.5);
#4786=CYLINDRICAL_SURFACE('',#19613,68.);
#4787=CYLINDRICAL_SURFACE('',#19615,76.5);
#4788=CYLINDRICAL_SURFACE('',#19617,68.);
#4789=CYLINDRICAL_SURFACE('',#19627,12.);
#4790=CYLINDRICAL_SURFACE('',#19634,10.);
#4791=CYLINDRICAL_SURFACE('',#19644,4.5);
#4792=CYLINDRICAL_SURFACE('',#19682,2.);
#4793=CYLINDRICAL_SURFACE('',#19686,2.);
#4794=CYLINDRICAL_SURFACE('',#19706,10.);
#4795=CYLINDRICAL_SURFACE('',#19717,10.);
#4796=CYLINDRICAL_SURFACE('',#19728,12.);
#4797=CYLINDRICAL_SURFACE('',#19729,12.);
#4798=CYLINDRICAL_SURFACE('',#19730,12.);
#4799=CYLINDRICAL_SURFACE('',#19734,2.);
#4800=CYLINDRICAL_SURFACE('',#19738,2.);
#4801=CYLINDRICAL_SURFACE('',#19741,12.);
#4802=CYLINDRICAL_SURFACE('',#19742,12.);
#4803=CYLINDRICAL_SURFACE('',#19743,12.);
#4804=CYLINDRICAL_SURFACE('',#19752,10.);
#4805=CYLINDRICAL_SURFACE('',#19756,6.);
#4806=CYLINDRICAL_SURFACE('',#19766,10.);
#4807=CYLINDRICAL_SURFACE('',#19804,2.5);
#4808=CYLINDRICAL_SURFACE('',#19810,6.00000000000001);
#4809=CYLINDRICAL_SURFACE('',#19813,6.00000000000001);
#4810=CYLINDRICAL_SURFACE('',#19816,2.5);
#4811=CYLINDRICAL_SURFACE('',#19819,6.00000000000001);
#4812=CYLINDRICAL_SURFACE('',#19846,6.);
#4813=CYLINDRICAL_SURFACE('',#19850,6.);
#4814=CYLINDRICAL_SURFACE('',#19862,23.5);
#4815=CYLINDRICAL_SURFACE('',#19871,20.5);
#4816=CYLINDRICAL_SURFACE('',#19889,12.);
#4817=CYLINDRICAL_SURFACE('',#19891,12.);
#4818=CYLINDRICAL_SURFACE('',#19893,12.);
#4819=CYLINDRICAL_SURFACE('',#19902,12.);
#5076=FACE_OUTER_BOUND('',#6189,.T.);
#5077=FACE_OUTER_BOUND('',#6190,.T.);
#5078=FACE_OUTER_BOUND('',#6191,.T.);
#5079=FACE_OUTER_BOUND('',#6192,.T.);
#5080=FACE_OUTER_BOUND('',#6193,.T.);
#5081=FACE_OUTER_BOUND('',#6194,.T.);
#5082=FACE_OUTER_BOUND('',#6195,.T.);
#5083=FACE_OUTER_BOUND('',#6196,.T.);
#5084=FACE_OUTER_BOUND('',#6197,.T.);
#5085=FACE_OUTER_BOUND('',#6198,.T.);
#5086=FACE_OUTER_BOUND('',#6200,.T.);
#5087=FACE_OUTER_BOUND('',#6202,.T.);
#5088=FACE_OUTER_BOUND('',#6203,.T.);
#5089=FACE_OUTER_BOUND('',#6204,.T.);
#5090=FACE_OUTER_BOUND('',#6206,.T.);
#5091=FACE_OUTER_BOUND('',#6207,.T.);
#5092=FACE_OUTER_BOUND('',#6208,.T.);
#5093=FACE_OUTER_BOUND('',#6209,.T.);
#5094=FACE_OUTER_BOUND('',#6210,.T.);
#5095=FACE_OUTER_BOUND('',#6211,.T.);
#5096=FACE_OUTER_BOUND('',#6212,.T.);
#5097=FACE_OUTER_BOUND('',#6213,.T.);
#5098=FACE_OUTER_BOUND('',#6214,.T.);
#5099=FACE_OUTER_BOUND('',#6215,.T.);
#5100=FACE_OUTER_BOUND('',#6216,.T.);
#5101=FACE_OUTER_BOUND('',#6217,.T.);
#5102=FACE_OUTER_BOUND('',#6218,.T.);
#5103=FACE_OUTER_BOUND('',#6219,.T.);
#5104=FACE_OUTER_BOUND('',#6220,.T.);
#5105=FACE_OUTER_BOUND('',#6221,.T.);
#5106=FACE_OUTER_BOUND('',#6222,.T.);
#5107=FACE_OUTER_BOUND('',#6223,.T.);
#5108=FACE_OUTER_BOUND('',#6224,.T.);
#5109=FACE_OUTER_BOUND('',#6225,.T.);
#5110=FACE_OUTER_BOUND('',#6226,.T.);
#5111=FACE_OUTER_BOUND('',#6227,.T.);
#5112=FACE_OUTER_BOUND('',#6228,.T.);
#5113=FACE_OUTER_BOUND('',#6229,.T.);
#5114=FACE_OUTER_BOUND('',#6230,.T.);
#5115=FACE_OUTER_BOUND('',#6231,.T.);
#5116=FACE_OUTER_BOUND('',#6232,.T.);
#5117=FACE_OUTER_BOUND('',#6233,.T.);
#5118=FACE_OUTER_BOUND('',#6234,.T.);
#5119=FACE_OUTER_BOUND('',#6235,.T.);
#5120=FACE_OUTER_BOUND('',#6236,.T.);
#5121=FACE_OUTER_BOUND('',#6237,.T.);
#5122=FACE_OUTER_BOUND('',#6238,.T.);
#5123=FACE_OUTER_BOUND('',#6239,.T.);
#5124=FACE_OUTER_BOUND('',#6240,.T.);
#5125=FACE_OUTER_BOUND('',#6241,.T.);
#5126=FACE_OUTER_BOUND('',#6242,.T.);
#5127=FACE_OUTER_BOUND('',#6243,.T.);
#5128=FACE_OUTER_BOUND('',#6244,.T.);
#5129=FACE_OUTER_BOUND('',#6245,.T.);
#5130=FACE_OUTER_BOUND('',#6246,.T.);
#5131=FACE_OUTER_BOUND('',#6247,.T.);
#5132=FACE_OUTER_BOUND('',#6249,.T.);
#5133=FACE_OUTER_BOUND('',#6250,.T.);
#5134=FACE_OUTER_BOUND('',#6251,.T.);
#5135=FACE_OUTER_BOUND('',#6252,.T.);
#5136=FACE_OUTER_BOUND('',#6253,.T.);
#5137=FACE_OUTER_BOUND('',#6254,.T.);
#5138=FACE_OUTER_BOUND('',#6255,.T.);
#5139=FACE_OUTER_BOUND('',#6256,.T.);
#5140=FACE_OUTER_BOUND('',#6257,.T.);
#5141=FACE_OUTER_BOUND('',#6258,.T.);
#5142=FACE_OUTER_BOUND('',#6259,.T.);
#5143=FACE_OUTER_BOUND('',#6260,.T.);
#5144=FACE_OUTER_BOUND('',#6261,.T.);
#5145=FACE_OUTER_BOUND('',#6262,.T.);
#5146=FACE_OUTER_BOUND('',#6263,.T.);
#5147=FACE_OUTER_BOUND('',#6264,.T.);
#5148=FACE_OUTER_BOUND('',#6265,.T.);
#5149=FACE_OUTER_BOUND('',#6266,.T.);
#5150=FACE_OUTER_BOUND('',#6267,.T.);
#5151=FACE_OUTER_BOUND('',#6268,.T.);
#5152=FACE_OUTER_BOUND('',#6269,.T.);
#5153=FACE_OUTER_BOUND('',#6270,.T.);
#5154=FACE_OUTER_BOUND('',#6271,.T.);
#5155=FACE_OUTER_BOUND('',#6272,.T.);
#5156=FACE_OUTER_BOUND('',#6273,.T.);
#5157=FACE_OUTER_BOUND('',#6274,.T.);
#5158=FACE_OUTER_BOUND('',#6275,.T.);
#5159=FACE_OUTER_BOUND('',#6276,.T.);
#5160=FACE_OUTER_BOUND('',#6277,.T.);
#5161=FACE_OUTER_BOUND('',#6278,.T.);
#5162=FACE_OUTER_BOUND('',#6279,.T.);
#5163=FACE_OUTER_BOUND('',#6280,.T.);
#5164=FACE_OUTER_BOUND('',#6281,.T.);
#5165=FACE_OUTER_BOUND('',#6282,.T.);
#5166=FACE_OUTER_BOUND('',#6283,.T.);
#5167=FACE_OUTER_BOUND('',#6284,.T.);
#5168=FACE_OUTER_BOUND('',#6285,.T.);
#5169=FACE_OUTER_BOUND('',#6286,.T.);
#5170=FACE_OUTER_BOUND('',#6287,.T.);
#5171=FACE_OUTER_BOUND('',#6288,.T.);
#5172=FACE_OUTER_BOUND('',#6289,.T.);
#5173=FACE_OUTER_BOUND('',#6290,.T.);
#5174=FACE_OUTER_BOUND('',#6291,.T.);
#5175=FACE_OUTER_BOUND('',#6292,.T.);
#5176=FACE_OUTER_BOUND('',#6293,.T.);
#5177=FACE_OUTER_BOUND('',#6294,.T.);
#5178=FACE_OUTER_BOUND('',#6295,.T.);
#5179=FACE_OUTER_BOUND('',#6296,.T.);
#5180=FACE_OUTER_BOUND('',#6297,.T.);
#5181=FACE_OUTER_BOUND('',#6298,.T.);
#5182=FACE_OUTER_BOUND('',#6299,.T.);
#5183=FACE_OUTER_BOUND('',#6300,.T.);
#5184=FACE_OUTER_BOUND('',#6301,.T.);
#5185=FACE_OUTER_BOUND('',#6302,.T.);
#5186=FACE_OUTER_BOUND('',#6303,.T.);
#5187=FACE_OUTER_BOUND('',#6304,.T.);
#5188=FACE_OUTER_BOUND('',#6305,.T.);
#5189=FACE_OUTER_BOUND('',#6306,.T.);
#5190=FACE_OUTER_BOUND('',#6307,.T.);
#5191=FACE_OUTER_BOUND('',#6308,.T.);
#5192=FACE_OUTER_BOUND('',#6309,.T.);
#5193=FACE_OUTER_BOUND('',#6310,.T.);
#5194=FACE_OUTER_BOUND('',#6311,.T.);
#5195=FACE_OUTER_BOUND('',#6312,.T.);
#5196=FACE_OUTER_BOUND('',#6313,.T.);
#5197=FACE_OUTER_BOUND('',#6314,.T.);
#5198=FACE_OUTER_BOUND('',#6315,.T.);
#5199=FACE_OUTER_BOUND('',#6316,.T.);
#5200=FACE_OUTER_BOUND('',#6317,.T.);
#5201=FACE_OUTER_BOUND('',#6318,.T.);
#5202=FACE_OUTER_BOUND('',#6319,.T.);
#5203=FACE_OUTER_BOUND('',#6320,.T.);
#5204=FACE_OUTER_BOUND('',#6321,.T.);
#5205=FACE_OUTER_BOUND('',#6322,.T.);
#5206=FACE_OUTER_BOUND('',#6323,.T.);
#5207=FACE_OUTER_BOUND('',#6324,.T.);
#5208=FACE_OUTER_BOUND('',#6325,.T.);
#5209=FACE_OUTER_BOUND('',#6326,.T.);
#5210=FACE_OUTER_BOUND('',#6327,.T.);
#5211=FACE_OUTER_BOUND('',#6328,.T.);
#5212=FACE_OUTER_BOUND('',#6329,.T.);
#5213=FACE_OUTER_BOUND('',#6330,.T.);
#5214=FACE_OUTER_BOUND('',#6331,.T.);
#5215=FACE_OUTER_BOUND('',#6332,.T.);
#5216=FACE_OUTER_BOUND('',#6333,.T.);
#5217=FACE_OUTER_BOUND('',#6334,.T.);
#5218=FACE_OUTER_BOUND('',#6335,.T.);
#5219=FACE_OUTER_BOUND('',#6336,.T.);
#5220=FACE_OUTER_BOUND('',#6337,.T.);
#5221=FACE_OUTER_BOUND('',#6338,.T.);
#5222=FACE_OUTER_BOUND('',#6339,.T.);
#5223=FACE_OUTER_BOUND('',#6340,.T.);
#5224=FACE_OUTER_BOUND('',#6341,.T.);
#5225=FACE_OUTER_BOUND('',#6342,.T.);
#5226=FACE_OUTER_BOUND('',#6343,.T.);
#5227=FACE_OUTER_BOUND('',#6344,.T.);
#5228=FACE_OUTER_BOUND('',#6345,.T.);
#5229=FACE_OUTER_BOUND('',#6346,.T.);
#5230=FACE_OUTER_BOUND('',#6347,.T.);
#5231=FACE_OUTER_BOUND('',#6348,.T.);
#5232=FACE_OUTER_BOUND('',#6349,.T.);
#5233=FACE_OUTER_BOUND('',#6350,.T.);
#5234=FACE_OUTER_BOUND('',#6351,.T.);
#5235=FACE_OUTER_BOUND('',#6352,.T.);
#5236=FACE_OUTER_BOUND('',#6353,.T.);
#5237=FACE_OUTER_BOUND('',#6354,.T.);
#5238=FACE_OUTER_BOUND('',#6355,.T.);
#5239=FACE_OUTER_BOUND('',#6356,.T.);
#5240=FACE_OUTER_BOUND('',#6357,.T.);
#5241=FACE_OUTER_BOUND('',#6358,.T.);
#5242=FACE_OUTER_BOUND('',#6359,.T.);
#5243=FACE_OUTER_BOUND('',#6360,.T.);
#5244=FACE_OUTER_BOUND('',#6361,.T.);
#5245=FACE_OUTER_BOUND('',#6362,.T.);
#5246=FACE_OUTER_BOUND('',#6363,.T.);
#5247=FACE_OUTER_BOUND('',#6365,.T.);
#5248=FACE_OUTER_BOUND('',#6366,.T.);
#5249=FACE_OUTER_BOUND('',#6368,.T.);
#5250=FACE_OUTER_BOUND('',#6370,.T.);
#5251=FACE_OUTER_BOUND('',#6371,.T.);
#5252=FACE_OUTER_BOUND('',#6373,.T.);
#5253=FACE_OUTER_BOUND('',#6374,.T.);
#5254=FACE_OUTER_BOUND('',#6375,.T.);
#5255=FACE_OUTER_BOUND('',#6376,.T.);
#5256=FACE_OUTER_BOUND('',#6377,.T.);
#5257=FACE_OUTER_BOUND('',#6378,.T.);
#5258=FACE_OUTER_BOUND('',#6379,.T.);
#5259=FACE_OUTER_BOUND('',#6380,.T.);
#5260=FACE_OUTER_BOUND('',#6381,.T.);
#5261=FACE_OUTER_BOUND('',#6382,.T.);
#5262=FACE_OUTER_BOUND('',#6383,.T.);
#5263=FACE_OUTER_BOUND('',#6384,.T.);
#5264=FACE_OUTER_BOUND('',#6385,.T.);
#5265=FACE_OUTER_BOUND('',#6387,.T.);
#5266=FACE_OUTER_BOUND('',#6389,.T.);
#5267=FACE_OUTER_BOUND('',#6391,.T.);
#5268=FACE_OUTER_BOUND('',#6393,.T.);
#5269=FACE_OUTER_BOUND('',#6394,.T.);
#5270=FACE_OUTER_BOUND('',#6395,.T.);
#5271=FACE_OUTER_BOUND('',#6396,.T.);
#5272=FACE_OUTER_BOUND('',#6397,.T.);
#5273=FACE_OUTER_BOUND('',#6398,.T.);
#5274=FACE_OUTER_BOUND('',#6399,.T.);
#5275=FACE_OUTER_BOUND('',#6400,.T.);
#5276=FACE_OUTER_BOUND('',#6401,.T.);
#5277=FACE_OUTER_BOUND('',#6402,.T.);
#5278=FACE_OUTER_BOUND('',#6403,.T.);
#5279=FACE_OUTER_BOUND('',#6404,.T.);
#5280=FACE_OUTER_BOUND('',#6405,.T.);
#5281=FACE_OUTER_BOUND('',#6406,.T.);
#5282=FACE_OUTER_BOUND('',#6407,.T.);
#5283=FACE_OUTER_BOUND('',#6408,.T.);
#5284=FACE_OUTER_BOUND('',#6409,.T.);
#5285=FACE_OUTER_BOUND('',#6410,.T.);
#5286=FACE_OUTER_BOUND('',#6411,.T.);
#5287=FACE_OUTER_BOUND('',#6412,.T.);
#5288=FACE_OUTER_BOUND('',#6413,.T.);
#5289=FACE_OUTER_BOUND('',#6414,.T.);
#5290=FACE_OUTER_BOUND('',#6415,.T.);
#5291=FACE_OUTER_BOUND('',#6416,.T.);
#5292=FACE_OUTER_BOUND('',#6417,.T.);
#5293=FACE_OUTER_BOUND('',#6418,.T.);
#5294=FACE_OUTER_BOUND('',#6419,.T.);
#5295=FACE_OUTER_BOUND('',#6420,.T.);
#5296=FACE_OUTER_BOUND('',#6421,.T.);
#5297=FACE_OUTER_BOUND('',#6422,.T.);
#5298=FACE_OUTER_BOUND('',#6423,.T.);
#5299=FACE_OUTER_BOUND('',#6424,.T.);
#5300=FACE_OUTER_BOUND('',#6425,.T.);
#5301=FACE_OUTER_BOUND('',#6426,.T.);
#5302=FACE_OUTER_BOUND('',#6427,.T.);
#5303=FACE_OUTER_BOUND('',#6428,.T.);
#5304=FACE_OUTER_BOUND('',#6429,.T.);
#5305=FACE_OUTER_BOUND('',#6430,.T.);
#5306=FACE_OUTER_BOUND('',#6431,.T.);
#5307=FACE_OUTER_BOUND('',#6432,.T.);
#5308=FACE_OUTER_BOUND('',#6433,.T.);
#5309=FACE_OUTER_BOUND('',#6434,.T.);
#5310=FACE_OUTER_BOUND('',#6435,.T.);
#5311=FACE_OUTER_BOUND('',#6436,.T.);
#5312=FACE_OUTER_BOUND('',#6437,.T.);
#5313=FACE_OUTER_BOUND('',#6438,.T.);
#5314=FACE_OUTER_BOUND('',#6439,.T.);
#5315=FACE_OUTER_BOUND('',#6440,.T.);
#5316=FACE_OUTER_BOUND('',#6441,.T.);
#5317=FACE_OUTER_BOUND('',#6442,.T.);
#5318=FACE_OUTER_BOUND('',#6443,.T.);
#5319=FACE_OUTER_BOUND('',#6444,.T.);
#5320=FACE_OUTER_BOUND('',#6445,.T.);
#5321=FACE_OUTER_BOUND('',#6446,.T.);
#5322=FACE_OUTER_BOUND('',#6447,.T.);
#5323=FACE_OUTER_BOUND('',#6448,.T.);
#5324=FACE_OUTER_BOUND('',#6449,.T.);
#5325=FACE_OUTER_BOUND('',#6450,.T.);
#5326=FACE_OUTER_BOUND('',#6451,.T.);
#5327=FACE_OUTER_BOUND('',#6452,.T.);
#5328=FACE_OUTER_BOUND('',#6453,.T.);
#5329=FACE_OUTER_BOUND('',#6454,.T.);
#5330=FACE_OUTER_BOUND('',#6455,.T.);
#5331=FACE_OUTER_BOUND('',#6456,.T.);
#5332=FACE_OUTER_BOUND('',#6457,.T.);
#5333=FACE_OUTER_BOUND('',#6458,.T.);
#5334=FACE_OUTER_BOUND('',#6459,.T.);
#5335=FACE_OUTER_BOUND('',#6460,.T.);
#5336=FACE_OUTER_BOUND('',#6461,.T.);
#5337=FACE_OUTER_BOUND('',#6462,.T.);
#5338=FACE_OUTER_BOUND('',#6463,.T.);
#5339=FACE_OUTER_BOUND('',#6464,.T.);
#5340=FACE_OUTER_BOUND('',#6465,.T.);
#5341=FACE_OUTER_BOUND('',#6467,.T.);
#5342=FACE_OUTER_BOUND('',#6468,.T.);
#5343=FACE_OUTER_BOUND('',#6469,.T.);
#5344=FACE_OUTER_BOUND('',#6470,.T.);
#5345=FACE_OUTER_BOUND('',#6471,.T.);
#5346=FACE_OUTER_BOUND('',#6472,.T.);
#5347=FACE_OUTER_BOUND('',#6473,.T.);
#5348=FACE_OUTER_BOUND('',#6474,.T.);
#5349=FACE_OUTER_BOUND('',#6475,.T.);
#5350=FACE_OUTER_BOUND('',#6476,.T.);
#5351=FACE_OUTER_BOUND('',#6477,.T.);
#5352=FACE_OUTER_BOUND('',#6478,.T.);
#5353=FACE_OUTER_BOUND('',#6479,.T.);
#5354=FACE_OUTER_BOUND('',#6480,.T.);
#5355=FACE_OUTER_BOUND('',#6481,.T.);
#5356=FACE_OUTER_BOUND('',#6482,.T.);
#5357=FACE_OUTER_BOUND('',#6483,.T.);
#5358=FACE_OUTER_BOUND('',#6486,.T.);
#5359=FACE_OUTER_BOUND('',#6487,.T.);
#5360=FACE_OUTER_BOUND('',#6488,.T.);
#5361=FACE_OUTER_BOUND('',#6489,.T.);
#5362=FACE_OUTER_BOUND('',#6490,.T.);
#5363=FACE_OUTER_BOUND('',#6491,.T.);
#5364=FACE_OUTER_BOUND('',#6492,.T.);
#5365=FACE_OUTER_BOUND('',#6493,.T.);
#5366=FACE_OUTER_BOUND('',#6494,.T.);
#5367=FACE_OUTER_BOUND('',#6495,.T.);
#5368=FACE_OUTER_BOUND('',#6496,.T.);
#5369=FACE_OUTER_BOUND('',#6497,.T.);
#5370=FACE_OUTER_BOUND('',#6498,.T.);
#5371=FACE_OUTER_BOUND('',#6499,.T.);
#5372=FACE_OUTER_BOUND('',#6500,.T.);
#5373=FACE_OUTER_BOUND('',#6501,.T.);
#5374=FACE_OUTER_BOUND('',#6502,.T.);
#5375=FACE_OUTER_BOUND('',#6503,.T.);
#5376=FACE_OUTER_BOUND('',#6504,.T.);
#5377=FACE_OUTER_BOUND('',#6506,.T.);
#5378=FACE_OUTER_BOUND('',#6507,.T.);
#5379=FACE_OUTER_BOUND('',#6508,.T.);
#5380=FACE_OUTER_BOUND('',#6509,.T.);
#5381=FACE_OUTER_BOUND('',#6510,.T.);
#5382=FACE_OUTER_BOUND('',#6511,.T.);
#5383=FACE_OUTER_BOUND('',#6512,.T.);
#5384=FACE_OUTER_BOUND('',#6513,.T.);
#5385=FACE_OUTER_BOUND('',#6514,.T.);
#5386=FACE_OUTER_BOUND('',#6515,.T.);
#5387=FACE_OUTER_BOUND('',#6516,.T.);
#5388=FACE_OUTER_BOUND('',#6517,.T.);
#5389=FACE_OUTER_BOUND('',#6518,.T.);
#5390=FACE_OUTER_BOUND('',#6519,.T.);
#5391=FACE_OUTER_BOUND('',#6520,.T.);
#5392=FACE_OUTER_BOUND('',#6521,.T.);
#5393=FACE_OUTER_BOUND('',#6522,.T.);
#5394=FACE_OUTER_BOUND('',#6523,.T.);
#5395=FACE_OUTER_BOUND('',#6524,.T.);
#5396=FACE_OUTER_BOUND('',#6525,.T.);
#5397=FACE_OUTER_BOUND('',#6526,.T.);
#5398=FACE_OUTER_BOUND('',#6527,.T.);
#5399=FACE_OUTER_BOUND('',#6528,.T.);
#5400=FACE_OUTER_BOUND('',#6529,.T.);
#5401=FACE_OUTER_BOUND('',#6530,.T.);
#5402=FACE_OUTER_BOUND('',#6531,.T.);
#5403=FACE_OUTER_BOUND('',#6532,.T.);
#5404=FACE_OUTER_BOUND('',#6533,.T.);
#5405=FACE_OUTER_BOUND('',#6534,.T.);
#5406=FACE_OUTER_BOUND('',#6535,.T.);
#5407=FACE_OUTER_BOUND('',#6536,.T.);
#5408=FACE_OUTER_BOUND('',#6537,.T.);
#5409=FACE_OUTER_BOUND('',#6538,.T.);
#5410=FACE_OUTER_BOUND('',#6539,.T.);
#5411=FACE_OUTER_BOUND('',#6540,.T.);
#5412=FACE_OUTER_BOUND('',#6541,.T.);
#5413=FACE_OUTER_BOUND('',#6542,.T.);
#5414=FACE_OUTER_BOUND('',#6543,.T.);
#5415=FACE_OUTER_BOUND('',#6544,.T.);
#5416=FACE_OUTER_BOUND('',#6545,.T.);
#5417=FACE_OUTER_BOUND('',#6546,.T.);
#5418=FACE_OUTER_BOUND('',#6547,.T.);
#5419=FACE_OUTER_BOUND('',#6548,.T.);
#5420=FACE_OUTER_BOUND('',#6549,.T.);
#5421=FACE_OUTER_BOUND('',#6551,.T.);
#5422=FACE_OUTER_BOUND('',#6552,.T.);
#5423=FACE_OUTER_BOUND('',#6553,.T.);
#5424=FACE_OUTER_BOUND('',#6554,.T.);
#5425=FACE_OUTER_BOUND('',#6555,.T.);
#5426=FACE_OUTER_BOUND('',#6556,.T.);
#5427=FACE_OUTER_BOUND('',#6558,.T.);
#5428=FACE_OUTER_BOUND('',#6559,.T.);
#5429=FACE_OUTER_BOUND('',#6561,.T.);
#5430=FACE_OUTER_BOUND('',#6563,.T.);
#5431=FACE_OUTER_BOUND('',#6564,.T.);
#5432=FACE_OUTER_BOUND('',#6565,.T.);
#5433=FACE_OUTER_BOUND('',#6566,.T.);
#5434=FACE_OUTER_BOUND('',#6567,.T.);
#5435=FACE_OUTER_BOUND('',#6568,.T.);
#5436=FACE_OUTER_BOUND('',#6570,.T.);
#5437=FACE_OUTER_BOUND('',#6571,.T.);
#5438=FACE_OUTER_BOUND('',#6572,.T.);
#5439=FACE_OUTER_BOUND('',#6573,.T.);
#5440=FACE_OUTER_BOUND('',#6574,.T.);
#5441=FACE_OUTER_BOUND('',#6575,.T.);
#5442=FACE_OUTER_BOUND('',#6576,.T.);
#5443=FACE_OUTER_BOUND('',#6577,.T.);
#5444=FACE_OUTER_BOUND('',#6578,.T.);
#5445=FACE_OUTER_BOUND('',#6580,.T.);
#5446=FACE_OUTER_BOUND('',#6581,.T.);
#5447=FACE_OUTER_BOUND('',#6582,.T.);
#5448=FACE_OUTER_BOUND('',#6583,.T.);
#5449=FACE_OUTER_BOUND('',#6584,.T.);
#5450=FACE_OUTER_BOUND('',#6586,.T.);
#5451=FACE_OUTER_BOUND('',#6587,.T.);
#5452=FACE_OUTER_BOUND('',#6589,.T.);
#5453=FACE_OUTER_BOUND('',#6590,.T.);
#5454=FACE_OUTER_BOUND('',#6591,.T.);
#5455=FACE_OUTER_BOUND('',#6592,.T.);
#5456=FACE_OUTER_BOUND('',#6593,.T.);
#5457=FACE_OUTER_BOUND('',#6595,.T.);
#5458=FACE_OUTER_BOUND('',#6597,.T.);
#5459=FACE_OUTER_BOUND('',#6598,.T.);
#5460=FACE_OUTER_BOUND('',#6599,.T.);
#5461=FACE_OUTER_BOUND('',#6600,.T.);
#5462=FACE_OUTER_BOUND('',#6601,.T.);
#5463=FACE_OUTER_BOUND('',#6602,.T.);
#5464=FACE_OUTER_BOUND('',#6603,.T.);
#5465=FACE_OUTER_BOUND('',#6604,.T.);
#5466=FACE_OUTER_BOUND('',#6605,.T.);
#5467=FACE_OUTER_BOUND('',#6607,.T.);
#5468=FACE_OUTER_BOUND('',#6608,.T.);
#5469=FACE_OUTER_BOUND('',#6609,.T.);
#5470=FACE_OUTER_BOUND('',#6610,.T.);
#5471=FACE_OUTER_BOUND('',#6611,.T.);
#5472=FACE_OUTER_BOUND('',#6612,.T.);
#5473=FACE_OUTER_BOUND('',#6613,.T.);
#5474=FACE_OUTER_BOUND('',#6614,.T.);
#5475=FACE_OUTER_BOUND('',#6615,.T.);
#5476=FACE_OUTER_BOUND('',#6617,.T.);
#5477=FACE_OUTER_BOUND('',#6618,.T.);
#5478=FACE_OUTER_BOUND('',#6619,.T.);
#5479=FACE_OUTER_BOUND('',#6620,.T.);
#5480=FACE_OUTER_BOUND('',#6621,.T.);
#5481=FACE_OUTER_BOUND('',#6622,.T.);
#5482=FACE_OUTER_BOUND('',#6623,.T.);
#5483=FACE_OUTER_BOUND('',#6624,.T.);
#5484=FACE_OUTER_BOUND('',#6625,.T.);
#5485=FACE_OUTER_BOUND('',#6627,.T.);
#5486=FACE_OUTER_BOUND('',#6628,.T.);
#5487=FACE_OUTER_BOUND('',#6629,.T.);
#5488=FACE_OUTER_BOUND('',#6630,.T.);
#5489=FACE_OUTER_BOUND('',#6631,.T.);
#5490=FACE_OUTER_BOUND('',#6632,.T.);
#5491=FACE_OUTER_BOUND('',#6633,.T.);
#5492=FACE_OUTER_BOUND('',#6634,.T.);
#5493=FACE_OUTER_BOUND('',#6635,.T.);
#5494=FACE_OUTER_BOUND('',#6636,.T.);
#5495=FACE_OUTER_BOUND('',#6637,.T.);
#5496=FACE_OUTER_BOUND('',#6638,.T.);
#5497=FACE_OUTER_BOUND('',#6639,.T.);
#5498=FACE_OUTER_BOUND('',#6640,.T.);
#5499=FACE_OUTER_BOUND('',#6641,.T.);
#5500=FACE_OUTER_BOUND('',#6643,.T.);
#5501=FACE_OUTER_BOUND('',#6645,.T.);
#5502=FACE_OUTER_BOUND('',#6646,.T.);
#5503=FACE_OUTER_BOUND('',#6647,.T.);
#5504=FACE_OUTER_BOUND('',#6648,.T.);
#5505=FACE_OUTER_BOUND('',#6649,.T.);
#5506=FACE_OUTER_BOUND('',#6650,.T.);
#5507=FACE_OUTER_BOUND('',#6651,.T.);
#5508=FACE_OUTER_BOUND('',#6652,.T.);
#5509=FACE_OUTER_BOUND('',#6653,.T.);
#5510=FACE_OUTER_BOUND('',#6654,.T.);
#5511=FACE_OUTER_BOUND('',#6655,.T.);
#5512=FACE_OUTER_BOUND('',#6656,.T.);
#5513=FACE_OUTER_BOUND('',#6657,.T.);
#5514=FACE_OUTER_BOUND('',#6658,.T.);
#5515=FACE_OUTER_BOUND('',#6659,.T.);
#5516=FACE_OUTER_BOUND('',#6660,.T.);
#5517=FACE_OUTER_BOUND('',#6661,.T.);
#5518=FACE_OUTER_BOUND('',#6662,.T.);
#5519=FACE_OUTER_BOUND('',#6663,.T.);
#5520=FACE_OUTER_BOUND('',#6664,.T.);
#5521=FACE_OUTER_BOUND('',#6665,.T.);
#5522=FACE_OUTER_BOUND('',#6666,.T.);
#5523=FACE_OUTER_BOUND('',#6667,.T.);
#5524=FACE_OUTER_BOUND('',#6668,.T.);
#5525=FACE_OUTER_BOUND('',#6669,.T.);
#5526=FACE_OUTER_BOUND('',#6671,.T.);
#5527=FACE_OUTER_BOUND('',#6672,.T.);
#5528=FACE_OUTER_BOUND('',#6673,.T.);
#5529=FACE_OUTER_BOUND('',#6674,.T.);
#5530=FACE_OUTER_BOUND('',#6675,.T.);
#5531=FACE_OUTER_BOUND('',#6676,.T.);
#5532=FACE_OUTER_BOUND('',#6677,.T.);
#5533=FACE_OUTER_BOUND('',#6678,.T.);
#5534=FACE_OUTER_BOUND('',#6679,.T.);
#5535=FACE_OUTER_BOUND('',#6680,.T.);
#5536=FACE_OUTER_BOUND('',#6681,.T.);
#5537=FACE_OUTER_BOUND('',#6682,.T.);
#5538=FACE_OUTER_BOUND('',#6683,.T.);
#5539=FACE_OUTER_BOUND('',#6684,.T.);
#5540=FACE_OUTER_BOUND('',#6685,.T.);
#5541=FACE_OUTER_BOUND('',#6686,.T.);
#5542=FACE_OUTER_BOUND('',#6687,.T.);
#5543=FACE_OUTER_BOUND('',#6689,.T.);
#5544=FACE_OUTER_BOUND('',#6690,.T.);
#5545=FACE_OUTER_BOUND('',#6691,.T.);
#5546=FACE_OUTER_BOUND('',#6693,.T.);
#5547=FACE_OUTER_BOUND('',#6694,.T.);
#5548=FACE_OUTER_BOUND('',#6695,.T.);
#5549=FACE_OUTER_BOUND('',#6696,.T.);
#5550=FACE_OUTER_BOUND('',#6697,.T.);
#5551=FACE_OUTER_BOUND('',#6698,.T.);
#5552=FACE_OUTER_BOUND('',#6699,.T.);
#5553=FACE_OUTER_BOUND('',#6700,.T.);
#5554=FACE_OUTER_BOUND('',#6701,.T.);
#5555=FACE_OUTER_BOUND('',#6702,.T.);
#5556=FACE_OUTER_BOUND('',#6703,.T.);
#5557=FACE_OUTER_BOUND('',#6705,.T.);
#5558=FACE_OUTER_BOUND('',#6707,.T.);
#5559=FACE_OUTER_BOUND('',#6709,.T.);
#5560=FACE_OUTER_BOUND('',#6711,.T.);
#5561=FACE_OUTER_BOUND('',#6713,.T.);
#5562=FACE_OUTER_BOUND('',#6714,.T.);
#5563=FACE_OUTER_BOUND('',#6715,.T.);
#5564=FACE_OUTER_BOUND('',#6716,.T.);
#5565=FACE_OUTER_BOUND('',#6717,.T.);
#5566=FACE_OUTER_BOUND('',#6718,.T.);
#5567=FACE_OUTER_BOUND('',#6719,.T.);
#5568=FACE_OUTER_BOUND('',#6720,.T.);
#5569=FACE_OUTER_BOUND('',#6721,.T.);
#5570=FACE_OUTER_BOUND('',#6722,.T.);
#5571=FACE_OUTER_BOUND('',#6723,.T.);
#5572=FACE_OUTER_BOUND('',#6724,.T.);
#5573=FACE_OUTER_BOUND('',#6725,.T.);
#5574=FACE_OUTER_BOUND('',#6726,.T.);
#5575=FACE_OUTER_BOUND('',#6727,.T.);
#5576=FACE_OUTER_BOUND('',#6728,.T.);
#5577=FACE_OUTER_BOUND('',#6729,.T.);
#5578=FACE_OUTER_BOUND('',#6730,.T.);
#5579=FACE_OUTER_BOUND('',#6731,.T.);
#5580=FACE_OUTER_BOUND('',#6732,.T.);
#5581=FACE_OUTER_BOUND('',#6733,.T.);
#5582=FACE_OUTER_BOUND('',#6734,.T.);
#5583=FACE_OUTER_BOUND('',#6735,.T.);
#5584=FACE_OUTER_BOUND('',#6736,.T.);
#5585=FACE_OUTER_BOUND('',#6737,.T.);
#5586=FACE_OUTER_BOUND('',#6738,.T.);
#5587=FACE_OUTER_BOUND('',#6739,.T.);
#5588=FACE_OUTER_BOUND('',#6741,.T.);
#5589=FACE_OUTER_BOUND('',#6742,.T.);
#5590=FACE_OUTER_BOUND('',#6743,.T.);
#5591=FACE_OUTER_BOUND('',#6744,.T.);
#5592=FACE_OUTER_BOUND('',#6745,.T.);
#5593=FACE_OUTER_BOUND('',#6746,.T.);
#5594=FACE_OUTER_BOUND('',#6747,.T.);
#5595=FACE_OUTER_BOUND('',#6749,.T.);
#5596=FACE_OUTER_BOUND('',#6750,.T.);
#5597=FACE_OUTER_BOUND('',#6751,.T.);
#5598=FACE_OUTER_BOUND('',#6752,.T.);
#5599=FACE_OUTER_BOUND('',#6753,.T.);
#5600=FACE_OUTER_BOUND('',#6754,.T.);
#5601=FACE_OUTER_BOUND('',#6755,.T.);
#5602=FACE_OUTER_BOUND('',#6756,.T.);
#5603=FACE_OUTER_BOUND('',#6757,.T.);
#5604=FACE_OUTER_BOUND('',#6758,.T.);
#5605=FACE_OUTER_BOUND('',#6759,.T.);
#5606=FACE_OUTER_BOUND('',#6760,.T.);
#5607=FACE_OUTER_BOUND('',#6761,.T.);
#5608=FACE_OUTER_BOUND('',#6762,.T.);
#5609=FACE_OUTER_BOUND('',#6763,.T.);
#5610=FACE_OUTER_BOUND('',#6764,.T.);
#5611=FACE_OUTER_BOUND('',#6765,.T.);
#5612=FACE_OUTER_BOUND('',#6766,.T.);
#5613=FACE_OUTER_BOUND('',#6767,.T.);
#5614=FACE_OUTER_BOUND('',#6768,.T.);
#5615=FACE_OUTER_BOUND('',#6769,.T.);
#5616=FACE_OUTER_BOUND('',#6770,.T.);
#5617=FACE_OUTER_BOUND('',#6771,.T.);
#5618=FACE_OUTER_BOUND('',#6772,.T.);
#5619=FACE_OUTER_BOUND('',#6773,.T.);
#5620=FACE_OUTER_BOUND('',#6774,.T.);
#5621=FACE_OUTER_BOUND('',#6775,.T.);
#5622=FACE_OUTER_BOUND('',#6776,.T.);
#5623=FACE_OUTER_BOUND('',#6777,.T.);
#5624=FACE_OUTER_BOUND('',#6778,.T.);
#5625=FACE_OUTER_BOUND('',#6779,.T.);
#5626=FACE_OUTER_BOUND('',#6780,.T.);
#5627=FACE_OUTER_BOUND('',#6782,.T.);
#5628=FACE_OUTER_BOUND('',#6783,.T.);
#5629=FACE_OUTER_BOUND('',#6784,.T.);
#5630=FACE_OUTER_BOUND('',#6785,.T.);
#5631=FACE_OUTER_BOUND('',#6786,.T.);
#5632=FACE_OUTER_BOUND('',#6787,.T.);
#5633=FACE_OUTER_BOUND('',#6788,.T.);
#5634=FACE_OUTER_BOUND('',#6789,.T.);
#5635=FACE_OUTER_BOUND('',#6790,.T.);
#5636=FACE_OUTER_BOUND('',#6791,.T.);
#5637=FACE_OUTER_BOUND('',#6792,.T.);
#5638=FACE_OUTER_BOUND('',#6793,.T.);
#5639=FACE_OUTER_BOUND('',#6794,.T.);
#5640=FACE_OUTER_BOUND('',#6795,.T.);
#5641=FACE_OUTER_BOUND('',#6796,.T.);
#5642=FACE_OUTER_BOUND('',#6797,.T.);
#5643=FACE_OUTER_BOUND('',#6798,.T.);
#5644=FACE_OUTER_BOUND('',#6799,.T.);
#5645=FACE_OUTER_BOUND('',#6800,.T.);
#5646=FACE_OUTER_BOUND('',#6801,.T.);
#5647=FACE_OUTER_BOUND('',#6802,.T.);
#5648=FACE_OUTER_BOUND('',#6803,.T.);
#5649=FACE_OUTER_BOUND('',#6804,.T.);
#5650=FACE_OUTER_BOUND('',#6805,.T.);
#5651=FACE_OUTER_BOUND('',#6806,.T.);
#5652=FACE_OUTER_BOUND('',#6807,.T.);
#5653=FACE_OUTER_BOUND('',#6808,.T.);
#5654=FACE_OUTER_BOUND('',#6809,.T.);
#5655=FACE_OUTER_BOUND('',#6810,.T.);
#5656=FACE_OUTER_BOUND('',#6811,.T.);
#5657=FACE_OUTER_BOUND('',#6812,.T.);
#5658=FACE_OUTER_BOUND('',#6813,.T.);
#5659=FACE_OUTER_BOUND('',#6814,.T.);
#5660=FACE_OUTER_BOUND('',#6815,.T.);
#5661=FACE_OUTER_BOUND('',#6816,.T.);
#5662=FACE_OUTER_BOUND('',#6817,.T.);
#5663=FACE_OUTER_BOUND('',#6819,.T.);
#5664=FACE_OUTER_BOUND('',#6820,.T.);
#5665=FACE_OUTER_BOUND('',#6826,.T.);
#5666=FACE_OUTER_BOUND('',#6827,.T.);
#5667=FACE_OUTER_BOUND('',#6828,.T.);
#5668=FACE_OUTER_BOUND('',#6829,.T.);
#5669=FACE_OUTER_BOUND('',#6830,.T.);
#5670=FACE_OUTER_BOUND('',#6831,.T.);
#5671=FACE_OUTER_BOUND('',#6832,.T.);
#5672=FACE_OUTER_BOUND('',#6833,.T.);
#5673=FACE_OUTER_BOUND('',#6834,.T.);
#5674=FACE_OUTER_BOUND('',#6835,.T.);
#5675=FACE_OUTER_BOUND('',#6836,.T.);
#5676=FACE_OUTER_BOUND('',#6837,.T.);
#5677=FACE_OUTER_BOUND('',#6838,.T.);
#5678=FACE_OUTER_BOUND('',#6839,.T.);
#5679=FACE_OUTER_BOUND('',#6840,.T.);
#5680=FACE_OUTER_BOUND('',#6841,.T.);
#5681=FACE_OUTER_BOUND('',#6842,.T.);
#5682=FACE_OUTER_BOUND('',#6844,.T.);
#5683=FACE_OUTER_BOUND('',#6845,.T.);
#5684=FACE_OUTER_BOUND('',#6847,.T.);
#5685=FACE_OUTER_BOUND('',#6848,.T.);
#5686=FACE_OUTER_BOUND('',#6850,.T.);
#5687=FACE_OUTER_BOUND('',#6851,.T.);
#5688=FACE_OUTER_BOUND('',#6852,.T.);
#5689=FACE_OUTER_BOUND('',#6853,.T.);
#5690=FACE_OUTER_BOUND('',#6854,.T.);
#5691=FACE_OUTER_BOUND('',#6855,.T.);
#5692=FACE_OUTER_BOUND('',#6856,.T.);
#5693=FACE_OUTER_BOUND('',#6858,.T.);
#5694=FACE_OUTER_BOUND('',#6859,.T.);
#5695=FACE_OUTER_BOUND('',#6861,.T.);
#5696=FACE_OUTER_BOUND('',#6863,.T.);
#5697=FACE_OUTER_BOUND('',#6864,.T.);
#5698=FACE_OUTER_BOUND('',#6865,.T.);
#5699=FACE_OUTER_BOUND('',#6866,.T.);
#5700=FACE_OUTER_BOUND('',#6867,.T.);
#5701=FACE_OUTER_BOUND('',#6868,.T.);
#5702=FACE_OUTER_BOUND('',#6869,.T.);
#5703=FACE_OUTER_BOUND('',#6870,.T.);
#5704=FACE_OUTER_BOUND('',#6871,.T.);
#5705=FACE_OUTER_BOUND('',#6872,.T.);
#5706=FACE_OUTER_BOUND('',#6873,.T.);
#5707=FACE_OUTER_BOUND('',#6874,.T.);
#5708=FACE_OUTER_BOUND('',#6875,.T.);
#5709=FACE_OUTER_BOUND('',#6876,.T.);
#5710=FACE_OUTER_BOUND('',#6878,.T.);
#5711=FACE_OUTER_BOUND('',#6879,.T.);
#5712=FACE_OUTER_BOUND('',#6880,.T.);
#5713=FACE_OUTER_BOUND('',#6881,.T.);
#5714=FACE_OUTER_BOUND('',#6882,.T.);
#5715=FACE_OUTER_BOUND('',#6883,.T.);
#5716=FACE_OUTER_BOUND('',#6884,.T.);
#5717=FACE_OUTER_BOUND('',#6885,.T.);
#5718=FACE_OUTER_BOUND('',#6886,.T.);
#5719=FACE_OUTER_BOUND('',#6887,.T.);
#5720=FACE_OUTER_BOUND('',#6888,.T.);
#5721=FACE_OUTER_BOUND('',#6889,.T.);
#5722=FACE_OUTER_BOUND('',#6890,.T.);
#5723=FACE_OUTER_BOUND('',#6891,.T.);
#5724=FACE_OUTER_BOUND('',#6892,.T.);
#5725=FACE_OUTER_BOUND('',#6893,.T.);
#5726=FACE_OUTER_BOUND('',#6895,.T.);
#5727=FACE_OUTER_BOUND('',#6896,.T.);
#5728=FACE_OUTER_BOUND('',#6897,.T.);
#5729=FACE_OUTER_BOUND('',#6899,.T.);
#5730=FACE_OUTER_BOUND('',#6900,.T.);
#5731=FACE_OUTER_BOUND('',#6901,.T.);
#5732=FACE_OUTER_BOUND('',#6902,.T.);
#5733=FACE_OUTER_BOUND('',#6903,.T.);
#5734=FACE_OUTER_BOUND('',#6904,.T.);
#5735=FACE_OUTER_BOUND('',#6905,.T.);
#5736=FACE_OUTER_BOUND('',#6907,.T.);
#5737=FACE_OUTER_BOUND('',#6908,.T.);
#5738=FACE_OUTER_BOUND('',#6909,.T.);
#5739=FACE_OUTER_BOUND('',#6910,.T.);
#5740=FACE_OUTER_BOUND('',#6911,.T.);
#5741=FACE_OUTER_BOUND('',#6912,.T.);
#5742=FACE_OUTER_BOUND('',#6913,.T.);
#5743=FACE_OUTER_BOUND('',#6914,.T.);
#5744=FACE_OUTER_BOUND('',#6915,.T.);
#5745=FACE_OUTER_BOUND('',#6916,.T.);
#5746=FACE_OUTER_BOUND('',#6917,.T.);
#5747=FACE_OUTER_BOUND('',#6918,.T.);
#5748=FACE_OUTER_BOUND('',#6919,.T.);
#5749=FACE_OUTER_BOUND('',#6920,.T.);
#5750=FACE_OUTER_BOUND('',#6921,.T.);
#5751=FACE_OUTER_BOUND('',#6922,.T.);
#5752=FACE_OUTER_BOUND('',#6923,.T.);
#5753=FACE_OUTER_BOUND('',#6924,.T.);
#5754=FACE_OUTER_BOUND('',#6925,.T.);
#5755=FACE_OUTER_BOUND('',#6926,.T.);
#5756=FACE_OUTER_BOUND('',#6927,.T.);
#5757=FACE_OUTER_BOUND('',#6928,.T.);
#5758=FACE_OUTER_BOUND('',#6929,.T.);
#5759=FACE_OUTER_BOUND('',#6931,.T.);
#5760=FACE_OUTER_BOUND('',#6932,.T.);
#5761=FACE_OUTER_BOUND('',#6933,.T.);
#5762=FACE_OUTER_BOUND('',#6934,.T.);
#5763=FACE_OUTER_BOUND('',#6935,.T.);
#5764=FACE_OUTER_BOUND('',#6936,.T.);
#5765=FACE_OUTER_BOUND('',#6937,.T.);
#5766=FACE_OUTER_BOUND('',#6939,.T.);
#5767=FACE_OUTER_BOUND('',#6940,.T.);
#5768=FACE_OUTER_BOUND('',#6941,.T.);
#5769=FACE_OUTER_BOUND('',#6942,.T.);
#5770=FACE_OUTER_BOUND('',#6944,.T.);
#5771=FACE_OUTER_BOUND('',#6945,.T.);
#5772=FACE_OUTER_BOUND('',#6946,.T.);
#5773=FACE_OUTER_BOUND('',#6947,.T.);
#5774=FACE_OUTER_BOUND('',#6948,.T.);
#5775=FACE_OUTER_BOUND('',#6950,.T.);
#5776=FACE_OUTER_BOUND('',#6951,.T.);
#5777=FACE_OUTER_BOUND('',#6952,.T.);
#5778=FACE_OUTER_BOUND('',#6955,.T.);
#5779=FACE_OUTER_BOUND('',#6956,.T.);
#5780=FACE_OUTER_BOUND('',#6957,.T.);
#5781=FACE_OUTER_BOUND('',#6958,.T.);
#5782=FACE_OUTER_BOUND('',#6959,.T.);
#5783=FACE_OUTER_BOUND('',#6960,.T.);
#5784=FACE_OUTER_BOUND('',#6961,.T.);
#5785=FACE_OUTER_BOUND('',#6962,.T.);
#5786=FACE_OUTER_BOUND('',#6963,.T.);
#5787=FACE_OUTER_BOUND('',#6964,.T.);
#5788=FACE_OUTER_BOUND('',#6965,.T.);
#5789=FACE_OUTER_BOUND('',#6966,.T.);
#6189=EDGE_LOOP('',(#13370,#13371,#13372,#13373,#13374));
#6190=EDGE_LOOP('',(#13375,#13376,#13377,#13378,#13379,#13380));
#6191=EDGE_LOOP('',(#13381,#13382,#13383,#13384,#13385,#13386));
#6192=EDGE_LOOP('',(#13387,#13388,#13389,#13390,#13391,#13392));
#6193=EDGE_LOOP('',(#13393,#13394,#13395,#13396));
#6194=EDGE_LOOP('',(#13397,#13398,#13399,#13400,#13401,#13402));
#6195=EDGE_LOOP('',(#13403,#13404,#13405,#13406,#13407));
#6196=EDGE_LOOP('',(#13408,#13409,#13410,#13411,#13412,#13413));
#6197=EDGE_LOOP('',(#13414,#13415,#13416,#13417,#13418,#13419));
#6198=EDGE_LOOP('',(#13420));
#6199=EDGE_LOOP('',(#13421));
#6200=EDGE_LOOP('',(#13422));
#6201=EDGE_LOOP('',(#13423));
#6202=EDGE_LOOP('',(#13424,#13425,#13426,#13427,#13428));
#6203=EDGE_LOOP('',(#13429,#13430,#13431,#13432,#13433));
#6204=EDGE_LOOP('',(#13434));
#6205=EDGE_LOOP('',(#13435));
#6206=EDGE_LOOP('',(#13436,#13437,#13438));
#6207=EDGE_LOOP('',(#13439));
#6208=EDGE_LOOP('',(#13440,#13441,#13442,#13443,#13444,#13445));
#6209=EDGE_LOOP('',(#13446,#13447,#13448,#13449));
#6210=EDGE_LOOP('',(#13450,#13451,#13452,#13453));
#6211=EDGE_LOOP('',(#13454,#13455,#13456,#13457,#13458));
#6212=EDGE_LOOP('',(#13459,#13460,#13461,#13462));
#6213=EDGE_LOOP('',(#13463,#13464,#13465,#13466));
#6214=EDGE_LOOP('',(#13467,#13468,#13469,#13470,#13471));
#6215=EDGE_LOOP('',(#13472,#13473,#13474,#13475,#13476));
#6216=EDGE_LOOP('',(#13477,#13478,#13479,#13480,#13481));
#6217=EDGE_LOOP('',(#13482,#13483,#13484,#13485,#13486));
#6218=EDGE_LOOP('',(#13487,#13488,#13489,#13490,#13491,#13492));
#6219=EDGE_LOOP('',(#13493,#13494,#13495,#13496,#13497));
#6220=EDGE_LOOP('',(#13498,#13499,#13500,#13501));
#6221=EDGE_LOOP('',(#13502,#13503,#13504,#13505));
#6222=EDGE_LOOP('',(#13506,#13507,#13508,#13509));
#6223=EDGE_LOOP('',(#13510,#13511,#13512,#13513));
#6224=EDGE_LOOP('',(#13514,#13515,#13516,#13517,#13518,#13519));
#6225=EDGE_LOOP('',(#13520,#13521,#13522,#13523));
#6226=EDGE_LOOP('',(#13524,#13525,#13526,#13527,#13528,#13529,#13530,#13531));
#6227=EDGE_LOOP('',(#13532,#13533,#13534,#13535));
#6228=EDGE_LOOP('',(#13536,#13537,#13538,#13539));
#6229=EDGE_LOOP('',(#13540,#13541,#13542,#13543,#13544,#13545,#13546,#13547,
#13548,#13549));
#6230=EDGE_LOOP('',(#13550,#13551,#13552,#13553,#13554,#13555,#13556,#13557));
#6231=EDGE_LOOP('',(#13558,#13559,#13560,#13561));
#6232=EDGE_LOOP('',(#13562,#13563,#13564,#13565));
#6233=EDGE_LOOP('',(#13566,#13567,#13568,#13569));
#6234=EDGE_LOOP('',(#13570,#13571,#13572,#13573));
#6235=EDGE_LOOP('',(#13574,#13575,#13576,#13577,#13578,#13579,#13580,#13581));
#6236=EDGE_LOOP('',(#13582,#13583,#13584,#13585));
#6237=EDGE_LOOP('',(#13586,#13587,#13588,#13589));
#6238=EDGE_LOOP('',(#13590,#13591,#13592,#13593,#13594));
#6239=EDGE_LOOP('',(#13595,#13596,#13597,#13598));
#6240=EDGE_LOOP('',(#13599,#13600,#13601,#13602));
#6241=EDGE_LOOP('',(#13603,#13604,#13605,#13606));
#6242=EDGE_LOOP('',(#13607,#13608,#13609,#13610));
#6243=EDGE_LOOP('',(#13611,#13612,#13613,#13614));
#6244=EDGE_LOOP('',(#13615,#13616,#13617,#13618));
#6245=EDGE_LOOP('',(#13619,#13620,#13621,#13622,#13623,#13624));
#6246=EDGE_LOOP('',(#13625,#13626,#13627,#13628,#13629,#13630));
#6247=EDGE_LOOP('',(#13631,#13632,#13633,#13634,#13635,#13636,#13637,#13638,
#13639,#13640,#13641,#13642,#13643,#13644,#13645,#13646,#13647,#13648,#13649,
#13650,#13651,#13652,#13653,#13654));
#6248=EDGE_LOOP('',(#13655,#13656));
#6249=EDGE_LOOP('',(#13657,#13658,#13659,#13660,#13661,#13662,#13663,#13664));
#6250=EDGE_LOOP('',(#13665,#13666,#13667,#13668));
#6251=EDGE_LOOP('',(#13669,#13670,#13671,#13672,#13673,#13674,#13675,#13676));
#6252=EDGE_LOOP('',(#13677,#13678,#13679,#13680,#13681,#13682));
#6253=EDGE_LOOP('',(#13683,#13684,#13685,#13686));
#6254=EDGE_LOOP('',(#13687,#13688,#13689,#13690));
#6255=EDGE_LOOP('',(#13691,#13692,#13693,#13694));
#6256=EDGE_LOOP('',(#13695,#13696,#13697,#13698));
#6257=EDGE_LOOP('',(#13699,#13700,#13701,#13702,#13703,#13704,#13705,#13706,
#13707,#13708,#13709,#13710));
#6258=EDGE_LOOP('',(#13711,#13712,#13713,#13714));
#6259=EDGE_LOOP('',(#13715,#13716,#13717,#13718));
#6260=EDGE_LOOP('',(#13719,#13720,#13721,#13722));
#6261=EDGE_LOOP('',(#13723,#13724,#13725,#13726));
#6262=EDGE_LOOP('',(#13727,#13728,#13729,#13730));
#6263=EDGE_LOOP('',(#13731,#13732,#13733,#13734));
#6264=EDGE_LOOP('',(#13735,#13736,#13737,#13738));
#6265=EDGE_LOOP('',(#13739,#13740,#13741,#13742));
#6266=EDGE_LOOP('',(#13743,#13744,#13745,#13746));
#6267=EDGE_LOOP('',(#13747,#13748,#13749,#13750));
#6268=EDGE_LOOP('',(#13751,#13752,#13753,#13754,#13755,#13756));
#6269=EDGE_LOOP('',(#13757,#13758,#13759,#13760));
#6270=EDGE_LOOP('',(#13761,#13762,#13763,#13764,#13765,#13766));
#6271=EDGE_LOOP('',(#13767,#13768,#13769,#13770,#13771,#13772));
#6272=EDGE_LOOP('',(#13773,#13774,#13775,#13776,#13777,#13778,#13779,#13780,
#13781,#13782,#13783,#13784,#13785,#13786,#13787,#13788,#13789,#13790,#13791,
#13792));
#6273=EDGE_LOOP('',(#13793,#13794,#13795,#13796));
#6274=EDGE_LOOP('',(#13797,#13798,#13799,#13800));
#6275=EDGE_LOOP('',(#13801,#13802,#13803,#13804,#13805));
#6276=EDGE_LOOP('',(#13806,#13807,#13808,#13809,#13810));
#6277=EDGE_LOOP('',(#13811,#13812,#13813,#13814));
#6278=EDGE_LOOP('',(#13815,#13816,#13817,#13818));
#6279=EDGE_LOOP('',(#13819,#13820));
#6280=EDGE_LOOP('',(#13821,#13822));
#6281=EDGE_LOOP('',(#13823,#13824,#13825,#13826,#13827));
#6282=EDGE_LOOP('',(#13828,#13829));
#6283=EDGE_LOOP('',(#13830,#13831,#13832,#13833,#13834,#13835,#13836,#13837));
#6284=EDGE_LOOP('',(#13838,#13839));
#6285=EDGE_LOOP('',(#13840,#13841,#13842,#13843,#13844));
#6286=EDGE_LOOP('',(#13845,#13846));
#6287=EDGE_LOOP('',(#13847,#13848,#13849,#13850,#13851));
#6288=EDGE_LOOP('',(#13852,#13853));
#6289=EDGE_LOOP('',(#13854,#13855));
#6290=EDGE_LOOP('',(#13856,#13857,#13858,#13859,#13860,#13861));
#6291=EDGE_LOOP('',(#13862,#13863,#13864,#13865,#13866,#13867));
#6292=EDGE_LOOP('',(#13868,#13869,#13870,#13871,#13872,#13873));
#6293=EDGE_LOOP('',(#13874,#13875,#13876,#13877,#13878,#13879));
#6294=EDGE_LOOP('',(#13880,#13881,#13882,#13883,#13884,#13885,#13886,#13887,
#13888,#13889,#13890,#13891,#13892,#13893,#13894,#13895));
#6295=EDGE_LOOP('',(#13896,#13897,#13898,#13899,#13900,#13901));
#6296=EDGE_LOOP('',(#13902,#13903,#13904,#13905,#13906,#13907));
#6297=EDGE_LOOP('',(#13908,#13909,#13910,#13911));
#6298=EDGE_LOOP('',(#13912,#13913,#13914,#13915));
#6299=EDGE_LOOP('',(#13916,#13917,#13918,#13919));
#6300=EDGE_LOOP('',(#13920,#13921,#13922,#13923));
#6301=EDGE_LOOP('',(#13924,#13925,#13926,#13927));
#6302=EDGE_LOOP('',(#13928,#13929,#13930,#13931));
#6303=EDGE_LOOP('',(#13932,#13933,#13934,#13935,#13936));
#6304=EDGE_LOOP('',(#13937,#13938,#13939,#13940));
#6305=EDGE_LOOP('',(#13941,#13942,#13943,#13944,#13945));
#6306=EDGE_LOOP('',(#13946,#13947,#13948,#13949));
#6307=EDGE_LOOP('',(#13950,#13951,#13952,#13953));
#6308=EDGE_LOOP('',(#13954,#13955,#13956,#13957));
#6309=EDGE_LOOP('',(#13958,#13959,#13960,#13961));
#6310=EDGE_LOOP('',(#13962,#13963,#13964,#13965));
#6311=EDGE_LOOP('',(#13966,#13967,#13968,#13969));
#6312=EDGE_LOOP('',(#13970,#13971,#13972,#13973,#13974));
#6313=EDGE_LOOP('',(#13975,#13976,#13977,#13978));
#6314=EDGE_LOOP('',(#13979,#13980,#13981,#13982,#13983));
#6315=EDGE_LOOP('',(#13984,#13985,#13986,#13987));
#6316=EDGE_LOOP('',(#13988,#13989,#13990,#13991));
#6317=EDGE_LOOP('',(#13992,#13993,#13994,#13995));
#6318=EDGE_LOOP('',(#13996,#13997,#13998,#13999));
#6319=EDGE_LOOP('',(#14000,#14001,#14002,#14003));
#6320=EDGE_LOOP('',(#14004,#14005,#14006,#14007));
#6321=EDGE_LOOP('',(#14008,#14009,#14010,#14011,#14012));
#6322=EDGE_LOOP('',(#14013,#14014,#14015,#14016));
#6323=EDGE_LOOP('',(#14017,#14018,#14019,#14020,#14021));
#6324=EDGE_LOOP('',(#14022,#14023,#14024,#14025,#14026,#14027,#14028,#14029,
#14030,#14031,#14032,#14033,#14034,#14035,#14036,#14037));
#6325=EDGE_LOOP('',(#14038,#14039,#14040,#14041));
#6326=EDGE_LOOP('',(#14042,#14043,#14044,#14045));
#6327=EDGE_LOOP('',(#14046,#14047,#14048,#14049));
#6328=EDGE_LOOP('',(#14050,#14051,#14052,#14053));
#6329=EDGE_LOOP('',(#14054,#14055,#14056,#14057));
#6330=EDGE_LOOP('',(#14058,#14059,#14060,#14061));
#6331=EDGE_LOOP('',(#14062,#14063,#14064,#14065,#14066));
#6332=EDGE_LOOP('',(#14067,#14068,#14069,#14070));
#6333=EDGE_LOOP('',(#14071,#14072,#14073,#14074,#14075));
#6334=EDGE_LOOP('',(#14076,#14077,#14078,#14079));
#6335=EDGE_LOOP('',(#14080,#14081,#14082,#14083));
#6336=EDGE_LOOP('',(#14084,#14085,#14086,#14087));
#6337=EDGE_LOOP('',(#14088,#14089,#14090,#14091));
#6338=EDGE_LOOP('',(#14092,#14093,#14094,#14095));
#6339=EDGE_LOOP('',(#14096,#14097,#14098,#14099));
#6340=EDGE_LOOP('',(#14100,#14101,#14102,#14103));
#6341=EDGE_LOOP('',(#14104,#14105,#14106,#14107));
#6342=EDGE_LOOP('',(#14108,#14109,#14110,#14111));
#6343=EDGE_LOOP('',(#14112,#14113,#14114,#14115));
#6344=EDGE_LOOP('',(#14116,#14117,#14118,#14119));
#6345=EDGE_LOOP('',(#14120,#14121,#14122,#14123));
#6346=EDGE_LOOP('',(#14124,#14125,#14126,#14127));
#6347=EDGE_LOOP('',(#14128,#14129,#14130,#14131));
#6348=EDGE_LOOP('',(#14132,#14133,#14134,#14135));
#6349=EDGE_LOOP('',(#14136,#14137,#14138,#14139));
#6350=EDGE_LOOP('',(#14140,#14141,#14142,#14143));
#6351=EDGE_LOOP('',(#14144,#14145,#14146,#14147));
#6352=EDGE_LOOP('',(#14148,#14149,#14150,#14151));
#6353=EDGE_LOOP('',(#14152,#14153,#14154,#14155));
#6354=EDGE_LOOP('',(#14156,#14157,#14158,#14159));
#6355=EDGE_LOOP('',(#14160,#14161,#14162,#14163));
#6356=EDGE_LOOP('',(#14164,#14165,#14166,#14167));
#6357=EDGE_LOOP('',(#14168,#14169,#14170,#14171));
#6358=EDGE_LOOP('',(#14172,#14173,#14174,#14175));
#6359=EDGE_LOOP('',(#14176,#14177,#14178,#14179));
#6360=EDGE_LOOP('',(#14180,#14181,#14182,#14183));
#6361=EDGE_LOOP('',(#14184,#14185,#14186,#14187));
#6362=EDGE_LOOP('',(#14188,#14189,#14190,#14191));
#6363=EDGE_LOOP('',(#14192,#14193,#14194,#14195,#14196,#14197));
#6364=EDGE_LOOP('',(#14198,#14199,#14200,#14201,#14202,#14203));
#6365=EDGE_LOOP('',(#14204,#14205,#14206,#14207));
#6366=EDGE_LOOP('',(#14208,#14209,#14210,#14211,#14212,#14213));
#6367=EDGE_LOOP('',(#14214,#14215,#14216,#14217,#14218,#14219));
#6368=EDGE_LOOP('',(#14220,#14221,#14222,#14223,#14224,#14225));
#6369=EDGE_LOOP('',(#14226,#14227,#14228,#14229,#14230,#14231));
#6370=EDGE_LOOP('',(#14232,#14233,#14234,#14235));
#6371=EDGE_LOOP('',(#14236,#14237,#14238,#14239,#14240,#14241));
#6372=EDGE_LOOP('',(#14242,#14243,#14244,#14245,#14246,#14247));
#6373=EDGE_LOOP('',(#14248,#14249,#14250,#14251));
#6374=EDGE_LOOP('',(#14252,#14253,#14254,#14255));
#6375=EDGE_LOOP('',(#14256,#14257,#14258,#14259));
#6376=EDGE_LOOP('',(#14260,#14261,#14262,#14263));
#6377=EDGE_LOOP('',(#14264,#14265,#14266,#14267));
#6378=EDGE_LOOP('',(#14268,#14269,#14270,#14271));
#6379=EDGE_LOOP('',(#14272,#14273,#14274,#14275));
#6380=EDGE_LOOP('',(#14276,#14277,#14278,#14279));
#6381=EDGE_LOOP('',(#14280,#14281,#14282,#14283));
#6382=EDGE_LOOP('',(#14284,#14285,#14286,#14287));
#6383=EDGE_LOOP('',(#14288,#14289,#14290,#14291));
#6384=EDGE_LOOP('',(#14292,#14293,#14294,#14295));
#6385=EDGE_LOOP('',(#14296,#14297,#14298,#14299,#14300,#14301,#14302,#14303,
#14304,#14305,#14306,#14307,#14308,#14309,#14310,#14311,#14312,#14313,#14314,
#14315,#14316,#14317,#14318,#14319,#14320,#14321,#14322,#14323,#14324,#14325,
#14326,#14327,#14328,#14329,#14330,#14331,#14332,#14333,#14334,#14335,#14336,
#14337,#14338,#14339,#14340,#14341,#14342,#14343,#14344,#14345,#14346,#14347,
#14348,#14349,#14350,#14351));
#6386=EDGE_LOOP('',(#14352,#14353,#14354,#14355,#14356,#14357,#14358,#14359,
#14360,#14361,#14362,#14363,#14364,#14365,#14366,#14367));
#6387=EDGE_LOOP('',(#14368));
#6388=EDGE_LOOP('',(#14369));
#6389=EDGE_LOOP('',(#14370));
#6390=EDGE_LOOP('',(#14371,#14372,#14373,#14374,#14375,#14376));
#6391=EDGE_LOOP('',(#14377));
#6392=EDGE_LOOP('',(#14378,#14379,#14380,#14381,#14382,#14383));
#6393=EDGE_LOOP('',(#14384,#14385,#14386,#14387));
#6394=EDGE_LOOP('',(#14388,#14389,#14390,#14391,#14392,#14393,#14394,#14395));
#6395=EDGE_LOOP('',(#14396,#14397,#14398,#14399));
#6396=EDGE_LOOP('',(#14400,#14401,#14402,#14403,#14404,#14405,#14406,#14407));
#6397=EDGE_LOOP('',(#14408,#14409,#14410,#14411));
#6398=EDGE_LOOP('',(#14412,#14413,#14414,#14415,#14416,#14417,#14418,#14419));
#6399=EDGE_LOOP('',(#14420,#14421,#14422,#14423));
#6400=EDGE_LOOP('',(#14424,#14425,#14426,#14427,#14428,#14429,#14430,#14431));
#6401=EDGE_LOOP('',(#14432,#14433,#14434,#14435,#14436));
#6402=EDGE_LOOP('',(#14437,#14438,#14439,#14440,#14441,#14442));
#6403=EDGE_LOOP('',(#14443,#14444,#14445,#14446,#14447));
#6404=EDGE_LOOP('',(#14448,#14449,#14450,#14451));
#6405=EDGE_LOOP('',(#14452,#14453));
#6406=EDGE_LOOP('',(#14454,#14455,#14456,#14457,#14458,#14459));
#6407=EDGE_LOOP('',(#14460,#14461,#14462,#14463));
#6408=EDGE_LOOP('',(#14464,#14465));
#6409=EDGE_LOOP('',(#14466,#14467,#14468,#14469,#14470,#14471));
#6410=EDGE_LOOP('',(#14472,#14473,#14474,#14475));
#6411=EDGE_LOOP('',(#14476,#14477));
#6412=EDGE_LOOP('',(#14478,#14479,#14480,#14481,#14482,#14483));
#6413=EDGE_LOOP('',(#14484,#14485,#14486,#14487));
#6414=EDGE_LOOP('',(#14488,#14489));
#6415=EDGE_LOOP('',(#14490,#14491,#14492,#14493,#14494,#14495));
#6416=EDGE_LOOP('',(#14496,#14497,#14498,#14499));
#6417=EDGE_LOOP('',(#14500,#14501));
#6418=EDGE_LOOP('',(#14502,#14503,#14504,#14505,#14506,#14507));
#6419=EDGE_LOOP('',(#14508,#14509));
#6420=EDGE_LOOP('',(#14510,#14511));
#6421=EDGE_LOOP('',(#14512,#14513,#14514,#14515,#14516,#14517));
#6422=EDGE_LOOP('',(#14518,#14519,#14520,#14521,#14522,#14523));
#6423=EDGE_LOOP('',(#14524,#14525));
#6424=EDGE_LOOP('',(#14526,#14527));
#6425=EDGE_LOOP('',(#14528,#14529,#14530,#14531));
#6426=EDGE_LOOP('',(#14532,#14533));
#6427=EDGE_LOOP('',(#14534,#14535,#14536,#14537,#14538,#14539));
#6428=EDGE_LOOP('',(#14540,#14541,#14542,#14543));
#6429=EDGE_LOOP('',(#14544,#14545));
#6430=EDGE_LOOP('',(#14546,#14547,#14548,#14549,#14550,#14551));
#6431=EDGE_LOOP('',(#14552,#14553,#14554,#14555));
#6432=EDGE_LOOP('',(#14556,#14557,#14558,#14559,#14560,#14561,#14562,#14563));
#6433=EDGE_LOOP('',(#14564,#14565));
#6434=EDGE_LOOP('',(#14566,#14567));
#6435=EDGE_LOOP('',(#14568,#14569));
#6436=EDGE_LOOP('',(#14570,#14571,#14572,#14573));
#6437=EDGE_LOOP('',(#14574,#14575));
#6438=EDGE_LOOP('',(#14576,#14577,#14578,#14579,#14580,#14581));
#6439=EDGE_LOOP('',(#14582,#14583,#14584,#14585));
#6440=EDGE_LOOP('',(#14586,#14587));
#6441=EDGE_LOOP('',(#14588,#14589,#14590,#14591,#14592,#14593));
#6442=EDGE_LOOP('',(#14594,#14595,#14596,#14597));
#6443=EDGE_LOOP('',(#14598,#14599));
#6444=EDGE_LOOP('',(#14600,#14601,#14602,#14603,#14604,#14605));
#6445=EDGE_LOOP('',(#14606,#14607,#14608,#14609));
#6446=EDGE_LOOP('',(#14610,#14611));
#6447=EDGE_LOOP('',(#14612,#14613,#14614,#14615,#14616,#14617));
#6448=EDGE_LOOP('',(#14618,#14619,#14620,#14621));
#6449=EDGE_LOOP('',(#14622,#14623,#14624,#14625,#14626));
#6450=EDGE_LOOP('',(#14627,#14628,#14629,#14630,#14631,#14632));
#6451=EDGE_LOOP('',(#14633,#14634,#14635,#14636,#14637,#14638));
#6452=EDGE_LOOP('',(#14639,#14640));
#6453=EDGE_LOOP('',(#14641,#14642,#14643,#14644));
#6454=EDGE_LOOP('',(#14645,#14646,#14647,#14648));
#6455=EDGE_LOOP('',(#14649,#14650));
#6456=EDGE_LOOP('',(#14651,#14652,#14653,#14654,#14655,#14656));
#6457=EDGE_LOOP('',(#14657,#14658,#14659,#14660));
#6458=EDGE_LOOP('',(#14661,#14662));
#6459=EDGE_LOOP('',(#14663,#14664,#14665,#14666,#14667,#14668));
#6460=EDGE_LOOP('',(#14669,#14670,#14671,#14672));
#6461=EDGE_LOOP('',(#14673,#14674));
#6462=EDGE_LOOP('',(#14675,#14676,#14677,#14678,#14679,#14680));
#6463=EDGE_LOOP('',(#14681,#14682,#14683,#14684));
#6464=EDGE_LOOP('',(#14685,#14686,#14687,#14688,#14689,#14690));
#6465=EDGE_LOOP('',(#14691,#14692,#14693,#14694,#14695,#14696,#14697,#14698));
#6466=EDGE_LOOP('',(#14699,#14700,#14701,#14702,#14703,#14704,#14705,#14706));
#6467=EDGE_LOOP('',(#14707,#14708,#14709,#14710));
#6468=EDGE_LOOP('',(#14711,#14712,#14713,#14714));
#6469=EDGE_LOOP('',(#14715,#14716,#14717,#14718));
#6470=EDGE_LOOP('',(#14719,#14720,#14721,#14722,#14723,#14724,#14725,#14726,
#14727,#14728,#14729,#14730,#14731,#14732,#14733,#14734,#14735,#14736,#14737,
#14738));
#6471=EDGE_LOOP('',(#14739,#14740,#14741,#14742));
#6472=EDGE_LOOP('',(#14743,#14744,#14745,#14746));
#6473=EDGE_LOOP('',(#14747,#14748,#14749,#14750));
#6474=EDGE_LOOP('',(#14751,#14752,#14753,#14754));
#6475=EDGE_LOOP('',(#14755,#14756,#14757,#14758));
#6476=EDGE_LOOP('',(#14759,#14760,#14761,#14762));
#6477=EDGE_LOOP('',(#14763,#14764,#14765,#14766,#14767,#14768,#14769,#14770,
#14771,#14772,#14773,#14774,#14775,#14776,#14777,#14778,#14779,#14780,#14781,
#14782));
#6478=EDGE_LOOP('',(#14783,#14784,#14785,#14786));
#6479=EDGE_LOOP('',(#14787,#14788,#14789,#14790));
#6480=EDGE_LOOP('',(#14791,#14792,#14793,#14794,#14795));
#6481=EDGE_LOOP('',(#14796,#14797,#14798,#14799,#14800,#14801,#14802,#14803,
#14804,#14805,#14806,#14807,#14808,#14809,#14810,#14811,#14812,#14813,#14814,
#14815));
#6482=EDGE_LOOP('',(#14816,#14817,#14818,#14819));
#6483=EDGE_LOOP('',(#14820,#14821,#14822,#14823));
#6484=EDGE_LOOP('',(#14824));
#6485=EDGE_LOOP('',(#14825));
#6486=EDGE_LOOP('',(#14826,#14827,#14828,#14829,#14830,#14831));
#6487=EDGE_LOOP('',(#14832,#14833,#14834,#14835));
#6488=EDGE_LOOP('',(#14836,#14837,#14838,#14839,#14840,#14841));
#6489=EDGE_LOOP('',(#14842,#14843,#14844,#14845,#14846,#14847));
#6490=EDGE_LOOP('',(#14848,#14849,#14850,#14851,#14852,#14853));
#6491=EDGE_LOOP('',(#14854,#14855,#14856,#14857));
#6492=EDGE_LOOP('',(#14858,#14859,#14860,#14861));
#6493=EDGE_LOOP('',(#14862,#14863,#14864,#14865));
#6494=EDGE_LOOP('',(#14866,#14867,#14868,#14869));
#6495=EDGE_LOOP('',(#14870,#14871,#14872,#14873));
#6496=EDGE_LOOP('',(#14874,#14875,#14876,#14877));
#6497=EDGE_LOOP('',(#14878,#14879,#14880,#14881));
#6498=EDGE_LOOP('',(#14882,#14883,#14884,#14885));
#6499=EDGE_LOOP('',(#14886,#14887,#14888,#14889));
#6500=EDGE_LOOP('',(#14890,#14891,#14892,#14893));
#6501=EDGE_LOOP('',(#14894,#14895,#14896,#14897));
#6502=EDGE_LOOP('',(#14898,#14899,#14900,#14901));
#6503=EDGE_LOOP('',(#14902,#14903,#14904,#14905));
#6504=EDGE_LOOP('',(#14906,#14907,#14908,#14909,#14910,#14911,#14912,#14913,
#14914,#14915,#14916,#14917,#14918,#14919,#14920,#14921,#14922,#14923,#14924,
#14925,#14926,#14927,#14928,#14929));
#6505=EDGE_LOOP('',(#14930,#14931,#14932,#14933,#14934,#14935,#14936,#14937,
#14938,#14939,#14940,#14941,#14942,#14943,#14944,#14945));
#6506=EDGE_LOOP('',(#14946,#14947,#14948,#14949,#14950,#14951));
#6507=EDGE_LOOP('',(#14952,#14953,#14954,#14955,#14956,#14957));
#6508=EDGE_LOOP('',(#14958,#14959,#14960,#14961));
#6509=EDGE_LOOP('',(#14962,#14963,#14964,#14965));
#6510=EDGE_LOOP('',(#14966,#14967,#14968,#14969));
#6511=EDGE_LOOP('',(#14970,#14971,#14972,#14973));
#6512=EDGE_LOOP('',(#14974,#14975,#14976,#14977));
#6513=EDGE_LOOP('',(#14978,#14979,#14980,#14981));
#6514=EDGE_LOOP('',(#14982,#14983,#14984,#14985,#14986,#14987));
#6515=EDGE_LOOP('',(#14988,#14989,#14990,#14991));
#6516=EDGE_LOOP('',(#14992,#14993,#14994,#14995));
#6517=EDGE_LOOP('',(#14996,#14997,#14998,#14999));
#6518=EDGE_LOOP('',(#15000,#15001,#15002,#15003));
#6519=EDGE_LOOP('',(#15004,#15005,#15006,#15007));
#6520=EDGE_LOOP('',(#15008,#15009,#15010,#15011,#15012,#15013));
#6521=EDGE_LOOP('',(#15014,#15015,#15016,#15017));
#6522=EDGE_LOOP('',(#15018,#15019,#15020,#15021));
#6523=EDGE_LOOP('',(#15022,#15023,#15024,#15025));
#6524=EDGE_LOOP('',(#15026,#15027,#15028,#15029));
#6525=EDGE_LOOP('',(#15030,#15031,#15032,#15033,#15034,#15035));
#6526=EDGE_LOOP('',(#15036,#15037,#15038,#15039));
#6527=EDGE_LOOP('',(#15040,#15041,#15042,#15043));
#6528=EDGE_LOOP('',(#15044,#15045,#15046,#15047));
#6529=EDGE_LOOP('',(#15048,#15049,#15050,#15051));
#6530=EDGE_LOOP('',(#15052,#15053,#15054,#15055));
#6531=EDGE_LOOP('',(#15056,#15057,#15058,#15059,#15060,#15061));
#6532=EDGE_LOOP('',(#15062,#15063,#15064,#15065));
#6533=EDGE_LOOP('',(#15066,#15067,#15068,#15069));
#6534=EDGE_LOOP('',(#15070,#15071,#15072,#15073));
#6535=EDGE_LOOP('',(#15074,#15075,#15076,#15077));
#6536=EDGE_LOOP('',(#15078,#15079,#15080,#15081));
#6537=EDGE_LOOP('',(#15082,#15083,#15084,#15085));
#6538=EDGE_LOOP('',(#15086,#15087,#15088,#15089));
#6539=EDGE_LOOP('',(#15090,#15091,#15092,#15093));
#6540=EDGE_LOOP('',(#15094,#15095,#15096,#15097));
#6541=EDGE_LOOP('',(#15098,#15099,#15100,#15101));
#6542=EDGE_LOOP('',(#15102,#15103,#15104,#15105));
#6543=EDGE_LOOP('',(#15106,#15107,#15108,#15109));
#6544=EDGE_LOOP('',(#15110,#15111,#15112,#15113));
#6545=EDGE_LOOP('',(#15114,#15115,#15116,#15117));
#6546=EDGE_LOOP('',(#15118,#15119,#15120,#15121));
#6547=EDGE_LOOP('',(#15122,#15123,#15124,#15125));
#6548=EDGE_LOOP('',(#15126,#15127,#15128,#15129));
#6549=EDGE_LOOP('',(#15130,#15131,#15132,#15133,#15134,#15135,#15136,#15137));
#6550=EDGE_LOOP('',(#15138,#15139,#15140,#15141));
#6551=EDGE_LOOP('',(#15142,#15143,#15144,#15145,#15146,#15147));
#6552=EDGE_LOOP('',(#15148,#15149,#15150,#15151));
#6553=EDGE_LOOP('',(#15152,#15153,#15154,#15155));
#6554=EDGE_LOOP('',(#15156,#15157,#15158,#15159));
#6555=EDGE_LOOP('',(#15160,#15161,#15162,#15163));
#6556=EDGE_LOOP('',(#15164,#15165,#15166,#15167,#15168,#15169,#15170,#15171,
#15172,#15173,#15174,#15175,#15176,#15177,#15178,#15179,#15180,#15181,#15182,
#15183,#15184,#15185,#15186,#15187));
#6557=EDGE_LOOP('',(#15188,#15189,#15190,#15191,#15192,#15193,#15194,#15195,
#15196,#15197,#15198,#15199,#15200,#15201,#15202,#15203));
#6558=EDGE_LOOP('',(#15204,#15205,#15206,#15207));
#6559=EDGE_LOOP('',(#15208));
#6560=EDGE_LOOP('',(#15209,#15210,#15211,#15212,#15213,#15214));
#6561=EDGE_LOOP('',(#15215));
#6562=EDGE_LOOP('',(#15216,#15217,#15218,#15219,#15220,#15221));
#6563=EDGE_LOOP('',(#15222,#15223,#15224,#15225,#15226,#15227));
#6564=EDGE_LOOP('',(#15228,#15229,#15230,#15231,#15232,#15233));
#6565=EDGE_LOOP('',(#15234,#15235,#15236,#15237,#15238,#15239,#15240,#15241,
#15242,#15243));
#6566=EDGE_LOOP('',(#15244,#15245,#15246,#15247));
#6567=EDGE_LOOP('',(#15248,#15249,#15250,#15251,#15252,#15253,#15254,#15255));
#6568=EDGE_LOOP('',(#15256,#15257,#15258,#15259,#15260,#15261));
#6569=EDGE_LOOP('',(#15262));
#6570=EDGE_LOOP('',(#15263,#15264,#15265,#15266,#15267));
#6571=EDGE_LOOP('',(#15268,#15269,#15270,#15271,#15272,#15273));
#6572=EDGE_LOOP('',(#15274,#15275,#15276,#15277,#15278,#15279));
#6573=EDGE_LOOP('',(#15280,#15281,#15282,#15283,#15284,#15285));
#6574=EDGE_LOOP('',(#15286,#15287,#15288,#15289,#15290,#15291,#15292,#15293));
#6575=EDGE_LOOP('',(#15294,#15295,#15296,#15297,#15298));
#6576=EDGE_LOOP('',(#15299,#15300,#15301,#15302));
#6577=EDGE_LOOP('',(#15303,#15304,#15305,#15306,#15307,#15308));
#6578=EDGE_LOOP('',(#15309,#15310,#15311,#15312,#15313,#15314));
#6579=EDGE_LOOP('',(#15315));
#6580=EDGE_LOOP('',(#15316,#15317,#15318,#15319,#15320,#15321));
#6581=EDGE_LOOP('',(#15322,#15323,#15324,#15325,#15326,#15327,#15328,#15329,
#15330,#15331));
#6582=EDGE_LOOP('',(#15332,#15333,#15334,#15335));
#6583=EDGE_LOOP('',(#15336,#15337,#15338,#15339,#15340,#15341));
#6584=EDGE_LOOP('',(#15342,#15343,#15344,#15345,#15346,#15347));
#6585=EDGE_LOOP('',(#15348));
#6586=EDGE_LOOP('',(#15349,#15350,#15351,#15352));
#6587=EDGE_LOOP('',(#15353,#15354,#15355,#15356,#15357,#15358));
#6588=EDGE_LOOP('',(#15359));
#6589=EDGE_LOOP('',(#15360,#15361,#15362,#15363,#15364,#15365));
#6590=EDGE_LOOP('',(#15366,#15367,#15368,#15369,#15370,#15371,#15372,#15373,
#15374,#15375));
#6591=EDGE_LOOP('',(#15376,#15377,#15378,#15379,#15380,#15381));
#6592=EDGE_LOOP('',(#15382,#15383,#15384,#15385));
#6593=EDGE_LOOP('',(#15386));
#6594=EDGE_LOOP('',(#15387));
#6595=EDGE_LOOP('',(#15388,#15389,#15390,#15391,#15392,#15393));
#6596=EDGE_LOOP('',(#15394));
#6597=EDGE_LOOP('',(#15395,#15396,#15397,#15398));
#6598=EDGE_LOOP('',(#15399,#15400,#15401,#15402,#15403,#15404,#15405,#15406));
#6599=EDGE_LOOP('',(#15407,#15408,#15409,#15410));
#6600=EDGE_LOOP('',(#15411,#15412,#15413,#15414));
#6601=EDGE_LOOP('',(#15415,#15416,#15417,#15418));
#6602=EDGE_LOOP('',(#15419,#15420,#15421,#15422));
#6603=EDGE_LOOP('',(#15423,#15424,#15425,#15426));
#6604=EDGE_LOOP('',(#15427,#15428,#15429,#15430,#15431,#15432,#15433,#15434));
#6605=EDGE_LOOP('',(#15435,#15436,#15437,#15438,#15439,#15440));
#6606=EDGE_LOOP('',(#15441));
#6607=EDGE_LOOP('',(#15442,#15443,#15444,#15445));
#6608=EDGE_LOOP('',(#15446,#15447,#15448,#15449,#15450,#15451,#15452,#15453));
#6609=EDGE_LOOP('',(#15454,#15455,#15456,#15457));
#6610=EDGE_LOOP('',(#15458,#15459,#15460,#15461,#15462,#15463));
#6611=EDGE_LOOP('',(#15464,#15465,#15466,#15467));
#6612=EDGE_LOOP('',(#15468,#15469,#15470,#15471,#15472,#15473));
#6613=EDGE_LOOP('',(#15474,#15475,#15476,#15477));
#6614=EDGE_LOOP('',(#15478,#15479,#15480,#15481,#15482,#15483,#15484,#15485));
#6615=EDGE_LOOP('',(#15486,#15487,#15488,#15489,#15490,#15491));
#6616=EDGE_LOOP('',(#15492));
#6617=EDGE_LOOP('',(#15493,#15494,#15495,#15496));
#6618=EDGE_LOOP('',(#15497,#15498,#15499,#15500,#15501,#15502,#15503,#15504));
#6619=EDGE_LOOP('',(#15505,#15506,#15507,#15508));
#6620=EDGE_LOOP('',(#15509,#15510,#15511,#15512));
#6621=EDGE_LOOP('',(#15513,#15514,#15515,#15516));
#6622=EDGE_LOOP('',(#15517,#15518,#15519,#15520));
#6623=EDGE_LOOP('',(#15521,#15522,#15523,#15524));
#6624=EDGE_LOOP('',(#15525,#15526,#15527,#15528,#15529,#15530,#15531,#15532));
#6625=EDGE_LOOP('',(#15533,#15534,#15535,#15536,#15537,#15538));
#6626=EDGE_LOOP('',(#15539));
#6627=EDGE_LOOP('',(#15540,#15541,#15542,#15543));
#6628=EDGE_LOOP('',(#15544,#15545,#15546,#15547,#15548,#15549,#15550,#15551));
#6629=EDGE_LOOP('',(#15552,#15553,#15554,#15555));
#6630=EDGE_LOOP('',(#15556,#15557,#15558,#15559));
#6631=EDGE_LOOP('',(#15560,#15561,#15562,#15563));
#6632=EDGE_LOOP('',(#15564,#15565,#15566,#15567));
#6633=EDGE_LOOP('',(#15568,#15569,#15570,#15571));
#6634=EDGE_LOOP('',(#15572,#15573,#15574,#15575,#15576,#15577,#15578,#15579));
#6635=EDGE_LOOP('',(#15580,#15581,#15582,#15583));
#6636=EDGE_LOOP('',(#15584,#15585,#15586,#15587));
#6637=EDGE_LOOP('',(#15588,#15589,#15590,#15591));
#6638=EDGE_LOOP('',(#15592,#15593,#15594,#15595));
#6639=EDGE_LOOP('',(#15596,#15597,#15598,#15599));
#6640=EDGE_LOOP('',(#15600,#15601,#15602,#15603));
#6641=EDGE_LOOP('',(#15604));
#6642=EDGE_LOOP('',(#15605));
#6643=EDGE_LOOP('',(#15606));
#6644=EDGE_LOOP('',(#15607));
#6645=EDGE_LOOP('',(#15608,#15609,#15610,#15611));
#6646=EDGE_LOOP('',(#15612,#15613,#15614,#15615,#15616));
#6647=EDGE_LOOP('',(#15617,#15618,#15619,#15620));
#6648=EDGE_LOOP('',(#15621,#15622,#15623,#15624,#15625));
#6649=EDGE_LOOP('',(#15626));
#6650=EDGE_LOOP('',(#15627));
#6651=EDGE_LOOP('',(#15628));
#6652=EDGE_LOOP('',(#15629));
#6653=EDGE_LOOP('',(#15630,#15631,#15632,#15633,#15634,#15635));
#6654=EDGE_LOOP('',(#15636,#15637,#15638,#15639,#15640,#15641,#15642,#15643));
#6655=EDGE_LOOP('',(#15644,#15645,#15646,#15647,#15648,#15649));
#6656=EDGE_LOOP('',(#15650,#15651,#15652,#15653,#15654,#15655,#15656,#15657,
#15658,#15659));
#6657=EDGE_LOOP('',(#15660,#15661,#15662,#15663,#15664,#15665));
#6658=EDGE_LOOP('',(#15666,#15667,#15668,#15669,#15670,#15671,#15672,#15673));
#6659=EDGE_LOOP('',(#15674,#15675,#15676,#15677,#15678,#15679));
#6660=EDGE_LOOP('',(#15680,#15681,#15682,#15683,#15684,#15685,#15686,#15687,
#15688,#15689));
#6661=EDGE_LOOP('',(#15690,#15691,#15692,#15693,#15694,#15695));
#6662=EDGE_LOOP('',(#15696,#15697,#15698,#15699,#15700,#15701,#15702,#15703));
#6663=EDGE_LOOP('',(#15704,#15705,#15706,#15707,#15708,#15709));
#6664=EDGE_LOOP('',(#15710,#15711,#15712,#15713,#15714,#15715,#15716,#15717,
#15718,#15719));
#6665=EDGE_LOOP('',(#15720,#15721,#15722,#15723,#15724,#15725));
#6666=EDGE_LOOP('',(#15726,#15727,#15728,#15729,#15730,#15731,#15732,#15733));
#6667=EDGE_LOOP('',(#15734,#15735,#15736,#15737,#15738,#15739));
#6668=EDGE_LOOP('',(#15740,#15741,#15742,#15743,#15744,#15745,#15746,#15747,
#15748,#15749));
#6669=EDGE_LOOP('',(#15750));
#6670=EDGE_LOOP('',(#15751,#15752,#15753,#15754,#15755,#15756));
#6671=EDGE_LOOP('',(#15757,#15758,#15759,#15760,#15761,#15762));
#6672=EDGE_LOOP('',(#15763,#15764,#15765,#15766));
#6673=EDGE_LOOP('',(#15767,#15768,#15769,#15770));
#6674=EDGE_LOOP('',(#15771,#15772,#15773,#15774));
#6675=EDGE_LOOP('',(#15775,#15776,#15777,#15778,#15779,#15780,#15781,#15782,
#15783));
#6676=EDGE_LOOP('',(#15784,#15785,#15786,#15787));
#6677=EDGE_LOOP('',(#15788,#15789,#15790,#15791));
#6678=EDGE_LOOP('',(#15792,#15793,#15794,#15795));
#6679=EDGE_LOOP('',(#15796,#15797,#15798,#15799));
#6680=EDGE_LOOP('',(#15800,#15801,#15802,#15803));
#6681=EDGE_LOOP('',(#15804,#15805,#15806,#15807));
#6682=EDGE_LOOP('',(#15808,#15809,#15810,#15811,#15812,#15813,#15814,#15815));
#6683=EDGE_LOOP('',(#15816,#15817,#15818,#15819));
#6684=EDGE_LOOP('',(#15820,#15821,#15822,#15823));
#6685=EDGE_LOOP('',(#15824,#15825,#15826,#15827));
#6686=EDGE_LOOP('',(#15828,#15829,#15830,#15831,#15832,#15833,#15834,#15835));
#6687=EDGE_LOOP('',(#15836,#15837,#15838,#15839,#15840,#15841,#15842,#15843));
#6688=EDGE_LOOP('',(#15844));
#6689=EDGE_LOOP('',(#15845,#15846,#15847,#15848));
#6690=EDGE_LOOP('',(#15849,#15850,#15851,#15852));
#6691=EDGE_LOOP('',(#15853,#15854,#15855,#15856,#15857,#15858,#15859,#15860));
#6692=EDGE_LOOP('',(#15861));
#6693=EDGE_LOOP('',(#15862,#15863,#15864,#15865,#15866,#15867));
#6694=EDGE_LOOP('',(#15868,#15869,#15870,#15871));
#6695=EDGE_LOOP('',(#15872,#15873,#15874,#15875));
#6696=EDGE_LOOP('',(#15876,#15877,#15878,#15879));
#6697=EDGE_LOOP('',(#15880,#15881,#15882,#15883));
#6698=EDGE_LOOP('',(#15884,#15885,#15886,#15887));
#6699=EDGE_LOOP('',(#15888,#15889,#15890,#15891));
#6700=EDGE_LOOP('',(#15892,#15893,#15894,#15895));
#6701=EDGE_LOOP('',(#15896,#15897,#15898,#15899,#15900,#15901));
#6702=EDGE_LOOP('',(#15902,#15903,#15904,#15905));
#6703=EDGE_LOOP('',(#15906));
#6704=EDGE_LOOP('',(#15907));
#6705=EDGE_LOOP('',(#15908));
#6706=EDGE_LOOP('',(#15909));
#6707=EDGE_LOOP('',(#15910));
#6708=EDGE_LOOP('',(#15911));
#6709=EDGE_LOOP('',(#15912));
#6710=EDGE_LOOP('',(#15913));
#6711=EDGE_LOOP('',(#15914));
#6712=EDGE_LOOP('',(#15915));
#6713=EDGE_LOOP('',(#15916,#15917));
#6714=EDGE_LOOP('',(#15918,#15919,#15920,#15921,#15922));
#6715=EDGE_LOOP('',(#15923,#15924,#15925,#15926,#15927,#15928));
#6716=EDGE_LOOP('',(#15929,#15930,#15931,#15932,#15933,#15934));
#6717=EDGE_LOOP('',(#15935,#15936,#15937,#15938,#15939,#15940));
#6718=EDGE_LOOP('',(#15941,#15942,#15943));
#6719=EDGE_LOOP('',(#15944,#15945,#15946,#15947));
#6720=EDGE_LOOP('',(#15948,#15949,#15950));
#6721=EDGE_LOOP('',(#15951,#15952,#15953));
#6722=EDGE_LOOP('',(#15954,#15955,#15956,#15957));
#6723=EDGE_LOOP('',(#15958,#15959,#15960));
#6724=EDGE_LOOP('',(#15961,#15962,#15963,#15964));
#6725=EDGE_LOOP('',(#15965,#15966,#15967));
#6726=EDGE_LOOP('',(#15968,#15969,#15970,#15971));
#6727=EDGE_LOOP('',(#15972,#15973,#15974));
#6728=EDGE_LOOP('',(#15975,#15976,#15977));
#6729=EDGE_LOOP('',(#15978,#15979,#15980,#15981));
#6730=EDGE_LOOP('',(#15982,#15983,#15984));
#6731=EDGE_LOOP('',(#15985,#15986,#15987,#15988));
#6732=EDGE_LOOP('',(#15989,#15990,#15991,#15992));
#6733=EDGE_LOOP('',(#15993,#15994,#15995,#15996));
#6734=EDGE_LOOP('',(#15997,#15998,#15999,#16000));
#6735=EDGE_LOOP('',(#16001,#16002,#16003,#16004));
#6736=EDGE_LOOP('',(#16005,#16006,#16007,#16008));
#6737=EDGE_LOOP('',(#16009,#16010,#16011,#16012,#16013));
#6738=EDGE_LOOP('',(#16014,#16015,#16016));
#6739=EDGE_LOOP('',(#16017,#16018,#16019,#16020,#16021,#16022));
#6740=EDGE_LOOP('',(#16023,#16024,#16025,#16026,#16027,#16028));
#6741=EDGE_LOOP('',(#16029,#16030,#16031));
#6742=EDGE_LOOP('',(#16032,#16033,#16034,#16035,#16036,#16037));
#6743=EDGE_LOOP('',(#16038,#16039,#16040,#16041,#16042,#16043));
#6744=EDGE_LOOP('',(#16044,#16045,#16046,#16047,#16048,#16049));
#6745=EDGE_LOOP('',(#16050,#16051,#16052,#16053,#16054,#16055));
#6746=EDGE_LOOP('',(#16056,#16057,#16058,#16059));
#6747=EDGE_LOOP('',(#16060,#16061,#16062,#16063));
#6748=EDGE_LOOP('',(#16064,#16065,#16066,#16067));
#6749=EDGE_LOOP('',(#16068,#16069,#16070,#16071));
#6750=EDGE_LOOP('',(#16072,#16073,#16074,#16075,#16076,#16077));
#6751=EDGE_LOOP('',(#16078,#16079,#16080,#16081,#16082,#16083));
#6752=EDGE_LOOP('',(#16084,#16085,#16086,#16087));
#6753=EDGE_LOOP('',(#16088,#16089,#16090,#16091));
#6754=EDGE_LOOP('',(#16092,#16093,#16094,#16095));
#6755=EDGE_LOOP('',(#16096,#16097,#16098,#16099));
#6756=EDGE_LOOP('',(#16100,#16101,#16102,#16103));
#6757=EDGE_LOOP('',(#16104,#16105,#16106,#16107));
#6758=EDGE_LOOP('',(#16108,#16109,#16110));
#6759=EDGE_LOOP('',(#16111,#16112,#16113,#16114));
#6760=EDGE_LOOP('',(#16115,#16116,#16117,#16118,#16119));
#6761=EDGE_LOOP('',(#16120,#16121,#16122,#16123));
#6762=EDGE_LOOP('',(#16124,#16125,#16126,#16127));
#6763=EDGE_LOOP('',(#16128,#16129,#16130,#16131));
#6764=EDGE_LOOP('',(#16132,#16133,#16134,#16135));
#6765=EDGE_LOOP('',(#16136,#16137,#16138,#16139));
#6766=EDGE_LOOP('',(#16140,#16141,#16142,#16143));
#6767=EDGE_LOOP('',(#16144,#16145,#16146,#16147));
#6768=EDGE_LOOP('',(#16148,#16149,#16150,#16151,#16152));
#6769=EDGE_LOOP('',(#16153,#16154,#16155,#16156));
#6770=EDGE_LOOP('',(#16157,#16158,#16159,#16160));
#6771=EDGE_LOOP('',(#16161,#16162,#16163,#16164));
#6772=EDGE_LOOP('',(#16165,#16166,#16167,#16168));
#6773=EDGE_LOOP('',(#16169,#16170,#16171,#16172));
#6774=EDGE_LOOP('',(#16173,#16174,#16175,#16176));
#6775=EDGE_LOOP('',(#16177,#16178,#16179,#16180));
#6776=EDGE_LOOP('',(#16181,#16182,#16183,#16184,#16185,#16186,#16187,#16188,
#16189,#16190,#16191,#16192,#16193,#16194,#16195,#16196,#16197,#16198));
#6777=EDGE_LOOP('',(#16199,#16200,#16201,#16202,#16203,#16204,#16205,#16206,
#16207,#16208,#16209,#16210,#16211,#16212,#16213,#16214,#16215,#16216,#16217,
#16218));
#6778=EDGE_LOOP('',(#16219,#16220,#16221,#16222,#16223,#16224));
#6779=EDGE_LOOP('',(#16225,#16226,#16227));
#6780=EDGE_LOOP('',(#16228,#16229,#16230,#16231,#16232,#16233));
#6781=EDGE_LOOP('',(#16234,#16235,#16236,#16237,#16238,#16239));
#6782=EDGE_LOOP('',(#16240,#16241,#16242));
#6783=EDGE_LOOP('',(#16243,#16244,#16245,#16246,#16247));
#6784=EDGE_LOOP('',(#16248,#16249,#16250,#16251,#16252,#16253));
#6785=EDGE_LOOP('',(#16254,#16255,#16256,#16257,#16258,#16259));
#6786=EDGE_LOOP('',(#16260,#16261,#16262,#16263));
#6787=EDGE_LOOP('',(#16264,#16265,#16266,#16267,#16268,#16269,#16270,#16271));
#6788=EDGE_LOOP('',(#16272,#16273,#16274));
#6789=EDGE_LOOP('',(#16275,#16276,#16277));
#6790=EDGE_LOOP('',(#16278,#16279,#16280,#16281,#16282,#16283,#16284,#16285));
#6791=EDGE_LOOP('',(#16286,#16287,#16288));
#6792=EDGE_LOOP('',(#16289,#16290,#16291,#16292));
#6793=EDGE_LOOP('',(#16293,#16294,#16295,#16296,#16297));
#6794=EDGE_LOOP('',(#16298,#16299,#16300,#16301,#16302,#16303,#16304,#16305,
#16306,#16307,#16308,#16309,#16310,#16311,#16312,#16313,#16314,#16315,#16316,
#16317,#16318,#16319,#16320,#16321,#16322,#16323,#16324,#16325,#16326));
#6795=EDGE_LOOP('',(#16327,#16328,#16329,#16330));
#6796=EDGE_LOOP('',(#16331,#16332,#16333,#16334));
#6797=EDGE_LOOP('',(#16335,#16336,#16337,#16338));
#6798=EDGE_LOOP('',(#16339,#16340,#16341,#16342));
#6799=EDGE_LOOP('',(#16343,#16344,#16345,#16346));
#6800=EDGE_LOOP('',(#16347,#16348,#16349,#16350));
#6801=EDGE_LOOP('',(#16351,#16352,#16353));
#6802=EDGE_LOOP('',(#16354,#16355,#16356));
#6803=EDGE_LOOP('',(#16357,#16358,#16359,#16360));
#6804=EDGE_LOOP('',(#16361,#16362,#16363,#16364,#16365));
#6805=EDGE_LOOP('',(#16366,#16367,#16368,#16369));
#6806=EDGE_LOOP('',(#16370,#16371,#16372,#16373));
#6807=EDGE_LOOP('',(#16374,#16375,#16376,#16377));
#6808=EDGE_LOOP('',(#16378,#16379,#16380,#16381));
#6809=EDGE_LOOP('',(#16382,#16383,#16384,#16385));
#6810=EDGE_LOOP('',(#16386,#16387,#16388,#16389));
#6811=EDGE_LOOP('',(#16390,#16391,#16392,#16393));
#6812=EDGE_LOOP('',(#16394,#16395,#16396,#16397));
#6813=EDGE_LOOP('',(#16398,#16399,#16400,#16401));
#6814=EDGE_LOOP('',(#16402,#16403,#16404,#16405));
#6815=EDGE_LOOP('',(#16406,#16407,#16408,#16409));
#6816=EDGE_LOOP('',(#16410,#16411,#16412,#16413));
#6817=EDGE_LOOP('',(#16414));
#6818=EDGE_LOOP('',(#16415));
#6819=EDGE_LOOP('',(#16416,#16417,#16418,#16419,#16420,#16421));
#6820=EDGE_LOOP('',(#16422));
#6821=EDGE_LOOP('',(#16423,#16424,#16425,#16426));
#6822=EDGE_LOOP('',(#16427));
#6823=EDGE_LOOP('',(#16428));
#6824=EDGE_LOOP('',(#16429));
#6825=EDGE_LOOP('',(#16430));
#6826=EDGE_LOOP('',(#16431,#16432,#16433,#16434,#16435,#16436));
#6827=EDGE_LOOP('',(#16437,#16438,#16439,#16440));
#6828=EDGE_LOOP('',(#16441,#16442,#16443,#16444,#16445,#16446));
#6829=EDGE_LOOP('',(#16447,#16448,#16449,#16450));
#6830=EDGE_LOOP('',(#16451,#16452,#16453,#16454));
#6831=EDGE_LOOP('',(#16455,#16456,#16457,#16458));
#6832=EDGE_LOOP('',(#16459,#16460,#16461,#16462));
#6833=EDGE_LOOP('',(#16463,#16464,#16465,#16466));
#6834=EDGE_LOOP('',(#16467,#16468,#16469,#16470));
#6835=EDGE_LOOP('',(#16471,#16472,#16473,#16474));
#6836=EDGE_LOOP('',(#16475,#16476,#16477,#16478,#16479,#16480));
#6837=EDGE_LOOP('',(#16481,#16482,#16483,#16484));
#6838=EDGE_LOOP('',(#16485,#16486,#16487,#16488));
#6839=EDGE_LOOP('',(#16489,#16490,#16491,#16492,#16493,#16494));
#6840=EDGE_LOOP('',(#16495,#16496,#16497,#16498));
#6841=EDGE_LOOP('',(#16499,#16500,#16501,#16502));
#6842=EDGE_LOOP('',(#16503));
#6843=EDGE_LOOP('',(#16504,#16505,#16506,#16507,#16508,#16509));
#6844=EDGE_LOOP('',(#16510,#16511,#16512,#16513));
#6845=EDGE_LOOP('',(#16514,#16515,#16516,#16517,#16518,#16519,#16520));
#6846=EDGE_LOOP('',(#16521,#16522,#16523,#16524,#16525,#16526));
#6847=EDGE_LOOP('',(#16527,#16528,#16529));
#6848=EDGE_LOOP('',(#16530,#16531,#16532,#16533,#16534,#16535,#16536));
#6849=EDGE_LOOP('',(#16537,#16538,#16539,#16540,#16541,#16542));
#6850=EDGE_LOOP('',(#16543,#16544,#16545,#16546,#16547,#16548,#16549,#16550,
#16551,#16552,#16553,#16554,#16555,#16556,#16557,#16558,#16559,#16560,#16561,
#16562,#16563,#16564,#16565,#16566,#16567,#16568,#16569,#16570,#16571));
#6851=EDGE_LOOP('',(#16572,#16573,#16574));
#6852=EDGE_LOOP('',(#16575,#16576,#16577,#16578));
#6853=EDGE_LOOP('',(#16579,#16580,#16581,#16582,#16583));
#6854=EDGE_LOOP('',(#16584,#16585,#16586,#16587));
#6855=EDGE_LOOP('',(#16588,#16589,#16590,#16591));
#6856=EDGE_LOOP('',(#16592,#16593,#16594,#16595,#16596,#16597,#16598));
#6857=EDGE_LOOP('',(#16599,#16600,#16601,#16602,#16603,#16604));
#6858=EDGE_LOOP('',(#16605,#16606,#16607,#16608,#16609));
#6859=EDGE_LOOP('',(#16610,#16611,#16612,#16613,#16614,#16615,#16616));
#6860=EDGE_LOOP('',(#16617,#16618,#16619,#16620,#16621,#16622));
#6861=EDGE_LOOP('',(#16623));
#6862=EDGE_LOOP('',(#16624,#16625,#16626,#16627,#16628,#16629));
#6863=EDGE_LOOP('',(#16630,#16631,#16632,#16633));
#6864=EDGE_LOOP('',(#16634,#16635,#16636,#16637));
#6865=EDGE_LOOP('',(#16638,#16639,#16640,#16641));
#6866=EDGE_LOOP('',(#16642,#16643,#16644,#16645));
#6867=EDGE_LOOP('',(#16646,#16647,#16648,#16649));
#6868=EDGE_LOOP('',(#16650,#16651,#16652,#16653));
#6869=EDGE_LOOP('',(#16654,#16655,#16656,#16657));
#6870=EDGE_LOOP('',(#16658,#16659,#16660,#16661));
#6871=EDGE_LOOP('',(#16662,#16663,#16664,#16665));
#6872=EDGE_LOOP('',(#16666,#16667,#16668,#16669));
#6873=EDGE_LOOP('',(#16670,#16671,#16672,#16673));
#6874=EDGE_LOOP('',(#16674,#16675,#16676,#16677));
#6875=EDGE_LOOP('',(#16678,#16679,#16680,#16681));
#6876=EDGE_LOOP('',(#16682));
#6877=EDGE_LOOP('',(#16683,#16684,#16685,#16686,#16687,#16688));
#6878=EDGE_LOOP('',(#16689,#16690,#16691,#16692,#16693));
#6879=EDGE_LOOP('',(#16694,#16695,#16696,#16697,#16698,#16699,#16700));
#6880=EDGE_LOOP('',(#16701,#16702));
#6881=EDGE_LOOP('',(#16703,#16704));
#6882=EDGE_LOOP('',(#16705,#16706,#16707));
#6883=EDGE_LOOP('',(#16708,#16709,#16710,#16711,#16712,#16713,#16714,#16715));
#6884=EDGE_LOOP('',(#16716,#16717,#16718,#16719,#16720,#16721));
#6885=EDGE_LOOP('',(#16722,#16723,#16724,#16725));
#6886=EDGE_LOOP('',(#16726,#16727,#16728,#16729,#16730,#16731));
#6887=EDGE_LOOP('',(#16732,#16733,#16734,#16735,#16736,#16737));
#6888=EDGE_LOOP('',(#16738,#16739,#16740,#16741,#16742,#16743,#16744,#16745));
#6889=EDGE_LOOP('',(#16746,#16747));
#6890=EDGE_LOOP('',(#16748,#16749));
#6891=EDGE_LOOP('',(#16750,#16751,#16752,#16753));
#6892=EDGE_LOOP('',(#16754,#16755,#16756,#16757));
#6893=EDGE_LOOP('',(#16758,#16759,#16760,#16761,#16762,#16763,#16764));
#6894=EDGE_LOOP('',(#16765));
#6895=EDGE_LOOP('',(#16766,#16767,#16768,#16769));
#6896=EDGE_LOOP('',(#16770,#16771,#16772,#16773));
#6897=EDGE_LOOP('',(#16774));
#6898=EDGE_LOOP('',(#16775,#16776,#16777,#16778,#16779,#16780));
#6899=EDGE_LOOP('',(#16781,#16782,#16783,#16784,#16785,#16786));
#6900=EDGE_LOOP('',(#16787,#16788,#16789,#16790));
#6901=EDGE_LOOP('',(#16791,#16792,#16793,#16794));
#6902=EDGE_LOOP('',(#16795,#16796,#16797,#16798));
#6903=EDGE_LOOP('',(#16799,#16800,#16801,#16802));
#6904=EDGE_LOOP('',(#16803,#16804,#16805,#16806));
#6905=EDGE_LOOP('',(#16807,#16808,#16809,#16810,#16811,#16812,#16813,#16814,
#16815,#16816,#16817,#16818,#16819,#16820));
#6906=EDGE_LOOP('',(#16821));
#6907=EDGE_LOOP('',(#16822,#16823,#16824,#16825));
#6908=EDGE_LOOP('',(#16826,#16827,#16828,#16829));
#6909=EDGE_LOOP('',(#16830,#16831,#16832,#16833));
#6910=EDGE_LOOP('',(#16834,#16835,#16836,#16837));
#6911=EDGE_LOOP('',(#16838,#16839,#16840,#16841));
#6912=EDGE_LOOP('',(#16842,#16843,#16844,#16845,#16846,#16847));
#6913=EDGE_LOOP('',(#16848,#16849,#16850,#16851));
#6914=EDGE_LOOP('',(#16852,#16853,#16854,#16855,#16856,#16857,#16858,#16859,
#16860,#16861,#16862,#16863));
#6915=EDGE_LOOP('',(#16864,#16865,#16866,#16867));
#6916=EDGE_LOOP('',(#16868,#16869,#16870,#16871));
#6917=EDGE_LOOP('',(#16872,#16873,#16874,#16875,#16876,#16877,#16878,#16879,
#16880,#16881,#16882,#16883,#16884,#16885));
#6918=EDGE_LOOP('',(#16886,#16887,#16888,#16889,#16890,#16891,#16892,#16893,
#16894,#16895));
#6919=EDGE_LOOP('',(#16896,#16897,#16898));
#6920=EDGE_LOOP('',(#16899,#16900,#16901,#16902));
#6921=EDGE_LOOP('',(#16903,#16904,#16905));
#6922=EDGE_LOOP('',(#16906,#16907,#16908,#16909,#16910,#16911));
#6923=EDGE_LOOP('',(#16912,#16913,#16914,#16915,#16916,#16917,#16918,#16919,
#16920,#16921,#16922,#16923));
#6924=EDGE_LOOP('',(#16924,#16925,#16926,#16927,#16928,#16929,#16930));
#6925=EDGE_LOOP('',(#16931,#16932,#16933,#16934,#16935,#16936));
#6926=EDGE_LOOP('',(#16937,#16938,#16939,#16940));
#6927=EDGE_LOOP('',(#16941,#16942,#16943,#16944));
#6928=EDGE_LOOP('',(#16945,#16946,#16947,#16948,#16949,#16950));
#6929=EDGE_LOOP('',(#16951,#16952,#16953,#16954,#16955,#16956));
#6930=EDGE_LOOP('',(#16957));
#6931=EDGE_LOOP('',(#16958,#16959,#16960,#16961));
#6932=EDGE_LOOP('',(#16962,#16963,#16964,#16965));
#6933=EDGE_LOOP('',(#16966,#16967,#16968,#16969));
#6934=EDGE_LOOP('',(#16970,#16971,#16972,#16973));
#6935=EDGE_LOOP('',(#16974,#16975,#16976,#16977,#16978,#16979,#16980));
#6936=EDGE_LOOP('',(#16981,#16982,#16983,#16984));
#6937=EDGE_LOOP('',(#16985,#16986,#16987,#16988));
#6938=EDGE_LOOP('',(#16989));
#6939=EDGE_LOOP('',(#16990,#16991,#16992,#16993));
#6940=EDGE_LOOP('',(#16994,#16995,#16996,#16997));
#6941=EDGE_LOOP('',(#16998,#16999,#17000,#17001));
#6942=EDGE_LOOP('',(#17002,#17003,#17004,#17005));
#6943=EDGE_LOOP('',(#17006));
#6944=EDGE_LOOP('',(#17007,#17008,#17009,#17010));
#6945=EDGE_LOOP('',(#17011,#17012,#17013,#17014));
#6946=EDGE_LOOP('',(#17015,#17016,#17017,#17018));
#6947=EDGE_LOOP('',(#17019,#17020,#17021,#17022));
#6948=EDGE_LOOP('',(#17023,#17024,#17025,#17026,#17027,#17028));
#6949=EDGE_LOOP('',(#17029));
#6950=EDGE_LOOP('',(#17030,#17031,#17032,#17033));
#6951=EDGE_LOOP('',(#17034,#17035,#17036,#17037));
#6952=EDGE_LOOP('',(#17038,#17039,#17040,#17041,#17042,#17043,#17044,#17045,
#17046,#17047,#17048,#17049,#17050,#17051,#17052,#17053,#17054,#17055,#17056,
#17057,#17058,#17059));
#6953=EDGE_LOOP('',(#17060));
#6954=EDGE_LOOP('',(#17061,#17062,#17063,#17064,#17065,#17066,#17067));
#6955=EDGE_LOOP('',(#17068,#17069,#17070,#17071));
#6956=EDGE_LOOP('',(#17072,#17073,#17074,#17075,#17076,#17077));
#6957=EDGE_LOOP('',(#17078,#17079,#17080,#17081,#17082,#17083,#17084,#17085,
#17086,#17087));
#6958=EDGE_LOOP('',(#17088,#17089,#17090,#17091,#17092,#17093));
#6959=EDGE_LOOP('',(#17094,#17095,#17096,#17097,#17098));
#6960=EDGE_LOOP('',(#17099,#17100,#17101,#17102));
#6961=EDGE_LOOP('',(#17103,#17104,#17105,#17106,#17107));
#6962=EDGE_LOOP('',(#17108,#17109,#17110,#17111,#17112,#17113));
#6963=EDGE_LOOP('',(#17114,#17115,#17116,#17117,#17118,#17119,#17120,#17121));
#6964=EDGE_LOOP('',(#17122,#17123,#17124,#17125,#17126,#17127));
#6965=EDGE_LOOP('',(#17128,#17129,#17130,#17131));
#6966=EDGE_LOOP('',(#17132,#17133,#17134,#17135,#17136,#17137,#17138,#17139,
#17140,#17141,#17142,#17143));
#6967=EDGE_LOOP('',(#17144));
#6968=EDGE_LOOP('',(#17145));
#6969=EDGE_LOOP('',(#17146));
#6970=EDGE_LOOP('',(#17147));
#7235=CIRCLE('',#18854,25.3339394440353);
#7236=CIRCLE('',#18855,5.00000000000101);
#7237=CIRCLE('',#18856,27.3317482398799);
#7238=CIRCLE('',#18857,27.3317482398799);
#7239=CIRCLE('',#18859,28.6682517601201);
#7240=CIRCLE('',#18860,4.99999999999874);
#7241=CIRCLE('',#18861,29.7575436501051);
#7242=CIRCLE('',#18862,29.7575436501051);
#7243=CIRCLE('',#18863,28.6682517601201);
#7244=CIRCLE('',#18865,45.3097394023382);
#7245=CIRCLE('',#18866,4.00000000000009);
#7246=CIRCLE('',#18867,49.0555555555557);
#7247=CIRCLE('',#18868,49.0555555555557);
#7248=CIRCLE('',#18869,45.3097394023382);
#7249=CIRCLE('',#18871,32.793965079916);
#7250=CIRCLE('',#18872,3.99999999999933);
#7251=CIRCLE('',#18873,34.8097394023382);
#7252=CIRCLE('',#18874,34.8097394023382);
#7253=CIRCLE('',#18875,32.793965079916);
#7254=CIRCLE('',#18877,55.);
#7255=CIRCLE('',#18878,55.);
#7256=CIRCLE('',#18881,50.0000000000001);
#7257=CIRCLE('',#18887,0.857142857149273);
#7258=CIRCLE('',#18888,0.857142857149273);
#7259=CIRCLE('',#18889,0.800000000003749);
#7260=CIRCLE('',#18891,0.999999999962782);
#7261=CIRCLE('',#18894,0.499999999966139);
#7262=CIRCLE('',#18906,9.75000000013422);
#7263=CIRCLE('',#18907,19.9999999999997);
#7264=CIRCLE('',#18908,6.75000000007079);
#7265=CIRCLE('',#18909,6.75000000007079);
#7266=CIRCLE('',#18911,6.75000000000001);
#7267=CIRCLE('',#18912,6.75000000000001);
#7268=CIRCLE('',#18914,6.75);
#7269=CIRCLE('',#18915,6.75);
#7270=CIRCLE('',#18917,6.75000000000001);
#7271=CIRCLE('',#18918,6.75000000000001);
#7272=CIRCLE('',#18920,6.75);
#7273=CIRCLE('',#18921,6.75);
#7274=CIRCLE('',#18923,7.00000000000001);
#7275=CIRCLE('',#18925,7.00000000000001);
#7276=CIRCLE('',#18928,27.5);
#7277=CIRCLE('',#18929,27.5);
#7278=CIRCLE('',#18931,100.);
#7279=CIRCLE('',#18932,105.377972911614);
#7280=CIRCLE('',#18933,107.1412427187);
#7281=CIRCLE('',#18934,106.259607815157);
#7282=CIRCLE('',#18936,22.);
#7283=CIRCLE('',#18937,22.);
#7284=CIRCLE('',#18939,7.);
#7285=CIRCLE('',#18940,7.);
#7286=CIRCLE('',#18942,7.);
#7287=CIRCLE('',#18943,7.);
#7288=CIRCLE('',#18944,7.);
#7289=CIRCLE('',#18945,7.);
#7290=CIRCLE('',#18947,7.);
#7291=CIRCLE('',#18949,7.);
#7292=CIRCLE('',#18950,7.);
#7293=CIRCLE('',#18951,7.);
#7294=CIRCLE('',#18954,80.);
#7295=CIRCLE('',#18955,80.);
#7296=CIRCLE('',#18957,40.);
#7297=CIRCLE('',#18958,40.);
#7298=CIRCLE('',#18965,12.);
#7299=CIRCLE('',#18968,53.);
#7300=CIRCLE('',#18969,53.);
#7301=CIRCLE('',#18970,53.);
#7302=CIRCLE('',#18972,4.5);
#7303=CIRCLE('',#18973,4.5);
#7304=CIRCLE('',#18975,4.5);
#7305=CIRCLE('',#18976,4.5);
#7306=CIRCLE('',#18978,4.5);
#7307=CIRCLE('',#18979,4.5);
#7308=CIRCLE('',#18981,4.5);
#7309=CIRCLE('',#18982,4.5);
#7310=CIRCLE('',#18984,20.);
#7311=CIRCLE('',#18985,20.);
#7312=CIRCLE('',#18987,12.);
#7313=CIRCLE('',#18989,10.);
#7314=CIRCLE('',#18994,68.);
#7315=CIRCLE('',#18995,76.5);
#7316=CIRCLE('',#18996,68.);
#7317=CIRCLE('',#18997,76.5);
#7318=CIRCLE('',#18998,68.);
#7319=CIRCLE('',#18999,68.);
#7320=CIRCLE('',#19000,76.5);
#7321=CIRCLE('',#19001,68.);
#7322=CIRCLE('',#19002,76.5);
#7323=CIRCLE('',#19005,7.);
#7324=CIRCLE('',#19006,7.00000000000001);
#7325=CIRCLE('',#19007,7.00000000000001);
#7326=CIRCLE('',#19008,7.);
#7327=CIRCLE('',#19010,12.);
#7328=CIRCLE('',#19011,12.);
#7329=CIRCLE('',#19013,68.);
#7330=CIRCLE('',#19014,68.);
#7331=CIRCLE('',#19015,68.);
#7332=CIRCLE('',#19017,6.0000000000113);
#7333=CIRCLE('',#19019,4.);
#7334=CIRCLE('',#19020,4.);
#7335=CIRCLE('',#19022,4.);
#7336=CIRCLE('',#19023,4.);
#7337=CIRCLE('',#19025,4.);
#7338=CIRCLE('',#19026,4.);
#7339=CIRCLE('',#19028,4.);
#7340=CIRCLE('',#19029,4.);
#7341=CIRCLE('',#19031,17.4625);
#7342=CIRCLE('',#19032,17.4625);
#7343=CIRCLE('',#19033,17.4625);
#7344=CIRCLE('',#19034,17.4625);
#7345=CIRCLE('',#19035,17.4625);
#7346=CIRCLE('',#19036,17.4625);
#7347=CIRCLE('',#19038,8.00000000000001);
#7348=CIRCLE('',#19039,7.99999999999999);
#7349=CIRCLE('',#19041,8.00000000000001);
#7350=CIRCLE('',#19042,8.00000000000001);
#7351=CIRCLE('',#19044,16.4625);
#7352=CIRCLE('',#19046,7.00000000000001);
#7353=CIRCLE('',#19047,7.00000000000001);
#7354=CIRCLE('',#19049,7.00000000000001);
#7355=CIRCLE('',#19050,7.00000000000001);
#7356=CIRCLE('',#19052,3.);
#7357=CIRCLE('',#19053,3.);
#7358=CIRCLE('',#19055,3.00000000000307);
#7359=CIRCLE('',#19056,3.00000000000307);
#7360=CIRCLE('',#19058,3.0000000000021);
#7361=CIRCLE('',#19059,3.0000000000021);
#7362=CIRCLE('',#19061,2.99999999999927);
#7363=CIRCLE('',#19062,2.99999999999927);
#7364=CIRCLE('',#19064,68.);
#7365=CIRCLE('',#19065,68.);
#7366=CIRCLE('',#19067,6.7500000000354);
#7367=CIRCLE('',#19068,6.7500000000354);
#7368=CIRCLE('',#19070,944.519985714474);
#7369=CIRCLE('',#19071,945.);
#7370=CIRCLE('',#19073,5.49999999998363);
#7371=CIRCLE('',#19074,5.49999999998363);
#7372=CIRCLE('',#19076,5.5);
#7373=CIRCLE('',#19077,5.5);
#7374=CIRCLE('',#19079,941.808101337222);
#7375=CIRCLE('',#19080,941.808086415458);
#7376=CIRCLE('',#19081,942.);
#7377=CIRCLE('',#19082,941.808086538241);
#7378=CIRCLE('',#19083,941.808101200289);
#7379=CIRCLE('',#19085,8.8000000000042);
#7380=CIRCLE('',#19086,8.80000000000425);
#7381=CIRCLE('',#19088,8.80000000000415);
#7382=CIRCLE('',#19089,8.80000000000425);
#7383=CIRCLE('',#19091,6.34999999994079);
#7384=CIRCLE('',#19093,5.5);
#7385=CIRCLE('',#19094,5.5);
#7386=CIRCLE('',#19095,5.5);
#7387=CIRCLE('',#19097,179.500000000001);
#7388=CIRCLE('',#19098,179.500000000005);
#7389=CIRCLE('',#19111,16.);
#7390=CIRCLE('',#19112,16.0000000000001);
#7391=CIRCLE('',#19113,179.500000000005);
#7392=CIRCLE('',#19114,15.9999999999999);
#7393=CIRCLE('',#19115,16.);
#7394=CIRCLE('',#19116,16.);
#7395=CIRCLE('',#19117,15.9999999999999);
#7396=CIRCLE('',#19118,179.500000000006);
#7397=CIRCLE('',#19119,16.);
#7398=CIRCLE('',#19120,15.9999999999999);
#7399=CIRCLE('',#19121,179.5);
#7400=CIRCLE('',#19131,7.00000000000003);
#7401=CIRCLE('',#19133,7.00000000000011);
#7402=CIRCLE('',#19134,7.00000000000007);
#7403=CIRCLE('',#19136,7.00000000000003);
#7404=CIRCLE('',#19144,7.00000000000001);
#7405=CIRCLE('',#19146,7.00000000000006);
#7406=CIRCLE('',#19147,7.00000000000003);
#7407=CIRCLE('',#19149,7.00000000000006);
#7408=CIRCLE('',#19157,7.00000000000001);
#7409=CIRCLE('',#19159,6.99999999999996);
#7410=CIRCLE('',#19160,6.99999999999999);
#7411=CIRCLE('',#19162,7.00000000000001);
#7412=CIRCLE('',#19164,7.00000000000001);
#7413=CIRCLE('',#19172,6.99999999999999);
#7414=CIRCLE('',#19174,6.99999999999999);
#7415=CIRCLE('',#19176,7.00000000000001);
#7416=CIRCLE('',#19178,16.0000000000001);
#7417=CIRCLE('',#19181,15.9999999999999);
#7418=CIRCLE('',#19183,179.500000000001);
#7419=CIRCLE('',#19185,16.0000000000001);
#7420=CIRCLE('',#19188,15.9999999999999);
#7421=CIRCLE('',#19190,179.500000000007);
#7422=CIRCLE('',#19192,16.);
#7423=CIRCLE('',#19195,15.9999999999999);
#7424=CIRCLE('',#19197,16.);
#7425=CIRCLE('',#19200,15.9999999999999);
#7426=CIRCLE('',#19202,179.500000000005);
#7427=CIRCLE('',#19204,19.7365042497449);
#7428=CIRCLE('',#19206,19.7365042497449);
#7429=CIRCLE('',#19208,19.7365042498482);
#7430=CIRCLE('',#19210,19.7365042497453);
#7431=CIRCLE('',#19212,19.7365042497445);
#7432=CIRCLE('',#19214,19.7365042497295);
#7433=CIRCLE('',#19216,19.7365042497448);
#7434=CIRCLE('',#19218,19.7365042497449);
#7435=CIRCLE('',#19220,19.7365042497272);
#7436=CIRCLE('',#19222,19.736504249745);
#7437=CIRCLE('',#19224,19.7365042497451);
#7438=CIRCLE('',#19226,19.7365042497215);
#7439=CIRCLE('',#19230,6.99999999999999);
#7440=CIRCLE('',#19233,7.00000000000003);
#7441=CIRCLE('',#19235,6.99999999999996);
#7442=CIRCLE('',#19238,6.99999999999997);
#7443=CIRCLE('',#19241,80.4999999999992);
#7444=CIRCLE('',#19245,80.4999999999997);
#7445=CIRCLE('',#19249,80.4999999999963);
#7446=CIRCLE('',#19253,80.4999999999957);
#7447=CIRCLE('',#19256,150.000000000136);
#7448=CIRCLE('',#19257,149.99999999991);
#7449=CIRCLE('',#19258,150.000000000245);
#7450=CIRCLE('',#19259,149.999999999925);
#7451=CIRCLE('',#19260,150.000000000098);
#7452=CIRCLE('',#19261,150.000000000117);
#7453=CIRCLE('',#19262,150.000000000073);
#7454=CIRCLE('',#19267,6.99999999999999);
#7455=CIRCLE('',#19270,7.00000000000003);
#7456=CIRCLE('',#19273,7.00000000000001);
#7457=CIRCLE('',#19276,6.99999999999999);
#7458=CIRCLE('',#19279,941.808101449981);
#7459=CIRCLE('',#19281,941.808118804699);
#7460=CIRCLE('',#19283,941.808118685871);
#7461=CIRCLE('',#19285,941.808101328173);
#7462=CIRCLE('',#19287,219.614732166431);
#7463=CIRCLE('',#19293,199.807995098081);
#7464=CIRCLE('',#19295,199.807995098081);
#7465=CIRCLE('',#19297,199.807995098081);
#7466=CIRCLE('',#19299,199.807995098081);
#7467=CIRCLE('',#19300,22.0736331396068);
#7468=CIRCLE('',#19302,941.807993346891);
#7469=CIRCLE('',#19304,941.807993346891);
#7470=CIRCLE('',#19305,15.0039593060322);
#7471=CIRCLE('',#19307,941.807993346891);
#7472=CIRCLE('',#19309,941.807993346891);
#7473=CIRCLE('',#19311,4.);
#7474=CIRCLE('',#19312,4.);
#7475=CIRCLE('',#19313,4.);
#7476=CIRCLE('',#19314,4.);
#7477=CIRCLE('',#19316,22.3000008196592);
#7478=CIRCLE('',#19318,86.00000081803);
#7479=CIRCLE('',#19320,22.3000010500621);
#7480=CIRCLE('',#19322,942.000001054498);
#7481=CIRCLE('',#19324,22.3000013536827);
#7482=CIRCLE('',#19326,86.0000013640202);
#7483=CIRCLE('',#19328,22.3000017511903);
#7484=CIRCLE('',#19330,22.3000017511903);
#7485=CIRCLE('',#19332,86.0000013640202);
#7486=CIRCLE('',#19334,32.8000013531573);
#7487=CIRCLE('',#19336,200.000000812291);
#7488=CIRCLE('',#19338,32.8000008122913);
#7489=CIRCLE('',#19340,86.0000008122913);
#7490=CIRCLE('',#19342,22.3000008122913);
#7491=CIRCLE('',#19344,941.999999061101);
#7492=CIRCLE('',#19348,4.);
#7493=CIRCLE('',#19351,4.);
#7494=CIRCLE('',#19353,4.);
#7495=CIRCLE('',#19355,4.);
#7496=CIRCLE('',#19357,14.8404677219111);
#7497=CIRCLE('',#19359,14.840467735277);
#7498=CIRCLE('',#19360,14.8404675855456);
#7499=CIRCLE('',#19362,14.8404677463308);
#7500=CIRCLE('',#19363,14.8409372248161);
#7501=CIRCLE('',#19366,13.3716191641864);
#7502=CIRCLE('',#19368,13.3716183569085);
#7503=CIRCLE('',#19370,14.8404675936254);
#7504=CIRCLE('',#19372,24.7856889787886);
#7505=CIRCLE('',#19373,24.7856889787948);
#7506=CIRCLE('',#19374,944.519985714474);
#7507=CIRCLE('',#19375,24.7856889787948);
#7508=CIRCLE('',#19376,24.7856889787949);
#7509=CIRCLE('',#19377,944.519985714474);
#7510=CIRCLE('',#19378,24.7856889787946);
#7511=CIRCLE('',#19379,34.5199857136054);
#7512=CIRCLE('',#19380,179.519985714474);
#7513=CIRCLE('',#19381,34.5199857136052);
#7514=CIRCLE('',#19382,24.7856889787945);
#7515=CIRCLE('',#19390,25.2657032643209);
#7516=CIRCLE('',#19395,25.2657032643207);
#7517=CIRCLE('',#19397,945.);
#7518=CIRCLE('',#19399,25.2657032643207);
#7519=CIRCLE('',#19404,25.2657032643145);
#7520=CIRCLE('',#19406,25.2657032643204);
#7521=CIRCLE('',#19411,34.9999999991313);
#7522=CIRCLE('',#19413,180.);
#7523=CIRCLE('',#19415,34.9999999991315);
#7524=CIRCLE('',#19420,25.2657032643206);
#7525=CIRCLE('',#19422,945.);
#7526=CIRCLE('',#19436,68.);
#7527=CIRCLE('',#19437,68.);
#7528=CIRCLE('',#19439,77.);
#7529=CIRCLE('',#19440,77.);
#7530=CIRCLE('',#19443,68.);
#7531=CIRCLE('',#19445,68.);
#7532=CIRCLE('',#19447,77.);
#7533=CIRCLE('',#19448,77.);
#7534=CIRCLE('',#19450,68.);
#7535=CIRCLE('',#19451,68.);
#7536=CIRCLE('',#19453,77.);
#7537=CIRCLE('',#19454,77.);
#7538=CIRCLE('',#19456,77.);
#7539=CIRCLE('',#19458,77.);
#7540=CIRCLE('',#19464,4.);
#7541=CIRCLE('',#19465,4.);
#7542=CIRCLE('',#19467,5.);
#7543=CIRCLE('',#19468,5.);
#7544=CIRCLE('',#19472,4.);
#7545=CIRCLE('',#19478,4.);
#7546=CIRCLE('',#19480,5.);
#7547=CIRCLE('',#19481,5.);
#7548=CIRCLE('',#19486,4.);
#7549=CIRCLE('',#19487,4.);
#7550=CIRCLE('',#19489,5.);
#7551=CIRCLE('',#19490,5.);
#7552=CIRCLE('',#19494,5.);
#7553=CIRCLE('',#19495,5.);
#7554=CIRCLE('',#19499,4.);
#7555=CIRCLE('',#19500,4.);
#7556=CIRCLE('',#19505,77.);
#7557=CIRCLE('',#19507,77.);
#7558=CIRCLE('',#19510,4.);
#7559=CIRCLE('',#19515,4.);
#7560=CIRCLE('',#19518,77.);
#7561=CIRCLE('',#19520,77.);
#7562=CIRCLE('',#19523,4.);
#7563=CIRCLE('',#19528,4.);
#7564=CIRCLE('',#19531,77.);
#7565=CIRCLE('',#19533,77.);
#7566=CIRCLE('',#19536,4.);
#7567=CIRCLE('',#19541,4.);
#7568=CIRCLE('',#19544,77.);
#7569=CIRCLE('',#19546,77.);
#7570=CIRCLE('',#19549,4.);
#7571=CIRCLE('',#19554,4.);
#7572=CIRCLE('',#19574,76.5);
#7573=CIRCLE('',#19575,68.);
#7574=CIRCLE('',#19576,68.);
#7575=CIRCLE('',#19579,68.);
#7576=CIRCLE('',#19582,76.5);
#7577=CIRCLE('',#19583,68.);
#7578=CIRCLE('',#19588,68.);
#7579=CIRCLE('',#19589,76.5);
#7580=CIRCLE('',#19592,68.);
#7581=CIRCLE('',#19595,68.);
#7582=CIRCLE('',#19596,76.5);
#7583=CIRCLE('',#19597,68.);
#7584=CIRCLE('',#19600,68.);
#7585=CIRCLE('',#19620,12.);
#7586=CIRCLE('',#19621,12.);
#7587=CIRCLE('',#19623,12.);
#7588=CIRCLE('',#19624,12.);
#7589=CIRCLE('',#19635,10.);
#7590=CIRCLE('',#19637,12.);
#7591=CIRCLE('',#19638,12.);
#7592=CIRCLE('',#19646,4.5);
#7593=CIRCLE('',#19652,12.);
#7594=CIRCLE('',#19655,12.);
#7595=CIRCLE('',#19657,12.);
#7596=CIRCLE('',#19660,12.);
#7597=CIRCLE('',#19662,12.);
#7598=CIRCLE('',#19663,12.);
#7599=CIRCLE('',#19665,12.);
#7600=CIRCLE('',#19668,12.);
#7601=CIRCLE('',#19670,12.);
#7602=CIRCLE('',#19673,12.);
#7603=CIRCLE('',#19683,2.);
#7604=CIRCLE('',#19685,2.);
#7605=CIRCLE('',#19705,6.);
#7606=CIRCLE('',#19707,10.);
#7607=CIRCLE('',#19708,10.);
#7608=CIRCLE('',#19710,2.5);
#7609=CIRCLE('',#19718,10.);
#7610=CIRCLE('',#19719,10.);
#7611=CIRCLE('',#19721,2.5);
#7612=CIRCLE('',#19735,2.);
#7613=CIRCLE('',#19737,2.);
#7614=CIRCLE('',#19746,6.00000000000001);
#7615=CIRCLE('',#19748,10.);
#7616=CIRCLE('',#19749,10.);
#7617=CIRCLE('',#19751,6.);
#7618=CIRCLE('',#19753,10.);
#7619=CIRCLE('',#19755,2.5);
#7620=CIRCLE('',#19765,6.00000000000001);
#7621=CIRCLE('',#19767,10.);
#7622=CIRCLE('',#19769,2.5);
#7623=CIRCLE('',#19796,12.);
#7624=CIRCLE('',#19800,12.);
#7625=CIRCLE('',#19806,6.00000000000001);
#7626=CIRCLE('',#19809,6.);
#7627=CIRCLE('',#19814,6.00000000000001);
#7628=CIRCLE('',#19818,6.00000000000001);
#7629=CIRCLE('',#19820,6.00000000000001);
#7630=CIRCLE('',#19822,6.);
#7631=CIRCLE('',#19841,12.);
#7632=CIRCLE('',#19843,12.);
#7633=CIRCLE('',#19847,6.);
#7634=CIRCLE('',#19848,6.);
#7635=CIRCLE('',#19851,6.);
#7636=CIRCLE('',#19852,6.);
#7637=CIRCLE('',#19856,12.);
#7638=CIRCLE('',#19858,12.);
#7639=CIRCLE('',#19860,105.377972911614);
#7640=CIRCLE('',#19861,20.5);
#7641=CIRCLE('',#19863,23.5);
#7642=CIRCLE('',#19864,23.5);
#7643=CIRCLE('',#19866,100.);
#7644=CIRCLE('',#19867,100.);
#7645=CIRCLE('',#19868,100.);
#7646=CIRCLE('',#19869,100.);
#7647=CIRCLE('',#19870,20.5);
#7648=CIRCLE('',#19873,106.259607815157);
#7649=CIRCLE('',#19890,12.);
#7650=CIRCLE('',#19892,12.);
#7651=CIRCLE('',#19894,12.);
#7652=CIRCLE('',#19903,12.);
#7653=CIRCLE('',#19905,107.1412427187);
#7654=CIRCLE('',#19907,107.1412427187);
#7655=CIRCLE('',#19909,107.1412427187);
#7656=CIRCLE('',#19911,107.1412427187);
#8122=VERTEX_POINT('',#30604);
#8123=VERTEX_POINT('',#30606);
#8124=VERTEX_POINT('',#30608);
#8125=VERTEX_POINT('',#30612);
#8126=VERTEX_POINT('',#30613);
#8127=VERTEX_POINT('',#30615);
#8128=VERTEX_POINT('',#30617);
#8129=VERTEX_POINT('',#30622);
#8130=VERTEX_POINT('',#30623);
#8131=VERTEX_POINT('',#30625);
#8132=VERTEX_POINT('',#30627);
#8133=VERTEX_POINT('',#30632);
#8134=VERTEX_POINT('',#30633);
#8135=VERTEX_POINT('',#30635);
#8136=VERTEX_POINT('',#30637);
#8137=VERTEX_POINT('',#30642);
#8138=VERTEX_POINT('',#30644);
#8139=VERTEX_POINT('',#30650);
#8140=VERTEX_POINT('',#30660);
#8141=VERTEX_POINT('',#30661);
#8142=VERTEX_POINT('',#30664);
#8143=VERTEX_POINT('',#30668);
#8144=VERTEX_POINT('',#30673);
#8145=VERTEX_POINT('',#30674);
#8146=VERTEX_POINT('',#30679);
#8147=VERTEX_POINT('',#30680);
#8148=VERTEX_POINT('',#30682);
#8149=VERTEX_POINT('',#30684);
#8150=VERTEX_POINT('',#30686);
#8151=VERTEX_POINT('',#30688);
#8152=VERTEX_POINT('',#30692);
#8153=VERTEX_POINT('',#30694);
#8154=VERTEX_POINT('',#30698);
#8155=VERTEX_POINT('',#30702);
#8156=VERTEX_POINT('',#30704);
#8157=VERTEX_POINT('',#30708);
#8158=VERTEX_POINT('',#30712);
#8159=VERTEX_POINT('',#30716);
#8160=VERTEX_POINT('',#30730);
#8161=VERTEX_POINT('',#30731);
#8162=VERTEX_POINT('',#30736);
#8163=VERTEX_POINT('',#30738);
#8164=VERTEX_POINT('',#30745);
#8165=VERTEX_POINT('',#30761);
#8166=VERTEX_POINT('',#30766);
#8167=VERTEX_POINT('',#30768);
#8168=VERTEX_POINT('',#30775);
#8169=VERTEX_POINT('',#30789);
#8170=VERTEX_POINT('',#30791);
#8171=VERTEX_POINT('',#30793);
#8172=VERTEX_POINT('',#30797);
#8173=VERTEX_POINT('',#30799);
#8174=VERTEX_POINT('',#30803);
#8175=VERTEX_POINT('',#30805);
#8176=VERTEX_POINT('',#30809);
#8177=VERTEX_POINT('',#30811);
#8178=VERTEX_POINT('',#30815);
#8179=VERTEX_POINT('',#30817);
#8180=VERTEX_POINT('',#30821);
#8181=VERTEX_POINT('',#30822);
#8182=VERTEX_POINT('',#30824);
#8183=VERTEX_POINT('',#30826);
#8184=VERTEX_POINT('',#30831);
#8185=VERTEX_POINT('',#30832);
#8186=VERTEX_POINT('',#30834);
#8187=VERTEX_POINT('',#30839);
#8188=VERTEX_POINT('',#30846);
#8189=VERTEX_POINT('',#30847);
#8190=VERTEX_POINT('',#30849);
#8191=VERTEX_POINT('',#30858);
#8192=VERTEX_POINT('',#30860);
#8193=VERTEX_POINT('',#30866);
#8194=VERTEX_POINT('',#30875);
#8195=VERTEX_POINT('',#30877);
#8196=VERTEX_POINT('',#30884);
#8197=VERTEX_POINT('',#30886);
#8198=VERTEX_POINT('',#30890);
#8199=VERTEX_POINT('',#30892);
#8200=VERTEX_POINT('',#30894);
#8201=VERTEX_POINT('',#30901);
#8202=VERTEX_POINT('',#30903);
#8203=VERTEX_POINT('',#30910);
#8204=VERTEX_POINT('',#30912);
#8205=VERTEX_POINT('',#30919);
#8206=VERTEX_POINT('',#30928);
#8207=VERTEX_POINT('',#30929);
#8208=VERTEX_POINT('',#30931);
#8209=VERTEX_POINT('',#30933);
#8210=VERTEX_POINT('',#30935);
#8211=VERTEX_POINT('',#30938);
#8212=VERTEX_POINT('',#30942);
#8213=VERTEX_POINT('',#30944);
#8214=VERTEX_POINT('',#30948);
#8215=VERTEX_POINT('',#30950);
#8216=VERTEX_POINT('',#30954);
#8217=VERTEX_POINT('',#30955);
#8218=VERTEX_POINT('',#30974);
#8219=VERTEX_POINT('',#30976);
#8220=VERTEX_POINT('',#30997);
#8221=VERTEX_POINT('',#30998);
#8222=VERTEX_POINT('',#31017);
#8223=VERTEX_POINT('',#31019);
#8224=VERTEX_POINT('',#31040);
#8225=VERTEX_POINT('',#31041);
#8226=VERTEX_POINT('',#31043);
#8227=VERTEX_POINT('',#31050);
#8228=VERTEX_POINT('',#31052);
#8229=VERTEX_POINT('',#31059);
#8230=VERTEX_POINT('',#31061);
#8231=VERTEX_POINT('',#31070);
#8232=VERTEX_POINT('',#31081);
#8233=VERTEX_POINT('',#31082);
#8234=VERTEX_POINT('',#31101);
#8235=VERTEX_POINT('',#31103);
#8236=VERTEX_POINT('',#31107);
#8237=VERTEX_POINT('',#31108);
#8238=VERTEX_POINT('',#31127);
#8239=VERTEX_POINT('',#31129);
#8240=VERTEX_POINT('',#31150);
#8241=VERTEX_POINT('',#31151);
#8242=VERTEX_POINT('',#31153);
#8243=VERTEX_POINT('',#31155);
#8244=VERTEX_POINT('',#31157);
#8245=VERTEX_POINT('',#31161);
#8246=VERTEX_POINT('',#31163);
#8247=VERTEX_POINT('',#31167);
#8248=VERTEX_POINT('',#31169);
#8249=VERTEX_POINT('',#31173);
#8250=VERTEX_POINT('',#31175);
#8251=VERTEX_POINT('',#31179);
#8252=VERTEX_POINT('',#31181);
#8253=VERTEX_POINT('',#31185);
#8254=VERTEX_POINT('',#31187);
#8255=VERTEX_POINT('',#31191);
#8256=VERTEX_POINT('',#31192);
#8257=VERTEX_POINT('',#31194);
#8258=VERTEX_POINT('',#31196);
#8259=VERTEX_POINT('',#31217);
#8260=VERTEX_POINT('',#31218);
#8261=VERTEX_POINT('',#31220);
#8262=VERTEX_POINT('',#31222);
#8263=VERTEX_POINT('',#31245);
#8264=VERTEX_POINT('',#31247);
#8265=VERTEX_POINT('',#31249);
#8266=VERTEX_POINT('',#31251);
#8267=VERTEX_POINT('',#31266);
#8268=VERTEX_POINT('',#31267);
#8269=VERTEX_POINT('',#31269);
#8270=VERTEX_POINT('',#31273);
#8271=VERTEX_POINT('',#31275);
#8272=VERTEX_POINT('',#31279);
#8273=VERTEX_POINT('',#31281);
#8274=VERTEX_POINT('',#31285);
#8275=VERTEX_POINT('',#31287);
#8276=VERTEX_POINT('',#31291);
#8277=VERTEX_POINT('',#31294);
#8278=VERTEX_POINT('',#31298);
#8279=VERTEX_POINT('',#31305);
#8280=VERTEX_POINT('',#31307);
#8281=VERTEX_POINT('',#31311);
#8282=VERTEX_POINT('',#31313);
#8283=VERTEX_POINT('',#31317);
#8284=VERTEX_POINT('',#31319);
#8285=VERTEX_POINT('',#31323);
#8286=VERTEX_POINT('',#31328);
#8287=VERTEX_POINT('',#31329);
#8288=VERTEX_POINT('',#31361);
#8289=VERTEX_POINT('',#31362);
#8290=VERTEX_POINT('',#31364);
#8291=VERTEX_POINT('',#31366);
#8292=VERTEX_POINT('',#31372);
#8293=VERTEX_POINT('',#31373);
#8294=VERTEX_POINT('',#31375);
#8295=VERTEX_POINT('',#31377);
#8296=VERTEX_POINT('',#31381);
#8297=VERTEX_POINT('',#31382);
#8298=VERTEX_POINT('',#31384);
#8299=VERTEX_POINT('',#31386);
#8300=VERTEX_POINT('',#31389);
#8301=VERTEX_POINT('',#31391);
#8302=VERTEX_POINT('',#31395);
#8303=VERTEX_POINT('',#31399);
#8304=VERTEX_POINT('',#31401);
#8305=VERTEX_POINT('',#31405);
#8306=VERTEX_POINT('',#31407);
#8307=VERTEX_POINT('',#31411);
#8308=VERTEX_POINT('',#31413);
#8309=VERTEX_POINT('',#31417);
#8310=VERTEX_POINT('',#31419);
#8311=VERTEX_POINT('',#31423);
#8312=VERTEX_POINT('',#31425);
#8313=VERTEX_POINT('',#31427);
#8314=VERTEX_POINT('',#31429);
#8315=VERTEX_POINT('',#31431);
#8316=VERTEX_POINT('',#31433);
#8317=VERTEX_POINT('',#31436);
#8318=VERTEX_POINT('',#31438);
#8319=VERTEX_POINT('',#31442);
#8320=VERTEX_POINT('',#31444);
#8321=VERTEX_POINT('',#31448);
#8322=VERTEX_POINT('',#31450);
#8323=VERTEX_POINT('',#31454);
#8324=VERTEX_POINT('',#31458);
#8325=VERTEX_POINT('',#31460);
#8326=VERTEX_POINT('',#31464);
#8327=VERTEX_POINT('',#31466);
#8328=VERTEX_POINT('',#31470);
#8329=VERTEX_POINT('',#31472);
#8330=VERTEX_POINT('',#31476);
#8331=VERTEX_POINT('',#31478);
#8332=VERTEX_POINT('',#31482);
#8333=VERTEX_POINT('',#31484);
#8334=VERTEX_POINT('',#31488);
#8335=VERTEX_POINT('',#31490);
#8336=VERTEX_POINT('',#31494);
#8337=VERTEX_POINT('',#31495);
#8338=VERTEX_POINT('',#31497);
#8339=VERTEX_POINT('',#31499);
#8340=VERTEX_POINT('',#31503);
#8341=VERTEX_POINT('',#31505);
#8342=VERTEX_POINT('',#31509);
#8343=VERTEX_POINT('',#31510);
#8344=VERTEX_POINT('',#31512);
#8345=VERTEX_POINT('',#31514);
#8346=VERTEX_POINT('',#31518);
#8347=VERTEX_POINT('',#31519);
#8348=VERTEX_POINT('',#31524);
#8349=VERTEX_POINT('',#31525);
#8350=VERTEX_POINT('',#31530);
#8351=VERTEX_POINT('',#31531);
#8352=VERTEX_POINT('',#31542);
#8353=VERTEX_POINT('',#31549);
#8354=VERTEX_POINT('',#31551);
#8355=VERTEX_POINT('',#31558);
#8356=VERTEX_POINT('',#31569);
#8357=VERTEX_POINT('',#31576);
#8358=VERTEX_POINT('',#31578);
#8359=VERTEX_POINT('',#31585);
#8360=VERTEX_POINT('',#31592);
#8361=VERTEX_POINT('',#31594);
#8362=VERTEX_POINT('',#31596);
#8363=VERTEX_POINT('',#31598);
#8364=VERTEX_POINT('',#31605);
#8365=VERTEX_POINT('',#31612);
#8366=VERTEX_POINT('',#31614);
#8367=VERTEX_POINT('',#31621);
#8368=VERTEX_POINT('',#31630);
#8369=VERTEX_POINT('',#31637);
#8370=VERTEX_POINT('',#31646);
#8371=VERTEX_POINT('',#31648);
#8372=VERTEX_POINT('',#31652);
#8373=VERTEX_POINT('',#31654);
#8374=VERTEX_POINT('',#31658);
#8375=VERTEX_POINT('',#31662);
#8376=VERTEX_POINT('',#31664);
#8377=VERTEX_POINT('',#31666);
#8378=VERTEX_POINT('',#31670);
#8379=VERTEX_POINT('',#31671);
#8380=VERTEX_POINT('',#31673);
#8381=VERTEX_POINT('',#31675);
#8382=VERTEX_POINT('',#31679);
#8383=VERTEX_POINT('',#31689);
#8384=VERTEX_POINT('',#31690);
#8385=VERTEX_POINT('',#31729);
#8386=VERTEX_POINT('',#31731);
#8387=VERTEX_POINT('',#31784);
#8388=VERTEX_POINT('',#31785);
#8389=VERTEX_POINT('',#31801);
#8390=VERTEX_POINT('',#31802);
#8391=VERTEX_POINT('',#31804);
#8392=VERTEX_POINT('',#31811);
#8393=VERTEX_POINT('',#31839);
#8394=VERTEX_POINT('',#31861);
#8395=VERTEX_POINT('',#31863);
#8396=VERTEX_POINT('',#31865);
#8397=VERTEX_POINT('',#31914);
#8398=VERTEX_POINT('',#31915);
#8399=VERTEX_POINT('',#31935);
#8400=VERTEX_POINT('',#31937);
#8401=VERTEX_POINT('',#31939);
#8402=VERTEX_POINT('',#31988);
#8403=VERTEX_POINT('',#31989);
#8404=VERTEX_POINT('',#32009);
#8405=VERTEX_POINT('',#32010);
#8406=VERTEX_POINT('',#32023);
#8407=VERTEX_POINT('',#32024);
#8408=VERTEX_POINT('',#32026);
#8409=VERTEX_POINT('',#32028);
#8410=VERTEX_POINT('',#32030);
#8411=VERTEX_POINT('',#32032);
#8412=VERTEX_POINT('',#32036);
#8413=VERTEX_POINT('',#32037);
#8414=VERTEX_POINT('',#32039);
#8415=VERTEX_POINT('',#32041);
#8416=VERTEX_POINT('',#32043);
#8417=VERTEX_POINT('',#32045);
#8418=VERTEX_POINT('',#32049);
#8419=VERTEX_POINT('',#32050);
#8420=VERTEX_POINT('',#32052);
#8421=VERTEX_POINT('',#32054);
#8422=VERTEX_POINT('',#32056);
#8423=VERTEX_POINT('',#32058);
#8424=VERTEX_POINT('',#32062);
#8425=VERTEX_POINT('',#32063);
#8426=VERTEX_POINT('',#32065);
#8427=VERTEX_POINT('',#32067);
#8428=VERTEX_POINT('',#32069);
#8429=VERTEX_POINT('',#32071);
#8430=VERTEX_POINT('',#32075);
#8431=VERTEX_POINT('',#32076);
#8432=VERTEX_POINT('',#32078);
#8433=VERTEX_POINT('',#32080);
#8434=VERTEX_POINT('',#32082);
#8435=VERTEX_POINT('',#32084);
#8436=VERTEX_POINT('',#32086);
#8437=VERTEX_POINT('',#32089);
#8438=VERTEX_POINT('',#32091);
#8439=VERTEX_POINT('',#32093);
#8440=VERTEX_POINT('',#32095);
#8441=VERTEX_POINT('',#32097);
#8442=VERTEX_POINT('',#32099);
#8443=VERTEX_POINT('',#32101);
#8444=VERTEX_POINT('',#32105);
#8445=VERTEX_POINT('',#32106);
#8446=VERTEX_POINT('',#32108);
#8447=VERTEX_POINT('',#32110);
#8448=VERTEX_POINT('',#32112);
#8449=VERTEX_POINT('',#32114);
#8450=VERTEX_POINT('',#32118);
#8451=VERTEX_POINT('',#32119);
#8452=VERTEX_POINT('',#32121);
#8453=VERTEX_POINT('',#32123);
#8454=VERTEX_POINT('',#32125);
#8455=VERTEX_POINT('',#32127);
#8456=VERTEX_POINT('',#32131);
#8457=VERTEX_POINT('',#32132);
#8458=VERTEX_POINT('',#32137);
#8459=VERTEX_POINT('',#32141);
#8460=VERTEX_POINT('',#32145);
#8461=VERTEX_POINT('',#32149);
#8462=VERTEX_POINT('',#32155);
#8463=VERTEX_POINT('',#32156);
#8464=VERTEX_POINT('',#32158);
#8465=VERTEX_POINT('',#32160);
#8466=VERTEX_POINT('',#32162);
#8467=VERTEX_POINT('',#32166);
#8468=VERTEX_POINT('',#32167);
#8469=VERTEX_POINT('',#32172);
#8470=VERTEX_POINT('',#32174);
#8471=VERTEX_POINT('',#32176);
#8472=VERTEX_POINT('',#32180);
#8473=VERTEX_POINT('',#32181);
#8474=VERTEX_POINT('',#32186);
#8475=VERTEX_POINT('',#32190);
#8476=VERTEX_POINT('',#32194);
#8477=VERTEX_POINT('',#32198);
#8478=VERTEX_POINT('',#32204);
#8479=VERTEX_POINT('',#32205);
#8480=VERTEX_POINT('',#32207);
#8481=VERTEX_POINT('',#32209);
#8482=VERTEX_POINT('',#32211);
#8483=VERTEX_POINT('',#32215);
#8484=VERTEX_POINT('',#32216);
#8485=VERTEX_POINT('',#32221);
#8486=VERTEX_POINT('',#32222);
#8487=VERTEX_POINT('',#32225);
#8488=VERTEX_POINT('',#32229);
#8489=VERTEX_POINT('',#32230);
#8490=VERTEX_POINT('',#32235);
#8491=VERTEX_POINT('',#32239);
#8492=VERTEX_POINT('',#32243);
#8493=VERTEX_POINT('',#32247);
#8494=VERTEX_POINT('',#32253);
#8495=VERTEX_POINT('',#32254);
#8496=VERTEX_POINT('',#32256);
#8497=VERTEX_POINT('',#32258);
#8498=VERTEX_POINT('',#32260);
#8499=VERTEX_POINT('',#32264);
#8500=VERTEX_POINT('',#32265);
#8501=VERTEX_POINT('',#32270);
#8502=VERTEX_POINT('',#32271);
#8503=VERTEX_POINT('',#32274);
#8504=VERTEX_POINT('',#32279);
#8505=VERTEX_POINT('',#32281);
#8506=VERTEX_POINT('',#32283);
#8507=VERTEX_POINT('',#32285);
#8508=VERTEX_POINT('',#32290);
#8509=VERTEX_POINT('',#32291);
#8510=VERTEX_POINT('',#32296);
#8511=VERTEX_POINT('',#32300);
#8512=VERTEX_POINT('',#32304);
#8513=VERTEX_POINT('',#32308);
#8514=VERTEX_POINT('',#32314);
#8515=VERTEX_POINT('',#32316);
#8516=VERTEX_POINT('',#32318);
#8517=VERTEX_POINT('',#32322);
#8518=VERTEX_POINT('',#32326);
#8519=VERTEX_POINT('',#32327);
#8520=VERTEX_POINT('',#32332);
#8521=VERTEX_POINT('',#32334);
#8522=VERTEX_POINT('',#32338);
#8523=VERTEX_POINT('',#32342);
#8524=VERTEX_POINT('',#32346);
#8525=VERTEX_POINT('',#32350);
#8526=VERTEX_POINT('',#32354);
#8527=VERTEX_POINT('',#32358);
#8528=VERTEX_POINT('',#32362);
#8529=VERTEX_POINT('',#32366);
#8530=VERTEX_POINT('',#32370);
#8531=VERTEX_POINT('',#32376);
#8532=VERTEX_POINT('',#32380);
#8533=VERTEX_POINT('',#32384);
#8534=VERTEX_POINT('',#32390);
#8535=VERTEX_POINT('',#32392);
#8536=VERTEX_POINT('',#32396);
#8537=VERTEX_POINT('',#32400);
#8538=VERTEX_POINT('',#32404);
#8539=VERTEX_POINT('',#32408);
#8540=VERTEX_POINT('',#32414);
#8541=VERTEX_POINT('',#32416);
#8542=VERTEX_POINT('',#32420);
#8543=VERTEX_POINT('',#32424);
#8544=VERTEX_POINT('',#32428);
#8545=VERTEX_POINT('',#32432);
#8546=VERTEX_POINT('',#32442);
#8547=VERTEX_POINT('',#32443);
#8548=VERTEX_POINT('',#32450);
#8549=VERTEX_POINT('',#32452);
#8550=VERTEX_POINT('',#32456);
#8551=VERTEX_POINT('',#32458);
#8552=VERTEX_POINT('',#32464);
#8553=VERTEX_POINT('',#32466);
#8554=VERTEX_POINT('',#32470);
#8555=VERTEX_POINT('',#32471);
#8556=VERTEX_POINT('',#32478);
#8557=VERTEX_POINT('',#32480);
#8558=VERTEX_POINT('',#32489);
#8559=VERTEX_POINT('',#32491);
#8560=VERTEX_POINT('',#32500);
#8561=VERTEX_POINT('',#32502);
#8562=VERTEX_POINT('',#32516);
#8563=VERTEX_POINT('',#32518);
#8564=VERTEX_POINT('',#32527);
#8565=VERTEX_POINT('',#32529);
#8566=VERTEX_POINT('',#32546);
#8567=VERTEX_POINT('',#32550);
#8568=VERTEX_POINT('',#32556);
#8569=VERTEX_POINT('',#32557);
#8570=VERTEX_POINT('',#32568);
#8571=VERTEX_POINT('',#32570);
#8572=VERTEX_POINT('',#32579);
#8573=VERTEX_POINT('',#32581);
#8574=VERTEX_POINT('',#32590);
#8575=VERTEX_POINT('',#32597);
#8576=VERTEX_POINT('',#32606);
#8577=VERTEX_POINT('',#32607);
#8578=VERTEX_POINT('',#32625);
#8579=VERTEX_POINT('',#32627);
#8580=VERTEX_POINT('',#32634);
#8581=VERTEX_POINT('',#32641);
#8582=VERTEX_POINT('',#32648);
#8583=VERTEX_POINT('',#32655);
#8584=VERTEX_POINT('',#32681);
#8585=VERTEX_POINT('',#32683);
#8586=VERTEX_POINT('',#32690);
#8587=VERTEX_POINT('',#32697);
#8588=VERTEX_POINT('',#32704);
#8589=VERTEX_POINT('',#32711);
#8590=VERTEX_POINT('',#32718);
#8591=VERTEX_POINT('',#32725);
#8592=VERTEX_POINT('',#32732);
#8593=VERTEX_POINT('',#32738);
#8594=VERTEX_POINT('',#32743);
#8595=VERTEX_POINT('',#32745);
#8596=VERTEX_POINT('',#32752);
#8597=VERTEX_POINT('',#32759);
#8598=VERTEX_POINT('',#32766);
#8599=VERTEX_POINT('',#32773);
#8600=VERTEX_POINT('',#32780);
#8601=VERTEX_POINT('',#32787);
#8602=VERTEX_POINT('',#32794);
#8603=VERTEX_POINT('',#32802);
#8604=VERTEX_POINT('',#32830);
#8605=VERTEX_POINT('',#32832);
#8606=VERTEX_POINT('',#32841);
#8607=VERTEX_POINT('',#32850);
#8608=VERTEX_POINT('',#32857);
#8609=VERTEX_POINT('',#32866);
#8610=VERTEX_POINT('',#32885);
#8611=VERTEX_POINT('',#32886);
#8612=VERTEX_POINT('',#32891);
#8613=VERTEX_POINT('',#32895);
#8614=VERTEX_POINT('',#32899);
#8615=VERTEX_POINT('',#32903);
#8616=VERTEX_POINT('',#32907);
#8617=VERTEX_POINT('',#32911);
#8618=VERTEX_POINT('',#33018);
#8619=VERTEX_POINT('',#33034);
#8620=VERTEX_POINT('',#33035);
#8621=VERTEX_POINT('',#33057);
#8622=VERTEX_POINT('',#33073);
#8623=VERTEX_POINT('',#33084);
#8624=VERTEX_POINT('',#33085);
#8625=VERTEX_POINT('',#33101);
#8626=VERTEX_POINT('',#33123);
#8627=VERTEX_POINT('',#33136);
#8628=VERTEX_POINT('',#33137);
#8629=VERTEX_POINT('',#33153);
#8630=VERTEX_POINT('',#33175);
#8631=VERTEX_POINT('',#33188);
#8632=VERTEX_POINT('',#33189);
#8633=VERTEX_POINT('',#33205);
#8634=VERTEX_POINT('',#33543);
#8635=VERTEX_POINT('',#33555);
#8636=VERTEX_POINT('',#33556);
#8637=VERTEX_POINT('',#33634);
#8638=VERTEX_POINT('',#33706);
#8639=VERTEX_POINT('',#33715);
#8640=VERTEX_POINT('',#33716);
#8641=VERTEX_POINT('',#33788);
#8642=VERTEX_POINT('',#33866);
#8643=VERTEX_POINT('',#33875);
#8644=VERTEX_POINT('',#33876);
#8645=VERTEX_POINT('',#33948);
#8646=VERTEX_POINT('',#34026);
#8647=VERTEX_POINT('',#34035);
#8648=VERTEX_POINT('',#34036);
#8649=VERTEX_POINT('',#34108);
#8650=VERTEX_POINT('',#34167);
#8651=VERTEX_POINT('',#35883);
#8652=VERTEX_POINT('',#35966);
#8653=VERTEX_POINT('',#35989);
#8654=VERTEX_POINT('',#35990);
#8655=VERTEX_POINT('',#36014);
#8656=VERTEX_POINT('',#36043);
#8657=VERTEX_POINT('',#36059);
#8658=VERTEX_POINT('',#36060);
#8659=VERTEX_POINT('',#36077);
#8660=VERTEX_POINT('',#36093);
#8661=VERTEX_POINT('',#36106);
#8662=VERTEX_POINT('',#36107);
#8663=VERTEX_POINT('',#36123);
#8664=VERTEX_POINT('',#36145);
#8665=VERTEX_POINT('',#36158);
#8666=VERTEX_POINT('',#36159);
#8667=VERTEX_POINT('',#36175);
#8668=VERTEX_POINT('',#36197);
#8669=VERTEX_POINT('',#36230);
#8670=VERTEX_POINT('',#36231);
#8671=VERTEX_POINT('',#36233);
#8672=VERTEX_POINT('',#36235);
#8673=VERTEX_POINT('',#36237);
#8674=VERTEX_POINT('',#36239);
#8675=VERTEX_POINT('',#36241);
#8676=VERTEX_POINT('',#36243);
#8677=VERTEX_POINT('',#36247);
#8678=VERTEX_POINT('',#36248);
#8679=VERTEX_POINT('',#36253);
#8680=VERTEX_POINT('',#36257);
#8681=VERTEX_POINT('',#36261);
#8682=VERTEX_POINT('',#36265);
#8683=VERTEX_POINT('',#36269);
#8684=VERTEX_POINT('',#36275);
#8685=VERTEX_POINT('',#36279);
#8686=VERTEX_POINT('',#36283);
#8687=VERTEX_POINT('',#36290);
#8688=VERTEX_POINT('',#36294);
#8689=VERTEX_POINT('',#36298);
#8690=VERTEX_POINT('',#36302);
#8691=VERTEX_POINT('',#36308);
#8692=VERTEX_POINT('',#36310);
#8693=VERTEX_POINT('',#36314);
#8694=VERTEX_POINT('',#36316);
#8695=VERTEX_POINT('',#36320);
#8696=VERTEX_POINT('',#36327);
#8697=VERTEX_POINT('',#36336);
#8698=VERTEX_POINT('',#36338);
#8699=VERTEX_POINT('',#36342);
#8700=VERTEX_POINT('',#36349);
#8701=VERTEX_POINT('',#36358);
#8702=VERTEX_POINT('',#36365);
#8703=VERTEX_POINT('',#36367);
#8704=VERTEX_POINT('',#36376);
#8705=VERTEX_POINT('',#36378);
#8706=VERTEX_POINT('',#36385);
#8707=VERTEX_POINT('',#36443);
#8708=VERTEX_POINT('',#36444);
#8709=VERTEX_POINT('',#36451);
#8710=VERTEX_POINT('',#36453);
#8711=VERTEX_POINT('',#36517);
#8712=VERTEX_POINT('',#36519);
#8713=VERTEX_POINT('',#36591);
#8714=VERTEX_POINT('',#36598);
#8715=VERTEX_POINT('',#36662);
#8716=VERTEX_POINT('',#36663);
#8717=VERTEX_POINT('',#36665);
#8718=VERTEX_POINT('',#36667);
#8719=VERTEX_POINT('',#36736);
#8720=VERTEX_POINT('',#36737);
#8721=VERTEX_POINT('',#36810);
#8722=VERTEX_POINT('',#36817);
#8723=VERTEX_POINT('',#36881);
#8724=VERTEX_POINT('',#36882);
#8725=VERTEX_POINT('',#36884);
#8726=VERTEX_POINT('',#36886);
#8727=VERTEX_POINT('',#36956);
#8728=VERTEX_POINT('',#36957);
#8729=VERTEX_POINT('',#37030);
#8730=VERTEX_POINT('',#37032);
#8731=VERTEX_POINT('',#37096);
#8732=VERTEX_POINT('',#37097);
#8733=VERTEX_POINT('',#37099);
#8734=VERTEX_POINT('',#37101);
#8735=VERTEX_POINT('',#37165);
#8736=VERTEX_POINT('',#37167);
#8737=VERTEX_POINT('',#37239);
#8738=VERTEX_POINT('',#37246);
#8739=VERTEX_POINT('',#37264);
#8740=VERTEX_POINT('',#37266);
#8741=VERTEX_POINT('',#37269);
#8742=VERTEX_POINT('',#37271);
#8743=VERTEX_POINT('',#37274);
#8744=VERTEX_POINT('',#37276);
#8745=VERTEX_POINT('',#37281);
#8746=VERTEX_POINT('',#37282);
#8747=VERTEX_POINT('',#37284);
#8748=VERTEX_POINT('',#37286);
#8749=VERTEX_POINT('',#37288);
#8750=VERTEX_POINT('',#37290);
#8751=VERTEX_POINT('',#37294);
#8752=VERTEX_POINT('',#37295);
#8753=VERTEX_POINT('',#37297);
#8754=VERTEX_POINT('',#37299);
#8755=VERTEX_POINT('',#37301);
#8756=VERTEX_POINT('',#37303);
#8757=VERTEX_POINT('',#37315);
#8758=VERTEX_POINT('',#37316);
#8759=VERTEX_POINT('',#37324);
#8760=VERTEX_POINT('',#37328);
#8761=VERTEX_POINT('',#37332);
#8762=VERTEX_POINT('',#37339);
#8763=VERTEX_POINT('',#37343);
#8764=VERTEX_POINT('',#37347);
#8765=VERTEX_POINT('',#37354);
#8766=VERTEX_POINT('',#37358);
#8767=VERTEX_POINT('',#37362);
#8768=VERTEX_POINT('',#37371);
#8769=VERTEX_POINT('',#37378);
#8770=VERTEX_POINT('',#37382);
#8771=VERTEX_POINT('',#37386);
#8772=VERTEX_POINT('',#37393);
#8773=VERTEX_POINT('',#37397);
#8774=VERTEX_POINT('',#37401);
#8775=VERTEX_POINT('',#37408);
#8776=VERTEX_POINT('',#37412);
#8777=VERTEX_POINT('',#37416);
#8778=VERTEX_POINT('',#37423);
#8779=VERTEX_POINT('',#37429);
#8780=VERTEX_POINT('',#37431);
#8781=VERTEX_POINT('',#37435);
#8782=VERTEX_POINT('',#37439);
#8783=VERTEX_POINT('',#37443);
#8784=VERTEX_POINT('',#37447);
#8785=VERTEX_POINT('',#37453);
#8786=VERTEX_POINT('',#37455);
#8787=VERTEX_POINT('',#37459);
#8788=VERTEX_POINT('',#37463);
#8789=VERTEX_POINT('',#37467);
#8790=VERTEX_POINT('',#37471);
#8791=VERTEX_POINT('',#37477);
#8792=VERTEX_POINT('',#37478);
#8793=VERTEX_POINT('',#37480);
#8794=VERTEX_POINT('',#37482);
#8795=VERTEX_POINT('',#37486);
#8796=VERTEX_POINT('',#37487);
#8797=VERTEX_POINT('',#37489);
#8798=VERTEX_POINT('',#37491);
#8799=VERTEX_POINT('',#37495);
#8800=VERTEX_POINT('',#37496);
#8801=VERTEX_POINT('',#37498);
#8802=VERTEX_POINT('',#37500);
#8803=VERTEX_POINT('',#37504);
#8804=VERTEX_POINT('',#37505);
#8805=VERTEX_POINT('',#37507);
#8806=VERTEX_POINT('',#37509);
#8807=VERTEX_POINT('',#37514);
#8808=VERTEX_POINT('',#37516);
#8809=VERTEX_POINT('',#37520);
#8810=VERTEX_POINT('',#37521);
#8811=VERTEX_POINT('',#37523);
#8812=VERTEX_POINT('',#37525);
#8813=VERTEX_POINT('',#37529);
#8814=VERTEX_POINT('',#37530);
#8815=VERTEX_POINT('',#37532);
#8816=VERTEX_POINT('',#37534);
#8817=VERTEX_POINT('',#37538);
#8818=VERTEX_POINT('',#37539);
#8819=VERTEX_POINT('',#37541);
#8820=VERTEX_POINT('',#37543);
#8821=VERTEX_POINT('',#37552);
#8822=VERTEX_POINT('',#37554);
#8823=VERTEX_POINT('',#37559);
#8824=VERTEX_POINT('',#37560);
#8825=VERTEX_POINT('',#37567);
#8826=VERTEX_POINT('',#37569);
#8827=VERTEX_POINT('',#37573);
#8828=VERTEX_POINT('',#37575);
#8829=VERTEX_POINT('',#37579);
#8830=VERTEX_POINT('',#37581);
#8831=VERTEX_POINT('',#37583);
#8832=VERTEX_POINT('',#37585);
#8833=VERTEX_POINT('',#37587);
#8834=VERTEX_POINT('',#37589);
#8835=VERTEX_POINT('',#37593);
#8836=VERTEX_POINT('',#37594);
#8837=VERTEX_POINT('',#37596);
#8838=VERTEX_POINT('',#37598);
#8839=VERTEX_POINT('',#37602);
#8840=VERTEX_POINT('',#37604);
#8841=VERTEX_POINT('',#37606);
#8842=VERTEX_POINT('',#37613);
#8843=VERTEX_POINT('',#37614);
#8844=VERTEX_POINT('',#37616);
#8845=VERTEX_POINT('',#37621);
#8846=VERTEX_POINT('',#37625);
#8847=VERTEX_POINT('',#37626);
#8848=VERTEX_POINT('',#37629);
#8849=VERTEX_POINT('',#37633);
#8850=VERTEX_POINT('',#37635);
#8851=VERTEX_POINT('',#37639);
#8852=VERTEX_POINT('',#37640);
#8853=VERTEX_POINT('',#37645);
#8854=VERTEX_POINT('',#37647);
#8855=VERTEX_POINT('',#37651);
#8856=VERTEX_POINT('',#37652);
#8857=VERTEX_POINT('',#37654);
#8858=VERTEX_POINT('',#37656);
#8859=VERTEX_POINT('',#37660);
#8860=VERTEX_POINT('',#37662);
#8861=VERTEX_POINT('',#37669);
#8862=VERTEX_POINT('',#37671);
#8863=VERTEX_POINT('',#37675);
#8864=VERTEX_POINT('',#37677);
#8865=VERTEX_POINT('',#37679);
#8866=VERTEX_POINT('',#37681);
#8867=VERTEX_POINT('',#37683);
#8868=VERTEX_POINT('',#37685);
#8869=VERTEX_POINT('',#37689);
#8870=VERTEX_POINT('',#37690);
#8871=VERTEX_POINT('',#37692);
#8872=VERTEX_POINT('',#37694);
#8873=VERTEX_POINT('',#37698);
#8874=VERTEX_POINT('',#37700);
#8875=VERTEX_POINT('',#37707);
#8876=VERTEX_POINT('',#37708);
#8877=VERTEX_POINT('',#37710);
#8878=VERTEX_POINT('',#37712);
#8879=VERTEX_POINT('',#37717);
#8880=VERTEX_POINT('',#37721);
#8881=VERTEX_POINT('',#37725);
#8882=VERTEX_POINT('',#37727);
#8883=VERTEX_POINT('',#37729);
#8884=VERTEX_POINT('',#37731);
#8885=VERTEX_POINT('',#37733);
#8886=VERTEX_POINT('',#37735);
#8887=VERTEX_POINT('',#37739);
#8888=VERTEX_POINT('',#37740);
#8889=VERTEX_POINT('',#37742);
#8890=VERTEX_POINT('',#37744);
#8891=VERTEX_POINT('',#37746);
#8892=VERTEX_POINT('',#37748);
#8893=VERTEX_POINT('',#37752);
#8894=VERTEX_POINT('',#37753);
#8895=VERTEX_POINT('',#37755);
#8896=VERTEX_POINT('',#37757);
#8897=VERTEX_POINT('',#37762);
#8898=VERTEX_POINT('',#37763);
#8899=VERTEX_POINT('',#37766);
#8900=VERTEX_POINT('',#37768);
#8901=VERTEX_POINT('',#37772);
#8902=VERTEX_POINT('',#37774);
#8903=VERTEX_POINT('',#37778);
#8904=VERTEX_POINT('',#37780);
#8905=VERTEX_POINT('',#37784);
#8906=VERTEX_POINT('',#37788);
#8907=VERTEX_POINT('',#37792);
#8908=VERTEX_POINT('',#37796);
#8909=VERTEX_POINT('',#37800);
#8910=VERTEX_POINT('',#37804);
#8911=VERTEX_POINT('',#37806);
#8912=VERTEX_POINT('',#37810);
#8913=VERTEX_POINT('',#37812);
#8914=VERTEX_POINT('',#37814);
#8915=VERTEX_POINT('',#37818);
#8916=VERTEX_POINT('',#37820);
#8917=VERTEX_POINT('',#37824);
#8918=VERTEX_POINT('',#37826);
#8919=VERTEX_POINT('',#37830);
#8920=VERTEX_POINT('',#37834);
#8921=VERTEX_POINT('',#37838);
#8922=VERTEX_POINT('',#37842);
#8923=VERTEX_POINT('',#37846);
#8924=VERTEX_POINT('',#37850);
#8925=VERTEX_POINT('',#37852);
#8926=VERTEX_POINT('',#37856);
#8927=VERTEX_POINT('',#37858);
#8928=VERTEX_POINT('',#37860);
#8929=VERTEX_POINT('',#37864);
#8930=VERTEX_POINT('',#37866);
#8931=VERTEX_POINT('',#37870);
#8932=VERTEX_POINT('',#37872);
#8933=VERTEX_POINT('',#37876);
#8934=VERTEX_POINT('',#37880);
#8935=VERTEX_POINT('',#37884);
#8936=VERTEX_POINT('',#37888);
#8937=VERTEX_POINT('',#37892);
#8938=VERTEX_POINT('',#37896);
#8939=VERTEX_POINT('',#37898);
#8940=VERTEX_POINT('',#37902);
#8941=VERTEX_POINT('',#37904);
#8942=VERTEX_POINT('',#37906);
#8943=VERTEX_POINT('',#37910);
#8944=VERTEX_POINT('',#37912);
#8945=VERTEX_POINT('',#37916);
#8946=VERTEX_POINT('',#37918);
#8947=VERTEX_POINT('',#37922);
#8948=VERTEX_POINT('',#37926);
#8949=VERTEX_POINT('',#37930);
#8950=VERTEX_POINT('',#37934);
#8951=VERTEX_POINT('',#37938);
#8952=VERTEX_POINT('',#37942);
#8953=VERTEX_POINT('',#37946);
#8954=VERTEX_POINT('',#37948);
#8955=VERTEX_POINT('',#37952);
#8956=VERTEX_POINT('',#37956);
#8957=VERTEX_POINT('',#37960);
#8958=VERTEX_POINT('',#37964);
#8959=VERTEX_POINT('',#37984);
#8960=VERTEX_POINT('',#37986);
#8961=VERTEX_POINT('',#37990);
#8962=VERTEX_POINT('',#37991);
#8963=VERTEX_POINT('',#37993);
#8964=VERTEX_POINT('',#37995);
#8965=VERTEX_POINT('',#37998);
#8966=VERTEX_POINT('',#38002);
#8967=VERTEX_POINT('',#38006);
#8968=VERTEX_POINT('',#38010);
#8969=VERTEX_POINT('',#38014);
#8970=VERTEX_POINT('',#38016);
#8971=VERTEX_POINT('',#38018);
#8972=VERTEX_POINT('',#38029);
#8973=VERTEX_POINT('',#38031);
#8974=VERTEX_POINT('',#38033);
#8975=VERTEX_POINT('',#38035);
#8976=VERTEX_POINT('',#38039);
#8977=VERTEX_POINT('',#38043);
#8978=VERTEX_POINT('',#38047);
#8979=VERTEX_POINT('',#38051);
#8980=VERTEX_POINT('',#38053);
#8981=VERTEX_POINT('',#38055);
#8982=VERTEX_POINT('',#38057);
#8983=VERTEX_POINT('',#38059);
#8984=VERTEX_POINT('',#38063);
#8985=VERTEX_POINT('',#38070);
#8986=VERTEX_POINT('',#38071);
#8987=VERTEX_POINT('',#38073);
#8988=VERTEX_POINT('',#38075);
#8989=VERTEX_POINT('',#38077);
#8990=VERTEX_POINT('',#38079);
#8991=VERTEX_POINT('',#38112);
#8992=VERTEX_POINT('',#38113);
#8993=VERTEX_POINT('',#38115);
#8994=VERTEX_POINT('',#38117);
#8995=VERTEX_POINT('',#38119);
#8996=VERTEX_POINT('',#38121);
#8997=VERTEX_POINT('',#38123);
#8998=VERTEX_POINT('',#38125);
#8999=VERTEX_POINT('',#38132);
#9000=VERTEX_POINT('',#38134);
#9001=VERTEX_POINT('',#38138);
#9002=VERTEX_POINT('',#38139);
#9003=VERTEX_POINT('',#38141);
#9004=VERTEX_POINT('',#38143);
#9005=VERTEX_POINT('',#38145);
#9006=VERTEX_POINT('',#38147);
#9007=VERTEX_POINT('',#38152);
#9008=VERTEX_POINT('',#38153);
#9009=VERTEX_POINT('',#38155);
#9010=VERTEX_POINT('',#38157);
#9011=VERTEX_POINT('',#38159);
#9012=VERTEX_POINT('',#38161);
#9013=VERTEX_POINT('',#38176);
#9014=VERTEX_POINT('',#38178);
#9015=VERTEX_POINT('',#38182);
#9016=VERTEX_POINT('',#38186);
#9017=VERTEX_POINT('',#38190);
#9018=VERTEX_POINT('',#38194);
#9019=VERTEX_POINT('',#38200);
#9020=VERTEX_POINT('',#38202);
#9021=VERTEX_POINT('',#38214);
#9022=VERTEX_POINT('',#38215);
#9023=VERTEX_POINT('',#38222);
#9024=VERTEX_POINT('',#38223);
#9025=VERTEX_POINT('',#38225);
#9026=VERTEX_POINT('',#38227);
#9027=VERTEX_POINT('',#38229);
#9028=VERTEX_POINT('',#38231);
#9029=VERTEX_POINT('',#38235);
#9030=VERTEX_POINT('',#38236);
#9031=VERTEX_POINT('',#38238);
#9032=VERTEX_POINT('',#38240);
#9033=VERTEX_POINT('',#38242);
#9034=VERTEX_POINT('',#38244);
#9035=VERTEX_POINT('',#38248);
#9036=VERTEX_POINT('',#38249);
#9037=VERTEX_POINT('',#38251);
#9038=VERTEX_POINT('',#38253);
#9039=VERTEX_POINT('',#38255);
#9040=VERTEX_POINT('',#38257);
#9041=VERTEX_POINT('',#38261);
#9042=VERTEX_POINT('',#38265);
#9043=VERTEX_POINT('',#38271);
#9044=VERTEX_POINT('',#38275);
#9045=VERTEX_POINT('',#38284);
#9046=VERTEX_POINT('',#38288);
#9047=VERTEX_POINT('',#38294);
#9048=VERTEX_POINT('',#38298);
#9049=VERTEX_POINT('',#38304);
#9050=VERTEX_POINT('',#38306);
#9051=VERTEX_POINT('',#38310);
#9052=VERTEX_POINT('',#38314);
#9053=VERTEX_POINT('',#38318);
#9054=VERTEX_POINT('',#38322);
#9055=VERTEX_POINT('',#38328);
#9056=VERTEX_POINT('',#38330);
#9057=VERTEX_POINT('',#38334);
#9058=VERTEX_POINT('',#38343);
#9059=VERTEX_POINT('',#38345);
#9060=VERTEX_POINT('',#38349);
#9061=VERTEX_POINT('',#38358);
#9062=VERTEX_POINT('',#38362);
#9063=VERTEX_POINT('',#38363);
#9064=VERTEX_POINT('',#38365);
#9065=VERTEX_POINT('',#38367);
#9066=VERTEX_POINT('',#38369);
#9067=VERTEX_POINT('',#38371);
#9068=VERTEX_POINT('',#38375);
#9069=VERTEX_POINT('',#38376);
#9070=VERTEX_POINT('',#38378);
#9071=VERTEX_POINT('',#38380);
#9072=VERTEX_POINT('',#38382);
#9073=VERTEX_POINT('',#38384);
#9074=VERTEX_POINT('',#38388);
#9075=VERTEX_POINT('',#38389);
#9076=VERTEX_POINT('',#38391);
#9077=VERTEX_POINT('',#38393);
#9078=VERTEX_POINT('',#38395);
#9079=VERTEX_POINT('',#38397);
#9080=VERTEX_POINT('',#38401);
#9081=VERTEX_POINT('',#38405);
#9082=VERTEX_POINT('',#38411);
#9083=VERTEX_POINT('',#38412);
#9084=VERTEX_POINT('',#38414);
#9085=VERTEX_POINT('',#38416);
#9086=VERTEX_POINT('',#38418);
#9087=VERTEX_POINT('',#38420);
#9088=VERTEX_POINT('',#38424);
#9089=VERTEX_POINT('',#38425);
#9090=VERTEX_POINT('',#38427);
#9091=VERTEX_POINT('',#38429);
#9092=VERTEX_POINT('',#38431);
#9093=VERTEX_POINT('',#38433);
#9094=VERTEX_POINT('',#38437);
#9095=VERTEX_POINT('',#38439);
#9096=VERTEX_POINT('',#38443);
#9097=VERTEX_POINT('',#38447);
#9098=VERTEX_POINT('',#38451);
#9099=VERTEX_POINT('',#38455);
#9100=VERTEX_POINT('',#38461);
#9101=VERTEX_POINT('',#38462);
#9102=VERTEX_POINT('',#38464);
#9103=VERTEX_POINT('',#38468);
#9104=VERTEX_POINT('',#38469);
#9105=VERTEX_POINT('',#38474);
#9106=VERTEX_POINT('',#38476);
#9107=VERTEX_POINT('',#38478);
#9108=VERTEX_POINT('',#38482);
#9109=VERTEX_POINT('',#38484);
#9110=VERTEX_POINT('',#38488);
#9111=VERTEX_POINT('',#38492);
#9112=VERTEX_POINT('',#38496);
#9113=VERTEX_POINT('',#38500);
#9114=VERTEX_POINT('',#38506);
#9115=VERTEX_POINT('',#38507);
#9116=VERTEX_POINT('',#38509);
#9117=VERTEX_POINT('',#38511);
#9118=VERTEX_POINT('',#38515);
#9119=VERTEX_POINT('',#38517);
#9120=VERTEX_POINT('',#38519);
#9121=VERTEX_POINT('',#38523);
#9122=VERTEX_POINT('',#38525);
#9123=VERTEX_POINT('',#38529);
#9124=VERTEX_POINT('',#38533);
#9125=VERTEX_POINT('',#38537);
#9126=VERTEX_POINT('',#38541);
#9127=VERTEX_POINT('',#38547);
#9128=VERTEX_POINT('',#38548);
#9129=VERTEX_POINT('',#38563);
#9130=VERTEX_POINT('',#38576);
#9131=VERTEX_POINT('',#38590);
#9132=VERTEX_POINT('',#38601);
#9133=VERTEX_POINT('',#38603);
#9134=VERTEX_POINT('',#38615);
#9135=VERTEX_POINT('',#38616);
#9136=VERTEX_POINT('',#38621);
#9137=VERTEX_POINT('',#38630);
#9138=VERTEX_POINT('',#38631);
#9139=VERTEX_POINT('',#38636);
#9140=VERTEX_POINT('',#38647);
#9141=VERTEX_POINT('',#38660);
#9142=VERTEX_POINT('',#38674);
#9143=VERTEX_POINT('',#38687);
#9144=VERTEX_POINT('',#38701);
#9145=VERTEX_POINT('',#38708);
#9146=VERTEX_POINT('',#38721);
#9147=VERTEX_POINT('',#38742);
#9148=VERTEX_POINT('',#38743);
#9149=VERTEX_POINT('',#38787);
#9150=VERTEX_POINT('',#38844);
#9151=VERTEX_POINT('',#38845);
#9152=VERTEX_POINT('',#38847);
#9153=VERTEX_POINT('',#38849);
#9154=VERTEX_POINT('',#38851);
#9155=VERTEX_POINT('',#38854);
#9156=VERTEX_POINT('',#38858);
#9157=VERTEX_POINT('',#38859);
#9158=VERTEX_POINT('',#38864);
#9159=VERTEX_POINT('',#38868);
#9160=VERTEX_POINT('',#38870);
#9161=VERTEX_POINT('',#38874);
#9162=VERTEX_POINT('',#38876);
#9163=VERTEX_POINT('',#38881);
#9164=VERTEX_POINT('',#38883);
#9165=VERTEX_POINT('',#38887);
#9166=VERTEX_POINT('',#38891);
#9167=VERTEX_POINT('',#38895);
#9168=VERTEX_POINT('',#38899);
#9169=VERTEX_POINT('',#38922);
#9170=VERTEX_POINT('',#38979);
#9171=VERTEX_POINT('',#38981);
#9172=VERTEX_POINT('',#38985);
#9173=VERTEX_POINT('',#38989);
#9174=VERTEX_POINT('',#38991);
#9175=VERTEX_POINT('',#38995);
#9176=VERTEX_POINT('',#38997);
#9177=VERTEX_POINT('',#39001);
#9178=VERTEX_POINT('',#39005);
#9179=VERTEX_POINT('',#39009);
#9180=VERTEX_POINT('',#39013);
#9181=VERTEX_POINT('',#39019);
#9182=VERTEX_POINT('',#39021);
#9183=VERTEX_POINT('',#39025);
#9184=VERTEX_POINT('',#39029);
#9185=VERTEX_POINT('',#39033);
#9186=VERTEX_POINT('',#39037);
#9187=VERTEX_POINT('',#39044);
#9188=VERTEX_POINT('',#39045);
#9189=VERTEX_POINT('',#39047);
#9190=VERTEX_POINT('',#39049);
#9191=VERTEX_POINT('',#39051);
#9192=VERTEX_POINT('',#39053);
#9193=VERTEX_POINT('',#39058);
#9194=VERTEX_POINT('',#39059);
#9195=VERTEX_POINT('',#39061);
#9196=VERTEX_POINT('',#39063);
#9197=VERTEX_POINT('',#39065);
#9198=VERTEX_POINT('',#39067);
#9199=VERTEX_POINT('',#39071);
#9200=VERTEX_POINT('',#39072);
#9201=VERTEX_POINT('',#39077);
#9202=VERTEX_POINT('',#39079);
#9203=VERTEX_POINT('',#39081);
#9204=VERTEX_POINT('',#39083);
#9205=VERTEX_POINT('',#39087);
#9206=VERTEX_POINT('',#39088);
#9207=VERTEX_POINT('',#39093);
#9208=VERTEX_POINT('',#39095);
#9209=VERTEX_POINT('',#39099);
#9210=VERTEX_POINT('',#39103);
#9211=VERTEX_POINT('',#39107);
#9212=VERTEX_POINT('',#39111);
#9213=VERTEX_POINT('',#39117);
#9214=VERTEX_POINT('',#39118);
#9215=VERTEX_POINT('',#39120);
#9216=VERTEX_POINT('',#39123);
#9217=VERTEX_POINT('',#39127);
#9218=VERTEX_POINT('',#39131);
#9219=VERTEX_POINT('',#39135);
#9220=VERTEX_POINT('',#39137);
#9221=VERTEX_POINT('',#39139);
#9222=VERTEX_POINT('',#39143);
#9223=VERTEX_POINT('',#39152);
#9224=VERTEX_POINT('',#39173);
#9225=VERTEX_POINT('',#39174);
#9226=VERTEX_POINT('',#39181);
#9227=VERTEX_POINT('',#39234);
#9228=VERTEX_POINT('',#39238);
#9229=VERTEX_POINT('',#39240);
#9230=VERTEX_POINT('',#39261);
#9231=VERTEX_POINT('',#39318);
#9232=VERTEX_POINT('',#39320);
#9233=VERTEX_POINT('',#39324);
#9234=VERTEX_POINT('',#39325);
#9235=VERTEX_POINT('',#39330);
#9236=VERTEX_POINT('',#39336);
#9237=VERTEX_POINT('',#39340);
#9238=VERTEX_POINT('',#39344);
#9239=VERTEX_POINT('',#39349);
#9240=VERTEX_POINT('',#39351);
#9241=VERTEX_POINT('',#39355);
#9242=VERTEX_POINT('',#39359);
#9243=VERTEX_POINT('',#39363);
#9244=VERTEX_POINT('',#39367);
#9245=VERTEX_POINT('',#39377);
#9246=VERTEX_POINT('',#39378);
#9247=VERTEX_POINT('',#39383);
#9248=VERTEX_POINT('',#39387);
#9249=VERTEX_POINT('',#39401);
#9250=VERTEX_POINT('',#39402);
#9251=VERTEX_POINT('',#39406);
#9252=VERTEX_POINT('',#39407);
#9253=VERTEX_POINT('',#39413);
#9254=VERTEX_POINT('',#39417);
#9255=VERTEX_POINT('',#39418);
#9256=VERTEX_POINT('',#39423);
#9257=VERTEX_POINT('',#39427);
#9258=VERTEX_POINT('',#39428);
#9259=VERTEX_POINT('',#39438);
#9260=VERTEX_POINT('',#39439);
#9261=VERTEX_POINT('',#39443);
#9262=VERTEX_POINT('',#39444);
#9263=VERTEX_POINT('',#39448);
#9264=VERTEX_POINT('',#39452);
#9265=VERTEX_POINT('',#39454);
#9266=VERTEX_POINT('',#39465);
#9267=VERTEX_POINT('',#39467);
#9268=VERTEX_POINT('',#39469);
#9269=VERTEX_POINT('',#39471);
#9270=VERTEX_POINT('',#39487);
#9271=VERTEX_POINT('',#39488);
#9272=VERTEX_POINT('',#39491);
#9273=VERTEX_POINT('',#39493);
#9274=VERTEX_POINT('',#39495);
#9275=VERTEX_POINT('',#39499);
#9276=VERTEX_POINT('',#39503);
#9277=VERTEX_POINT('',#39505);
#9278=VERTEX_POINT('',#39509);
#9279=VERTEX_POINT('',#39513);
#9280=VERTEX_POINT('',#39515);
#9281=VERTEX_POINT('',#39519);
#9282=VERTEX_POINT('',#39523);
#9283=VERTEX_POINT('',#39524);
#9284=VERTEX_POINT('',#39526);
#9285=VERTEX_POINT('',#39528);
#9286=VERTEX_POINT('',#39530);
#9287=VERTEX_POINT('',#39532);
#9288=VERTEX_POINT('',#39535);
#9289=VERTEX_POINT('',#39537);
#9290=VERTEX_POINT('',#39539);
#9291=VERTEX_POINT('',#39543);
#9292=VERTEX_POINT('',#39547);
#9293=VERTEX_POINT('',#39548);
#9294=VERTEX_POINT('',#39553);
#9295=VERTEX_POINT('',#39557);
#9296=VERTEX_POINT('',#39558);
#9297=VERTEX_POINT('',#39563);
#9298=VERTEX_POINT('',#39567);
#9299=VERTEX_POINT('',#39568);
#9300=VERTEX_POINT('',#39571);
#9301=VERTEX_POINT('',#39573);
#9302=VERTEX_POINT('',#39577);
#9303=VERTEX_POINT('',#39578);
#9304=VERTEX_POINT('',#39583);
#9305=VERTEX_POINT('',#39588);
#9306=VERTEX_POINT('',#39589);
#9307=VERTEX_POINT('',#39594);
#9308=VERTEX_POINT('',#39595);
#9309=VERTEX_POINT('',#39600);
#9310=VERTEX_POINT('',#39604);
#9311=VERTEX_POINT('',#39609);
#9312=VERTEX_POINT('',#39617);
#9313=VERTEX_POINT('',#39621);
#9314=VERTEX_POINT('',#39626);
#9315=VERTEX_POINT('',#39629);
#9316=VERTEX_POINT('',#39635);
#9317=VERTEX_POINT('',#39642);
#9318=VERTEX_POINT('',#39649);
#9319=VERTEX_POINT('',#39658);
#9320=VERTEX_POINT('',#39659);
#9321=VERTEX_POINT('',#39661);
#9322=VERTEX_POINT('',#39666);
#9323=VERTEX_POINT('',#39668);
#9324=VERTEX_POINT('',#39672);
#9325=VERTEX_POINT('',#39683);
#9326=VERTEX_POINT('',#39684);
#9327=VERTEX_POINT('',#39689);
#9328=VERTEX_POINT('',#39693);
#9329=VERTEX_POINT('',#39697);
#9330=VERTEX_POINT('',#39699);
#9331=VERTEX_POINT('',#39703);
#9332=VERTEX_POINT('',#39704);
#9333=VERTEX_POINT('',#39709);
#9334=VERTEX_POINT('',#39713);
#9335=VERTEX_POINT('',#39723);
#9336=VERTEX_POINT('',#39724);
#9337=VERTEX_POINT('',#39727);
#9338=VERTEX_POINT('',#39731);
#9339=VERTEX_POINT('',#39735);
#9340=VERTEX_POINT('',#39737);
#9341=VERTEX_POINT('',#39741);
#9342=VERTEX_POINT('',#39743);
#9343=VERTEX_POINT('',#39747);
#9344=VERTEX_POINT('',#39751);
#9345=VERTEX_POINT('',#39755);
#9346=VERTEX_POINT('',#39759);
#9347=VERTEX_POINT('',#39763);
#9348=VERTEX_POINT('',#39767);
#9349=VERTEX_POINT('',#39771);
#9350=VERTEX_POINT('',#39775);
#9351=VERTEX_POINT('',#39779);
#9352=VERTEX_POINT('',#39783);
#10065=EDGE_CURVE('',#8122,#8122,#7235,.T.);
#10066=EDGE_CURVE('',#8122,#8123,#7236,.T.);
#10067=EDGE_CURVE('',#8124,#8123,#7237,.T.);
#10068=EDGE_CURVE('',#8123,#8124,#7238,.T.);
#10069=EDGE_CURVE('',#8125,#8126,#7239,.T.);
#10070=EDGE_CURVE('',#8125,#8127,#7240,.T.);
#10071=EDGE_CURVE('',#8127,#8128,#7241,.T.);
#10072=EDGE_CURVE('',#8128,#8127,#7242,.T.);
#10073=EDGE_CURVE('',#8126,#8125,#7243,.T.);
#10074=EDGE_CURVE('',#8129,#8130,#7244,.T.);
#10075=EDGE_CURVE('',#8129,#8131,#7245,.T.);
#10076=EDGE_CURVE('',#8131,#8132,#7246,.T.);
#10077=EDGE_CURVE('',#8132,#8131,#7247,.T.);
#10078=EDGE_CURVE('',#8130,#8129,#7248,.T.);
#10079=EDGE_CURVE('',#8133,#8134,#7249,.T.);
#10080=EDGE_CURVE('',#8133,#8135,#7250,.T.);
#10081=EDGE_CURVE('',#8136,#8135,#7251,.T.);
#10082=EDGE_CURVE('',#8135,#8136,#7252,.T.);
#10083=EDGE_CURVE('',#8134,#8133,#7253,.T.);
#10084=EDGE_CURVE('',#8137,#8137,#7254,.T.);
#10085=EDGE_CURVE('',#8137,#8138,#1790,.T.);
#10086=EDGE_CURVE('',#8138,#8138,#7255,.T.);
#10087=EDGE_CURVE('',#8126,#8124,#1791,.T.);
#10088=EDGE_CURVE('',#8132,#8139,#1792,.T.);
#10089=EDGE_CURVE('',#8139,#8139,#7256,.T.);
#10090=EDGE_CURVE('',#8134,#8128,#1793,.T.);
#10091=EDGE_CURVE('',#8130,#8136,#1794,.T.);
#10092=EDGE_CURVE('',#8140,#8141,#7257,.T.);
#10093=EDGE_CURVE('',#8141,#8140,#7258,.T.);
#10094=EDGE_CURVE('',#8140,#8142,#1795,.T.);
#10095=EDGE_CURVE('',#8142,#8142,#7259,.T.);
#10096=EDGE_CURVE('',#8141,#8143,#1796,.T.);
#10097=EDGE_CURVE('',#8143,#8143,#7260,.T.);
#10098=EDGE_CURVE('',#8144,#8145,#1797,.T.);
#10099=EDGE_CURVE('',#8145,#8145,#7261,.T.);
#10100=EDGE_CURVE('',#8146,#8147,#1798,.T.);
#10101=EDGE_CURVE('',#8147,#8148,#1799,.T.);
#10102=EDGE_CURVE('',#8148,#8149,#1800,.T.);
#10103=EDGE_CURVE('',#8149,#8150,#1801,.T.);
#10104=EDGE_CURVE('',#8150,#8151,#1802,.T.);
#10105=EDGE_CURVE('',#8151,#8146,#1803,.T.);
#10106=EDGE_CURVE('',#8148,#8152,#1804,.T.);
#10107=EDGE_CURVE('',#8153,#8147,#1805,.T.);
#10108=EDGE_CURVE('',#8152,#8153,#1806,.T.);
#10109=EDGE_CURVE('',#8154,#8146,#1807,.T.);
#10110=EDGE_CURVE('',#8153,#8154,#1808,.T.);
#10111=EDGE_CURVE('',#8155,#8151,#1809,.T.);
#10112=EDGE_CURVE('',#8156,#8155,#1810,.T.);
#10113=EDGE_CURVE('',#8154,#8156,#1811,.T.);
#10114=EDGE_CURVE('',#8157,#8150,#1812,.T.);
#10115=EDGE_CURVE('',#8155,#8157,#1813,.T.);
#10116=EDGE_CURVE('',#8158,#8149,#1814,.T.);
#10117=EDGE_CURVE('',#8157,#8158,#1815,.T.);
#10118=EDGE_CURVE('',#8158,#8159,#1816,.T.);
#10119=EDGE_CURVE('',#8159,#8152,#1817,.T.);
#10120=EDGE_CURVE('',#8156,#8159,#1818,.T.);
#10121=EDGE_CURVE('',#8160,#8161,#97,.T.);
#10122=EDGE_CURVE('',#8160,#8162,#1819,.T.);
#10123=EDGE_CURVE('',#8162,#8163,#1118,.T.);
#10124=EDGE_CURVE('',#8163,#8164,#1119,.T.);
#10125=EDGE_CURVE('',#8161,#8164,#1820,.T.);
#10126=EDGE_CURVE('',#8165,#8160,#98,.T.);
#10127=EDGE_CURVE('',#8165,#8166,#1821,.T.);
#10128=EDGE_CURVE('',#8166,#8167,#1120,.T.);
#10129=EDGE_CURVE('',#8167,#8168,#1121,.T.);
#10130=EDGE_CURVE('',#8168,#8162,#1122,.T.);
#10131=EDGE_CURVE('',#8169,#8169,#7262,.T.);
#10132=EDGE_CURVE('',#8169,#8170,#7263,.T.);
#10133=EDGE_CURVE('',#8170,#8171,#7264,.T.);
#10134=EDGE_CURVE('',#8171,#8170,#7265,.T.);
#10135=EDGE_CURVE('',#8172,#8172,#7266,.T.);
#10136=EDGE_CURVE('',#8172,#8173,#1822,.T.);
#10137=EDGE_CURVE('',#8173,#8173,#7267,.T.);
#10138=EDGE_CURVE('',#8174,#8174,#7268,.T.);
#10139=EDGE_CURVE('',#8174,#8175,#1823,.T.);
#10140=EDGE_CURVE('',#8175,#8175,#7269,.T.);
#10141=EDGE_CURVE('',#8176,#8176,#7270,.T.);
#10142=EDGE_CURVE('',#8176,#8177,#1824,.T.);
#10143=EDGE_CURVE('',#8177,#8177,#7271,.T.);
#10144=EDGE_CURVE('',#8178,#8178,#7272,.T.);
#10145=EDGE_CURVE('',#8178,#8179,#1825,.T.);
#10146=EDGE_CURVE('',#8179,#8179,#7273,.T.);
#10147=EDGE_CURVE('',#8180,#8181,#7274,.T.);
#10148=EDGE_CURVE('',#8182,#8180,#1377,.T.);
#10149=EDGE_CURVE('',#8182,#8183,#1826,.T.);
#10150=EDGE_CURVE('',#8183,#8183,#7275,.T.);
#10151=EDGE_CURVE('',#8181,#8182,#1378,.T.);
#10152=EDGE_CURVE('',#8184,#8185,#7276,.T.);
#10153=EDGE_CURVE('',#8185,#8186,#1123,.T.);
#10154=EDGE_CURVE('',#8186,#8187,#7277,.T.);
#10155=EDGE_CURVE('',#8187,#8184,#1124,.T.);
#10156=EDGE_CURVE('',#8188,#8189,#7278,.T.);
#10157=EDGE_CURVE('',#8189,#8190,#1125,.T.);
#10158=EDGE_CURVE('',#8191,#8190,#7279,.T.);
#10159=EDGE_CURVE('',#8191,#8192,#1126,.T.);
#10160=EDGE_CURVE('',#8192,#8186,#7280,.T.);
#10161=EDGE_CURVE('',#8185,#8193,#7281,.T.);
#10162=EDGE_CURVE('',#8193,#8188,#1127,.T.);
#10163=EDGE_CURVE('',#8191,#8194,#7282,.T.);
#10164=EDGE_CURVE('',#8194,#8195,#1128,.T.);
#10165=EDGE_CURVE('',#8195,#8192,#7283,.T.);
#10166=EDGE_CURVE('',#8196,#8196,#7284,.T.);
#10167=EDGE_CURVE('',#8196,#8197,#1827,.T.);
#10168=EDGE_CURVE('',#8197,#8197,#7285,.T.);
#10169=EDGE_CURVE('',#8198,#8198,#7286,.T.);
#10170=EDGE_CURVE('',#8198,#8199,#1828,.T.);
#10171=EDGE_CURVE('',#8199,#8200,#1129,.T.);
#10172=EDGE_CURVE('',#8201,#8200,#7287,.T.);
#10173=EDGE_CURVE('',#8201,#8202,#1130,.T.);
#10174=EDGE_CURVE('',#8203,#8202,#7288,.T.);
#10175=EDGE_CURVE('',#8203,#8204,#1131,.T.);
#10176=EDGE_CURVE('',#8205,#8204,#7289,.T.);
#10177=EDGE_CURVE('',#8205,#8199,#1132,.T.);
#10178=EDGE_CURVE('',#8206,#8207,#7290,.T.);
#10179=EDGE_CURVE('',#8208,#8206,#1379,.T.);
#10180=EDGE_CURVE('',#8208,#8209,#7291,.T.);
#10181=EDGE_CURVE('',#8209,#8210,#1829,.T.);
#10182=EDGE_CURVE('',#8210,#8210,#7292,.T.);
#10183=EDGE_CURVE('',#8209,#8211,#7293,.T.);
#10184=EDGE_CURVE('',#8207,#8211,#1380,.T.);
#10185=EDGE_CURVE('',#8212,#8212,#7294,.T.);
#10186=EDGE_CURVE('',#8212,#8213,#1830,.T.);
#10187=EDGE_CURVE('',#8213,#8213,#7295,.T.);
#10188=EDGE_CURVE('',#8214,#8214,#7296,.T.);
#10189=EDGE_CURVE('',#8214,#8215,#1831,.T.);
#10190=EDGE_CURVE('',#8215,#8215,#7297,.T.);
#10191=EDGE_CURVE('',#8216,#8217,#1133,.F.);
#10192=EDGE_CURVE('',#8218,#8216,#1832,.T.);
#10193=EDGE_CURVE('',#8219,#8218,#1134,.F.);
#10194=EDGE_CURVE('',#8217,#8219,#1833,.T.);
#10195=EDGE_CURVE('',#8220,#8221,#1135,.F.);
#10196=EDGE_CURVE('',#8222,#8220,#1834,.T.);
#10197=EDGE_CURVE('',#8223,#8222,#1136,.F.);
#10198=EDGE_CURVE('',#8221,#8223,#1835,.T.);
#10199=EDGE_CURVE('',#8224,#8225,#1381,.T.);
#10200=EDGE_CURVE('',#8226,#8224,#1137,.T.);
#10201=EDGE_CURVE('',#8227,#8226,#1836,.T.);
#10202=EDGE_CURVE('',#8228,#8227,#1138,.T.);
#10203=EDGE_CURVE('',#8229,#8228,#1382,.T.);
#10204=EDGE_CURVE('',#8230,#8229,#1139,.T.);
#10205=EDGE_CURVE('',#8231,#8230,#1837,.T.);
#10206=EDGE_CURVE('',#8225,#8231,#1140,.T.);
#10207=EDGE_CURVE('',#8232,#8233,#1141,.F.);
#10208=EDGE_CURVE('',#8234,#8232,#1838,.T.);
#10209=EDGE_CURVE('',#8235,#8234,#7298,.T.);
#10210=EDGE_CURVE('',#8233,#8235,#1839,.T.);
#10211=EDGE_CURVE('',#8236,#8237,#1142,.F.);
#10212=EDGE_CURVE('',#8238,#8236,#1840,.T.);
#10213=EDGE_CURVE('',#8239,#8238,#1143,.F.);
#10214=EDGE_CURVE('',#8237,#8239,#1841,.T.);
#10215=EDGE_CURVE('',#8240,#8241,#7299,.T.);
#10216=EDGE_CURVE('',#8241,#8242,#7300,.T.);
#10217=EDGE_CURVE('',#8242,#8243,#1842,.T.);
#10218=EDGE_CURVE('',#8243,#8244,#7301,.T.);
#10219=EDGE_CURVE('',#8240,#8244,#1843,.T.);
#10220=EDGE_CURVE('',#8245,#8245,#7302,.T.);
#10221=EDGE_CURVE('',#8245,#8246,#1844,.T.);
#10222=EDGE_CURVE('',#8246,#8246,#7303,.T.);
#10223=EDGE_CURVE('',#8247,#8247,#7304,.T.);
#10224=EDGE_CURVE('',#8247,#8248,#1845,.T.);
#10225=EDGE_CURVE('',#8248,#8248,#7305,.T.);
#10226=EDGE_CURVE('',#8249,#8249,#7306,.T.);
#10227=EDGE_CURVE('',#8249,#8250,#1846,.T.);
#10228=EDGE_CURVE('',#8250,#8250,#7307,.T.);
#10229=EDGE_CURVE('',#8251,#8251,#7308,.T.);
#10230=EDGE_CURVE('',#8251,#8252,#1847,.T.);
#10231=EDGE_CURVE('',#8252,#8252,#7309,.T.);
#10232=EDGE_CURVE('',#8253,#8253,#7310,.T.);
#10233=EDGE_CURVE('',#8253,#8254,#1848,.T.);
#10234=EDGE_CURVE('',#8254,#8254,#7311,.T.);
#10235=EDGE_CURVE('',#8255,#8256,#7312,.T.);
#10236=EDGE_CURVE('',#8257,#8255,#1849,.T.);
#10237=EDGE_CURVE('',#8258,#8257,#1144,.F.);
#10238=EDGE_CURVE('',#8256,#8258,#1850,.T.);
#10239=EDGE_CURVE('',#8259,#8260,#7313,.T.);
#10240=EDGE_CURVE('',#8261,#8259,#1851,.T.);
#10241=EDGE_CURVE('',#8262,#8261,#1145,.F.);
#10242=EDGE_CURVE('',#8226,#8262,#1146,.F.);
#10243=EDGE_CURVE('',#8260,#8224,#1852,.T.);
#10244=EDGE_CURVE('',#8263,#8261,#1383,.T.);
#10245=EDGE_CURVE('',#8264,#8263,#1853,.T.);
#10246=EDGE_CURVE('',#8265,#8264,#1384,.T.);
#10247=EDGE_CURVE('',#8266,#8265,#1147,.F.);
#10248=EDGE_CURVE('',#8262,#8266,#1854,.T.);
#10249=EDGE_CURVE('',#8267,#8268,#7314,.T.);
#10250=EDGE_CURVE('',#8268,#8269,#99,.T.);
#10251=EDGE_CURVE('',#8269,#8270,#7315,.T.);
#10252=EDGE_CURVE('',#8270,#8271,#100,.T.);
#10253=EDGE_CURVE('',#8271,#8272,#7316,.T.);
#10254=EDGE_CURVE('',#8272,#8273,#101,.T.);
#10255=EDGE_CURVE('',#8273,#8274,#7317,.T.);
#10256=EDGE_CURVE('',#8274,#8275,#102,.T.);
#10257=EDGE_CURVE('',#8275,#8276,#7318,.T.);
#10258=EDGE_CURVE('',#8276,#8241,#1855,.T.);
#10259=EDGE_CURVE('',#8277,#8240,#103,.T.);
#10260=EDGE_CURVE('',#8277,#8278,#104,.T.);
#10261=EDGE_CURVE('',#8278,#8242,#105,.T.);
#10262=EDGE_CURVE('',#8276,#8279,#7319,.T.);
#10263=EDGE_CURVE('',#8279,#8280,#106,.T.);
#10264=EDGE_CURVE('',#8280,#8281,#7320,.T.);
#10265=EDGE_CURVE('',#8281,#8282,#107,.T.);
#10266=EDGE_CURVE('',#8282,#8283,#7321,.T.);
#10267=EDGE_CURVE('',#8283,#8284,#108,.T.);
#10268=EDGE_CURVE('',#8284,#8285,#7322,.T.);
#10269=EDGE_CURVE('',#8285,#8267,#109,.T.);
#10270=EDGE_CURVE('',#8286,#8287,#1148,.T.);
#10271=EDGE_CURVE('',#8286,#8287,#1149,.F.);
#10272=EDGE_CURVE('',#8288,#8289,#1385,.T.);
#10273=EDGE_CURVE('',#8289,#8290,#7323,.T.);
#10274=EDGE_CURVE('',#8290,#8291,#1856,.T.);
#10275=EDGE_CURVE('',#8291,#8287,#7324,.T.);
#10276=EDGE_CURVE('',#8286,#8291,#7325,.T.);
#10277=EDGE_CURVE('',#8290,#8288,#7326,.T.);
#10278=EDGE_CURVE('',#8292,#8293,#7327,.T.);
#10279=EDGE_CURVE('',#8294,#8292,#1857,.T.);
#10280=EDGE_CURVE('',#8295,#8294,#7328,.T.);
#10281=EDGE_CURVE('',#8293,#8295,#1858,.T.);
#10282=EDGE_CURVE('',#8296,#8297,#7329,.T.);
#10283=EDGE_CURVE('',#8297,#8298,#1859,.T.);
#10284=EDGE_CURVE('',#8298,#8299,#7330,.T.);
#10285=EDGE_CURVE('',#8283,#8299,#1860,.T.);
#10286=EDGE_CURVE('',#8282,#8300,#1861,.T.);
#10287=EDGE_CURVE('',#8300,#8301,#7331,.T.);
#10288=EDGE_CURVE('',#8301,#8296,#1862,.T.);
#10289=EDGE_CURVE('',#8291,#8302,#1863,.T.);
#10290=EDGE_CURVE('',#8302,#8302,#7332,.T.);
#10291=EDGE_CURVE('',#8303,#8303,#7333,.T.);
#10292=EDGE_CURVE('',#8303,#8304,#1864,.T.);
#10293=EDGE_CURVE('',#8304,#8304,#7334,.T.);
#10294=EDGE_CURVE('',#8305,#8305,#7335,.T.);
#10295=EDGE_CURVE('',#8305,#8306,#1865,.T.);
#10296=EDGE_CURVE('',#8306,#8306,#7336,.T.);
#10297=EDGE_CURVE('',#8307,#8307,#7337,.T.);
#10298=EDGE_CURVE('',#8307,#8308,#1866,.T.);
#10299=EDGE_CURVE('',#8308,#8308,#7338,.T.);
#10300=EDGE_CURVE('',#8309,#8309,#7339,.T.);
#10301=EDGE_CURVE('',#8309,#8310,#1867,.T.);
#10302=EDGE_CURVE('',#8310,#8310,#7340,.T.);
#10303=EDGE_CURVE('',#8311,#8311,#7341,.T.);
#10304=EDGE_CURVE('',#8311,#8312,#1868,.T.);
#10305=EDGE_CURVE('',#8312,#8313,#7342,.T.);
#10306=EDGE_CURVE('',#8313,#8314,#1869,.T.);
#10307=EDGE_CURVE('',#8314,#8315,#7343,.T.);
#10308=EDGE_CURVE('',#8315,#8316,#1870,.T.);
#10309=EDGE_CURVE('',#8316,#8316,#7344,.T.);
#10310=EDGE_CURVE('',#8315,#8317,#7345,.T.);
#10311=EDGE_CURVE('',#8317,#8318,#1871,.T.);
#10312=EDGE_CURVE('',#8318,#8312,#7346,.T.);
#10313=EDGE_CURVE('',#8319,#8319,#7347,.T.);
#10314=EDGE_CURVE('',#8319,#8320,#1872,.T.);
#10315=EDGE_CURVE('',#8320,#8320,#7348,.T.);
#10316=EDGE_CURVE('',#8321,#8321,#7349,.T.);
#10317=EDGE_CURVE('',#8321,#8322,#1873,.T.);
#10318=EDGE_CURVE('',#8322,#8322,#7350,.T.);
#10319=EDGE_CURVE('',#8316,#8323,#1874,.T.);
#10320=EDGE_CURVE('',#8323,#8323,#7351,.T.);
#10321=EDGE_CURVE('',#8324,#8324,#7352,.T.);
#10322=EDGE_CURVE('',#8324,#8325,#1875,.T.);
#10323=EDGE_CURVE('',#8325,#8325,#7353,.T.);
#10324=EDGE_CURVE('',#8326,#8326,#7354,.T.);
#10325=EDGE_CURVE('',#8326,#8327,#1876,.T.);
#10326=EDGE_CURVE('',#8327,#8327,#7355,.T.);
#10327=EDGE_CURVE('',#8328,#8328,#7356,.T.);
#10328=EDGE_CURVE('',#8328,#8329,#1877,.T.);
#10329=EDGE_CURVE('',#8329,#8329,#7357,.T.);
#10330=EDGE_CURVE('',#8330,#8330,#7358,.T.);
#10331=EDGE_CURVE('',#8330,#8331,#1878,.T.);
#10332=EDGE_CURVE('',#8331,#8331,#7359,.T.);
#10333=EDGE_CURVE('',#8332,#8332,#7360,.T.);
#10334=EDGE_CURVE('',#8332,#8333,#1879,.T.);
#10335=EDGE_CURVE('',#8333,#8333,#7361,.T.);
#10336=EDGE_CURVE('',#8334,#8334,#7362,.T.);
#10337=EDGE_CURVE('',#8334,#8335,#1880,.T.);
#10338=EDGE_CURVE('',#8335,#8335,#7363,.T.);
#10339=EDGE_CURVE('',#8336,#8337,#7364,.T.);
#10340=EDGE_CURVE('',#8338,#8337,#1881,.T.);
#10341=EDGE_CURVE('',#8338,#8339,#7365,.T.);
#10342=EDGE_CURVE('',#8336,#8339,#1882,.T.);
#10343=EDGE_CURVE('',#8171,#8340,#1883,.T.);
#10344=EDGE_CURVE('',#8341,#8340,#7366,.T.);
#10345=EDGE_CURVE('',#8340,#8341,#7367,.T.);
#10346=EDGE_CURVE('',#8342,#8343,#7368,.T.);
#10347=EDGE_CURVE('',#8344,#8343,#1884,.T.);
#10348=EDGE_CURVE('',#8345,#8344,#7369,.T.);
#10349=EDGE_CURVE('',#8345,#8342,#1885,.T.);
#10350=EDGE_CURVE('',#8346,#8347,#7370,.T.);
#10351=EDGE_CURVE('',#8347,#8346,#7371,.T.);
#10352=EDGE_CURVE('',#8347,#8341,#1886,.T.);
#10353=EDGE_CURVE('',#8348,#8349,#7372,.T.);
#10354=EDGE_CURVE('',#8349,#8348,#7373,.T.);
#10355=EDGE_CURVE('',#8349,#8346,#1887,.T.);
#10356=EDGE_CURVE('',#8350,#8351,#1150,.T.);
#10357=EDGE_CURVE('',#8351,#8352,#1151,.T.);
#10358=EDGE_CURVE('',#8352,#8353,#7374,.T.);
#10359=EDGE_CURVE('',#8353,#8354,#1152,.T.);
#10360=EDGE_CURVE('',#8354,#8355,#1153,.T.);
#10361=EDGE_CURVE('',#8355,#8356,#1154,.T.);
#10362=EDGE_CURVE('',#8356,#8357,#7375,.T.);
#10363=EDGE_CURVE('',#8357,#8358,#1155,.T.);
#10364=EDGE_CURVE('',#8358,#8359,#1156,.T.);
#10365=EDGE_CURVE('',#8360,#8359,#1888,.T.);
#10366=EDGE_CURVE('',#8361,#8360,#7376,.T.);
#10367=EDGE_CURVE('',#8361,#8362,#1889,.T.);
#10368=EDGE_CURVE('',#8362,#8363,#1157,.T.);
#10369=EDGE_CURVE('',#8363,#8364,#1158,.T.);
#10370=EDGE_CURVE('',#8364,#8365,#7377,.T.);
#10371=EDGE_CURVE('',#8365,#8366,#1159,.T.);
#10372=EDGE_CURVE('',#8366,#8367,#1160,.T.);
#10373=EDGE_CURVE('',#8367,#8368,#1161,.T.);
#10374=EDGE_CURVE('',#8368,#8369,#7378,.T.);
#10375=EDGE_CURVE('',#8369,#8350,#1162,.T.);
#10376=EDGE_CURVE('',#8370,#8370,#7379,.T.);
#10377=EDGE_CURVE('',#8370,#8371,#1890,.T.);
#10378=EDGE_CURVE('',#8371,#8371,#7380,.T.);
#10379=EDGE_CURVE('',#8372,#8372,#7381,.T.);
#10380=EDGE_CURVE('',#8372,#8373,#1891,.T.);
#10381=EDGE_CURVE('',#8373,#8373,#7382,.T.);
#10382=EDGE_CURVE('',#8348,#8374,#1892,.T.);
#10383=EDGE_CURVE('',#8374,#8374,#7383,.T.);
#10384=EDGE_CURVE('',#8375,#8375,#7384,.T.);
#10385=EDGE_CURVE('',#8375,#8376,#1893,.T.);
#10386=EDGE_CURVE('',#8377,#8376,#7385,.T.);
#10387=EDGE_CURVE('',#8376,#8377,#7386,.T.);
#10388=EDGE_CURVE('',#8378,#8379,#7387,.T.);
#10389=EDGE_CURVE('',#8378,#8380,#1894,.T.);
#10390=EDGE_CURVE('',#8381,#8380,#7388,.T.);
#10391=EDGE_CURVE('',#8379,#8381,#1895,.T.);
#10392=EDGE_CURVE('',#8382,#8377,#1896,.T.);
#10393=EDGE_CURVE('',#8383,#8384,#1386,.T.);
#10394=EDGE_CURVE('',#8384,#8383,#1163,.T.);
#10395=EDGE_CURVE('',#8165,#8359,#1387,.T.);
#10396=EDGE_CURVE('',#8359,#8165,#1164,.T.);
#10397=EDGE_CURVE('',#8359,#8385,#1897,.T.);
#10398=EDGE_CURVE('',#8386,#8385,#1165,.T.);
#10399=EDGE_CURVE('',#8386,#8166,#1166,.T.);
#10400=EDGE_CURVE('',#8387,#8388,#1898,.T.);
#10401=EDGE_CURVE('',#8388,#8387,#1167,.T.);
#10402=EDGE_CURVE('',#8389,#8390,#1899,.T.);
#10403=EDGE_CURVE('',#8391,#8389,#1168,.T.);
#10404=EDGE_CURVE('',#8392,#8391,#1169,.T.);
#10405=EDGE_CURVE('',#8392,#8366,#1900,.T.);
#10406=EDGE_CURVE('',#8364,#8365,#1170,.T.);
#10407=EDGE_CURVE('',#8390,#8363,#1171,.T.);
#10408=EDGE_CURVE('',#8362,#8393,#1388,.T.);
#10409=EDGE_CURVE('',#8393,#8362,#1172,.T.);
#10410=EDGE_CURVE('',#8362,#8394,#1901,.T.);
#10411=EDGE_CURVE('',#8393,#8395,#1902,.T.);
#10412=EDGE_CURVE('',#8395,#8396,#1173,.T.);
#10413=EDGE_CURVE('',#8394,#8396,#1174,.T.);
#10414=EDGE_CURVE('',#8397,#8398,#1389,.T.);
#10415=EDGE_CURVE('',#8398,#8397,#1175,.T.);
#10416=EDGE_CURVE('',#8397,#8399,#1903,.T.);
#10417=EDGE_CURVE('',#8398,#8400,#1904,.T.);
#10418=EDGE_CURVE('',#8401,#8400,#1176,.T.);
#10419=EDGE_CURVE('',#8401,#8399,#1177,.T.);
#10420=EDGE_CURVE('',#8402,#8403,#1390,.T.);
#10421=EDGE_CURVE('',#8403,#8402,#1178,.T.);
#10422=EDGE_CURVE('',#8404,#8405,#1391,.T.);
#10423=EDGE_CURVE('',#8405,#8404,#1179,.T.);
#10424=EDGE_CURVE('',#8406,#8407,#1905,.T.);
#10425=EDGE_CURVE('',#8408,#8406,#1906,.T.);
#10426=EDGE_CURVE('',#8409,#8408,#1907,.T.);
#10427=EDGE_CURVE('',#8410,#8409,#1908,.T.);
#10428=EDGE_CURVE('',#8411,#8410,#1909,.T.);
#10429=EDGE_CURVE('',#8407,#8411,#1910,.T.);
#10430=EDGE_CURVE('',#8412,#8413,#1911,.T.);
#10431=EDGE_CURVE('',#8414,#8412,#1912,.T.);
#10432=EDGE_CURVE('',#8415,#8414,#1913,.T.);
#10433=EDGE_CURVE('',#8416,#8415,#1914,.T.);
#10434=EDGE_CURVE('',#8417,#8416,#1915,.T.);
#10435=EDGE_CURVE('',#8413,#8417,#1916,.T.);
#10436=EDGE_CURVE('',#8418,#8419,#1917,.T.);
#10437=EDGE_CURVE('',#8420,#8418,#1918,.T.);
#10438=EDGE_CURVE('',#8421,#8420,#1919,.T.);
#10439=EDGE_CURVE('',#8422,#8421,#1920,.T.);
#10440=EDGE_CURVE('',#8423,#8422,#1921,.T.);
#10441=EDGE_CURVE('',#8419,#8423,#1922,.T.);
#10442=EDGE_CURVE('',#8424,#8425,#1923,.T.);
#10443=EDGE_CURVE('',#8426,#8424,#1924,.T.);
#10444=EDGE_CURVE('',#8427,#8426,#1925,.T.);
#10445=EDGE_CURVE('',#8428,#8427,#1926,.T.);
#10446=EDGE_CURVE('',#8429,#8428,#1927,.T.);
#10447=EDGE_CURVE('',#8425,#8429,#1928,.T.);
#10448=EDGE_CURVE('',#8430,#8431,#7389,.T.);
#10449=EDGE_CURVE('',#8431,#8432,#1929,.T.);
#10450=EDGE_CURVE('',#8432,#8433,#7390,.T.);
#10451=EDGE_CURVE('',#8433,#8434,#7391,.T.);
#10452=EDGE_CURVE('',#8434,#8435,#7392,.T.);
#10453=EDGE_CURVE('',#8435,#8436,#1930,.T.);
#10454=EDGE_CURVE('',#8436,#8378,#7393,.T.);
#10455=EDGE_CURVE('',#8379,#8437,#7394,.T.);
#10456=EDGE_CURVE('',#8437,#8438,#1931,.T.);
#10457=EDGE_CURVE('',#8438,#8439,#7395,.T.);
#10458=EDGE_CURVE('',#8439,#8440,#7396,.T.);
#10459=EDGE_CURVE('',#8440,#8441,#7397,.T.);
#10460=EDGE_CURVE('',#8441,#8442,#1932,.T.);
#10461=EDGE_CURVE('',#8442,#8443,#7398,.T.);
#10462=EDGE_CURVE('',#8443,#8430,#7399,.T.);
#10463=EDGE_CURVE('',#8444,#8445,#1933,.T.);
#10464=EDGE_CURVE('',#8445,#8446,#1934,.T.);
#10465=EDGE_CURVE('',#8446,#8447,#1935,.T.);
#10466=EDGE_CURVE('',#8447,#8448,#1936,.T.);
#10467=EDGE_CURVE('',#8448,#8449,#1937,.T.);
#10468=EDGE_CURVE('',#8449,#8444,#1938,.T.);
#10469=EDGE_CURVE('',#8450,#8451,#1939,.T.);
#10470=EDGE_CURVE('',#8451,#8452,#1940,.T.);
#10471=EDGE_CURVE('',#8452,#8453,#1941,.T.);
#10472=EDGE_CURVE('',#8453,#8454,#1942,.T.);
#10473=EDGE_CURVE('',#8454,#8455,#1943,.T.);
#10474=EDGE_CURVE('',#8455,#8450,#1944,.T.);
#10475=EDGE_CURVE('',#8456,#8457,#1945,.T.);
#10476=EDGE_CURVE('',#8410,#8457,#1946,.T.);
#10477=EDGE_CURVE('',#8456,#8409,#1947,.T.);
#10478=EDGE_CURVE('',#8457,#8458,#1948,.T.);
#10479=EDGE_CURVE('',#8411,#8458,#1949,.T.);
#10480=EDGE_CURVE('',#8458,#8459,#1950,.T.);
#10481=EDGE_CURVE('',#8407,#8459,#1951,.T.);
#10482=EDGE_CURVE('',#8459,#8460,#1952,.T.);
#10483=EDGE_CURVE('',#8406,#8460,#1953,.T.);
#10484=EDGE_CURVE('',#8460,#8461,#1954,.T.);
#10485=EDGE_CURVE('',#8408,#8461,#1955,.T.);
#10486=EDGE_CURVE('',#8461,#8456,#1956,.T.);
#10487=EDGE_CURVE('',#8462,#8463,#1957,.T.);
#10488=EDGE_CURVE('',#8462,#8464,#1958,.T.);
#10489=EDGE_CURVE('',#8464,#8465,#1959,.T.);
#10490=EDGE_CURVE('',#8466,#8465,#1960,.T.);
#10491=EDGE_CURVE('',#8463,#8466,#7400,.T.);
#10492=EDGE_CURVE('',#8467,#8468,#1961,.T.);
#10493=EDGE_CURVE('',#8465,#8468,#7401,.T.);
#10494=EDGE_CURVE('',#8464,#8467,#7402,.T.);
#10495=EDGE_CURVE('',#8468,#8469,#1962,.T.);
#10496=EDGE_CURVE('',#8467,#8470,#1963,.T.);
#10497=EDGE_CURVE('',#8471,#8470,#1964,.T.);
#10498=EDGE_CURVE('',#8469,#8471,#7403,.T.);
#10499=EDGE_CURVE('',#8472,#8473,#1965,.T.);
#10500=EDGE_CURVE('',#8415,#8472,#1966,.T.);
#10501=EDGE_CURVE('',#8473,#8414,#1967,.T.);
#10502=EDGE_CURVE('',#8473,#8474,#1968,.T.);
#10503=EDGE_CURVE('',#8474,#8412,#1969,.T.);
#10504=EDGE_CURVE('',#8474,#8475,#1970,.T.);
#10505=EDGE_CURVE('',#8475,#8413,#1971,.T.);
#10506=EDGE_CURVE('',#8475,#8476,#1972,.T.);
#10507=EDGE_CURVE('',#8476,#8417,#1973,.T.);
#10508=EDGE_CURVE('',#8476,#8477,#1974,.T.);
#10509=EDGE_CURVE('',#8477,#8416,#1975,.T.);
#10510=EDGE_CURVE('',#8477,#8472,#1976,.T.);
#10511=EDGE_CURVE('',#8478,#8479,#1977,.T.);
#10512=EDGE_CURVE('',#8478,#8480,#1978,.T.);
#10513=EDGE_CURVE('',#8481,#8480,#1979,.T.);
#10514=EDGE_CURVE('',#8482,#8481,#1980,.T.);
#10515=EDGE_CURVE('',#8479,#8482,#7404,.T.);
#10516=EDGE_CURVE('',#8483,#8484,#1981,.T.);
#10517=EDGE_CURVE('',#8480,#8484,#7405,.T.);
#10518=EDGE_CURVE('',#8483,#8478,#7406,.T.);
#10519=EDGE_CURVE('',#8485,#8486,#1982,.T.);
#10520=EDGE_CURVE('',#8484,#8485,#1983,.T.);
#10521=EDGE_CURVE('',#8487,#8483,#1984,.T.);
#10522=EDGE_CURVE('',#8486,#8487,#7407,.T.);
#10523=EDGE_CURVE('',#8488,#8489,#1985,.T.);
#10524=EDGE_CURVE('',#8421,#8488,#1986,.T.);
#10525=EDGE_CURVE('',#8489,#8420,#1987,.T.);
#10526=EDGE_CURVE('',#8489,#8490,#1988,.T.);
#10527=EDGE_CURVE('',#8490,#8418,#1989,.T.);
#10528=EDGE_CURVE('',#8490,#8491,#1990,.T.);
#10529=EDGE_CURVE('',#8491,#8419,#1991,.T.);
#10530=EDGE_CURVE('',#8491,#8492,#1992,.T.);
#10531=EDGE_CURVE('',#8492,#8423,#1993,.T.);
#10532=EDGE_CURVE('',#8492,#8493,#1994,.T.);
#10533=EDGE_CURVE('',#8493,#8422,#1995,.T.);
#10534=EDGE_CURVE('',#8493,#8488,#1996,.T.);
#10535=EDGE_CURVE('',#8494,#8495,#1997,.T.);
#10536=EDGE_CURVE('',#8494,#8496,#1998,.T.);
#10537=EDGE_CURVE('',#8497,#8496,#1999,.T.);
#10538=EDGE_CURVE('',#8498,#8497,#2000,.T.);
#10539=EDGE_CURVE('',#8495,#8498,#7408,.T.);
#10540=EDGE_CURVE('',#8499,#8500,#2001,.T.);
#10541=EDGE_CURVE('',#8496,#8500,#7409,.T.);
#10542=EDGE_CURVE('',#8499,#8494,#7410,.T.);
#10543=EDGE_CURVE('',#8501,#8502,#2002,.T.);
#10544=EDGE_CURVE('',#8500,#8501,#2003,.T.);
#10545=EDGE_CURVE('',#8503,#8499,#2004,.T.);
#10546=EDGE_CURVE('',#8502,#8503,#7411,.T.);
#10547=EDGE_CURVE('',#8487,#8469,#2005,.T.);
#10548=EDGE_CURVE('',#8504,#8479,#2006,.T.);
#10549=EDGE_CURVE('',#8504,#8505,#2007,.T.);
#10550=EDGE_CURVE('',#8505,#8506,#7412,.T.);
#10551=EDGE_CURVE('',#8506,#8507,#2008,.T.);
#10552=EDGE_CURVE('',#8503,#8507,#2009,.T.);
#10553=EDGE_CURVE('',#8466,#8495,#2010,.T.);
#10554=EDGE_CURVE('',#8508,#8509,#2011,.T.);
#10555=EDGE_CURVE('',#8427,#8508,#2012,.T.);
#10556=EDGE_CURVE('',#8509,#8426,#2013,.T.);
#10557=EDGE_CURVE('',#8509,#8510,#2014,.T.);
#10558=EDGE_CURVE('',#8510,#8424,#2015,.T.);
#10559=EDGE_CURVE('',#8510,#8511,#2016,.T.);
#10560=EDGE_CURVE('',#8511,#8425,#2017,.T.);
#10561=EDGE_CURVE('',#8511,#8512,#2018,.T.);
#10562=EDGE_CURVE('',#8512,#8429,#2019,.T.);
#10563=EDGE_CURVE('',#8512,#8513,#2020,.T.);
#10564=EDGE_CURVE('',#8513,#8428,#2021,.T.);
#10565=EDGE_CURVE('',#8513,#8508,#2022,.T.);
#10566=EDGE_CURVE('',#8506,#8514,#2023,.T.);
#10567=EDGE_CURVE('',#8515,#8514,#2024,.T.);
#10568=EDGE_CURVE('',#8516,#8515,#2025,.T.);
#10569=EDGE_CURVE('',#8507,#8516,#7413,.T.);
#10570=EDGE_CURVE('',#8505,#8517,#2026,.T.);
#10571=EDGE_CURVE('',#8514,#8517,#7414,.T.);
#10572=EDGE_CURVE('',#8518,#8519,#2027,.T.);
#10573=EDGE_CURVE('',#8517,#8518,#2028,.T.);
#10574=EDGE_CURVE('',#8519,#8504,#7415,.T.);
#10575=EDGE_CURVE('',#8520,#8433,#2029,.T.);
#10576=EDGE_CURVE('',#8432,#8521,#2030,.T.);
#10577=EDGE_CURVE('',#8520,#8521,#7416,.T.);
#10578=EDGE_CURVE('',#8431,#8522,#2031,.T.);
#10579=EDGE_CURVE('',#8521,#8522,#2032,.T.);
#10580=EDGE_CURVE('',#8430,#8523,#2033,.T.);
#10581=EDGE_CURVE('',#8522,#8523,#7417,.T.);
#10582=EDGE_CURVE('',#8443,#8524,#2034,.T.);
#10583=EDGE_CURVE('',#8523,#8524,#7418,.T.);
#10584=EDGE_CURVE('',#8442,#8525,#2035,.T.);
#10585=EDGE_CURVE('',#8524,#8525,#7419,.T.);
#10586=EDGE_CURVE('',#8441,#8526,#2036,.T.);
#10587=EDGE_CURVE('',#8525,#8526,#2037,.T.);
#10588=EDGE_CURVE('',#8440,#8527,#2038,.T.);
#10589=EDGE_CURVE('',#8526,#8527,#7420,.T.);
#10590=EDGE_CURVE('',#8439,#8528,#2039,.T.);
#10591=EDGE_CURVE('',#8527,#8528,#7421,.T.);
#10592=EDGE_CURVE('',#8438,#8529,#2040,.T.);
#10593=EDGE_CURVE('',#8528,#8529,#7422,.T.);
#10594=EDGE_CURVE('',#8437,#8530,#2041,.T.);
#10595=EDGE_CURVE('',#8529,#8530,#2042,.T.);
#10596=EDGE_CURVE('',#8530,#8381,#7423,.T.);
#10597=EDGE_CURVE('',#8436,#8531,#2043,.T.);
#10598=EDGE_CURVE('',#8380,#8531,#7424,.T.);
#10599=EDGE_CURVE('',#8435,#8532,#2044,.T.);
#10600=EDGE_CURVE('',#8531,#8532,#2045,.T.);
#10601=EDGE_CURVE('',#8434,#8533,#2046,.T.);
#10602=EDGE_CURVE('',#8532,#8533,#7425,.T.);
#10603=EDGE_CURVE('',#8533,#8520,#7426,.T.);
#10604=EDGE_CURVE('',#8534,#8446,#2047,.T.);
#10605=EDGE_CURVE('',#8445,#8535,#2048,.T.);
#10606=EDGE_CURVE('',#8534,#8535,#7427,.T.);
#10607=EDGE_CURVE('',#8444,#8536,#2049,.T.);
#10608=EDGE_CURVE('',#8535,#8536,#7428,.T.);
#10609=EDGE_CURVE('',#8449,#8537,#2050,.T.);
#10610=EDGE_CURVE('',#8536,#8537,#7429,.T.);
#10611=EDGE_CURVE('',#8448,#8538,#2051,.T.);
#10612=EDGE_CURVE('',#8537,#8538,#7430,.T.);
#10613=EDGE_CURVE('',#8447,#8539,#2052,.T.);
#10614=EDGE_CURVE('',#8538,#8539,#7431,.T.);
#10615=EDGE_CURVE('',#8539,#8534,#7432,.T.);
#10616=EDGE_CURVE('',#8540,#8452,#2053,.T.);
#10617=EDGE_CURVE('',#8451,#8541,#2054,.T.);
#10618=EDGE_CURVE('',#8540,#8541,#7433,.T.);
#10619=EDGE_CURVE('',#8450,#8542,#2055,.T.);
#10620=EDGE_CURVE('',#8541,#8542,#7434,.T.);
#10621=EDGE_CURVE('',#8455,#8543,#2056,.T.);
#10622=EDGE_CURVE('',#8542,#8543,#7435,.T.);
#10623=EDGE_CURVE('',#8454,#8544,#2057,.T.);
#10624=EDGE_CURVE('',#8543,#8544,#7436,.T.);
#10625=EDGE_CURVE('',#8453,#8545,#2058,.T.);
#10626=EDGE_CURVE('',#8544,#8545,#7437,.T.);
#10627=EDGE_CURVE('',#8545,#8540,#7438,.T.);
#10628=EDGE_CURVE('',#8463,#8498,#2059,.T.);
#10629=EDGE_CURVE('',#8486,#8471,#2060,.T.);
#10630=EDGE_CURVE('',#8546,#8547,#7439,.T.);
#10631=EDGE_CURVE('',#8470,#8546,#2061,.T.);
#10632=EDGE_CURVE('',#8547,#8462,#2062,.T.);
#10633=EDGE_CURVE('',#8519,#8482,#2063,.T.);
#10634=EDGE_CURVE('',#8548,#8485,#2064,.T.);
#10635=EDGE_CURVE('',#8549,#8548,#7440,.T.);
#10636=EDGE_CURVE('',#8481,#8549,#2065,.T.);
#10637=EDGE_CURVE('',#8550,#8501,#2066,.T.);
#10638=EDGE_CURVE('',#8551,#8550,#7441,.T.);
#10639=EDGE_CURVE('',#8497,#8551,#2067,.T.);
#10640=EDGE_CURVE('',#8502,#8516,#2068,.T.);
#10641=EDGE_CURVE('',#8552,#8518,#2069,.T.);
#10642=EDGE_CURVE('',#8553,#8552,#7442,.T.);
#10643=EDGE_CURVE('',#8515,#8553,#2070,.T.);
#10644=EDGE_CURVE('',#8554,#8555,#1180,.T.);
#10645=EDGE_CURVE('',#8556,#8554,#2071,.T.);
#10646=EDGE_CURVE('',#8557,#8556,#2072,.T.);
#10647=EDGE_CURVE('',#8555,#8557,#1181,.T.);
#10648=EDGE_CURVE('',#8558,#8556,#7443,.T.);
#10649=EDGE_CURVE('',#8559,#8558,#2073,.T.);
#10650=EDGE_CURVE('',#8557,#8559,#1182,.T.);
#10651=EDGE_CURVE('',#8560,#8558,#2074,.T.);
#10652=EDGE_CURVE('',#8561,#8560,#1183,.T.);
#10653=EDGE_CURVE('',#8559,#8561,#1184,.T.);
#10654=EDGE_CURVE('',#8562,#8401,#2075,.T.);
#10655=EDGE_CURVE('',#8563,#8562,#2076,.T.);
#10656=EDGE_CURVE('',#8399,#8563,#1185,.T.);
#10657=EDGE_CURVE('',#8564,#8562,#7444,.T.);
#10658=EDGE_CURVE('',#8565,#8564,#2077,.T.);
#10659=EDGE_CURVE('',#8563,#8565,#1186,.T.);
#10660=EDGE_CURVE('',#8565,#8395,#1187,.T.);
#10661=EDGE_CURVE('',#8396,#8564,#2078,.T.);
#10662=EDGE_CURVE('',#8566,#8386,#2079,.T.);
#10663=EDGE_CURVE('',#8167,#8566,#2080,.T.);
#10664=EDGE_CURVE('',#8567,#8566,#7445,.T.);
#10665=EDGE_CURVE('',#8168,#8567,#2081,.T.);
#10666=EDGE_CURVE('',#8163,#8567,#2082,.T.);
#10667=EDGE_CURVE('',#8568,#8569,#1188,.T.);
#10668=EDGE_CURVE('',#8570,#8569,#2083,.T.);
#10669=EDGE_CURVE('',#8571,#8570,#2084,.T.);
#10670=EDGE_CURVE('',#8568,#8571,#1189,.T.);
#10671=EDGE_CURVE('',#8572,#8570,#7446,.T.);
#10672=EDGE_CURVE('',#8573,#8572,#2085,.T.);
#10673=EDGE_CURVE('',#8571,#8573,#1190,.T.);
#10674=EDGE_CURVE('',#8573,#8574,#1191,.T.);
#10675=EDGE_CURVE('',#8575,#8572,#2086,.T.);
#10676=EDGE_CURVE('',#8574,#8575,#1192,.T.);
#10677=EDGE_CURVE('',#8576,#8577,#1193,.T.);
#10678=EDGE_CURVE('',#8164,#8577,#110,.T.);
#10679=EDGE_CURVE('',#8385,#8386,#1194,.T.);
#10680=EDGE_CURVE('',#8578,#8385,#7447,.T.);
#10681=EDGE_CURVE('',#8578,#8579,#1195,.T.);
#10682=EDGE_CURVE('',#8579,#8580,#1196,.T.);
#10683=EDGE_CURVE('',#8580,#8581,#1197,.T.);
#10684=EDGE_CURVE('',#8581,#8582,#1198,.T.);
#10685=EDGE_CURVE('',#8582,#8583,#1199,.T.);
#10686=EDGE_CURVE('',#8583,#8392,#1200,.T.);
#10687=EDGE_CURVE('',#8394,#8391,#7448,.T.);
#10688=EDGE_CURVE('',#8396,#8394,#1201,.T.);
#10689=EDGE_CURVE('',#8400,#8401,#1202,.T.);
#10690=EDGE_CURVE('',#8584,#8400,#7449,.T.);
#10691=EDGE_CURVE('',#8584,#8585,#1203,.T.);
#10692=EDGE_CURVE('',#8585,#8586,#1204,.T.);
#10693=EDGE_CURVE('',#8586,#8587,#1205,.T.);
#10694=EDGE_CURVE('',#8587,#8588,#1206,.T.);
#10695=EDGE_CURVE('',#8588,#8589,#1207,.T.);
#10696=EDGE_CURVE('',#8589,#8590,#1208,.T.);
#10697=EDGE_CURVE('',#8590,#8591,#1209,.T.);
#10698=EDGE_CURVE('',#8592,#8591,#7450,.T.);
#10699=EDGE_CURVE('',#8560,#8592,#111,.T.);
#10700=EDGE_CURVE('',#8593,#8554,#112,.T.);
#10701=EDGE_CURVE('',#8594,#8593,#7451,.T.);
#10702=EDGE_CURVE('',#8594,#8595,#1210,.T.);
#10703=EDGE_CURVE('',#8595,#8596,#1211,.T.);
#10704=EDGE_CURVE('',#8596,#8597,#1212,.T.);
#10705=EDGE_CURVE('',#8597,#8598,#1213,.T.);
#10706=EDGE_CURVE('',#8598,#8599,#1214,.T.);
#10707=EDGE_CURVE('',#8599,#8600,#1215,.T.);
#10708=EDGE_CURVE('',#8600,#8601,#1216,.T.);
#10709=EDGE_CURVE('',#8602,#8601,#7452,.T.);
#10710=EDGE_CURVE('',#8575,#8602,#1217,.T.);
#10711=EDGE_CURVE('',#8569,#8603,#1218,.T.);
#10712=EDGE_CURVE('',#8604,#8603,#7453,.T.);
#10713=EDGE_CURVE('',#8604,#8605,#1219,.T.);
#10714=EDGE_CURVE('',#8605,#8606,#1220,.T.);
#10715=EDGE_CURVE('',#8606,#8607,#1221,.T.);
#10716=EDGE_CURVE('',#8607,#8608,#1222,.T.);
#10717=EDGE_CURVE('',#8608,#8609,#1223,.T.);
#10718=EDGE_CURVE('',#8609,#8576,#1224,.T.);
#10719=EDGE_CURVE('',#8610,#8611,#7454,.T.);
#10720=EDGE_CURVE('',#8551,#8611,#2087,.T.);
#10721=EDGE_CURVE('',#8610,#8550,#2088,.T.);
#10722=EDGE_CURVE('',#8611,#8612,#2089,.T.);
#10723=EDGE_CURVE('',#8547,#8612,#2090,.T.);
#10724=EDGE_CURVE('',#8612,#8613,#7455,.T.);
#10725=EDGE_CURVE('',#8546,#8613,#2091,.T.);
#10726=EDGE_CURVE('',#8613,#8614,#2092,.T.);
#10727=EDGE_CURVE('',#8548,#8614,#2093,.T.);
#10728=EDGE_CURVE('',#8614,#8615,#7456,.T.);
#10729=EDGE_CURVE('',#8549,#8615,#2094,.T.);
#10730=EDGE_CURVE('',#8615,#8616,#2095,.T.);
#10731=EDGE_CURVE('',#8552,#8616,#2096,.T.);
#10732=EDGE_CURVE('',#8616,#8617,#7457,.T.);
#10733=EDGE_CURVE('',#8553,#8617,#2097,.T.);
#10734=EDGE_CURVE('',#8617,#8610,#2098,.T.);
#10735=EDGE_CURVE('',#8404,#8555,#2099,.T.);
#10736=EDGE_CURVE('',#8593,#8405,#2100,.T.);
#10737=EDGE_CURVE('',#8403,#8561,#2101,.T.);
#10738=EDGE_CURVE('',#8404,#8403,#1225,.T.);
#10739=EDGE_CURVE('',#8402,#8592,#2102,.T.);
#10740=EDGE_CURVE('',#8591,#8618,#1226,.T.);
#10741=EDGE_CURVE('',#8402,#8618,#1227,.T.);
#10742=EDGE_CURVE('',#8619,#8620,#7458,.T.);
#10743=EDGE_CURVE('',#8619,#8620,#1228,.T.);
#10744=EDGE_CURVE('',#8618,#8619,#1229,.T.);
#10745=EDGE_CURVE('',#8590,#8621,#2103,.T.);
#10746=EDGE_CURVE('',#8620,#8621,#1230,.T.);
#10747=EDGE_CURVE('',#8589,#8622,#2104,.T.);
#10748=EDGE_CURVE('',#8621,#8622,#1231,.T.);
#10749=EDGE_CURVE('',#8623,#8624,#7459,.T.);
#10750=EDGE_CURVE('',#8623,#8624,#1232,.T.);
#10751=EDGE_CURVE('',#8588,#8625,#2105,.T.);
#10752=EDGE_CURVE('',#8624,#8625,#1233,.T.);
#10753=EDGE_CURVE('',#8622,#8623,#1234,.T.);
#10754=EDGE_CURVE('',#8587,#8626,#2106,.T.);
#10755=EDGE_CURVE('',#8625,#8626,#1235,.F.);
#10756=EDGE_CURVE('',#8627,#8628,#7460,.T.);
#10757=EDGE_CURVE('',#8627,#8628,#1236,.T.);
#10758=EDGE_CURVE('',#8586,#8629,#2107,.T.);
#10759=EDGE_CURVE('',#8628,#8629,#1237,.T.);
#10760=EDGE_CURVE('',#8626,#8627,#1238,.T.);
#10761=EDGE_CURVE('',#8585,#8630,#2108,.T.);
#10762=EDGE_CURVE('',#8629,#8630,#1239,.T.);
#10763=EDGE_CURVE('',#8631,#8632,#7461,.T.);
#10764=EDGE_CURVE('',#8631,#8632,#1240,.T.);
#10765=EDGE_CURVE('',#8633,#8584,#1241,.T.);
#10766=EDGE_CURVE('',#8632,#8633,#1242,.T.);
#10767=EDGE_CURVE('',#8630,#8631,#1243,.T.);
#10768=EDGE_CURVE('',#8633,#8398,#1244,.T.);
#10769=EDGE_CURVE('',#8397,#8393,#1245,.T.);
#10770=EDGE_CURVE('',#8356,#8357,#1246,.T.);
#10771=EDGE_CURVE('',#8358,#8388,#1247,.T.);
#10772=EDGE_CURVE('',#8387,#8578,#1248,.T.);
#10773=EDGE_CURVE('',#8389,#8390,#7462,.T.);
#10774=EDGE_CURVE('',#8583,#8367,#2109,.T.);
#10775=EDGE_CURVE('',#8368,#8369,#1249,.T.);
#10776=EDGE_CURVE('',#8582,#8350,#2110,.T.);
#10777=EDGE_CURVE('',#8581,#8351,#2111,.T.);
#10778=EDGE_CURVE('',#8352,#8353,#1250,.T.);
#10779=EDGE_CURVE('',#8580,#8354,#2112,.T.);
#10780=EDGE_CURVE('',#8579,#8355,#2113,.T.);
#10781=EDGE_CURVE('',#8165,#8160,#1251,.T.);
#10782=EDGE_CURVE('',#8160,#8161,#1252,.T.);
#10783=EDGE_CURVE('',#8577,#8634,#1253,.T.);
#10784=EDGE_CURVE('',#8161,#8634,#1254,.T.);
#10785=EDGE_CURVE('',#8635,#8636,#7463,.T.);
#10786=EDGE_CURVE('',#8635,#8636,#1255,.T.);
#10787=EDGE_CURVE('',#8634,#8635,#1256,.T.);
#10788=EDGE_CURVE('',#8576,#8637,#2114,.T.);
#10789=EDGE_CURVE('',#8636,#8637,#1257,.T.);
#10790=EDGE_CURVE('',#8609,#8638,#2115,.T.);
#10791=EDGE_CURVE('',#8637,#8638,#1258,.T.);
#10792=EDGE_CURVE('',#8639,#8640,#7464,.T.);
#10793=EDGE_CURVE('',#8639,#8640,#1259,.T.);
#10794=EDGE_CURVE('',#8608,#8641,#2116,.T.);
#10795=EDGE_CURVE('',#8640,#8641,#1260,.T.);
#10796=EDGE_CURVE('',#8638,#8639,#1261,.T.);
#10797=EDGE_CURVE('',#8607,#8642,#2117,.T.);
#10798=EDGE_CURVE('',#8641,#8642,#1262,.T.);
#10799=EDGE_CURVE('',#8643,#8644,#7465,.T.);
#10800=EDGE_CURVE('',#8643,#8644,#1263,.T.);
#10801=EDGE_CURVE('',#8606,#8645,#2118,.T.);
#10802=EDGE_CURVE('',#8644,#8645,#1264,.T.);
#10803=EDGE_CURVE('',#8642,#8643,#1265,.T.);
#10804=EDGE_CURVE('',#8605,#8646,#2119,.T.);
#10805=EDGE_CURVE('',#8645,#8646,#1266,.T.);
#10806=EDGE_CURVE('',#8647,#8648,#7466,.T.);
#10807=EDGE_CURVE('',#8647,#8648,#1267,.T.);
#10808=EDGE_CURVE('',#8649,#8604,#1268,.T.);
#10809=EDGE_CURVE('',#8648,#8649,#1269,.T.);
#10810=EDGE_CURVE('',#8646,#8647,#1270,.T.);
#10811=EDGE_CURVE('',#8603,#8650,#1271,.T.);
#10812=EDGE_CURVE('',#8649,#8650,#1272,.T.);
#10813=EDGE_CURVE('',#8651,#8568,#1273,.T.);
#10814=EDGE_CURVE('',#8650,#8651,#1274,.T.);
#10815=EDGE_CURVE('',#8652,#8574,#2120,.T.);
#10816=EDGE_CURVE('',#8651,#8652,#1275,.T.);
#10817=EDGE_CURVE('',#8383,#8602,#2121,.T.);
#10818=EDGE_CURVE('',#8652,#8384,#7467,.T.);
#10819=EDGE_CURVE('',#8653,#8654,#7468,.T.);
#10820=EDGE_CURVE('',#8653,#8654,#1276,.T.);
#10821=EDGE_CURVE('',#8655,#8405,#1277,.T.);
#10822=EDGE_CURVE('',#8655,#8594,#1278,.T.);
#10823=EDGE_CURVE('',#8601,#8656,#1279,.T.);
#10824=EDGE_CURVE('',#8383,#8656,#1280,.T.);
#10825=EDGE_CURVE('',#8657,#8658,#7469,.T.);
#10826=EDGE_CURVE('',#8657,#8658,#7470,.T.);
#10827=EDGE_CURVE('',#8656,#8657,#1281,.T.);
#10828=EDGE_CURVE('',#8600,#8659,#2122,.T.);
#10829=EDGE_CURVE('',#8658,#8659,#1282,.T.);
#10830=EDGE_CURVE('',#8599,#8660,#2123,.T.);
#10831=EDGE_CURVE('',#8659,#8660,#1283,.T.);
#10832=EDGE_CURVE('',#8661,#8662,#7471,.T.);
#10833=EDGE_CURVE('',#8661,#8662,#1284,.T.);
#10834=EDGE_CURVE('',#8598,#8663,#2124,.T.);
#10835=EDGE_CURVE('',#8662,#8663,#1285,.T.);
#10836=EDGE_CURVE('',#8660,#8661,#1286,.T.);
#10837=EDGE_CURVE('',#8597,#8664,#2125,.T.);
#10838=EDGE_CURVE('',#8663,#8664,#1287,.T.);
#10839=EDGE_CURVE('',#8665,#8666,#7472,.T.);
#10840=EDGE_CURVE('',#8665,#8666,#1288,.T.);
#10841=EDGE_CURVE('',#8596,#8667,#2126,.T.);
#10842=EDGE_CURVE('',#8666,#8667,#1289,.T.);
#10843=EDGE_CURVE('',#8664,#8665,#1290,.T.);
#10844=EDGE_CURVE('',#8595,#8668,#2127,.T.);
#10845=EDGE_CURVE('',#8667,#8668,#1291,.T.);
#10846=EDGE_CURVE('',#8654,#8655,#1292,.T.);
#10847=EDGE_CURVE('',#8668,#8653,#1293,.T.);
#10848=EDGE_CURVE('',#8669,#8670,#2128,.T.);
#10849=EDGE_CURVE('',#8671,#8669,#7473,.T.);
#10850=EDGE_CURVE('',#8672,#8671,#2129,.T.);
#10851=EDGE_CURVE('',#8673,#8672,#7474,.T.);
#10852=EDGE_CURVE('',#8674,#8673,#2130,.T.);
#10853=EDGE_CURVE('',#8675,#8674,#7475,.T.);
#10854=EDGE_CURVE('',#8676,#8675,#2131,.T.);
#10855=EDGE_CURVE('',#8670,#8676,#7476,.T.);
#10856=EDGE_CURVE('',#8677,#8678,#7477,.T.);
#10857=EDGE_CURVE('',#8405,#8677,#2132,.T.);
#10858=EDGE_CURVE('',#8678,#8404,#2133,.T.);
#10859=EDGE_CURVE('',#8678,#8679,#7478,.T.);
#10860=EDGE_CURVE('',#8679,#8403,#2134,.T.);
#10861=EDGE_CURVE('',#8679,#8680,#7479,.T.);
#10862=EDGE_CURVE('',#8680,#8402,#2135,.T.);
#10863=EDGE_CURVE('',#8681,#8398,#2136,.T.);
#10864=EDGE_CURVE('',#8680,#8681,#7480,.T.);
#10865=EDGE_CURVE('',#8681,#8682,#7481,.T.);
#10866=EDGE_CURVE('',#8682,#8397,#2137,.T.);
#10867=EDGE_CURVE('',#8682,#8683,#7482,.T.);
#10868=EDGE_CURVE('',#8683,#8393,#2138,.T.);
#10869=EDGE_CURVE('',#8683,#8361,#7483,.T.);
#10870=EDGE_CURVE('',#8360,#8684,#7484,.T.);
#10871=EDGE_CURVE('',#8684,#8165,#2139,.T.);
#10872=EDGE_CURVE('',#8684,#8685,#7485,.T.);
#10873=EDGE_CURVE('',#8685,#8160,#2140,.T.);
#10874=EDGE_CURVE('',#8685,#8686,#7486,.T.);
#10875=EDGE_CURVE('',#8686,#8161,#1294,.T.);
#10876=EDGE_CURVE('',#8687,#8650,#2141,.T.);
#10877=EDGE_CURVE('',#8686,#8687,#7487,.T.);
#10878=EDGE_CURVE('',#8687,#8688,#7488,.T.);
#10879=EDGE_CURVE('',#8688,#8651,#2142,.T.);
#10880=EDGE_CURVE('',#8688,#8689,#7489,.T.);
#10881=EDGE_CURVE('',#8689,#8652,#2143,.T.);
#10882=EDGE_CURVE('',#8689,#8690,#7490,.T.);
#10883=EDGE_CURVE('',#8690,#8383,#2144,.T.);
#10884=EDGE_CURVE('',#8690,#8677,#7491,.T.);
#10885=EDGE_CURVE('',#8674,#8691,#2145,.T.);
#10886=EDGE_CURVE('',#8692,#8673,#2146,.T.);
#10887=EDGE_CURVE('',#8691,#8692,#2147,.T.);
#10888=EDGE_CURVE('',#8676,#8693,#2148,.T.);
#10889=EDGE_CURVE('',#8694,#8675,#2149,.T.);
#10890=EDGE_CURVE('',#8693,#8694,#2150,.T.);
#10891=EDGE_CURVE('',#8695,#8691,#1295,.T.);
#10892=EDGE_CURVE('',#8695,#8696,#7492,.T.);
#10893=EDGE_CURVE('',#8694,#8696,#1296,.T.);
#10894=EDGE_CURVE('',#8669,#8697,#2151,.T.);
#10895=EDGE_CURVE('',#8698,#8670,#2152,.T.);
#10896=EDGE_CURVE('',#8697,#8698,#2153,.T.);
#10897=EDGE_CURVE('',#8699,#8693,#1297,.T.);
#10898=EDGE_CURVE('',#8699,#8700,#7493,.T.);
#10899=EDGE_CURVE('',#8698,#8700,#1298,.T.);
#10900=EDGE_CURVE('',#8701,#8697,#1299,.T.);
#10901=EDGE_CURVE('',#8701,#8702,#7494,.T.);
#10902=EDGE_CURVE('',#8703,#8702,#1300,.T.);
#10903=EDGE_CURVE('',#8671,#8703,#2154,.T.);
#10904=EDGE_CURVE('',#8704,#8672,#2155,.T.);
#10905=EDGE_CURVE('',#8705,#8704,#1301,.T.);
#10906=EDGE_CURVE('',#8705,#8706,#7495,.T.);
#10907=EDGE_CURVE('',#8692,#8706,#1302,.T.);
#10908=EDGE_CURVE('',#8704,#8703,#2156,.T.);
#10909=EDGE_CURVE('',#8707,#8708,#1303,.T.);
#10910=EDGE_CURVE('',#8707,#8709,#2157,.T.);
#10911=EDGE_CURVE('',#8710,#8709,#7496,.T.);
#10912=EDGE_CURVE('',#8708,#8710,#1304,.T.);
#10913=EDGE_CURVE('',#8711,#8707,#1392,.T.);
#10914=EDGE_CURVE('',#8711,#8712,#2158,.T.);
#10915=EDGE_CURVE('',#8709,#8712,#1305,.T.);
#10916=EDGE_CURVE('',#8713,#8711,#1306,.T.);
#10917=EDGE_CURVE('',#8714,#8713,#1307,.T.);
#10918=EDGE_CURVE('',#8712,#8714,#7497,.T.);
#10919=EDGE_CURVE('',#8715,#8716,#2159,.T.);
#10920=EDGE_CURVE('',#8715,#8717,#7498,.T.);
#10921=EDGE_CURVE('',#8718,#8717,#1308,.T.);
#10922=EDGE_CURVE('',#8716,#8718,#1309,.T.);
#10923=EDGE_CURVE('',#8719,#8720,#2160,.T.);
#10924=EDGE_CURVE('',#8715,#8719,#1310,.T.);
#10925=EDGE_CURVE('',#8720,#8716,#1393,.T.);
#10926=EDGE_CURVE('',#8721,#8720,#1311,.T.);
#10927=EDGE_CURVE('',#8722,#8721,#1312,.T.);
#10928=EDGE_CURVE('',#8719,#8722,#7499,.T.);
#10929=EDGE_CURVE('',#8723,#8724,#2161,.T.);
#10930=EDGE_CURVE('',#8723,#8725,#7500,.T.);
#10931=EDGE_CURVE('',#8726,#8725,#1313,.T.);
#10932=EDGE_CURVE('',#8724,#8726,#1314,.T.);
#10933=EDGE_CURVE('',#8727,#8728,#2162,.T.);
#10934=EDGE_CURVE('',#8723,#8727,#1315,.T.);
#10935=EDGE_CURVE('',#8728,#8724,#1394,.T.);
#10936=EDGE_CURVE('',#8729,#8728,#1395,.T.);
#10937=EDGE_CURVE('',#8730,#8729,#1316,.T.);
#10938=EDGE_CURVE('',#8727,#8730,#7501,.T.);
#10939=EDGE_CURVE('',#8731,#8732,#1396,.T.);
#10940=EDGE_CURVE('',#8731,#8733,#2163,.T.);
#10941=EDGE_CURVE('',#8734,#8733,#7502,.T.);
#10942=EDGE_CURVE('',#8732,#8734,#1317,.T.);
#10943=EDGE_CURVE('',#8735,#8731,#1397,.T.);
#10944=EDGE_CURVE('',#8735,#8736,#2164,.T.);
#10945=EDGE_CURVE('',#8733,#8736,#1318,.T.);
#10946=EDGE_CURVE('',#8737,#8735,#1319,.T.);
#10947=EDGE_CURVE('',#8738,#8737,#1320,.T.);
#10948=EDGE_CURVE('',#8736,#8738,#7503,.T.);
#10949=EDGE_CURVE('',#8721,#8342,#7504,.T.);
#10950=EDGE_CURVE('',#8739,#8718,#7505,.T.);
#10951=EDGE_CURVE('',#8740,#8739,#7506,.T.);
#10952=EDGE_CURVE('',#8713,#8740,#7507,.T.);
#10953=EDGE_CURVE('',#8741,#8708,#7508,.T.);
#10954=EDGE_CURVE('',#8742,#8741,#7509,.T.);
#10955=EDGE_CURVE('',#8737,#8742,#7510,.T.);
#10956=EDGE_CURVE('',#8743,#8732,#7511,.T.);
#10957=EDGE_CURVE('',#8744,#8743,#7512,.T.);
#10958=EDGE_CURVE('',#8729,#8744,#7513,.T.);
#10959=EDGE_CURVE('',#8343,#8726,#7514,.T.);
#10960=EDGE_CURVE('',#8745,#8746,#2165,.T.);
#10961=EDGE_CURVE('',#8746,#8747,#2166,.T.);
#10962=EDGE_CURVE('',#8747,#8748,#2167,.T.);
#10963=EDGE_CURVE('',#8748,#8749,#2168,.T.);
#10964=EDGE_CURVE('',#8749,#8750,#2169,.T.);
#10965=EDGE_CURVE('',#8750,#8745,#2170,.T.);
#10966=EDGE_CURVE('',#8751,#8752,#2171,.T.);
#10967=EDGE_CURVE('',#8752,#8753,#2172,.T.);
#10968=EDGE_CURVE('',#8753,#8754,#2173,.T.);
#10969=EDGE_CURVE('',#8754,#8755,#2174,.T.);
#10970=EDGE_CURVE('',#8755,#8756,#2175,.T.);
#10971=EDGE_CURVE('',#8756,#8751,#2176,.T.);
#10972=EDGE_CURVE('',#8706,#8695,#2177,.T.);
#10973=EDGE_CURVE('',#8696,#8699,#2178,.T.);
#10974=EDGE_CURVE('',#8700,#8701,#2179,.T.);
#10975=EDGE_CURVE('',#8702,#8705,#2180,.T.);
#10976=EDGE_CURVE('',#8757,#8758,#7515,.T.);
#10977=EDGE_CURVE('',#8741,#8757,#2181,.T.);
#10978=EDGE_CURVE('',#8758,#8708,#1321,.T.);
#10979=EDGE_CURVE('',#8759,#8710,#2182,.T.);
#10980=EDGE_CURVE('',#8758,#8759,#2183,.T.);
#10981=EDGE_CURVE('',#8760,#8714,#2184,.T.);
#10982=EDGE_CURVE('',#8759,#8760,#2185,.T.);
#10983=EDGE_CURVE('',#8761,#8713,#1322,.T.);
#10984=EDGE_CURVE('',#8760,#8761,#2186,.T.);
#10985=EDGE_CURVE('',#8761,#8762,#7516,.T.);
#10986=EDGE_CURVE('',#8762,#8740,#2187,.T.);
#10987=EDGE_CURVE('',#8763,#8739,#2188,.T.);
#10988=EDGE_CURVE('',#8762,#8763,#7517,.T.);
#10989=EDGE_CURVE('',#8763,#8764,#7518,.T.);
#10990=EDGE_CURVE('',#8764,#8718,#1323,.T.);
#10991=EDGE_CURVE('',#8765,#8717,#2189,.T.);
#10992=EDGE_CURVE('',#8764,#8765,#2190,.T.);
#10993=EDGE_CURVE('',#8766,#8722,#2191,.T.);
#10994=EDGE_CURVE('',#8765,#8766,#2192,.T.);
#10995=EDGE_CURVE('',#8767,#8721,#1324,.T.);
#10996=EDGE_CURVE('',#8766,#8767,#2193,.T.);
#10997=EDGE_CURVE('',#8767,#8345,#7519,.T.);
#10998=EDGE_CURVE('',#8344,#8768,#7520,.T.);
#10999=EDGE_CURVE('',#8768,#8726,#1325,.T.);
#11000=EDGE_CURVE('',#8769,#8725,#2194,.T.);
#11001=EDGE_CURVE('',#8768,#8769,#2195,.T.);
#11002=EDGE_CURVE('',#8770,#8730,#2196,.T.);
#11003=EDGE_CURVE('',#8769,#8770,#2197,.T.);
#11004=EDGE_CURVE('',#8771,#8729,#1326,.T.);
#11005=EDGE_CURVE('',#8770,#8771,#2198,.T.);
#11006=EDGE_CURVE('',#8771,#8772,#7521,.T.);
#11007=EDGE_CURVE('',#8772,#8744,#2199,.T.);
#11008=EDGE_CURVE('',#8773,#8743,#2200,.T.);
#11009=EDGE_CURVE('',#8772,#8773,#7522,.T.);
#11010=EDGE_CURVE('',#8773,#8774,#7523,.T.);
#11011=EDGE_CURVE('',#8774,#8732,#1327,.T.);
#11012=EDGE_CURVE('',#8775,#8734,#2201,.T.);
#11013=EDGE_CURVE('',#8774,#8775,#2202,.T.);
#11014=EDGE_CURVE('',#8776,#8738,#2203,.T.);
#11015=EDGE_CURVE('',#8775,#8776,#2204,.T.);
#11016=EDGE_CURVE('',#8777,#8737,#1328,.T.);
#11017=EDGE_CURVE('',#8776,#8777,#2205,.T.);
#11018=EDGE_CURVE('',#8777,#8778,#7524,.T.);
#11019=EDGE_CURVE('',#8778,#8742,#2206,.T.);
#11020=EDGE_CURVE('',#8778,#8757,#7525,.T.);
#11021=EDGE_CURVE('',#8779,#8745,#2207,.T.);
#11022=EDGE_CURVE('',#8750,#8780,#2208,.T.);
#11023=EDGE_CURVE('',#8779,#8780,#2209,.T.);
#11024=EDGE_CURVE('',#8749,#8781,#2210,.T.);
#11025=EDGE_CURVE('',#8780,#8781,#2211,.T.);
#11026=EDGE_CURVE('',#8748,#8782,#2212,.T.);
#11027=EDGE_CURVE('',#8781,#8782,#2213,.T.);
#11028=EDGE_CURVE('',#8747,#8783,#2214,.T.);
#11029=EDGE_CURVE('',#8782,#8783,#2215,.T.);
#11030=EDGE_CURVE('',#8746,#8784,#2216,.T.);
#11031=EDGE_CURVE('',#8783,#8784,#2217,.T.);
#11032=EDGE_CURVE('',#8784,#8779,#2218,.T.);
#11033=EDGE_CURVE('',#8785,#8751,#2219,.T.);
#11034=EDGE_CURVE('',#8756,#8786,#2220,.T.);
#11035=EDGE_CURVE('',#8785,#8786,#2221,.T.);
#11036=EDGE_CURVE('',#8755,#8787,#2222,.T.);
#11037=EDGE_CURVE('',#8786,#8787,#2223,.T.);
#11038=EDGE_CURVE('',#8754,#8788,#2224,.T.);
#11039=EDGE_CURVE('',#8787,#8788,#2225,.T.);
#11040=EDGE_CURVE('',#8753,#8789,#2226,.T.);
#11041=EDGE_CURVE('',#8788,#8789,#2227,.T.);
#11042=EDGE_CURVE('',#8752,#8790,#2228,.T.);
#11043=EDGE_CURVE('',#8789,#8790,#2229,.T.);
#11044=EDGE_CURVE('',#8790,#8785,#2230,.T.);
#11045=EDGE_CURVE('',#8791,#8792,#7526,.T.);
#11046=EDGE_CURVE('',#8793,#8791,#2231,.T.);
#11047=EDGE_CURVE('',#8793,#8794,#7527,.T.);
#11048=EDGE_CURVE('',#8792,#8794,#2232,.T.);
#11049=EDGE_CURVE('',#8795,#8796,#7528,.T.);
#11050=EDGE_CURVE('',#8797,#8796,#2233,.T.);
#11051=EDGE_CURVE('',#8798,#8797,#7529,.T.);
#11052=EDGE_CURVE('',#8795,#8798,#2234,.T.);
#11053=EDGE_CURVE('',#8799,#8800,#2235,.T.);
#11054=EDGE_CURVE('',#8800,#8801,#2236,.T.);
#11055=EDGE_CURVE('',#8801,#8802,#2237,.T.);
#11056=EDGE_CURVE('',#8802,#8799,#2238,.T.);
#11057=EDGE_CURVE('',#8803,#8804,#2239,.T.);
#11058=EDGE_CURVE('',#8805,#8803,#7530,.T.);
#11059=EDGE_CURVE('',#8806,#8805,#2240,.T.);
#11060=EDGE_CURVE('',#8806,#8801,#2241,.T.);
#11061=EDGE_CURVE('',#8800,#8804,#2242,.T.);
#11062=EDGE_CURVE('',#8805,#8807,#2243,.T.);
#11063=EDGE_CURVE('',#8808,#8803,#2244,.T.);
#11064=EDGE_CURVE('',#8807,#8808,#7531,.T.);
#11065=EDGE_CURVE('',#8809,#8810,#7532,.T.);
#11066=EDGE_CURVE('',#8811,#8810,#2245,.T.);
#11067=EDGE_CURVE('',#8812,#8811,#7533,.T.);
#11068=EDGE_CURVE('',#8809,#8812,#2246,.T.);
#11069=EDGE_CURVE('',#8813,#8814,#7534,.T.);
#11070=EDGE_CURVE('',#8815,#8813,#2247,.T.);
#11071=EDGE_CURVE('',#8815,#8816,#7535,.T.);
#11072=EDGE_CURVE('',#8814,#8816,#2248,.T.);
#11073=EDGE_CURVE('',#8817,#8818,#7536,.T.);
#11074=EDGE_CURVE('',#8819,#8818,#2249,.T.);
#11075=EDGE_CURVE('',#8820,#8819,#7537,.T.);
#11076=EDGE_CURVE('',#8817,#8820,#2250,.T.);
#11077=EDGE_CURVE('',#8813,#8819,#2251,.T.);
#11078=EDGE_CURVE('',#8812,#8814,#2252,.T.);
#11079=EDGE_CURVE('',#8807,#8811,#2253,.T.);
#11080=EDGE_CURVE('',#8798,#8808,#2254,.T.);
#11081=EDGE_CURVE('',#8791,#8797,#2255,.T.);
#11082=EDGE_CURVE('',#8821,#8792,#2256,.T.);
#11083=EDGE_CURVE('',#8822,#8821,#7538,.T.);
#11084=EDGE_CURVE('',#8339,#8822,#2257,.T.);
#11085=EDGE_CURVE('',#8820,#8338,#2258,.T.);
#11086=EDGE_CURVE('',#8823,#8824,#7539,.T.);
#11087=EDGE_CURVE('',#8822,#8824,#2259,.T.);
#11088=EDGE_CURVE('',#8823,#8821,#2260,.T.);
#11089=EDGE_CURVE('',#8794,#8825,#2261,.T.);
#11090=EDGE_CURVE('',#8825,#8826,#2262,.T.);
#11091=EDGE_CURVE('',#8826,#8823,#2263,.T.);
#11092=EDGE_CURVE('',#8796,#8827,#2264,.T.);
#11093=EDGE_CURVE('',#8827,#8828,#2265,.T.);
#11094=EDGE_CURVE('',#8828,#8793,#2266,.T.);
#11095=EDGE_CURVE('',#8828,#8829,#2267,.T.);
#11096=EDGE_CURVE('',#8830,#8829,#7540,.T.);
#11097=EDGE_CURVE('',#8830,#8831,#2268,.T.);
#11098=EDGE_CURVE('',#8831,#8832,#2269,.T.);
#11099=EDGE_CURVE('',#8832,#8833,#2270,.T.);
#11100=EDGE_CURVE('',#8834,#8833,#7541,.T.);
#11101=EDGE_CURVE('',#8834,#8825,#2271,.T.);
#11102=EDGE_CURVE('',#8835,#8836,#2272,.T.);
#11103=EDGE_CURVE('',#8837,#8836,#7542,.T.);
#11104=EDGE_CURVE('',#8837,#8838,#2273,.T.);
#11105=EDGE_CURVE('',#8838,#8835,#7543,.T.);
#11106=EDGE_CURVE('',#8804,#8839,#2274,.T.);
#11107=EDGE_CURVE('',#8839,#8840,#2275,.T.);
#11108=EDGE_CURVE('',#8840,#8841,#2276,.T.);
#11109=EDGE_CURVE('',#8841,#8795,#2277,.T.);
#11110=EDGE_CURVE('',#8841,#8835,#2278,.T.);
#11111=EDGE_CURVE('',#8838,#8827,#2279,.T.);
#11112=EDGE_CURVE('',#8842,#8843,#2280,.T.);
#11113=EDGE_CURVE('',#8844,#8842,#7544,.T.);
#11114=EDGE_CURVE('',#8844,#8840,#2281,.T.);
#11115=EDGE_CURVE('',#8839,#8843,#2282,.T.);
#11116=EDGE_CURVE('',#8845,#8843,#2283,.T.);
#11117=EDGE_CURVE('',#8799,#8845,#2284,.T.);
#11118=EDGE_CURVE('',#8846,#8847,#2285,.T.);
#11119=EDGE_CURVE('',#8847,#8802,#2286,.T.);
#11120=EDGE_CURVE('',#8848,#8806,#2287,.T.);
#11121=EDGE_CURVE('',#8848,#8846,#2288,.T.);
#11122=EDGE_CURVE('',#8847,#8849,#2289,.T.);
#11123=EDGE_CURVE('',#8849,#8850,#2290,.T.);
#11124=EDGE_CURVE('',#8850,#8845,#2291,.T.);
#11125=EDGE_CURVE('',#8851,#8852,#2292,.T.);
#11126=EDGE_CURVE('',#8852,#8848,#2293,.T.);
#11127=EDGE_CURVE('',#8810,#8851,#2294,.T.);
#11128=EDGE_CURVE('',#8852,#8853,#2295,.T.);
#11129=EDGE_CURVE('',#8854,#8853,#7545,.T.);
#11130=EDGE_CURVE('',#8854,#8846,#2296,.T.);
#11131=EDGE_CURVE('',#8855,#8856,#2297,.T.);
#11132=EDGE_CURVE('',#8857,#8856,#7546,.T.);
#11133=EDGE_CURVE('',#8857,#8858,#2298,.T.);
#11134=EDGE_CURVE('',#8858,#8855,#7547,.T.);
#11135=EDGE_CURVE('',#8816,#8859,#2299,.T.);
#11136=EDGE_CURVE('',#8859,#8860,#2300,.T.);
#11137=EDGE_CURVE('',#8860,#8809,#2301,.T.);
#11138=EDGE_CURVE('',#8860,#8855,#2302,.T.);
#11139=EDGE_CURVE('',#8858,#8851,#2303,.T.);
#11140=EDGE_CURVE('',#8818,#8861,#2304,.T.);
#11141=EDGE_CURVE('',#8861,#8862,#2305,.T.);
#11142=EDGE_CURVE('',#8862,#8815,#2306,.T.);
#11143=EDGE_CURVE('',#8862,#8863,#2307,.T.);
#11144=EDGE_CURVE('',#8864,#8863,#7548,.T.);
#11145=EDGE_CURVE('',#8864,#8865,#2308,.T.);
#11146=EDGE_CURVE('',#8865,#8866,#2309,.T.);
#11147=EDGE_CURVE('',#8866,#8867,#2310,.T.);
#11148=EDGE_CURVE('',#8868,#8867,#7549,.T.);
#11149=EDGE_CURVE('',#8868,#8859,#2311,.T.);
#11150=EDGE_CURVE('',#8869,#8870,#2312,.T.);
#11151=EDGE_CURVE('',#8871,#8870,#7550,.T.);
#11152=EDGE_CURVE('',#8871,#8872,#2313,.T.);
#11153=EDGE_CURVE('',#8872,#8869,#7551,.T.);
#11154=EDGE_CURVE('',#8337,#8873,#2314,.T.);
#11155=EDGE_CURVE('',#8873,#8874,#2315,.T.);
#11156=EDGE_CURVE('',#8874,#8817,#2316,.T.);
#11157=EDGE_CURVE('',#8874,#8869,#2317,.T.);
#11158=EDGE_CURVE('',#8872,#8861,#2318,.T.);
#11159=EDGE_CURVE('',#8875,#8876,#2319,.T.);
#11160=EDGE_CURVE('',#8877,#8876,#7552,.T.);
#11161=EDGE_CURVE('',#8877,#8878,#2320,.T.);
#11162=EDGE_CURVE('',#8878,#8875,#7553,.T.);
#11163=EDGE_CURVE('',#8826,#8875,#2321,.T.);
#11164=EDGE_CURVE('',#8878,#8879,#2322,.T.);
#11165=EDGE_CURVE('',#8824,#8879,#2323,.T.);
#11166=EDGE_CURVE('',#8879,#8880,#2324,.T.);
#11167=EDGE_CURVE('',#8880,#8336,#2325,.T.);
#11168=EDGE_CURVE('',#8880,#8881,#2326,.T.);
#11169=EDGE_CURVE('',#8882,#8881,#7554,.T.);
#11170=EDGE_CURVE('',#8882,#8883,#2327,.T.);
#11171=EDGE_CURVE('',#8883,#8884,#2328,.T.);
#11172=EDGE_CURVE('',#8884,#8885,#2329,.T.);
#11173=EDGE_CURVE('',#8886,#8885,#7555,.T.);
#11174=EDGE_CURVE('',#8886,#8873,#2330,.T.);
#11175=EDGE_CURVE('',#8887,#8888,#2331,.T.);
#11176=EDGE_CURVE('',#8888,#8889,#2332,.T.);
#11177=EDGE_CURVE('',#8889,#8890,#2333,.T.);
#11178=EDGE_CURVE('',#8890,#8891,#2334,.T.);
#11179=EDGE_CURVE('',#8891,#8892,#2335,.T.);
#11180=EDGE_CURVE('',#8892,#8887,#2336,.T.);
#11181=EDGE_CURVE('',#8893,#8894,#2337,.T.);
#11182=EDGE_CURVE('',#8894,#8895,#2338,.T.);
#11183=EDGE_CURVE('',#8896,#8895,#2339,.T.);
#11184=EDGE_CURVE('',#8896,#8893,#2340,.T.);
#11185=EDGE_CURVE('',#8897,#8898,#2341,.T.);
#11186=EDGE_CURVE('',#8898,#8877,#2342,.T.);
#11187=EDGE_CURVE('',#8876,#8899,#2343,.T.);
#11188=EDGE_CURVE('',#8899,#8900,#2344,.T.);
#11189=EDGE_CURVE('',#8897,#8900,#7556,.T.);
#11190=EDGE_CURVE('',#8900,#8901,#2345,.T.);
#11191=EDGE_CURVE('',#8901,#8902,#7557,.T.);
#11192=EDGE_CURVE('',#8902,#8897,#2346,.T.);
#11193=EDGE_CURVE('',#8903,#8834,#2347,.T.);
#11194=EDGE_CURVE('',#8904,#8903,#2348,.T.);
#11195=EDGE_CURVE('',#8904,#8899,#2349,.T.);
#11196=EDGE_CURVE('',#8833,#8905,#2350,.T.);
#11197=EDGE_CURVE('',#8903,#8905,#7558,.T.);
#11198=EDGE_CURVE('',#8832,#8906,#2351,.T.);
#11199=EDGE_CURVE('',#8905,#8906,#2352,.T.);
#11200=EDGE_CURVE('',#8831,#8907,#2353,.T.);
#11201=EDGE_CURVE('',#8906,#8907,#2354,.T.);
#11202=EDGE_CURVE('',#8908,#8830,#2355,.T.);
#11203=EDGE_CURVE('',#8907,#8908,#2356,.T.);
#11204=EDGE_CURVE('',#8829,#8909,#2357,.T.);
#11205=EDGE_CURVE('',#8908,#8909,#7559,.T.);
#11206=EDGE_CURVE('',#8910,#8837,#2358,.T.);
#11207=EDGE_CURVE('',#8910,#8911,#2359,.T.);
#11208=EDGE_CURVE('',#8909,#8911,#2360,.T.);
#11209=EDGE_CURVE('',#8912,#8910,#2361,.T.);
#11210=EDGE_CURVE('',#8836,#8913,#2362,.T.);
#11211=EDGE_CURVE('',#8913,#8914,#2363,.T.);
#11212=EDGE_CURVE('',#8912,#8914,#7560,.T.);
#11213=EDGE_CURVE('',#8914,#8915,#2364,.T.);
#11214=EDGE_CURVE('',#8915,#8916,#7561,.T.);
#11215=EDGE_CURVE('',#8916,#8912,#2365,.T.);
#11216=EDGE_CURVE('',#8917,#8844,#2366,.T.);
#11217=EDGE_CURVE('',#8918,#8917,#2367,.T.);
#11218=EDGE_CURVE('',#8918,#8913,#2368,.T.);
#11219=EDGE_CURVE('',#8842,#8919,#2369,.T.);
#11220=EDGE_CURVE('',#8917,#8919,#7562,.T.);
#11221=EDGE_CURVE('',#8850,#8920,#2370,.T.);
#11222=EDGE_CURVE('',#8919,#8920,#2371,.T.);
#11223=EDGE_CURVE('',#8849,#8921,#2372,.T.);
#11224=EDGE_CURVE('',#8920,#8921,#2373,.T.);
#11225=EDGE_CURVE('',#8922,#8854,#2374,.T.);
#11226=EDGE_CURVE('',#8921,#8922,#2375,.T.);
#11227=EDGE_CURVE('',#8853,#8923,#2376,.T.);
#11228=EDGE_CURVE('',#8922,#8923,#7563,.T.);
#11229=EDGE_CURVE('',#8924,#8857,#2377,.T.);
#11230=EDGE_CURVE('',#8924,#8925,#2378,.T.);
#11231=EDGE_CURVE('',#8923,#8925,#2379,.T.);
#11232=EDGE_CURVE('',#8926,#8924,#2380,.T.);
#11233=EDGE_CURVE('',#8856,#8927,#2381,.T.);
#11234=EDGE_CURVE('',#8927,#8928,#2382,.T.);
#11235=EDGE_CURVE('',#8926,#8928,#7564,.T.);
#11236=EDGE_CURVE('',#8928,#8929,#2383,.T.);
#11237=EDGE_CURVE('',#8929,#8930,#7565,.T.);
#11238=EDGE_CURVE('',#8930,#8926,#2384,.T.);
#11239=EDGE_CURVE('',#8931,#8868,#2385,.T.);
#11240=EDGE_CURVE('',#8932,#8931,#2386,.T.);
#11241=EDGE_CURVE('',#8932,#8927,#2387,.T.);
#11242=EDGE_CURVE('',#8867,#8933,#2388,.T.);
#11243=EDGE_CURVE('',#8931,#8933,#7566,.T.);
#11244=EDGE_CURVE('',#8866,#8934,#2389,.T.);
#11245=EDGE_CURVE('',#8933,#8934,#2390,.T.);
#11246=EDGE_CURVE('',#8865,#8935,#2391,.T.);
#11247=EDGE_CURVE('',#8934,#8935,#2392,.T.);
#11248=EDGE_CURVE('',#8936,#8864,#2393,.T.);
#11249=EDGE_CURVE('',#8935,#8936,#2394,.T.);
#11250=EDGE_CURVE('',#8863,#8937,#2395,.T.);
#11251=EDGE_CURVE('',#8936,#8937,#7567,.T.);
#11252=EDGE_CURVE('',#8938,#8871,#2396,.T.);
#11253=EDGE_CURVE('',#8938,#8939,#2397,.T.);
#11254=EDGE_CURVE('',#8937,#8939,#2398,.T.);
#11255=EDGE_CURVE('',#8940,#8938,#2399,.T.);
#11256=EDGE_CURVE('',#8870,#8941,#2400,.T.);
#11257=EDGE_CURVE('',#8941,#8942,#2401,.T.);
#11258=EDGE_CURVE('',#8940,#8942,#7568,.T.);
#11259=EDGE_CURVE('',#8942,#8943,#2402,.T.);
#11260=EDGE_CURVE('',#8943,#8944,#7569,.T.);
#11261=EDGE_CURVE('',#8944,#8940,#2403,.T.);
#11262=EDGE_CURVE('',#8945,#8886,#2404,.T.);
#11263=EDGE_CURVE('',#8946,#8945,#2405,.T.);
#11264=EDGE_CURVE('',#8946,#8941,#2406,.T.);
#11265=EDGE_CURVE('',#8885,#8947,#2407,.T.);
#11266=EDGE_CURVE('',#8945,#8947,#7570,.T.);
#11267=EDGE_CURVE('',#8884,#8948,#2408,.T.);
#11268=EDGE_CURVE('',#8947,#8948,#2409,.T.);
#11269=EDGE_CURVE('',#8883,#8949,#2410,.T.);
#11270=EDGE_CURVE('',#8948,#8949,#2411,.T.);
#11271=EDGE_CURVE('',#8950,#8882,#2412,.T.);
#11272=EDGE_CURVE('',#8949,#8950,#2413,.T.);
#11273=EDGE_CURVE('',#8881,#8951,#2414,.T.);
#11274=EDGE_CURVE('',#8950,#8951,#7571,.T.);
#11275=EDGE_CURVE('',#8898,#8952,#2415,.T.);
#11276=EDGE_CURVE('',#8951,#8952,#2416,.T.);
#11277=EDGE_CURVE('',#8892,#8953,#2417,.T.);
#11278=EDGE_CURVE('',#8954,#8953,#2418,.T.);
#11279=EDGE_CURVE('',#8954,#8887,#2419,.T.);
#11280=EDGE_CURVE('',#8891,#8955,#2420,.T.);
#11281=EDGE_CURVE('',#8953,#8955,#2421,.T.);
#11282=EDGE_CURVE('',#8890,#8956,#2422,.T.);
#11283=EDGE_CURVE('',#8955,#8956,#2423,.T.);
#11284=EDGE_CURVE('',#8889,#8957,#2424,.T.);
#11285=EDGE_CURVE('',#8956,#8957,#2425,.T.);
#11286=EDGE_CURVE('',#8888,#8958,#2426,.T.);
#11287=EDGE_CURVE('',#8957,#8958,#2427,.T.);
#11288=EDGE_CURVE('',#8958,#8954,#2428,.T.);
#11289=EDGE_CURVE('',#8895,#8317,#2429,.T.);
#11290=EDGE_CURVE('',#8894,#8318,#2430,.T.);
#11291=EDGE_CURVE('',#8893,#8313,#2431,.T.);
#11292=EDGE_CURVE('',#8314,#8896,#2432,.T.);
#11293=EDGE_CURVE('',#8902,#8959,#2433,.T.);
#11294=EDGE_CURVE('',#8960,#8959,#2434,.T.);
#11295=EDGE_CURVE('',#8952,#8960,#2435,.T.);
#11296=EDGE_CURVE('',#8961,#8962,#2436,.T.);
#11297=EDGE_CURVE('',#8963,#8961,#7572,.T.);
#11298=EDGE_CURVE('',#8964,#8963,#2437,.T.);
#11299=EDGE_CURVE('',#8959,#8964,#7573,.T.);
#11300=EDGE_CURVE('',#8901,#8965,#2438,.T.);
#11301=EDGE_CURVE('',#8962,#8965,#7574,.T.);
#11302=EDGE_CURVE('',#8966,#8904,#2439,.T.);
#11303=EDGE_CURVE('',#8965,#8966,#2440,.T.);
#11304=EDGE_CURVE('',#8911,#8967,#2441,.T.);
#11305=EDGE_CURVE('',#8966,#8967,#7575,.T.);
#11306=EDGE_CURVE('',#8916,#8968,#2442,.T.);
#11307=EDGE_CURVE('',#8967,#8968,#2443,.T.);
#11308=EDGE_CURVE('',#8969,#8300,#2444,.T.);
#11309=EDGE_CURVE('',#8970,#8969,#7576,.T.);
#11310=EDGE_CURVE('',#8971,#8970,#2445,.T.);
#11311=EDGE_CURVE('',#8968,#8971,#7577,.T.);
#11312=EDGE_CURVE('',#8915,#8301,#2446,.T.);
#11313=EDGE_CURVE('',#8296,#8918,#2447,.T.);
#11314=EDGE_CURVE('',#8925,#8297,#2448,.T.);
#11315=EDGE_CURVE('',#8930,#8298,#2449,.T.);
#11316=EDGE_CURVE('',#8929,#8972,#2450,.T.);
#11317=EDGE_CURVE('',#8973,#8972,#7578,.T.);
#11318=EDGE_CURVE('',#8974,#8973,#2451,.T.);
#11319=EDGE_CURVE('',#8975,#8974,#7579,.T.);
#11320=EDGE_CURVE('',#8299,#8975,#2452,.T.);
#11321=EDGE_CURVE('',#8976,#8932,#2453,.T.);
#11322=EDGE_CURVE('',#8972,#8976,#2454,.T.);
#11323=EDGE_CURVE('',#8939,#8977,#2455,.T.);
#11324=EDGE_CURVE('',#8976,#8977,#7580,.T.);
#11325=EDGE_CURVE('',#8944,#8978,#2456,.T.);
#11326=EDGE_CURVE('',#8977,#8978,#2457,.T.);
#11327=EDGE_CURVE('',#8943,#8979,#2458,.T.);
#11328=EDGE_CURVE('',#8980,#8979,#7581,.T.);
#11329=EDGE_CURVE('',#8981,#8980,#2459,.T.);
#11330=EDGE_CURVE('',#8982,#8981,#7582,.T.);
#11331=EDGE_CURVE('',#8983,#8982,#2460,.T.);
#11332=EDGE_CURVE('',#8978,#8983,#7583,.T.);
#11333=EDGE_CURVE('',#8984,#8946,#2461,.T.);
#11334=EDGE_CURVE('',#8979,#8984,#2462,.T.);
#11335=EDGE_CURVE('',#8984,#8960,#7584,.T.);
#11336=EDGE_CURVE('',#8985,#8986,#2463,.T.);
#11337=EDGE_CURVE('',#8986,#8987,#2464,.T.);
#11338=EDGE_CURVE('',#8987,#8988,#2465,.T.);
#11339=EDGE_CURVE('',#8988,#8989,#2466,.T.);
#11340=EDGE_CURVE('',#8989,#8990,#2467,.T.);
#11341=EDGE_CURVE('',#8990,#8985,#2468,.T.);
#11342=EDGE_CURVE('',#8273,#8963,#2469,.T.);
#11343=EDGE_CURVE('',#8272,#8964,#2470,.T.);
#11344=EDGE_CURVE('',#8274,#8961,#2471,.T.);
#11345=EDGE_CURVE('',#8275,#8962,#2472,.T.);
#11346=EDGE_CURVE('',#8279,#8971,#2473,.T.);
#11347=EDGE_CURVE('',#8280,#8970,#2474,.T.);
#11348=EDGE_CURVE('',#8281,#8969,#2475,.T.);
#11349=EDGE_CURVE('',#8284,#8975,#2476,.T.);
#11350=EDGE_CURVE('',#8285,#8974,#2477,.T.);
#11351=EDGE_CURVE('',#8267,#8973,#2478,.T.);
#11352=EDGE_CURVE('',#8268,#8983,#2479,.T.);
#11353=EDGE_CURVE('',#8269,#8982,#2480,.T.);
#11354=EDGE_CURVE('',#8270,#8981,#2481,.T.);
#11355=EDGE_CURVE('',#8271,#8980,#2482,.T.);
#11356=EDGE_CURVE('',#8991,#8992,#2483,.T.);
#11357=EDGE_CURVE('',#8993,#8991,#2484,.T.);
#11358=EDGE_CURVE('',#8994,#8993,#2485,.T.);
#11359=EDGE_CURVE('',#8995,#8994,#2486,.T.);
#11360=EDGE_CURVE('',#8996,#8995,#2487,.T.);
#11361=EDGE_CURVE('',#8997,#8996,#2488,.T.);
#11362=EDGE_CURVE('',#8998,#8997,#2489,.T.);
#11363=EDGE_CURVE('',#8992,#8998,#2490,.T.);
#11364=EDGE_CURVE('',#8292,#8995,#7585,.T.);
#11365=EDGE_CURVE('',#8996,#8293,#7586,.T.);
#11366=EDGE_CURVE('',#8999,#8294,#7587,.T.);
#11367=EDGE_CURVE('',#9000,#8999,#2491,.T.);
#11368=EDGE_CURVE('',#8295,#9000,#7588,.T.);
#11369=EDGE_CURVE('',#9001,#9002,#2492,.T.);
#11370=EDGE_CURVE('',#9003,#9001,#2493,.T.);
#11371=EDGE_CURVE('',#9004,#9003,#2494,.T.);
#11372=EDGE_CURVE('',#9004,#9005,#2495,.T.);
#11373=EDGE_CURVE('',#9006,#9005,#2496,.T.);
#11374=EDGE_CURVE('',#9000,#9006,#2497,.T.);
#11375=EDGE_CURVE('',#9002,#8999,#2498,.T.);
#11376=EDGE_CURVE('',#9007,#9008,#2499,.T.);
#11377=EDGE_CURVE('',#9008,#9009,#2500,.T.);
#11378=EDGE_CURVE('',#9009,#9010,#2501,.T.);
#11379=EDGE_CURVE('',#9010,#9011,#2502,.T.);
#11380=EDGE_CURVE('',#9011,#9012,#2503,.T.);
#11381=EDGE_CURVE('',#9012,#9007,#2504,.T.);
#11382=EDGE_CURVE('',#8266,#8227,#1329,.T.);
#11383=EDGE_CURVE('',#8989,#9013,#2505,.T.);
#11384=EDGE_CURVE('',#9013,#9014,#2506,.T.);
#11385=EDGE_CURVE('',#9014,#8990,#2507,.T.);
#11386=EDGE_CURVE('',#9014,#9015,#2508,.T.);
#11387=EDGE_CURVE('',#9015,#8985,#2509,.T.);
#11388=EDGE_CURVE('',#9015,#9016,#2510,.T.);
#11389=EDGE_CURVE('',#9016,#8986,#2511,.T.);
#11390=EDGE_CURVE('',#9016,#9017,#2512,.T.);
#11391=EDGE_CURVE('',#9017,#8987,#2513,.T.);
#11392=EDGE_CURVE('',#9017,#9018,#2514,.T.);
#11393=EDGE_CURVE('',#9018,#8988,#2515,.T.);
#11394=EDGE_CURVE('',#9018,#9013,#2516,.T.);
#11395=EDGE_CURVE('',#9019,#8265,#2517,.T.);
#11396=EDGE_CURVE('',#9019,#9020,#7589,.T.);
#11397=EDGE_CURVE('',#8228,#9020,#2518,.T.);
#11398=EDGE_CURVE('',#8255,#9003,#7590,.T.);
#11399=EDGE_CURVE('',#9004,#8256,#7591,.T.);
#11400=EDGE_CURVE('',#9021,#9022,#1398,.T.);
#11401=EDGE_CURVE('',#9021,#9022,#7592,.T.);
#11402=EDGE_CURVE('',#8289,#9021,#2519,.T.);
#11403=EDGE_CURVE('',#9022,#8288,#2520,.T.);
#11404=EDGE_CURVE('',#9023,#9024,#2521,.T.);
#11405=EDGE_CURVE('',#9024,#9025,#2522,.T.);
#11406=EDGE_CURVE('',#9025,#9026,#2523,.T.);
#11407=EDGE_CURVE('',#9026,#9027,#2524,.T.);
#11408=EDGE_CURVE('',#9027,#9028,#2525,.T.);
#11409=EDGE_CURVE('',#9028,#9023,#2526,.T.);
#11410=EDGE_CURVE('',#9029,#9030,#2527,.T.);
#11411=EDGE_CURVE('',#9030,#9031,#2528,.T.);
#11412=EDGE_CURVE('',#9031,#9032,#2529,.T.);
#11413=EDGE_CURVE('',#9032,#9033,#2530,.T.);
#11414=EDGE_CURVE('',#9033,#9034,#2531,.T.);
#11415=EDGE_CURVE('',#9034,#9029,#2532,.T.);
#11416=EDGE_CURVE('',#9035,#9036,#2533,.T.);
#11417=EDGE_CURVE('',#9036,#9037,#2534,.T.);
#11418=EDGE_CURVE('',#9037,#9038,#2535,.T.);
#11419=EDGE_CURVE('',#9038,#9039,#2536,.T.);
#11420=EDGE_CURVE('',#9039,#9040,#2537,.T.);
#11421=EDGE_CURVE('',#9040,#9035,#2538,.T.);
#11422=EDGE_CURVE('',#9003,#9041,#7593,.T.);
#11423=EDGE_CURVE('',#9041,#9001,#2539,.T.);
#11424=EDGE_CURVE('',#9042,#9002,#2540,.T.);
#11425=EDGE_CURVE('',#9041,#9042,#2541,.T.);
#11426=EDGE_CURVE('',#9042,#8999,#7594,.T.);
#11427=EDGE_CURVE('',#8995,#9043,#7595,.T.);
#11428=EDGE_CURVE('',#9043,#8994,#2542,.T.);
#11429=EDGE_CURVE('',#9044,#8993,#2543,.T.);
#11430=EDGE_CURVE('',#9043,#9044,#2544,.T.);
#11431=EDGE_CURVE('',#9044,#8991,#7596,.T.);
#11432=EDGE_CURVE('',#8991,#8234,#7597,.T.);
#11433=EDGE_CURVE('',#8235,#8992,#7598,.T.);
#11434=EDGE_CURVE('',#8992,#9045,#7599,.T.);
#11435=EDGE_CURVE('',#9045,#8998,#2545,.T.);
#11436=EDGE_CURVE('',#9046,#8997,#2546,.T.);
#11437=EDGE_CURVE('',#9045,#9046,#2547,.T.);
#11438=EDGE_CURVE('',#9046,#8996,#7600,.T.);
#11439=EDGE_CURVE('',#9000,#9047,#7601,.T.);
#11440=EDGE_CURVE('',#9047,#9006,#2548,.T.);
#11441=EDGE_CURVE('',#9048,#9005,#2549,.T.);
#11442=EDGE_CURVE('',#9047,#9048,#2550,.T.);
#11443=EDGE_CURVE('',#9048,#9004,#7602,.T.);
#11444=EDGE_CURVE('',#9011,#9049,#2551,.T.);
#11445=EDGE_CURVE('',#9050,#9049,#2552,.T.);
#11446=EDGE_CURVE('',#9050,#9012,#2553,.T.);
#11447=EDGE_CURVE('',#9010,#9051,#2554,.T.);
#11448=EDGE_CURVE('',#9049,#9051,#2555,.T.);
#11449=EDGE_CURVE('',#9009,#9052,#2556,.T.);
#11450=EDGE_CURVE('',#9051,#9052,#2557,.T.);
#11451=EDGE_CURVE('',#9008,#9053,#2558,.T.);
#11452=EDGE_CURVE('',#9052,#9053,#2559,.T.);
#11453=EDGE_CURVE('',#9007,#9054,#2560,.T.);
#11454=EDGE_CURVE('',#9053,#9054,#2561,.T.);
#11455=EDGE_CURVE('',#9054,#9050,#2562,.T.);
#11456=EDGE_CURVE('',#8229,#9055,#1399,.T.);
#11457=EDGE_CURVE('',#9020,#9056,#2563,.T.);
#11458=EDGE_CURVE('',#9055,#9056,#2564,.T.);
#11459=EDGE_CURVE('',#9056,#9057,#7603,.T.);
#11460=EDGE_CURVE('',#9055,#9057,#1330,.T.);
#11461=EDGE_CURVE('',#9058,#9019,#2565,.T.);
#11462=EDGE_CURVE('',#9059,#9058,#7604,.T.);
#11463=EDGE_CURVE('',#9057,#9059,#2566,.T.);
#11464=EDGE_CURVE('',#9060,#9058,#2567,.T.);
#11465=EDGE_CURVE('',#9059,#9060,#1331,.T.);
#11466=EDGE_CURVE('',#9061,#8264,#1400,.T.);
#11467=EDGE_CURVE('',#9060,#9061,#1401,.T.);
#11468=EDGE_CURVE('',#9062,#9063,#2568,.T.);
#11469=EDGE_CURVE('',#9063,#9064,#2569,.T.);
#11470=EDGE_CURVE('',#9064,#9065,#2570,.T.);
#11471=EDGE_CURVE('',#9065,#9066,#2571,.T.);
#11472=EDGE_CURVE('',#9066,#9067,#2572,.T.);
#11473=EDGE_CURVE('',#9067,#9062,#2573,.T.);
#11474=EDGE_CURVE('',#9068,#9069,#2574,.T.);
#11475=EDGE_CURVE('',#9069,#9070,#2575,.T.);
#11476=EDGE_CURVE('',#9070,#9071,#2576,.T.);
#11477=EDGE_CURVE('',#9071,#9072,#2577,.T.);
#11478=EDGE_CURVE('',#9072,#9073,#2578,.T.);
#11479=EDGE_CURVE('',#9073,#9068,#2579,.T.);
#11480=EDGE_CURVE('',#9074,#9075,#2580,.T.);
#11481=EDGE_CURVE('',#9075,#9076,#2581,.T.);
#11482=EDGE_CURVE('',#9076,#9077,#2582,.T.);
#11483=EDGE_CURVE('',#9077,#9078,#2583,.T.);
#11484=EDGE_CURVE('',#9078,#9079,#2584,.T.);
#11485=EDGE_CURVE('',#9079,#9074,#2585,.T.);
#11486=EDGE_CURVE('',#8244,#9080,#2586,.T.);
#11487=EDGE_CURVE('',#9080,#8277,#2587,.T.);
#11488=EDGE_CURVE('',#9080,#9081,#2588,.T.);
#11489=EDGE_CURVE('',#9081,#8278,#2589,.T.);
#11490=EDGE_CURVE('',#9081,#8243,#2590,.T.);
#11491=EDGE_CURVE('',#9082,#9083,#2591,.T.);
#11492=EDGE_CURVE('',#9083,#9084,#2592,.T.);
#11493=EDGE_CURVE('',#9084,#9085,#2593,.T.);
#11494=EDGE_CURVE('',#9085,#9086,#2594,.T.);
#11495=EDGE_CURVE('',#9086,#9087,#2595,.T.);
#11496=EDGE_CURVE('',#9087,#9082,#2596,.T.);
#11497=EDGE_CURVE('',#9088,#9089,#2597,.T.);
#11498=EDGE_CURVE('',#9089,#9090,#2598,.T.);
#11499=EDGE_CURVE('',#9090,#9091,#2599,.T.);
#11500=EDGE_CURVE('',#9091,#9092,#2600,.T.);
#11501=EDGE_CURVE('',#9092,#9093,#2601,.T.);
#11502=EDGE_CURVE('',#9093,#9088,#2602,.T.);
#11503=EDGE_CURVE('',#9094,#9023,#2603,.T.);
#11504=EDGE_CURVE('',#9028,#9095,#2604,.T.);
#11505=EDGE_CURVE('',#9094,#9095,#2605,.T.);
#11506=EDGE_CURVE('',#9027,#9096,#2606,.T.);
#11507=EDGE_CURVE('',#9095,#9096,#2607,.T.);
#11508=EDGE_CURVE('',#9026,#9097,#2608,.T.);
#11509=EDGE_CURVE('',#9096,#9097,#2609,.T.);
#11510=EDGE_CURVE('',#9025,#9098,#2610,.T.);
#11511=EDGE_CURVE('',#9097,#9098,#2611,.T.);
#11512=EDGE_CURVE('',#9024,#9099,#2612,.T.);
#11513=EDGE_CURVE('',#9098,#9099,#2613,.T.);
#11514=EDGE_CURVE('',#9099,#9094,#2614,.T.);
#11515=EDGE_CURVE('',#9100,#9101,#2615,.T.);
#11516=EDGE_CURVE('',#9102,#9101,#7605,.T.);
#11517=EDGE_CURVE('',#9102,#9100,#2616,.T.);
#11518=EDGE_CURVE('',#9103,#9104,#2617,.T.);
#11519=EDGE_CURVE('',#9103,#9101,#7606,.T.);
#11520=EDGE_CURVE('',#9100,#9104,#7607,.T.);
#11521=EDGE_CURVE('',#9104,#9105,#2618,.T.);
#11522=EDGE_CURVE('',#9105,#9106,#2619,.T.);
#11523=EDGE_CURVE('',#9107,#9106,#7608,.T.);
#11524=EDGE_CURVE('',#9107,#9103,#2620,.T.);
#11525=EDGE_CURVE('',#9033,#9108,#2621,.T.);
#11526=EDGE_CURVE('',#9108,#9109,#2622,.T.);
#11527=EDGE_CURVE('',#9109,#9034,#2623,.T.);
#11528=EDGE_CURVE('',#9109,#9110,#2624,.T.);
#11529=EDGE_CURVE('',#9110,#9029,#2625,.T.);
#11530=EDGE_CURVE('',#9110,#9111,#2626,.T.);
#11531=EDGE_CURVE('',#9111,#9030,#2627,.T.);
#11532=EDGE_CURVE('',#9111,#9112,#2628,.T.);
#11533=EDGE_CURVE('',#9112,#9031,#2629,.T.);
#11534=EDGE_CURVE('',#9112,#9113,#2630,.T.);
#11535=EDGE_CURVE('',#9113,#9032,#2631,.T.);
#11536=EDGE_CURVE('',#9113,#9108,#2632,.T.);
#11537=EDGE_CURVE('',#9114,#9115,#2633,.T.);
#11538=EDGE_CURVE('',#9114,#9116,#7609,.T.);
#11539=EDGE_CURVE('',#9117,#9116,#2634,.T.);
#11540=EDGE_CURVE('',#9115,#9117,#7610,.T.);
#11541=EDGE_CURVE('',#9116,#9118,#2635,.T.);
#11542=EDGE_CURVE('',#9119,#9118,#7611,.T.);
#11543=EDGE_CURVE('',#9119,#9120,#2636,.T.);
#11544=EDGE_CURVE('',#9117,#9120,#2637,.T.);
#11545=EDGE_CURVE('',#9039,#9121,#2638,.T.);
#11546=EDGE_CURVE('',#9122,#9121,#2639,.T.);
#11547=EDGE_CURVE('',#9122,#9040,#2640,.T.);
#11548=EDGE_CURVE('',#9038,#9123,#2641,.T.);
#11549=EDGE_CURVE('',#9121,#9123,#2642,.T.);
#11550=EDGE_CURVE('',#9037,#9124,#2643,.T.);
#11551=EDGE_CURVE('',#9123,#9124,#2644,.T.);
#11552=EDGE_CURVE('',#9036,#9125,#2645,.T.);
#11553=EDGE_CURVE('',#9124,#9125,#2646,.T.);
#11554=EDGE_CURVE('',#9035,#9126,#2647,.T.);
#11555=EDGE_CURVE('',#9125,#9126,#2648,.T.);
#11556=EDGE_CURVE('',#9126,#9122,#2649,.T.);
#11557=EDGE_CURVE('',#9127,#9128,#2650,.T.);
#11558=EDGE_CURVE('',#8238,#9128,#1332,.T.);
#11559=EDGE_CURVE('',#9127,#8236,#1333,.T.);
#11560=EDGE_CURVE('',#9129,#8232,#1334,.T.);
#11561=EDGE_CURVE('',#8237,#9129,#1335,.T.);
#11562=EDGE_CURVE('',#9130,#8239,#1336,.T.);
#11563=EDGE_CURVE('',#8257,#9130,#1337,.T.);
#11564=EDGE_CURVE('',#9131,#8258,#1338,.T.);
#11565=EDGE_CURVE('',#9061,#9131,#1339,.T.);
#11566=EDGE_CURVE('',#9132,#8263,#1402,.T.);
#11567=EDGE_CURVE('',#9133,#9132,#1340,.T.);
#11568=EDGE_CURVE('',#8233,#9133,#1341,.T.);
#11569=EDGE_CURVE('',#9134,#9135,#2651,.T.);
#11570=EDGE_CURVE('',#9132,#9134,#1403,.T.);
#11571=EDGE_CURVE('',#9135,#8259,#2652,.T.);
#11572=EDGE_CURVE('',#9136,#9135,#7612,.T.);
#11573=EDGE_CURVE('',#9134,#9136,#1342,.T.);
#11574=EDGE_CURVE('',#9137,#9138,#7613,.T.);
#11575=EDGE_CURVE('',#9136,#9137,#2653,.T.);
#11576=EDGE_CURVE('',#9138,#8260,#2654,.T.);
#11577=EDGE_CURVE('',#9139,#9138,#2655,.T.);
#11578=EDGE_CURVE('',#9137,#9139,#1343,.T.);
#11579=EDGE_CURVE('',#9139,#8225,#1404,.T.);
#11580=EDGE_CURVE('',#9140,#8220,#1344,.T.);
#11581=EDGE_CURVE('',#8231,#9140,#1345,.T.);
#11582=EDGE_CURVE('',#9141,#8230,#1346,.T.);
#11583=EDGE_CURVE('',#8222,#9141,#1347,.T.);
#11584=EDGE_CURVE('',#9142,#8216,#1348,.T.);
#11585=EDGE_CURVE('',#8221,#9142,#1349,.T.);
#11586=EDGE_CURVE('',#9143,#8223,#1350,.T.);
#11587=EDGE_CURVE('',#8218,#9143,#1351,.T.);
#11588=EDGE_CURVE('',#9144,#8219,#1352,.T.);
#11589=EDGE_CURVE('',#9144,#9145,#2656,.T.);
#11590=EDGE_CURVE('',#8217,#9145,#1353,.T.);
#11591=EDGE_CURVE('',#9118,#9107,#2657,.T.);
#11592=EDGE_CURVE('',#9145,#9114,#2658,.T.);
#11593=EDGE_CURVE('',#9101,#9144,#2659,.T.);
#11594=EDGE_CURVE('',#9146,#9115,#2660,.T.);
#11595=EDGE_CURVE('',#9114,#9146,#7614,.T.);
#11596=EDGE_CURVE('',#9147,#9148,#1354,.T.);
#11597=EDGE_CURVE('',#9149,#9147,#1355,.T.);
#11598=EDGE_CURVE('',#9149,#9148,#1356,.T.);
#11599=EDGE_CURVE('',#9150,#9151,#2661,.T.);
#11600=EDGE_CURVE('',#9152,#9150,#2662,.T.);
#11601=EDGE_CURVE('',#9153,#9152,#2663,.T.);
#11602=EDGE_CURVE('',#9153,#9154,#7615,.T.);
#11603=EDGE_CURVE('',#9128,#9154,#2664,.T.);
#11604=EDGE_CURVE('',#9155,#9127,#2665,.T.);
#11605=EDGE_CURVE('',#9155,#9151,#7616,.T.);
#11606=EDGE_CURVE('',#9156,#9157,#2666,.T.);
#11607=EDGE_CURVE('',#9154,#9156,#7617,.T.);
#11608=EDGE_CURVE('',#9154,#9157,#2667,.T.);
#11609=EDGE_CURVE('',#9158,#9153,#2668,.T.);
#11610=EDGE_CURVE('',#9157,#9158,#7618,.T.);
#11611=EDGE_CURVE('',#9159,#9152,#7619,.T.);
#11612=EDGE_CURVE('',#9159,#9160,#2669,.T.);
#11613=EDGE_CURVE('',#9158,#9160,#2670,.T.);
#11614=EDGE_CURVE('',#9161,#9156,#2671,.T.);
#11615=EDGE_CURVE('',#9162,#9161,#1405,.T.);
#11616=EDGE_CURVE('',#9147,#9162,#2672,.T.);
#11617=EDGE_CURVE('',#9148,#9102,#2673,.T.);
#11618=EDGE_CURVE('',#9066,#9163,#2674,.T.);
#11619=EDGE_CURVE('',#9164,#9163,#2675,.T.);
#11620=EDGE_CURVE('',#9164,#9067,#2676,.T.);
#11621=EDGE_CURVE('',#9065,#9165,#2677,.T.);
#11622=EDGE_CURVE('',#9163,#9165,#2678,.T.);
#11623=EDGE_CURVE('',#9064,#9166,#2679,.T.);
#11624=EDGE_CURVE('',#9165,#9166,#2680,.T.);
#11625=EDGE_CURVE('',#9063,#9167,#2681,.T.);
#11626=EDGE_CURVE('',#9166,#9167,#2682,.T.);
#11627=EDGE_CURVE('',#9062,#9168,#2683,.T.);
#11628=EDGE_CURVE('',#9167,#9168,#2684,.T.);
#11629=EDGE_CURVE('',#9168,#9164,#2685,.T.);
#11630=EDGE_CURVE('',#9169,#9161,#1357,.T.);
#11631=EDGE_CURVE('',#9162,#9169,#1358,.T.);
#11632=EDGE_CURVE('',#9170,#9155,#2686,.T.);
#11633=EDGE_CURVE('',#9171,#9155,#7620,.T.);
#11634=EDGE_CURVE('',#9171,#9170,#2687,.T.);
#11635=EDGE_CURVE('',#9151,#9172,#2688,.T.);
#11636=EDGE_CURVE('',#9170,#9172,#7621,.T.);
#11637=EDGE_CURVE('',#9172,#9173,#2689,.T.);
#11638=EDGE_CURVE('',#9173,#9174,#2690,.T.);
#11639=EDGE_CURVE('',#9150,#9174,#7622,.T.);
#11640=EDGE_CURVE('',#9072,#9175,#2691,.T.);
#11641=EDGE_CURVE('',#9175,#9176,#2692,.T.);
#11642=EDGE_CURVE('',#9176,#9073,#2693,.T.);
#11643=EDGE_CURVE('',#9176,#9177,#2694,.T.);
#11644=EDGE_CURVE('',#9177,#9068,#2695,.T.);
#11645=EDGE_CURVE('',#9177,#9178,#2696,.T.);
#11646=EDGE_CURVE('',#9178,#9069,#2697,.T.);
#11647=EDGE_CURVE('',#9178,#9179,#2698,.T.);
#11648=EDGE_CURVE('',#9179,#9070,#2699,.T.);
#11649=EDGE_CURVE('',#9179,#9180,#2700,.T.);
#11650=EDGE_CURVE('',#9180,#9071,#2701,.T.);
#11651=EDGE_CURVE('',#9180,#9175,#2702,.T.);
#11652=EDGE_CURVE('',#9181,#9077,#2703,.T.);
#11653=EDGE_CURVE('',#9076,#9182,#2704,.T.);
#11654=EDGE_CURVE('',#9181,#9182,#2705,.T.);
#11655=EDGE_CURVE('',#9075,#9183,#2706,.T.);
#11656=EDGE_CURVE('',#9182,#9183,#2707,.T.);
#11657=EDGE_CURVE('',#9074,#9184,#2708,.T.);
#11658=EDGE_CURVE('',#9183,#9184,#2709,.T.);
#11659=EDGE_CURVE('',#9079,#9185,#2710,.T.);
#11660=EDGE_CURVE('',#9184,#9185,#2711,.T.);
#11661=EDGE_CURVE('',#9078,#9186,#2712,.T.);
#11662=EDGE_CURVE('',#9185,#9186,#2713,.T.);
#11663=EDGE_CURVE('',#9186,#9181,#2714,.T.);
#11664=EDGE_CURVE('',#9187,#9188,#2715,.T.);
#11665=EDGE_CURVE('',#9188,#9189,#2716,.T.);
#11666=EDGE_CURVE('',#9189,#9190,#2717,.T.);
#11667=EDGE_CURVE('',#9190,#9191,#2718,.T.);
#11668=EDGE_CURVE('',#9191,#9192,#2719,.T.);
#11669=EDGE_CURVE('',#9192,#9187,#2720,.T.);
#11670=EDGE_CURVE('',#9193,#9194,#2721,.T.);
#11671=EDGE_CURVE('',#9195,#9193,#2722,.T.);
#11672=EDGE_CURVE('',#9196,#9195,#2723,.T.);
#11673=EDGE_CURVE('',#9197,#9196,#2724,.T.);
#11674=EDGE_CURVE('',#9198,#9197,#2725,.T.);
#11675=EDGE_CURVE('',#9194,#9198,#2726,.T.);
#11676=EDGE_CURVE('',#9199,#9200,#2727,.T.);
#11677=EDGE_CURVE('',#9193,#9200,#2728,.T.);
#11678=EDGE_CURVE('',#9199,#9194,#2729,.T.);
#11679=EDGE_CURVE('',#9200,#9201,#2730,.T.);
#11680=EDGE_CURVE('',#9202,#9199,#2731,.T.);
#11681=EDGE_CURVE('',#9203,#9202,#2732,.T.);
#11682=EDGE_CURVE('',#9204,#9203,#2733,.T.);
#11683=EDGE_CURVE('',#9201,#9204,#2734,.T.);
#11684=EDGE_CURVE('',#9205,#9206,#2735,.T.);
#11685=EDGE_CURVE('',#9204,#9206,#2736,.T.);
#11686=EDGE_CURVE('',#9205,#9203,#2737,.T.);
#11687=EDGE_CURVE('',#9207,#9082,#2738,.T.);
#11688=EDGE_CURVE('',#9087,#9208,#2739,.T.);
#11689=EDGE_CURVE('',#9207,#9208,#2740,.T.);
#11690=EDGE_CURVE('',#9086,#9209,#2741,.T.);
#11691=EDGE_CURVE('',#9208,#9209,#2742,.T.);
#11692=EDGE_CURVE('',#9085,#9210,#2743,.T.);
#11693=EDGE_CURVE('',#9209,#9210,#2744,.T.);
#11694=EDGE_CURVE('',#9084,#9211,#2745,.T.);
#11695=EDGE_CURVE('',#9210,#9211,#2746,.T.);
#11696=EDGE_CURVE('',#9083,#9212,#2747,.T.);
#11697=EDGE_CURVE('',#9211,#9212,#2748,.T.);
#11698=EDGE_CURVE('',#9212,#9207,#2749,.T.);
#11699=EDGE_CURVE('',#9213,#9214,#7623,.T.);
#11700=EDGE_CURVE('',#9215,#9213,#2750,.T.);
#11701=EDGE_CURVE('',#9215,#9088,#2751,.T.);
#11702=EDGE_CURVE('',#9093,#9216,#2752,.T.);
#11703=EDGE_CURVE('',#9214,#9216,#2753,.T.);
#11704=EDGE_CURVE('',#9092,#9217,#2754,.T.);
#11705=EDGE_CURVE('',#9216,#9217,#2755,.T.);
#11706=EDGE_CURVE('',#9091,#9218,#2756,.T.);
#11707=EDGE_CURVE('',#9217,#9218,#2757,.T.);
#11708=EDGE_CURVE('',#9090,#9219,#2758,.T.);
#11709=EDGE_CURVE('',#9220,#9219,#2759,.T.);
#11710=EDGE_CURVE('',#9221,#9220,#7624,.T.);
#11711=EDGE_CURVE('',#9218,#9221,#2760,.T.);
#11712=EDGE_CURVE('',#9089,#9222,#2761,.T.);
#11713=EDGE_CURVE('',#9219,#9222,#2762,.T.);
#11714=EDGE_CURVE('',#9222,#9215,#2763,.T.);
#11715=EDGE_CURVE('',#9106,#9119,#2764,.T.);
#11716=EDGE_CURVE('',#9223,#9149,#7625,.T.);
#11717=EDGE_CURVE('',#9223,#9105,#2765,.T.);
#11718=EDGE_CURVE('',#9224,#9225,#1359,.T.);
#11719=EDGE_CURVE('',#9226,#9224,#1360,.T.);
#11720=EDGE_CURVE('',#9225,#9226,#1406,.T.);
#11721=EDGE_CURVE('',#9146,#9225,#2766,.T.);
#11722=EDGE_CURVE('',#9120,#9227,#2767,.T.);
#11723=EDGE_CURVE('',#9224,#9227,#7626,.T.);
#11724=EDGE_CURVE('',#9226,#9228,#2768,.T.);
#11725=EDGE_CURVE('',#9229,#9228,#1407,.T.);
#11726=EDGE_CURVE('',#9229,#9171,#2769,.T.);
#11727=EDGE_CURVE('',#9230,#9228,#1361,.T.);
#11728=EDGE_CURVE('',#9230,#9229,#1362,.T.);
#11729=EDGE_CURVE('',#9206,#9231,#2770,.T.);
#11730=EDGE_CURVE('',#9232,#9205,#2771,.T.);
#11731=EDGE_CURVE('',#9231,#9232,#2772,.T.);
#11732=EDGE_CURVE('',#9233,#9234,#7627,.T.);
#11733=EDGE_CURVE('',#9233,#9223,#2773,.T.);
#11734=EDGE_CURVE('',#9234,#9147,#2774,.T.);
#11735=EDGE_CURVE('',#9234,#9235,#2775,.T.);
#11736=EDGE_CURVE('',#9235,#9162,#2776,.T.);
#11737=EDGE_CURVE('',#9174,#9159,#2777,.T.);
#11738=EDGE_CURVE('',#9160,#9236,#2778,.T.);
#11739=EDGE_CURVE('',#9169,#9236,#7628,.T.);
#11740=EDGE_CURVE('',#9235,#9237,#7629,.T.);
#11741=EDGE_CURVE('',#9236,#9237,#2779,.T.);
#11742=EDGE_CURVE('',#9238,#9230,#7630,.T.);
#11743=EDGE_CURVE('',#9238,#9173,#2780,.T.);
#11744=EDGE_CURVE('',#9239,#9187,#2781,.T.);
#11745=EDGE_CURVE('',#9192,#9240,#2782,.T.);
#11746=EDGE_CURVE('',#9239,#9240,#2783,.T.);
#11747=EDGE_CURVE('',#9191,#9241,#2784,.T.);
#11748=EDGE_CURVE('',#9240,#9241,#2785,.T.);
#11749=EDGE_CURVE('',#9190,#9242,#2786,.T.);
#11750=EDGE_CURVE('',#9241,#9242,#2787,.T.);
#11751=EDGE_CURVE('',#9189,#9243,#2788,.T.);
#11752=EDGE_CURVE('',#9242,#9243,#2789,.T.);
#11753=EDGE_CURVE('',#9188,#9244,#2790,.T.);
#11754=EDGE_CURVE('',#9243,#9244,#2791,.T.);
#11755=EDGE_CURVE('',#9244,#9239,#2792,.T.);
#11756=EDGE_CURVE('',#9232,#9202,#2793,.T.);
#11757=EDGE_CURVE('',#9202,#9198,#2794,.T.);
#11758=EDGE_CURVE('',#9245,#9246,#2795,.T.);
#11759=EDGE_CURVE('',#9198,#9245,#2796,.T.);
#11760=EDGE_CURVE('',#9246,#9197,#2797,.T.);
#11761=EDGE_CURVE('',#9246,#9247,#2798,.T.);
#11762=EDGE_CURVE('',#9247,#9196,#2799,.T.);
#11763=EDGE_CURVE('',#9247,#9248,#2800,.T.);
#11764=EDGE_CURVE('',#9248,#9195,#2801,.T.);
#11765=EDGE_CURVE('',#9195,#9201,#2802,.T.);
#11766=EDGE_CURVE('',#9201,#9231,#2803,.T.);
#11767=EDGE_CURVE('',#9221,#9214,#2804,.T.);
#11768=EDGE_CURVE('',#9213,#8203,#2805,.T.);
#11769=EDGE_CURVE('',#8202,#9220,#2806,.T.);
#11770=EDGE_CURVE('',#9249,#9250,#2807,.T.);
#11771=EDGE_CURVE('',#9249,#9250,#7631,.T.);
#11772=EDGE_CURVE('',#9251,#9252,#2808,.T.);
#11773=EDGE_CURVE('',#9251,#9252,#7632,.T.);
#11774=EDGE_CURVE('',#8211,#8208,#2809,.T.);
#11775=EDGE_CURVE('',#9253,#9233,#2810,.T.);
#11776=EDGE_CURVE('',#9227,#9253,#2811,.T.);
#11777=EDGE_CURVE('',#9254,#9255,#7633,.T.);
#11778=EDGE_CURVE('',#9255,#9226,#2812,.T.);
#11779=EDGE_CURVE('',#9254,#9253,#7634,.T.);
#11780=EDGE_CURVE('',#9228,#9256,#2813,.T.);
#11781=EDGE_CURVE('',#9255,#9256,#2814,.T.);
#11782=EDGE_CURVE('',#9257,#9258,#7635,.T.);
#11783=EDGE_CURVE('',#9257,#9238,#2815,.T.);
#11784=EDGE_CURVE('',#9256,#9258,#7636,.T.);
#11785=EDGE_CURVE('',#9231,#9237,#2816,.T.);
#11786=EDGE_CURVE('',#9233,#9232,#2817,.T.);
#11787=EDGE_CURVE('',#9237,#9257,#2818,.T.);
#11788=EDGE_CURVE('',#9259,#9260,#2819,.T.);
#11789=EDGE_CURVE('',#9259,#9260,#7637,.T.);
#11790=EDGE_CURVE('',#9261,#9262,#2820,.T.);
#11791=EDGE_CURVE('',#9261,#9262,#7638,.T.);
#11792=EDGE_CURVE('',#8194,#9263,#7639,.T.);
#11793=EDGE_CURVE('',#8190,#9263,#7640,.T.);
#11794=EDGE_CURVE('',#9264,#8188,#7641,.T.);
#11795=EDGE_CURVE('',#9265,#8193,#7642,.T.);
#11796=EDGE_CURVE('',#9264,#9265,#1363,.T.);
#11797=EDGE_CURVE('',#9266,#9264,#7643,.T.);
#11798=EDGE_CURVE('',#9267,#9266,#7644,.T.);
#11799=EDGE_CURVE('',#9268,#9267,#7645,.T.);
#11800=EDGE_CURVE('',#9269,#9268,#7646,.T.);
#11801=EDGE_CURVE('',#9269,#8189,#7647,.T.);
#11802=EDGE_CURVE('',#9263,#9269,#1364,.T.);
#11803=EDGE_CURVE('',#9265,#8184,#7648,.T.);
#11804=EDGE_CURVE('',#9270,#9271,#2821,.T.);
#11805=EDGE_CURVE('',#9232,#9270,#2822,.T.);
#11806=EDGE_CURVE('',#9272,#9232,#2823,.T.);
#11807=EDGE_CURVE('',#9273,#9272,#2824,.T.);
#11808=EDGE_CURVE('',#9274,#9273,#2825,.T.);
#11809=EDGE_CURVE('',#9271,#9274,#2826,.T.);
#11810=EDGE_CURVE('',#9202,#9275,#2827,.T.);
#11811=EDGE_CURVE('',#9272,#9275,#2828,.T.);
#11812=EDGE_CURVE('',#9276,#9202,#2829,.T.);
#11813=EDGE_CURVE('',#9277,#9276,#2830,.T.);
#11814=EDGE_CURVE('',#9275,#9277,#2831,.T.);
#11815=EDGE_CURVE('',#9278,#9198,#2832,.T.);
#11816=EDGE_CURVE('',#9276,#9278,#2833,.T.);
#11817=EDGE_CURVE('',#9278,#9279,#2834,.T.);
#11818=EDGE_CURVE('',#9280,#9198,#2835,.T.);
#11819=EDGE_CURVE('',#9279,#9280,#2836,.T.);
#11820=EDGE_CURVE('',#9281,#9245,#2837,.T.);
#11821=EDGE_CURVE('',#9280,#9281,#2838,.T.);
#11822=EDGE_CURVE('',#9282,#9283,#2839,.T.);
#11823=EDGE_CURVE('',#9284,#9282,#2840,.T.);
#11824=EDGE_CURVE('',#9285,#9284,#2841,.T.);
#11825=EDGE_CURVE('',#9286,#9285,#2842,.T.);
#11826=EDGE_CURVE('',#9287,#9286,#2843,.T.);
#11827=EDGE_CURVE('',#9281,#9287,#2844,.T.);
#11828=EDGE_CURVE('',#9288,#9248,#2845,.T.);
#11829=EDGE_CURVE('',#9289,#9288,#2846,.T.);
#11830=EDGE_CURVE('',#9290,#9289,#2847,.T.);
#11831=EDGE_CURVE('',#9283,#9290,#2848,.T.);
#11832=EDGE_CURVE('',#9291,#9195,#2849,.T.);
#11833=EDGE_CURVE('',#9288,#9291,#2850,.T.);
#11834=EDGE_CURVE('',#9292,#9293,#2851,.T.);
#11835=EDGE_CURVE('',#9291,#9292,#2852,.T.);
#11836=EDGE_CURVE('',#9293,#9195,#2853,.T.);
#11837=EDGE_CURVE('',#9201,#9294,#2854,.T.);
#11838=EDGE_CURVE('',#9293,#9294,#2855,.T.);
#11839=EDGE_CURVE('',#9295,#9296,#2856,.T.);
#11840=EDGE_CURVE('',#9294,#9295,#2857,.T.);
#11841=EDGE_CURVE('',#9296,#9201,#2858,.T.);
#11842=EDGE_CURVE('',#9231,#9297,#2859,.T.);
#11843=EDGE_CURVE('',#9296,#9297,#2860,.T.);
#11844=EDGE_CURVE('',#9298,#9299,#2861,.T.);
#11845=EDGE_CURVE('',#9297,#9298,#2862,.T.);
#11846=EDGE_CURVE('',#9300,#9231,#2863,.T.);
#11847=EDGE_CURVE('',#9301,#9300,#2864,.T.);
#11848=EDGE_CURVE('',#9299,#9301,#2865,.T.);
#11849=EDGE_CURVE('',#9302,#9303,#2866,.T.);
#11850=EDGE_CURVE('',#9303,#8201,#2867,.T.);
#11851=EDGE_CURVE('',#8200,#9302,#2868,.T.);
#11852=EDGE_CURVE('',#9303,#9304,#7649,.T.);
#11853=EDGE_CURVE('',#9260,#9304,#2869,.T.);
#11854=EDGE_CURVE('',#8204,#9259,#2870,.T.);
#11855=EDGE_CURVE('',#9305,#9306,#7650,.T.);
#11856=EDGE_CURVE('',#9250,#9306,#2871,.T.);
#11857=EDGE_CURVE('',#9305,#9249,#2872,.T.);
#11858=EDGE_CURVE('',#9307,#9308,#7651,.T.);
#11859=EDGE_CURVE('',#9252,#9308,#2873,.T.);
#11860=EDGE_CURVE('',#9307,#9251,#2874,.T.);
#11861=EDGE_CURVE('',#9308,#9309,#2875,.T.);
#11862=EDGE_CURVE('',#8206,#9309,#2876,.T.);
#11863=EDGE_CURVE('',#9270,#8207,#2877,.T.);
#11864=EDGE_CURVE('',#9310,#9271,#2878,.T.);
#11865=EDGE_CURVE('',#9310,#9305,#2879,.T.);
#11866=EDGE_CURVE('',#9306,#9307,#2880,.T.);
#11867=EDGE_CURVE('',#9309,#9311,#2881,.T.);
#11868=EDGE_CURVE('',#9253,#9311,#2882,.T.);
#11869=EDGE_CURVE('',#9311,#9254,#2883,.T.);
#11870=EDGE_CURVE('',#9254,#9258,#2884,.T.);
#11871=EDGE_CURVE('',#9258,#9312,#2885,.T.);
#11872=EDGE_CURVE('',#9257,#9312,#2886,.T.);
#11873=EDGE_CURVE('',#9312,#9313,#2887,.T.);
#11874=EDGE_CURVE('',#9300,#9313,#2888,.T.);
#11875=EDGE_CURVE('',#9262,#8205,#2889,.T.);
#11876=EDGE_CURVE('',#9304,#9314,#2890,.T.);
#11877=EDGE_CURVE('',#9301,#9314,#2891,.T.);
#11878=EDGE_CURVE('',#9313,#9315,#2892,.T.);
#11879=EDGE_CURVE('',#9315,#9261,#2893,.T.);
#11880=EDGE_CURVE('',#9315,#9302,#7652,.T.);
#11881=EDGE_CURVE('',#9266,#9316,#1365,.T.);
#11882=EDGE_CURVE('',#8187,#9316,#7653,.T.);
#11883=EDGE_CURVE('',#9316,#9317,#7654,.T.);
#11884=EDGE_CURVE('',#9267,#9317,#1366,.T.);
#11885=EDGE_CURVE('',#9268,#9318,#1367,.T.);
#11886=EDGE_CURVE('',#9317,#9318,#7655,.T.);
#11887=EDGE_CURVE('',#9318,#8195,#7656,.T.);
#11888=EDGE_CURVE('',#9319,#9320,#2894,.T.);
#11889=EDGE_CURVE('',#9321,#9320,#2895,.T.);
#11890=EDGE_CURVE('',#9321,#9310,#2896,.T.);
#11891=EDGE_CURVE('',#9319,#9274,#2897,.T.);
#11892=EDGE_CURVE('',#9320,#9322,#2898,.T.);
#11893=EDGE_CURVE('',#9323,#9322,#2899,.T.);
#11894=EDGE_CURVE('',#9323,#9321,#2900,.T.);
#11895=EDGE_CURVE('',#9324,#9319,#2901,.T.);
#11896=EDGE_CURVE('',#9324,#9273,#2902,.T.);
#11897=EDGE_CURVE('',#9273,#9277,#2903,.T.);
#11898=EDGE_CURVE('',#9277,#9279,#2904,.T.);
#11899=EDGE_CURVE('',#8181,#9287,#2905,.T.);
#11900=EDGE_CURVE('',#9279,#8180,#2906,.T.);
#11901=EDGE_CURVE('',#9325,#9326,#2907,.T.);
#11902=EDGE_CURVE('',#9287,#9325,#2908,.T.);
#11903=EDGE_CURVE('',#9326,#9286,#2909,.T.);
#11904=EDGE_CURVE('',#9326,#9327,#2910,.T.);
#11905=EDGE_CURVE('',#9327,#9285,#2911,.T.);
#11906=EDGE_CURVE('',#9327,#9328,#2912,.T.);
#11907=EDGE_CURVE('',#9328,#9284,#2913,.T.);
#11908=EDGE_CURVE('',#9329,#9282,#2914,.T.);
#11909=EDGE_CURVE('',#9330,#9329,#2915,.T.);
#11910=EDGE_CURVE('',#9284,#9330,#2916,.T.);
#11911=EDGE_CURVE('',#9331,#9332,#2917,.T.);
#11912=EDGE_CURVE('',#9282,#9331,#2918,.T.);
#11913=EDGE_CURVE('',#9332,#9283,#2919,.T.);
#11914=EDGE_CURVE('',#9332,#9333,#2920,.T.);
#11915=EDGE_CURVE('',#9333,#9290,#2921,.T.);
#11916=EDGE_CURVE('',#9333,#9334,#2922,.T.);
#11917=EDGE_CURVE('',#9334,#9289,#2923,.T.);
#11918=EDGE_CURVE('',#9289,#9292,#2924,.T.);
#11919=EDGE_CURVE('',#9292,#9295,#2925,.T.);
#11920=EDGE_CURVE('',#9295,#9298,#2926,.T.);
#11921=EDGE_CURVE('',#9335,#9336,#2927,.T.);
#11922=EDGE_CURVE('',#9299,#9336,#2928,.T.);
#11923=EDGE_CURVE('',#9314,#9337,#2929,.T.);
#11924=EDGE_CURVE('',#9335,#9337,#2930,.T.);
#11925=EDGE_CURVE('',#9336,#9338,#2931,.T.);
#11926=EDGE_CURVE('',#9298,#9338,#2932,.T.);
#11927=EDGE_CURVE('',#9339,#9335,#2933,.T.);
#11928=EDGE_CURVE('',#9337,#9340,#2934,.T.);
#11929=EDGE_CURVE('',#9339,#9340,#2935,.T.);
#11930=EDGE_CURVE('',#9341,#9323,#2936,.T.);
#11931=EDGE_CURVE('',#9342,#9341,#2937,.T.);
#11932=EDGE_CURVE('',#9340,#9342,#2938,.T.);
#11933=EDGE_CURVE('',#9322,#9343,#2939,.T.);
#11934=EDGE_CURVE('',#9341,#9343,#2940,.T.);
#11935=EDGE_CURVE('',#9344,#9324,#2941,.T.);
#11936=EDGE_CURVE('',#9343,#9344,#2942,.T.);
#11937=EDGE_CURVE('',#9345,#9325,#2943,.T.);
#11938=EDGE_CURVE('',#9344,#9345,#2944,.T.);
#11939=EDGE_CURVE('',#9346,#9328,#2945,.T.);
#11940=EDGE_CURVE('',#9345,#9346,#2946,.T.);
#11941=EDGE_CURVE('',#9347,#9330,#2947,.T.);
#11942=EDGE_CURVE('',#9346,#9347,#2948,.T.);
#11943=EDGE_CURVE('',#9348,#9329,#2949,.T.);
#11944=EDGE_CURVE('',#9347,#9348,#2950,.T.);
#11945=EDGE_CURVE('',#9349,#9331,#2951,.T.);
#11946=EDGE_CURVE('',#9348,#9349,#2952,.T.);
#11947=EDGE_CURVE('',#9350,#9334,#2953,.T.);
#11948=EDGE_CURVE('',#9349,#9350,#2954,.T.);
#11949=EDGE_CURVE('',#9338,#9351,#2955,.T.);
#11950=EDGE_CURVE('',#9350,#9351,#2956,.T.);
#11951=EDGE_CURVE('',#9352,#9339,#2957,.T.);
#11952=EDGE_CURVE('',#9351,#9352,#2958,.T.);
#11953=EDGE_CURVE('',#9352,#9342,#2959,.T.);
#13370=ORIENTED_EDGE('',*,*,#10065,.T.);
#13371=ORIENTED_EDGE('',*,*,#10066,.T.);
#13372=ORIENTED_EDGE('',*,*,#10067,.F.);
#13373=ORIENTED_EDGE('',*,*,#10068,.F.);
#13374=ORIENTED_EDGE('',*,*,#10066,.F.);
#13375=ORIENTED_EDGE('',*,*,#10069,.F.);
#13376=ORIENTED_EDGE('',*,*,#10070,.T.);
#13377=ORIENTED_EDGE('',*,*,#10071,.T.);
#13378=ORIENTED_EDGE('',*,*,#10072,.T.);
#13379=ORIENTED_EDGE('',*,*,#10070,.F.);
#13380=ORIENTED_EDGE('',*,*,#10073,.F.);
#13381=ORIENTED_EDGE('',*,*,#10074,.F.);
#13382=ORIENTED_EDGE('',*,*,#10075,.T.);
#13383=ORIENTED_EDGE('',*,*,#10076,.T.);
#13384=ORIENTED_EDGE('',*,*,#10077,.T.);
#13385=ORIENTED_EDGE('',*,*,#10075,.F.);
#13386=ORIENTED_EDGE('',*,*,#10078,.F.);
#13387=ORIENTED_EDGE('',*,*,#10079,.F.);
#13388=ORIENTED_EDGE('',*,*,#10080,.T.);
#13389=ORIENTED_EDGE('',*,*,#10081,.F.);
#13390=ORIENTED_EDGE('',*,*,#10082,.F.);
#13391=ORIENTED_EDGE('',*,*,#10080,.F.);
#13392=ORIENTED_EDGE('',*,*,#10083,.F.);
#13393=ORIENTED_EDGE('',*,*,#10084,.F.);
#13394=ORIENTED_EDGE('',*,*,#10085,.T.);
#13395=ORIENTED_EDGE('',*,*,#10086,.T.);
#13396=ORIENTED_EDGE('',*,*,#10085,.F.);
#13397=ORIENTED_EDGE('',*,*,#10069,.T.);
#13398=ORIENTED_EDGE('',*,*,#10087,.T.);
#13399=ORIENTED_EDGE('',*,*,#10067,.T.);
#13400=ORIENTED_EDGE('',*,*,#10068,.T.);
#13401=ORIENTED_EDGE('',*,*,#10087,.F.);
#13402=ORIENTED_EDGE('',*,*,#10073,.T.);
#13403=ORIENTED_EDGE('',*,*,#10077,.F.);
#13404=ORIENTED_EDGE('',*,*,#10088,.T.);
#13405=ORIENTED_EDGE('',*,*,#10089,.T.);
#13406=ORIENTED_EDGE('',*,*,#10088,.F.);
#13407=ORIENTED_EDGE('',*,*,#10076,.F.);
#13408=ORIENTED_EDGE('',*,*,#10079,.T.);
#13409=ORIENTED_EDGE('',*,*,#10090,.T.);
#13410=ORIENTED_EDGE('',*,*,#10071,.F.);
#13411=ORIENTED_EDGE('',*,*,#10072,.F.);
#13412=ORIENTED_EDGE('',*,*,#10090,.F.);
#13413=ORIENTED_EDGE('',*,*,#10083,.T.);
#13414=ORIENTED_EDGE('',*,*,#10074,.T.);
#13415=ORIENTED_EDGE('',*,*,#10091,.T.);
#13416=ORIENTED_EDGE('',*,*,#10081,.T.);
#13417=ORIENTED_EDGE('',*,*,#10082,.T.);
#13418=ORIENTED_EDGE('',*,*,#10091,.F.);
#13419=ORIENTED_EDGE('',*,*,#10078,.T.);
#13420=ORIENTED_EDGE('',*,*,#10086,.F.);
#13421=ORIENTED_EDGE('',*,*,#10065,.F.);
#13422=ORIENTED_EDGE('',*,*,#10084,.T.);
#13423=ORIENTED_EDGE('',*,*,#10089,.F.);
#13424=ORIENTED_EDGE('',*,*,#10092,.T.);
#13425=ORIENTED_EDGE('',*,*,#10093,.T.);
#13426=ORIENTED_EDGE('',*,*,#10094,.T.);
#13427=ORIENTED_EDGE('',*,*,#10095,.T.);
#13428=ORIENTED_EDGE('',*,*,#10094,.F.);
#13429=ORIENTED_EDGE('',*,*,#10092,.F.);
#13430=ORIENTED_EDGE('',*,*,#10093,.F.);
#13431=ORIENTED_EDGE('',*,*,#10096,.T.);
#13432=ORIENTED_EDGE('',*,*,#10097,.T.);
#13433=ORIENTED_EDGE('',*,*,#10096,.F.);
#13434=ORIENTED_EDGE('',*,*,#10097,.F.);
#13435=ORIENTED_EDGE('',*,*,#10095,.F.);
#13436=ORIENTED_EDGE('',*,*,#10098,.T.);
#13437=ORIENTED_EDGE('',*,*,#10099,.F.);
#13438=ORIENTED_EDGE('',*,*,#10098,.F.);
#13439=ORIENTED_EDGE('',*,*,#10099,.T.);
#13440=ORIENTED_EDGE('',*,*,#10100,.T.);
#13441=ORIENTED_EDGE('',*,*,#10101,.T.);
#13442=ORIENTED_EDGE('',*,*,#10102,.T.);
#13443=ORIENTED_EDGE('',*,*,#10103,.T.);
#13444=ORIENTED_EDGE('',*,*,#10104,.T.);
#13445=ORIENTED_EDGE('',*,*,#10105,.T.);
#13446=ORIENTED_EDGE('',*,*,#10106,.F.);
#13447=ORIENTED_EDGE('',*,*,#10101,.F.);
#13448=ORIENTED_EDGE('',*,*,#10107,.F.);
#13449=ORIENTED_EDGE('',*,*,#10108,.F.);
#13450=ORIENTED_EDGE('',*,*,#10107,.T.);
#13451=ORIENTED_EDGE('',*,*,#10100,.F.);
#13452=ORIENTED_EDGE('',*,*,#10109,.F.);
#13453=ORIENTED_EDGE('',*,*,#10110,.F.);
#13454=ORIENTED_EDGE('',*,*,#10109,.T.);
#13455=ORIENTED_EDGE('',*,*,#10105,.F.);
#13456=ORIENTED_EDGE('',*,*,#10111,.F.);
#13457=ORIENTED_EDGE('',*,*,#10112,.F.);
#13458=ORIENTED_EDGE('',*,*,#10113,.F.);
#13459=ORIENTED_EDGE('',*,*,#10111,.T.);
#13460=ORIENTED_EDGE('',*,*,#10104,.F.);
#13461=ORIENTED_EDGE('',*,*,#10114,.F.);
#13462=ORIENTED_EDGE('',*,*,#10115,.F.);
#13463=ORIENTED_EDGE('',*,*,#10114,.T.);
#13464=ORIENTED_EDGE('',*,*,#10103,.F.);
#13465=ORIENTED_EDGE('',*,*,#10116,.F.);
#13466=ORIENTED_EDGE('',*,*,#10117,.F.);
#13467=ORIENTED_EDGE('',*,*,#10118,.F.);
#13468=ORIENTED_EDGE('',*,*,#10116,.T.);
#13469=ORIENTED_EDGE('',*,*,#10102,.F.);
#13470=ORIENTED_EDGE('',*,*,#10106,.T.);
#13471=ORIENTED_EDGE('',*,*,#10119,.F.);
#13472=ORIENTED_EDGE('',*,*,#10113,.T.);
#13473=ORIENTED_EDGE('',*,*,#10120,.T.);
#13474=ORIENTED_EDGE('',*,*,#10119,.T.);
#13475=ORIENTED_EDGE('',*,*,#10108,.T.);
#13476=ORIENTED_EDGE('',*,*,#10110,.T.);
#13477=ORIENTED_EDGE('',*,*,#10115,.T.);
#13478=ORIENTED_EDGE('',*,*,#10117,.T.);
#13479=ORIENTED_EDGE('',*,*,#10118,.T.);
#13480=ORIENTED_EDGE('',*,*,#10120,.F.);
#13481=ORIENTED_EDGE('',*,*,#10112,.T.);
#13482=ORIENTED_EDGE('',*,*,#10121,.F.);
#13483=ORIENTED_EDGE('',*,*,#10122,.T.);
#13484=ORIENTED_EDGE('',*,*,#10123,.T.);
#13485=ORIENTED_EDGE('',*,*,#10124,.T.);
#13486=ORIENTED_EDGE('',*,*,#10125,.F.);
#13487=ORIENTED_EDGE('',*,*,#10126,.F.);
#13488=ORIENTED_EDGE('',*,*,#10127,.T.);
#13489=ORIENTED_EDGE('',*,*,#10128,.T.);
#13490=ORIENTED_EDGE('',*,*,#10129,.T.);
#13491=ORIENTED_EDGE('',*,*,#10130,.T.);
#13492=ORIENTED_EDGE('',*,*,#10122,.F.);
#13493=ORIENTED_EDGE('',*,*,#10131,.F.);
#13494=ORIENTED_EDGE('',*,*,#10132,.T.);
#13495=ORIENTED_EDGE('',*,*,#10133,.T.);
#13496=ORIENTED_EDGE('',*,*,#10134,.T.);
#13497=ORIENTED_EDGE('',*,*,#10132,.F.);
#13498=ORIENTED_EDGE('',*,*,#10135,.F.);
#13499=ORIENTED_EDGE('',*,*,#10136,.T.);
#13500=ORIENTED_EDGE('',*,*,#10137,.F.);
#13501=ORIENTED_EDGE('',*,*,#10136,.F.);
#13502=ORIENTED_EDGE('',*,*,#10138,.F.);
#13503=ORIENTED_EDGE('',*,*,#10139,.T.);
#13504=ORIENTED_EDGE('',*,*,#10140,.F.);
#13505=ORIENTED_EDGE('',*,*,#10139,.F.);
#13506=ORIENTED_EDGE('',*,*,#10141,.F.);
#13507=ORIENTED_EDGE('',*,*,#10142,.T.);
#13508=ORIENTED_EDGE('',*,*,#10143,.F.);
#13509=ORIENTED_EDGE('',*,*,#10142,.F.);
#13510=ORIENTED_EDGE('',*,*,#10144,.F.);
#13511=ORIENTED_EDGE('',*,*,#10145,.T.);
#13512=ORIENTED_EDGE('',*,*,#10146,.F.);
#13513=ORIENTED_EDGE('',*,*,#10145,.F.);
#13514=ORIENTED_EDGE('',*,*,#10147,.F.);
#13515=ORIENTED_EDGE('',*,*,#10148,.F.);
#13516=ORIENTED_EDGE('',*,*,#10149,.T.);
#13517=ORIENTED_EDGE('',*,*,#10150,.T.);
#13518=ORIENTED_EDGE('',*,*,#10149,.F.);
#13519=ORIENTED_EDGE('',*,*,#10151,.F.);
#13520=ORIENTED_EDGE('',*,*,#10152,.T.);
#13521=ORIENTED_EDGE('',*,*,#10153,.T.);
#13522=ORIENTED_EDGE('',*,*,#10154,.T.);
#13523=ORIENTED_EDGE('',*,*,#10155,.T.);
#13524=ORIENTED_EDGE('',*,*,#10156,.T.);
#13525=ORIENTED_EDGE('',*,*,#10157,.T.);
#13526=ORIENTED_EDGE('',*,*,#10158,.F.);
#13527=ORIENTED_EDGE('',*,*,#10159,.T.);
#13528=ORIENTED_EDGE('',*,*,#10160,.T.);
#13529=ORIENTED_EDGE('',*,*,#10153,.F.);
#13530=ORIENTED_EDGE('',*,*,#10161,.T.);
#13531=ORIENTED_EDGE('',*,*,#10162,.T.);
#13532=ORIENTED_EDGE('',*,*,#10163,.T.);
#13533=ORIENTED_EDGE('',*,*,#10164,.T.);
#13534=ORIENTED_EDGE('',*,*,#10165,.T.);
#13535=ORIENTED_EDGE('',*,*,#10159,.F.);
#13536=ORIENTED_EDGE('',*,*,#10166,.T.);
#13537=ORIENTED_EDGE('',*,*,#10167,.T.);
#13538=ORIENTED_EDGE('',*,*,#10168,.T.);
#13539=ORIENTED_EDGE('',*,*,#10167,.F.);
#13540=ORIENTED_EDGE('',*,*,#10169,.T.);
#13541=ORIENTED_EDGE('',*,*,#10170,.T.);
#13542=ORIENTED_EDGE('',*,*,#10171,.T.);
#13543=ORIENTED_EDGE('',*,*,#10172,.F.);
#13544=ORIENTED_EDGE('',*,*,#10173,.T.);
#13545=ORIENTED_EDGE('',*,*,#10174,.F.);
#13546=ORIENTED_EDGE('',*,*,#10175,.T.);
#13547=ORIENTED_EDGE('',*,*,#10176,.F.);
#13548=ORIENTED_EDGE('',*,*,#10177,.T.);
#13549=ORIENTED_EDGE('',*,*,#10170,.F.);
#13550=ORIENTED_EDGE('',*,*,#10178,.F.);
#13551=ORIENTED_EDGE('',*,*,#10179,.F.);
#13552=ORIENTED_EDGE('',*,*,#10180,.T.);
#13553=ORIENTED_EDGE('',*,*,#10181,.T.);
#13554=ORIENTED_EDGE('',*,*,#10182,.T.);
#13555=ORIENTED_EDGE('',*,*,#10181,.F.);
#13556=ORIENTED_EDGE('',*,*,#10183,.T.);
#13557=ORIENTED_EDGE('',*,*,#10184,.F.);
#13558=ORIENTED_EDGE('',*,*,#10185,.T.);
#13559=ORIENTED_EDGE('',*,*,#10186,.T.);
#13560=ORIENTED_EDGE('',*,*,#10187,.F.);
#13561=ORIENTED_EDGE('',*,*,#10186,.F.);
#13562=ORIENTED_EDGE('',*,*,#10188,.T.);
#13563=ORIENTED_EDGE('',*,*,#10189,.T.);
#13564=ORIENTED_EDGE('',*,*,#10190,.T.);
#13565=ORIENTED_EDGE('',*,*,#10189,.F.);
#13566=ORIENTED_EDGE('',*,*,#10191,.F.);
#13567=ORIENTED_EDGE('',*,*,#10192,.F.);
#13568=ORIENTED_EDGE('',*,*,#10193,.F.);
#13569=ORIENTED_EDGE('',*,*,#10194,.F.);
#13570=ORIENTED_EDGE('',*,*,#10195,.F.);
#13571=ORIENTED_EDGE('',*,*,#10196,.F.);
#13572=ORIENTED_EDGE('',*,*,#10197,.F.);
#13573=ORIENTED_EDGE('',*,*,#10198,.F.);
#13574=ORIENTED_EDGE('',*,*,#10199,.F.);
#13575=ORIENTED_EDGE('',*,*,#10200,.F.);
#13576=ORIENTED_EDGE('',*,*,#10201,.F.);
#13577=ORIENTED_EDGE('',*,*,#10202,.F.);
#13578=ORIENTED_EDGE('',*,*,#10203,.F.);
#13579=ORIENTED_EDGE('',*,*,#10204,.F.);
#13580=ORIENTED_EDGE('',*,*,#10205,.F.);
#13581=ORIENTED_EDGE('',*,*,#10206,.F.);
#13582=ORIENTED_EDGE('',*,*,#10207,.F.);
#13583=ORIENTED_EDGE('',*,*,#10208,.F.);
#13584=ORIENTED_EDGE('',*,*,#10209,.F.);
#13585=ORIENTED_EDGE('',*,*,#10210,.F.);
#13586=ORIENTED_EDGE('',*,*,#10211,.F.);
#13587=ORIENTED_EDGE('',*,*,#10212,.F.);
#13588=ORIENTED_EDGE('',*,*,#10213,.F.);
#13589=ORIENTED_EDGE('',*,*,#10214,.F.);
#13590=ORIENTED_EDGE('',*,*,#10215,.T.);
#13591=ORIENTED_EDGE('',*,*,#10216,.T.);
#13592=ORIENTED_EDGE('',*,*,#10217,.T.);
#13593=ORIENTED_EDGE('',*,*,#10218,.T.);
#13594=ORIENTED_EDGE('',*,*,#10219,.F.);
#13595=ORIENTED_EDGE('',*,*,#10220,.T.);
#13596=ORIENTED_EDGE('',*,*,#10221,.T.);
#13597=ORIENTED_EDGE('',*,*,#10222,.F.);
#13598=ORIENTED_EDGE('',*,*,#10221,.F.);
#13599=ORIENTED_EDGE('',*,*,#10223,.T.);
#13600=ORIENTED_EDGE('',*,*,#10224,.T.);
#13601=ORIENTED_EDGE('',*,*,#10225,.F.);
#13602=ORIENTED_EDGE('',*,*,#10224,.F.);
#13603=ORIENTED_EDGE('',*,*,#10226,.T.);
#13604=ORIENTED_EDGE('',*,*,#10227,.T.);
#13605=ORIENTED_EDGE('',*,*,#10228,.F.);
#13606=ORIENTED_EDGE('',*,*,#10227,.F.);
#13607=ORIENTED_EDGE('',*,*,#10229,.T.);
#13608=ORIENTED_EDGE('',*,*,#10230,.T.);
#13609=ORIENTED_EDGE('',*,*,#10231,.F.);
#13610=ORIENTED_EDGE('',*,*,#10230,.F.);
#13611=ORIENTED_EDGE('',*,*,#10232,.F.);
#13612=ORIENTED_EDGE('',*,*,#10233,.T.);
#13613=ORIENTED_EDGE('',*,*,#10234,.T.);
#13614=ORIENTED_EDGE('',*,*,#10233,.F.);
#13615=ORIENTED_EDGE('',*,*,#10235,.F.);
#13616=ORIENTED_EDGE('',*,*,#10236,.F.);
#13617=ORIENTED_EDGE('',*,*,#10237,.F.);
#13618=ORIENTED_EDGE('',*,*,#10238,.F.);
#13619=ORIENTED_EDGE('',*,*,#10239,.F.);
#13620=ORIENTED_EDGE('',*,*,#10240,.F.);
#13621=ORIENTED_EDGE('',*,*,#10241,.F.);
#13622=ORIENTED_EDGE('',*,*,#10242,.F.);
#13623=ORIENTED_EDGE('',*,*,#10200,.T.);
#13624=ORIENTED_EDGE('',*,*,#10243,.F.);
#13625=ORIENTED_EDGE('',*,*,#10241,.T.);
#13626=ORIENTED_EDGE('',*,*,#10244,.F.);
#13627=ORIENTED_EDGE('',*,*,#10245,.F.);
#13628=ORIENTED_EDGE('',*,*,#10246,.F.);
#13629=ORIENTED_EDGE('',*,*,#10247,.F.);
#13630=ORIENTED_EDGE('',*,*,#10248,.F.);
#13631=ORIENTED_EDGE('',*,*,#10249,.T.);
#13632=ORIENTED_EDGE('',*,*,#10250,.T.);
#13633=ORIENTED_EDGE('',*,*,#10251,.T.);
#13634=ORIENTED_EDGE('',*,*,#10252,.T.);
#13635=ORIENTED_EDGE('',*,*,#10253,.T.);
#13636=ORIENTED_EDGE('',*,*,#10254,.T.);
#13637=ORIENTED_EDGE('',*,*,#10255,.T.);
#13638=ORIENTED_EDGE('',*,*,#10256,.T.);
#13639=ORIENTED_EDGE('',*,*,#10257,.T.);
#13640=ORIENTED_EDGE('',*,*,#10258,.T.);
#13641=ORIENTED_EDGE('',*,*,#10215,.F.);
#13642=ORIENTED_EDGE('',*,*,#10259,.F.);
#13643=ORIENTED_EDGE('',*,*,#10260,.T.);
#13644=ORIENTED_EDGE('',*,*,#10261,.T.);
#13645=ORIENTED_EDGE('',*,*,#10216,.F.);
#13646=ORIENTED_EDGE('',*,*,#10258,.F.);
#13647=ORIENTED_EDGE('',*,*,#10262,.T.);
#13648=ORIENTED_EDGE('',*,*,#10263,.T.);
#13649=ORIENTED_EDGE('',*,*,#10264,.T.);
#13650=ORIENTED_EDGE('',*,*,#10265,.T.);
#13651=ORIENTED_EDGE('',*,*,#10266,.T.);
#13652=ORIENTED_EDGE('',*,*,#10267,.T.);
#13653=ORIENTED_EDGE('',*,*,#10268,.T.);
#13654=ORIENTED_EDGE('',*,*,#10269,.T.);
#13655=ORIENTED_EDGE('',*,*,#10270,.T.);
#13656=ORIENTED_EDGE('',*,*,#10271,.F.);
#13657=ORIENTED_EDGE('',*,*,#10272,.T.);
#13658=ORIENTED_EDGE('',*,*,#10273,.T.);
#13659=ORIENTED_EDGE('',*,*,#10274,.T.);
#13660=ORIENTED_EDGE('',*,*,#10275,.T.);
#13661=ORIENTED_EDGE('',*,*,#10270,.F.);
#13662=ORIENTED_EDGE('',*,*,#10276,.T.);
#13663=ORIENTED_EDGE('',*,*,#10274,.F.);
#13664=ORIENTED_EDGE('',*,*,#10277,.T.);
#13665=ORIENTED_EDGE('',*,*,#10278,.F.);
#13666=ORIENTED_EDGE('',*,*,#10279,.F.);
#13667=ORIENTED_EDGE('',*,*,#10280,.F.);
#13668=ORIENTED_EDGE('',*,*,#10281,.F.);
#13669=ORIENTED_EDGE('',*,*,#10282,.T.);
#13670=ORIENTED_EDGE('',*,*,#10283,.T.);
#13671=ORIENTED_EDGE('',*,*,#10284,.T.);
#13672=ORIENTED_EDGE('',*,*,#10285,.F.);
#13673=ORIENTED_EDGE('',*,*,#10266,.F.);
#13674=ORIENTED_EDGE('',*,*,#10286,.T.);
#13675=ORIENTED_EDGE('',*,*,#10287,.T.);
#13676=ORIENTED_EDGE('',*,*,#10288,.T.);
#13677=ORIENTED_EDGE('',*,*,#10271,.T.);
#13678=ORIENTED_EDGE('',*,*,#10275,.F.);
#13679=ORIENTED_EDGE('',*,*,#10289,.T.);
#13680=ORIENTED_EDGE('',*,*,#10290,.T.);
#13681=ORIENTED_EDGE('',*,*,#10289,.F.);
#13682=ORIENTED_EDGE('',*,*,#10276,.F.);
#13683=ORIENTED_EDGE('',*,*,#10291,.F.);
#13684=ORIENTED_EDGE('',*,*,#10292,.T.);
#13685=ORIENTED_EDGE('',*,*,#10293,.F.);
#13686=ORIENTED_EDGE('',*,*,#10292,.F.);
#13687=ORIENTED_EDGE('',*,*,#10294,.F.);
#13688=ORIENTED_EDGE('',*,*,#10295,.T.);
#13689=ORIENTED_EDGE('',*,*,#10296,.F.);
#13690=ORIENTED_EDGE('',*,*,#10295,.F.);
#13691=ORIENTED_EDGE('',*,*,#10297,.F.);
#13692=ORIENTED_EDGE('',*,*,#10298,.T.);
#13693=ORIENTED_EDGE('',*,*,#10299,.F.);
#13694=ORIENTED_EDGE('',*,*,#10298,.F.);
#13695=ORIENTED_EDGE('',*,*,#10300,.F.);
#13696=ORIENTED_EDGE('',*,*,#10301,.T.);
#13697=ORIENTED_EDGE('',*,*,#10302,.F.);
#13698=ORIENTED_EDGE('',*,*,#10301,.F.);
#13699=ORIENTED_EDGE('',*,*,#10303,.F.);
#13700=ORIENTED_EDGE('',*,*,#10304,.T.);
#13701=ORIENTED_EDGE('',*,*,#10305,.T.);
#13702=ORIENTED_EDGE('',*,*,#10306,.T.);
#13703=ORIENTED_EDGE('',*,*,#10307,.T.);
#13704=ORIENTED_EDGE('',*,*,#10308,.T.);
#13705=ORIENTED_EDGE('',*,*,#10309,.T.);
#13706=ORIENTED_EDGE('',*,*,#10308,.F.);
#13707=ORIENTED_EDGE('',*,*,#10310,.T.);
#13708=ORIENTED_EDGE('',*,*,#10311,.T.);
#13709=ORIENTED_EDGE('',*,*,#10312,.T.);
#13710=ORIENTED_EDGE('',*,*,#10304,.F.);
#13711=ORIENTED_EDGE('',*,*,#10313,.F.);
#13712=ORIENTED_EDGE('',*,*,#10314,.T.);
#13713=ORIENTED_EDGE('',*,*,#10315,.F.);
#13714=ORIENTED_EDGE('',*,*,#10314,.F.);
#13715=ORIENTED_EDGE('',*,*,#10316,.F.);
#13716=ORIENTED_EDGE('',*,*,#10317,.T.);
#13717=ORIENTED_EDGE('',*,*,#10318,.T.);
#13718=ORIENTED_EDGE('',*,*,#10317,.F.);
#13719=ORIENTED_EDGE('',*,*,#10309,.F.);
#13720=ORIENTED_EDGE('',*,*,#10319,.T.);
#13721=ORIENTED_EDGE('',*,*,#10320,.T.);
#13722=ORIENTED_EDGE('',*,*,#10319,.F.);
#13723=ORIENTED_EDGE('',*,*,#10321,.F.);
#13724=ORIENTED_EDGE('',*,*,#10322,.T.);
#13725=ORIENTED_EDGE('',*,*,#10323,.T.);
#13726=ORIENTED_EDGE('',*,*,#10322,.F.);
#13727=ORIENTED_EDGE('',*,*,#10324,.F.);
#13728=ORIENTED_EDGE('',*,*,#10325,.T.);
#13729=ORIENTED_EDGE('',*,*,#10326,.T.);
#13730=ORIENTED_EDGE('',*,*,#10325,.F.);
#13731=ORIENTED_EDGE('',*,*,#10327,.F.);
#13732=ORIENTED_EDGE('',*,*,#10328,.T.);
#13733=ORIENTED_EDGE('',*,*,#10329,.T.);
#13734=ORIENTED_EDGE('',*,*,#10328,.F.);
#13735=ORIENTED_EDGE('',*,*,#10330,.F.);
#13736=ORIENTED_EDGE('',*,*,#10331,.T.);
#13737=ORIENTED_EDGE('',*,*,#10332,.T.);
#13738=ORIENTED_EDGE('',*,*,#10331,.F.);
#13739=ORIENTED_EDGE('',*,*,#10333,.F.);
#13740=ORIENTED_EDGE('',*,*,#10334,.T.);
#13741=ORIENTED_EDGE('',*,*,#10335,.T.);
#13742=ORIENTED_EDGE('',*,*,#10334,.F.);
#13743=ORIENTED_EDGE('',*,*,#10336,.F.);
#13744=ORIENTED_EDGE('',*,*,#10337,.T.);
#13745=ORIENTED_EDGE('',*,*,#10338,.T.);
#13746=ORIENTED_EDGE('',*,*,#10337,.F.);
#13747=ORIENTED_EDGE('',*,*,#10339,.T.);
#13748=ORIENTED_EDGE('',*,*,#10340,.F.);
#13749=ORIENTED_EDGE('',*,*,#10341,.T.);
#13750=ORIENTED_EDGE('',*,*,#10342,.F.);
#13751=ORIENTED_EDGE('',*,*,#10134,.F.);
#13752=ORIENTED_EDGE('',*,*,#10343,.T.);
#13753=ORIENTED_EDGE('',*,*,#10344,.F.);
#13754=ORIENTED_EDGE('',*,*,#10345,.F.);
#13755=ORIENTED_EDGE('',*,*,#10343,.F.);
#13756=ORIENTED_EDGE('',*,*,#10133,.F.);
#13757=ORIENTED_EDGE('',*,*,#10346,.T.);
#13758=ORIENTED_EDGE('',*,*,#10347,.F.);
#13759=ORIENTED_EDGE('',*,*,#10348,.F.);
#13760=ORIENTED_EDGE('',*,*,#10349,.T.);
#13761=ORIENTED_EDGE('',*,*,#10350,.F.);
#13762=ORIENTED_EDGE('',*,*,#10351,.F.);
#13763=ORIENTED_EDGE('',*,*,#10352,.T.);
#13764=ORIENTED_EDGE('',*,*,#10344,.T.);
#13765=ORIENTED_EDGE('',*,*,#10345,.T.);
#13766=ORIENTED_EDGE('',*,*,#10352,.F.);
#13767=ORIENTED_EDGE('',*,*,#10353,.F.);
#13768=ORIENTED_EDGE('',*,*,#10354,.F.);
#13769=ORIENTED_EDGE('',*,*,#10355,.T.);
#13770=ORIENTED_EDGE('',*,*,#10350,.T.);
#13771=ORIENTED_EDGE('',*,*,#10351,.T.);
#13772=ORIENTED_EDGE('',*,*,#10355,.F.);
#13773=ORIENTED_EDGE('',*,*,#10356,.T.);
#13774=ORIENTED_EDGE('',*,*,#10357,.T.);
#13775=ORIENTED_EDGE('',*,*,#10358,.T.);
#13776=ORIENTED_EDGE('',*,*,#10359,.T.);
#13777=ORIENTED_EDGE('',*,*,#10360,.T.);
#13778=ORIENTED_EDGE('',*,*,#10361,.T.);
#13779=ORIENTED_EDGE('',*,*,#10362,.T.);
#13780=ORIENTED_EDGE('',*,*,#10363,.T.);
#13781=ORIENTED_EDGE('',*,*,#10364,.T.);
#13782=ORIENTED_EDGE('',*,*,#10365,.F.);
#13783=ORIENTED_EDGE('',*,*,#10366,.F.);
#13784=ORIENTED_EDGE('',*,*,#10367,.T.);
#13785=ORIENTED_EDGE('',*,*,#10368,.T.);
#13786=ORIENTED_EDGE('',*,*,#10369,.T.);
#13787=ORIENTED_EDGE('',*,*,#10370,.T.);
#13788=ORIENTED_EDGE('',*,*,#10371,.T.);
#13789=ORIENTED_EDGE('',*,*,#10372,.T.);
#13790=ORIENTED_EDGE('',*,*,#10373,.T.);
#13791=ORIENTED_EDGE('',*,*,#10374,.T.);
#13792=ORIENTED_EDGE('',*,*,#10375,.T.);
#13793=ORIENTED_EDGE('',*,*,#10376,.T.);
#13794=ORIENTED_EDGE('',*,*,#10377,.T.);
#13795=ORIENTED_EDGE('',*,*,#10378,.F.);
#13796=ORIENTED_EDGE('',*,*,#10377,.F.);
#13797=ORIENTED_EDGE('',*,*,#10379,.T.);
#13798=ORIENTED_EDGE('',*,*,#10380,.T.);
#13799=ORIENTED_EDGE('',*,*,#10381,.F.);
#13800=ORIENTED_EDGE('',*,*,#10380,.F.);
#13801=ORIENTED_EDGE('',*,*,#10353,.T.);
#13802=ORIENTED_EDGE('',*,*,#10354,.T.);
#13803=ORIENTED_EDGE('',*,*,#10382,.T.);
#13804=ORIENTED_EDGE('',*,*,#10383,.F.);
#13805=ORIENTED_EDGE('',*,*,#10382,.F.);
#13806=ORIENTED_EDGE('',*,*,#10384,.T.);
#13807=ORIENTED_EDGE('',*,*,#10385,.T.);
#13808=ORIENTED_EDGE('',*,*,#10386,.F.);
#13809=ORIENTED_EDGE('',*,*,#10387,.F.);
#13810=ORIENTED_EDGE('',*,*,#10385,.F.);
#13811=ORIENTED_EDGE('',*,*,#10388,.F.);
#13812=ORIENTED_EDGE('',*,*,#10389,.T.);
#13813=ORIENTED_EDGE('',*,*,#10390,.F.);
#13814=ORIENTED_EDGE('',*,*,#10391,.F.);
#13815=ORIENTED_EDGE('',*,*,#10392,.T.);
#13816=ORIENTED_EDGE('',*,*,#10386,.T.);
#13817=ORIENTED_EDGE('',*,*,#10387,.T.);
#13818=ORIENTED_EDGE('',*,*,#10392,.F.);
#13819=ORIENTED_EDGE('',*,*,#10393,.F.);
#13820=ORIENTED_EDGE('',*,*,#10394,.F.);
#13821=ORIENTED_EDGE('',*,*,#10395,.F.);
#13822=ORIENTED_EDGE('',*,*,#10396,.F.);
#13823=ORIENTED_EDGE('',*,*,#10127,.F.);
#13824=ORIENTED_EDGE('',*,*,#10395,.T.);
#13825=ORIENTED_EDGE('',*,*,#10397,.T.);
#13826=ORIENTED_EDGE('',*,*,#10398,.F.);
#13827=ORIENTED_EDGE('',*,*,#10399,.T.);
#13828=ORIENTED_EDGE('',*,*,#10400,.F.);
#13829=ORIENTED_EDGE('',*,*,#10401,.F.);
#13830=ORIENTED_EDGE('',*,*,#10402,.F.);
#13831=ORIENTED_EDGE('',*,*,#10403,.F.);
#13832=ORIENTED_EDGE('',*,*,#10404,.F.);
#13833=ORIENTED_EDGE('',*,*,#10405,.T.);
#13834=ORIENTED_EDGE('',*,*,#10371,.F.);
#13835=ORIENTED_EDGE('',*,*,#10406,.F.);
#13836=ORIENTED_EDGE('',*,*,#10369,.F.);
#13837=ORIENTED_EDGE('',*,*,#10407,.F.);
#13838=ORIENTED_EDGE('',*,*,#10408,.F.);
#13839=ORIENTED_EDGE('',*,*,#10409,.F.);
#13840=ORIENTED_EDGE('',*,*,#10410,.F.);
#13841=ORIENTED_EDGE('',*,*,#10408,.T.);
#13842=ORIENTED_EDGE('',*,*,#10411,.T.);
#13843=ORIENTED_EDGE('',*,*,#10412,.T.);
#13844=ORIENTED_EDGE('',*,*,#10413,.F.);
#13845=ORIENTED_EDGE('',*,*,#10414,.F.);
#13846=ORIENTED_EDGE('',*,*,#10415,.F.);
#13847=ORIENTED_EDGE('',*,*,#10416,.F.);
#13848=ORIENTED_EDGE('',*,*,#10414,.T.);
#13849=ORIENTED_EDGE('',*,*,#10417,.T.);
#13850=ORIENTED_EDGE('',*,*,#10418,.F.);
#13851=ORIENTED_EDGE('',*,*,#10419,.T.);
#13852=ORIENTED_EDGE('',*,*,#10420,.F.);
#13853=ORIENTED_EDGE('',*,*,#10421,.F.);
#13854=ORIENTED_EDGE('',*,*,#10422,.F.);
#13855=ORIENTED_EDGE('',*,*,#10423,.F.);
#13856=ORIENTED_EDGE('',*,*,#10424,.F.);
#13857=ORIENTED_EDGE('',*,*,#10425,.F.);
#13858=ORIENTED_EDGE('',*,*,#10426,.F.);
#13859=ORIENTED_EDGE('',*,*,#10427,.F.);
#13860=ORIENTED_EDGE('',*,*,#10428,.F.);
#13861=ORIENTED_EDGE('',*,*,#10429,.F.);
#13862=ORIENTED_EDGE('',*,*,#10430,.F.);
#13863=ORIENTED_EDGE('',*,*,#10431,.F.);
#13864=ORIENTED_EDGE('',*,*,#10432,.F.);
#13865=ORIENTED_EDGE('',*,*,#10433,.F.);
#13866=ORIENTED_EDGE('',*,*,#10434,.F.);
#13867=ORIENTED_EDGE('',*,*,#10435,.F.);
#13868=ORIENTED_EDGE('',*,*,#10436,.F.);
#13869=ORIENTED_EDGE('',*,*,#10437,.F.);
#13870=ORIENTED_EDGE('',*,*,#10438,.F.);
#13871=ORIENTED_EDGE('',*,*,#10439,.F.);
#13872=ORIENTED_EDGE('',*,*,#10440,.F.);
#13873=ORIENTED_EDGE('',*,*,#10441,.F.);
#13874=ORIENTED_EDGE('',*,*,#10442,.F.);
#13875=ORIENTED_EDGE('',*,*,#10443,.F.);
#13876=ORIENTED_EDGE('',*,*,#10444,.F.);
#13877=ORIENTED_EDGE('',*,*,#10445,.F.);
#13878=ORIENTED_EDGE('',*,*,#10446,.F.);
#13879=ORIENTED_EDGE('',*,*,#10447,.F.);
#13880=ORIENTED_EDGE('',*,*,#10448,.T.);
#13881=ORIENTED_EDGE('',*,*,#10449,.T.);
#13882=ORIENTED_EDGE('',*,*,#10450,.T.);
#13883=ORIENTED_EDGE('',*,*,#10451,.T.);
#13884=ORIENTED_EDGE('',*,*,#10452,.T.);
#13885=ORIENTED_EDGE('',*,*,#10453,.T.);
#13886=ORIENTED_EDGE('',*,*,#10454,.T.);
#13887=ORIENTED_EDGE('',*,*,#10388,.T.);
#13888=ORIENTED_EDGE('',*,*,#10455,.T.);
#13889=ORIENTED_EDGE('',*,*,#10456,.T.);
#13890=ORIENTED_EDGE('',*,*,#10457,.T.);
#13891=ORIENTED_EDGE('',*,*,#10458,.T.);
#13892=ORIENTED_EDGE('',*,*,#10459,.T.);
#13893=ORIENTED_EDGE('',*,*,#10460,.T.);
#13894=ORIENTED_EDGE('',*,*,#10461,.T.);
#13895=ORIENTED_EDGE('',*,*,#10462,.T.);
#13896=ORIENTED_EDGE('',*,*,#10463,.T.);
#13897=ORIENTED_EDGE('',*,*,#10464,.T.);
#13898=ORIENTED_EDGE('',*,*,#10465,.T.);
#13899=ORIENTED_EDGE('',*,*,#10466,.T.);
#13900=ORIENTED_EDGE('',*,*,#10467,.T.);
#13901=ORIENTED_EDGE('',*,*,#10468,.T.);
#13902=ORIENTED_EDGE('',*,*,#10469,.T.);
#13903=ORIENTED_EDGE('',*,*,#10470,.T.);
#13904=ORIENTED_EDGE('',*,*,#10471,.T.);
#13905=ORIENTED_EDGE('',*,*,#10472,.T.);
#13906=ORIENTED_EDGE('',*,*,#10473,.T.);
#13907=ORIENTED_EDGE('',*,*,#10474,.T.);
#13908=ORIENTED_EDGE('',*,*,#10475,.T.);
#13909=ORIENTED_EDGE('',*,*,#10476,.F.);
#13910=ORIENTED_EDGE('',*,*,#10427,.T.);
#13911=ORIENTED_EDGE('',*,*,#10477,.F.);
#13912=ORIENTED_EDGE('',*,*,#10478,.T.);
#13913=ORIENTED_EDGE('',*,*,#10479,.F.);
#13914=ORIENTED_EDGE('',*,*,#10428,.T.);
#13915=ORIENTED_EDGE('',*,*,#10476,.T.);
#13916=ORIENTED_EDGE('',*,*,#10480,.T.);
#13917=ORIENTED_EDGE('',*,*,#10481,.F.);
#13918=ORIENTED_EDGE('',*,*,#10429,.T.);
#13919=ORIENTED_EDGE('',*,*,#10479,.T.);
#13920=ORIENTED_EDGE('',*,*,#10482,.T.);
#13921=ORIENTED_EDGE('',*,*,#10483,.F.);
#13922=ORIENTED_EDGE('',*,*,#10424,.T.);
#13923=ORIENTED_EDGE('',*,*,#10481,.T.);
#13924=ORIENTED_EDGE('',*,*,#10484,.T.);
#13925=ORIENTED_EDGE('',*,*,#10485,.F.);
#13926=ORIENTED_EDGE('',*,*,#10425,.T.);
#13927=ORIENTED_EDGE('',*,*,#10483,.T.);
#13928=ORIENTED_EDGE('',*,*,#10486,.T.);
#13929=ORIENTED_EDGE('',*,*,#10477,.T.);
#13930=ORIENTED_EDGE('',*,*,#10426,.T.);
#13931=ORIENTED_EDGE('',*,*,#10485,.T.);
#13932=ORIENTED_EDGE('',*,*,#10487,.F.);
#13933=ORIENTED_EDGE('',*,*,#10488,.T.);
#13934=ORIENTED_EDGE('',*,*,#10489,.T.);
#13935=ORIENTED_EDGE('',*,*,#10490,.F.);
#13936=ORIENTED_EDGE('',*,*,#10491,.F.);
#13937=ORIENTED_EDGE('',*,*,#10492,.T.);
#13938=ORIENTED_EDGE('',*,*,#10493,.F.);
#13939=ORIENTED_EDGE('',*,*,#10489,.F.);
#13940=ORIENTED_EDGE('',*,*,#10494,.T.);
#13941=ORIENTED_EDGE('',*,*,#10495,.F.);
#13942=ORIENTED_EDGE('',*,*,#10492,.F.);
#13943=ORIENTED_EDGE('',*,*,#10496,.T.);
#13944=ORIENTED_EDGE('',*,*,#10497,.F.);
#13945=ORIENTED_EDGE('',*,*,#10498,.F.);
#13946=ORIENTED_EDGE('',*,*,#10499,.F.);
#13947=ORIENTED_EDGE('',*,*,#10500,.F.);
#13948=ORIENTED_EDGE('',*,*,#10432,.T.);
#13949=ORIENTED_EDGE('',*,*,#10501,.F.);
#13950=ORIENTED_EDGE('',*,*,#10502,.F.);
#13951=ORIENTED_EDGE('',*,*,#10501,.T.);
#13952=ORIENTED_EDGE('',*,*,#10431,.T.);
#13953=ORIENTED_EDGE('',*,*,#10503,.F.);
#13954=ORIENTED_EDGE('',*,*,#10504,.F.);
#13955=ORIENTED_EDGE('',*,*,#10503,.T.);
#13956=ORIENTED_EDGE('',*,*,#10430,.T.);
#13957=ORIENTED_EDGE('',*,*,#10505,.F.);
#13958=ORIENTED_EDGE('',*,*,#10506,.F.);
#13959=ORIENTED_EDGE('',*,*,#10505,.T.);
#13960=ORIENTED_EDGE('',*,*,#10435,.T.);
#13961=ORIENTED_EDGE('',*,*,#10507,.F.);
#13962=ORIENTED_EDGE('',*,*,#10508,.F.);
#13963=ORIENTED_EDGE('',*,*,#10507,.T.);
#13964=ORIENTED_EDGE('',*,*,#10434,.T.);
#13965=ORIENTED_EDGE('',*,*,#10509,.F.);
#13966=ORIENTED_EDGE('',*,*,#10510,.F.);
#13967=ORIENTED_EDGE('',*,*,#10509,.T.);
#13968=ORIENTED_EDGE('',*,*,#10433,.T.);
#13969=ORIENTED_EDGE('',*,*,#10500,.T.);
#13970=ORIENTED_EDGE('',*,*,#10511,.F.);
#13971=ORIENTED_EDGE('',*,*,#10512,.T.);
#13972=ORIENTED_EDGE('',*,*,#10513,.F.);
#13973=ORIENTED_EDGE('',*,*,#10514,.F.);
#13974=ORIENTED_EDGE('',*,*,#10515,.F.);
#13975=ORIENTED_EDGE('',*,*,#10516,.T.);
#13976=ORIENTED_EDGE('',*,*,#10517,.F.);
#13977=ORIENTED_EDGE('',*,*,#10512,.F.);
#13978=ORIENTED_EDGE('',*,*,#10518,.F.);
#13979=ORIENTED_EDGE('',*,*,#10519,.F.);
#13980=ORIENTED_EDGE('',*,*,#10520,.F.);
#13981=ORIENTED_EDGE('',*,*,#10516,.F.);
#13982=ORIENTED_EDGE('',*,*,#10521,.F.);
#13983=ORIENTED_EDGE('',*,*,#10522,.F.);
#13984=ORIENTED_EDGE('',*,*,#10523,.F.);
#13985=ORIENTED_EDGE('',*,*,#10524,.F.);
#13986=ORIENTED_EDGE('',*,*,#10438,.T.);
#13987=ORIENTED_EDGE('',*,*,#10525,.F.);
#13988=ORIENTED_EDGE('',*,*,#10526,.F.);
#13989=ORIENTED_EDGE('',*,*,#10525,.T.);
#13990=ORIENTED_EDGE('',*,*,#10437,.T.);
#13991=ORIENTED_EDGE('',*,*,#10527,.F.);
#13992=ORIENTED_EDGE('',*,*,#10528,.F.);
#13993=ORIENTED_EDGE('',*,*,#10527,.T.);
#13994=ORIENTED_EDGE('',*,*,#10436,.T.);
#13995=ORIENTED_EDGE('',*,*,#10529,.F.);
#13996=ORIENTED_EDGE('',*,*,#10530,.F.);
#13997=ORIENTED_EDGE('',*,*,#10529,.T.);
#13998=ORIENTED_EDGE('',*,*,#10441,.T.);
#13999=ORIENTED_EDGE('',*,*,#10531,.F.);
#14000=ORIENTED_EDGE('',*,*,#10532,.F.);
#14001=ORIENTED_EDGE('',*,*,#10531,.T.);
#14002=ORIENTED_EDGE('',*,*,#10440,.T.);
#14003=ORIENTED_EDGE('',*,*,#10533,.F.);
#14004=ORIENTED_EDGE('',*,*,#10534,.F.);
#14005=ORIENTED_EDGE('',*,*,#10533,.T.);
#14006=ORIENTED_EDGE('',*,*,#10439,.T.);
#14007=ORIENTED_EDGE('',*,*,#10524,.T.);
#14008=ORIENTED_EDGE('',*,*,#10535,.F.);
#14009=ORIENTED_EDGE('',*,*,#10536,.T.);
#14010=ORIENTED_EDGE('',*,*,#10537,.F.);
#14011=ORIENTED_EDGE('',*,*,#10538,.F.);
#14012=ORIENTED_EDGE('',*,*,#10539,.F.);
#14013=ORIENTED_EDGE('',*,*,#10540,.T.);
#14014=ORIENTED_EDGE('',*,*,#10541,.F.);
#14015=ORIENTED_EDGE('',*,*,#10536,.F.);
#14016=ORIENTED_EDGE('',*,*,#10542,.F.);
#14017=ORIENTED_EDGE('',*,*,#10543,.F.);
#14018=ORIENTED_EDGE('',*,*,#10544,.F.);
#14019=ORIENTED_EDGE('',*,*,#10540,.F.);
#14020=ORIENTED_EDGE('',*,*,#10545,.F.);
#14021=ORIENTED_EDGE('',*,*,#10546,.F.);
#14022=ORIENTED_EDGE('',*,*,#10490,.T.);
#14023=ORIENTED_EDGE('',*,*,#10493,.T.);
#14024=ORIENTED_EDGE('',*,*,#10495,.T.);
#14025=ORIENTED_EDGE('',*,*,#10547,.F.);
#14026=ORIENTED_EDGE('',*,*,#10521,.T.);
#14027=ORIENTED_EDGE('',*,*,#10518,.T.);
#14028=ORIENTED_EDGE('',*,*,#10511,.T.);
#14029=ORIENTED_EDGE('',*,*,#10548,.F.);
#14030=ORIENTED_EDGE('',*,*,#10549,.T.);
#14031=ORIENTED_EDGE('',*,*,#10550,.T.);
#14032=ORIENTED_EDGE('',*,*,#10551,.T.);
#14033=ORIENTED_EDGE('',*,*,#10552,.F.);
#14034=ORIENTED_EDGE('',*,*,#10545,.T.);
#14035=ORIENTED_EDGE('',*,*,#10542,.T.);
#14036=ORIENTED_EDGE('',*,*,#10535,.T.);
#14037=ORIENTED_EDGE('',*,*,#10553,.F.);
#14038=ORIENTED_EDGE('',*,*,#10554,.F.);
#14039=ORIENTED_EDGE('',*,*,#10555,.F.);
#14040=ORIENTED_EDGE('',*,*,#10444,.T.);
#14041=ORIENTED_EDGE('',*,*,#10556,.F.);
#14042=ORIENTED_EDGE('',*,*,#10557,.F.);
#14043=ORIENTED_EDGE('',*,*,#10556,.T.);
#14044=ORIENTED_EDGE('',*,*,#10443,.T.);
#14045=ORIENTED_EDGE('',*,*,#10558,.F.);
#14046=ORIENTED_EDGE('',*,*,#10559,.F.);
#14047=ORIENTED_EDGE('',*,*,#10558,.T.);
#14048=ORIENTED_EDGE('',*,*,#10442,.T.);
#14049=ORIENTED_EDGE('',*,*,#10560,.F.);
#14050=ORIENTED_EDGE('',*,*,#10561,.F.);
#14051=ORIENTED_EDGE('',*,*,#10560,.T.);
#14052=ORIENTED_EDGE('',*,*,#10447,.T.);
#14053=ORIENTED_EDGE('',*,*,#10562,.F.);
#14054=ORIENTED_EDGE('',*,*,#10563,.F.);
#14055=ORIENTED_EDGE('',*,*,#10562,.T.);
#14056=ORIENTED_EDGE('',*,*,#10446,.T.);
#14057=ORIENTED_EDGE('',*,*,#10564,.F.);
#14058=ORIENTED_EDGE('',*,*,#10565,.F.);
#14059=ORIENTED_EDGE('',*,*,#10564,.T.);
#14060=ORIENTED_EDGE('',*,*,#10445,.T.);
#14061=ORIENTED_EDGE('',*,*,#10555,.T.);
#14062=ORIENTED_EDGE('',*,*,#10551,.F.);
#14063=ORIENTED_EDGE('',*,*,#10566,.T.);
#14064=ORIENTED_EDGE('',*,*,#10567,.F.);
#14065=ORIENTED_EDGE('',*,*,#10568,.F.);
#14066=ORIENTED_EDGE('',*,*,#10569,.F.);
#14067=ORIENTED_EDGE('',*,*,#10570,.T.);
#14068=ORIENTED_EDGE('',*,*,#10571,.F.);
#14069=ORIENTED_EDGE('',*,*,#10566,.F.);
#14070=ORIENTED_EDGE('',*,*,#10550,.F.);
#14071=ORIENTED_EDGE('',*,*,#10572,.F.);
#14072=ORIENTED_EDGE('',*,*,#10573,.F.);
#14073=ORIENTED_EDGE('',*,*,#10570,.F.);
#14074=ORIENTED_EDGE('',*,*,#10549,.F.);
#14075=ORIENTED_EDGE('',*,*,#10574,.F.);
#14076=ORIENTED_EDGE('',*,*,#10575,.T.);
#14077=ORIENTED_EDGE('',*,*,#10450,.F.);
#14078=ORIENTED_EDGE('',*,*,#10576,.T.);
#14079=ORIENTED_EDGE('',*,*,#10577,.F.);
#14080=ORIENTED_EDGE('',*,*,#10576,.F.);
#14081=ORIENTED_EDGE('',*,*,#10449,.F.);
#14082=ORIENTED_EDGE('',*,*,#10578,.T.);
#14083=ORIENTED_EDGE('',*,*,#10579,.F.);
#14084=ORIENTED_EDGE('',*,*,#10578,.F.);
#14085=ORIENTED_EDGE('',*,*,#10448,.F.);
#14086=ORIENTED_EDGE('',*,*,#10580,.T.);
#14087=ORIENTED_EDGE('',*,*,#10581,.F.);
#14088=ORIENTED_EDGE('',*,*,#10580,.F.);
#14089=ORIENTED_EDGE('',*,*,#10462,.F.);
#14090=ORIENTED_EDGE('',*,*,#10582,.T.);
#14091=ORIENTED_EDGE('',*,*,#10583,.F.);
#14092=ORIENTED_EDGE('',*,*,#10582,.F.);
#14093=ORIENTED_EDGE('',*,*,#10461,.F.);
#14094=ORIENTED_EDGE('',*,*,#10584,.T.);
#14095=ORIENTED_EDGE('',*,*,#10585,.F.);
#14096=ORIENTED_EDGE('',*,*,#10584,.F.);
#14097=ORIENTED_EDGE('',*,*,#10460,.F.);
#14098=ORIENTED_EDGE('',*,*,#10586,.T.);
#14099=ORIENTED_EDGE('',*,*,#10587,.F.);
#14100=ORIENTED_EDGE('',*,*,#10586,.F.);
#14101=ORIENTED_EDGE('',*,*,#10459,.F.);
#14102=ORIENTED_EDGE('',*,*,#10588,.T.);
#14103=ORIENTED_EDGE('',*,*,#10589,.F.);
#14104=ORIENTED_EDGE('',*,*,#10458,.F.);
#14105=ORIENTED_EDGE('',*,*,#10590,.T.);
#14106=ORIENTED_EDGE('',*,*,#10591,.F.);
#14107=ORIENTED_EDGE('',*,*,#10588,.F.);
#14108=ORIENTED_EDGE('',*,*,#10590,.F.);
#14109=ORIENTED_EDGE('',*,*,#10457,.F.);
#14110=ORIENTED_EDGE('',*,*,#10592,.T.);
#14111=ORIENTED_EDGE('',*,*,#10593,.F.);
#14112=ORIENTED_EDGE('',*,*,#10592,.F.);
#14113=ORIENTED_EDGE('',*,*,#10456,.F.);
#14114=ORIENTED_EDGE('',*,*,#10594,.T.);
#14115=ORIENTED_EDGE('',*,*,#10595,.F.);
#14116=ORIENTED_EDGE('',*,*,#10594,.F.);
#14117=ORIENTED_EDGE('',*,*,#10455,.F.);
#14118=ORIENTED_EDGE('',*,*,#10391,.T.);
#14119=ORIENTED_EDGE('',*,*,#10596,.F.);
#14120=ORIENTED_EDGE('',*,*,#10389,.F.);
#14121=ORIENTED_EDGE('',*,*,#10454,.F.);
#14122=ORIENTED_EDGE('',*,*,#10597,.T.);
#14123=ORIENTED_EDGE('',*,*,#10598,.F.);
#14124=ORIENTED_EDGE('',*,*,#10597,.F.);
#14125=ORIENTED_EDGE('',*,*,#10453,.F.);
#14126=ORIENTED_EDGE('',*,*,#10599,.T.);
#14127=ORIENTED_EDGE('',*,*,#10600,.F.);
#14128=ORIENTED_EDGE('',*,*,#10599,.F.);
#14129=ORIENTED_EDGE('',*,*,#10452,.F.);
#14130=ORIENTED_EDGE('',*,*,#10601,.T.);
#14131=ORIENTED_EDGE('',*,*,#10602,.F.);
#14132=ORIENTED_EDGE('',*,*,#10451,.F.);
#14133=ORIENTED_EDGE('',*,*,#10575,.F.);
#14134=ORIENTED_EDGE('',*,*,#10603,.F.);
#14135=ORIENTED_EDGE('',*,*,#10601,.F.);
#14136=ORIENTED_EDGE('',*,*,#10604,.T.);
#14137=ORIENTED_EDGE('',*,*,#10464,.F.);
#14138=ORIENTED_EDGE('',*,*,#10605,.T.);
#14139=ORIENTED_EDGE('',*,*,#10606,.F.);
#14140=ORIENTED_EDGE('',*,*,#10605,.F.);
#14141=ORIENTED_EDGE('',*,*,#10463,.F.);
#14142=ORIENTED_EDGE('',*,*,#10607,.T.);
#14143=ORIENTED_EDGE('',*,*,#10608,.F.);
#14144=ORIENTED_EDGE('',*,*,#10607,.F.);
#14145=ORIENTED_EDGE('',*,*,#10468,.F.);
#14146=ORIENTED_EDGE('',*,*,#10609,.T.);
#14147=ORIENTED_EDGE('',*,*,#10610,.F.);
#14148=ORIENTED_EDGE('',*,*,#10609,.F.);
#14149=ORIENTED_EDGE('',*,*,#10467,.F.);
#14150=ORIENTED_EDGE('',*,*,#10611,.T.);
#14151=ORIENTED_EDGE('',*,*,#10612,.F.);
#14152=ORIENTED_EDGE('',*,*,#10611,.F.);
#14153=ORIENTED_EDGE('',*,*,#10466,.F.);
#14154=ORIENTED_EDGE('',*,*,#10613,.T.);
#14155=ORIENTED_EDGE('',*,*,#10614,.F.);
#14156=ORIENTED_EDGE('',*,*,#10613,.F.);
#14157=ORIENTED_EDGE('',*,*,#10465,.F.);
#14158=ORIENTED_EDGE('',*,*,#10604,.F.);
#14159=ORIENTED_EDGE('',*,*,#10615,.F.);
#14160=ORIENTED_EDGE('',*,*,#10616,.T.);
#14161=ORIENTED_EDGE('',*,*,#10470,.F.);
#14162=ORIENTED_EDGE('',*,*,#10617,.T.);
#14163=ORIENTED_EDGE('',*,*,#10618,.F.);
#14164=ORIENTED_EDGE('',*,*,#10617,.F.);
#14165=ORIENTED_EDGE('',*,*,#10469,.F.);
#14166=ORIENTED_EDGE('',*,*,#10619,.T.);
#14167=ORIENTED_EDGE('',*,*,#10620,.F.);
#14168=ORIENTED_EDGE('',*,*,#10619,.F.);
#14169=ORIENTED_EDGE('',*,*,#10474,.F.);
#14170=ORIENTED_EDGE('',*,*,#10621,.T.);
#14171=ORIENTED_EDGE('',*,*,#10622,.F.);
#14172=ORIENTED_EDGE('',*,*,#10621,.F.);
#14173=ORIENTED_EDGE('',*,*,#10473,.F.);
#14174=ORIENTED_EDGE('',*,*,#10623,.T.);
#14175=ORIENTED_EDGE('',*,*,#10624,.F.);
#14176=ORIENTED_EDGE('',*,*,#10623,.F.);
#14177=ORIENTED_EDGE('',*,*,#10472,.F.);
#14178=ORIENTED_EDGE('',*,*,#10625,.T.);
#14179=ORIENTED_EDGE('',*,*,#10626,.F.);
#14180=ORIENTED_EDGE('',*,*,#10625,.F.);
#14181=ORIENTED_EDGE('',*,*,#10471,.F.);
#14182=ORIENTED_EDGE('',*,*,#10616,.F.);
#14183=ORIENTED_EDGE('',*,*,#10627,.F.);
#14184=ORIENTED_EDGE('',*,*,#10539,.T.);
#14185=ORIENTED_EDGE('',*,*,#10628,.F.);
#14186=ORIENTED_EDGE('',*,*,#10491,.T.);
#14187=ORIENTED_EDGE('',*,*,#10553,.T.);
#14188=ORIENTED_EDGE('',*,*,#10522,.T.);
#14189=ORIENTED_EDGE('',*,*,#10547,.T.);
#14190=ORIENTED_EDGE('',*,*,#10498,.T.);
#14191=ORIENTED_EDGE('',*,*,#10629,.F.);
#14192=ORIENTED_EDGE('',*,*,#10630,.F.);
#14193=ORIENTED_EDGE('',*,*,#10631,.F.);
#14194=ORIENTED_EDGE('',*,*,#10496,.F.);
#14195=ORIENTED_EDGE('',*,*,#10494,.F.);
#14196=ORIENTED_EDGE('',*,*,#10488,.F.);
#14197=ORIENTED_EDGE('',*,*,#10632,.F.);
#14198=ORIENTED_EDGE('',*,*,#10484,.F.);
#14199=ORIENTED_EDGE('',*,*,#10482,.F.);
#14200=ORIENTED_EDGE('',*,*,#10480,.F.);
#14201=ORIENTED_EDGE('',*,*,#10478,.F.);
#14202=ORIENTED_EDGE('',*,*,#10475,.F.);
#14203=ORIENTED_EDGE('',*,*,#10486,.F.);
#14204=ORIENTED_EDGE('',*,*,#10515,.T.);
#14205=ORIENTED_EDGE('',*,*,#10633,.F.);
#14206=ORIENTED_EDGE('',*,*,#10574,.T.);
#14207=ORIENTED_EDGE('',*,*,#10548,.T.);
#14208=ORIENTED_EDGE('',*,*,#10517,.T.);
#14209=ORIENTED_EDGE('',*,*,#10520,.T.);
#14210=ORIENTED_EDGE('',*,*,#10634,.F.);
#14211=ORIENTED_EDGE('',*,*,#10635,.F.);
#14212=ORIENTED_EDGE('',*,*,#10636,.F.);
#14213=ORIENTED_EDGE('',*,*,#10513,.T.);
#14214=ORIENTED_EDGE('',*,*,#10508,.T.);
#14215=ORIENTED_EDGE('',*,*,#10510,.T.);
#14216=ORIENTED_EDGE('',*,*,#10499,.T.);
#14217=ORIENTED_EDGE('',*,*,#10502,.T.);
#14218=ORIENTED_EDGE('',*,*,#10504,.T.);
#14219=ORIENTED_EDGE('',*,*,#10506,.T.);
#14220=ORIENTED_EDGE('',*,*,#10541,.T.);
#14221=ORIENTED_EDGE('',*,*,#10544,.T.);
#14222=ORIENTED_EDGE('',*,*,#10637,.F.);
#14223=ORIENTED_EDGE('',*,*,#10638,.F.);
#14224=ORIENTED_EDGE('',*,*,#10639,.F.);
#14225=ORIENTED_EDGE('',*,*,#10537,.T.);
#14226=ORIENTED_EDGE('',*,*,#10532,.T.);
#14227=ORIENTED_EDGE('',*,*,#10534,.T.);
#14228=ORIENTED_EDGE('',*,*,#10523,.T.);
#14229=ORIENTED_EDGE('',*,*,#10526,.T.);
#14230=ORIENTED_EDGE('',*,*,#10528,.T.);
#14231=ORIENTED_EDGE('',*,*,#10530,.T.);
#14232=ORIENTED_EDGE('',*,*,#10569,.T.);
#14233=ORIENTED_EDGE('',*,*,#10640,.F.);
#14234=ORIENTED_EDGE('',*,*,#10546,.T.);
#14235=ORIENTED_EDGE('',*,*,#10552,.T.);
#14236=ORIENTED_EDGE('',*,*,#10571,.T.);
#14237=ORIENTED_EDGE('',*,*,#10573,.T.);
#14238=ORIENTED_EDGE('',*,*,#10641,.F.);
#14239=ORIENTED_EDGE('',*,*,#10642,.F.);
#14240=ORIENTED_EDGE('',*,*,#10643,.F.);
#14241=ORIENTED_EDGE('',*,*,#10567,.T.);
#14242=ORIENTED_EDGE('',*,*,#10563,.T.);
#14243=ORIENTED_EDGE('',*,*,#10565,.T.);
#14244=ORIENTED_EDGE('',*,*,#10554,.T.);
#14245=ORIENTED_EDGE('',*,*,#10557,.T.);
#14246=ORIENTED_EDGE('',*,*,#10559,.T.);
#14247=ORIENTED_EDGE('',*,*,#10561,.T.);
#14248=ORIENTED_EDGE('',*,*,#10644,.F.);
#14249=ORIENTED_EDGE('',*,*,#10645,.F.);
#14250=ORIENTED_EDGE('',*,*,#10646,.F.);
#14251=ORIENTED_EDGE('',*,*,#10647,.F.);
#14252=ORIENTED_EDGE('',*,*,#10646,.T.);
#14253=ORIENTED_EDGE('',*,*,#10648,.F.);
#14254=ORIENTED_EDGE('',*,*,#10649,.F.);
#14255=ORIENTED_EDGE('',*,*,#10650,.F.);
#14256=ORIENTED_EDGE('',*,*,#10649,.T.);
#14257=ORIENTED_EDGE('',*,*,#10651,.F.);
#14258=ORIENTED_EDGE('',*,*,#10652,.F.);
#14259=ORIENTED_EDGE('',*,*,#10653,.F.);
#14260=ORIENTED_EDGE('',*,*,#10419,.F.);
#14261=ORIENTED_EDGE('',*,*,#10654,.F.);
#14262=ORIENTED_EDGE('',*,*,#10655,.F.);
#14263=ORIENTED_EDGE('',*,*,#10656,.F.);
#14264=ORIENTED_EDGE('',*,*,#10655,.T.);
#14265=ORIENTED_EDGE('',*,*,#10657,.F.);
#14266=ORIENTED_EDGE('',*,*,#10658,.F.);
#14267=ORIENTED_EDGE('',*,*,#10659,.F.);
#14268=ORIENTED_EDGE('',*,*,#10660,.F.);
#14269=ORIENTED_EDGE('',*,*,#10658,.T.);
#14270=ORIENTED_EDGE('',*,*,#10661,.F.);
#14271=ORIENTED_EDGE('',*,*,#10412,.F.);
#14272=ORIENTED_EDGE('',*,*,#10399,.F.);
#14273=ORIENTED_EDGE('',*,*,#10662,.F.);
#14274=ORIENTED_EDGE('',*,*,#10663,.F.);
#14275=ORIENTED_EDGE('',*,*,#10128,.F.);
#14276=ORIENTED_EDGE('',*,*,#10663,.T.);
#14277=ORIENTED_EDGE('',*,*,#10664,.F.);
#14278=ORIENTED_EDGE('',*,*,#10665,.F.);
#14279=ORIENTED_EDGE('',*,*,#10129,.F.);
#14280=ORIENTED_EDGE('',*,*,#10130,.F.);
#14281=ORIENTED_EDGE('',*,*,#10665,.T.);
#14282=ORIENTED_EDGE('',*,*,#10666,.F.);
#14283=ORIENTED_EDGE('',*,*,#10123,.F.);
#14284=ORIENTED_EDGE('',*,*,#10667,.T.);
#14285=ORIENTED_EDGE('',*,*,#10668,.F.);
#14286=ORIENTED_EDGE('',*,*,#10669,.F.);
#14287=ORIENTED_EDGE('',*,*,#10670,.F.);
#14288=ORIENTED_EDGE('',*,*,#10669,.T.);
#14289=ORIENTED_EDGE('',*,*,#10671,.F.);
#14290=ORIENTED_EDGE('',*,*,#10672,.F.);
#14291=ORIENTED_EDGE('',*,*,#10673,.F.);
#14292=ORIENTED_EDGE('',*,*,#10674,.F.);
#14293=ORIENTED_EDGE('',*,*,#10672,.T.);
#14294=ORIENTED_EDGE('',*,*,#10675,.F.);
#14295=ORIENTED_EDGE('',*,*,#10676,.F.);
#14296=ORIENTED_EDGE('',*,*,#10677,.T.);
#14297=ORIENTED_EDGE('',*,*,#10678,.F.);
#14298=ORIENTED_EDGE('',*,*,#10124,.F.);
#14299=ORIENTED_EDGE('',*,*,#10666,.T.);
#14300=ORIENTED_EDGE('',*,*,#10664,.T.);
#14301=ORIENTED_EDGE('',*,*,#10662,.T.);
#14302=ORIENTED_EDGE('',*,*,#10679,.F.);
#14303=ORIENTED_EDGE('',*,*,#10680,.F.);
#14304=ORIENTED_EDGE('',*,*,#10681,.T.);
#14305=ORIENTED_EDGE('',*,*,#10682,.T.);
#14306=ORIENTED_EDGE('',*,*,#10683,.T.);
#14307=ORIENTED_EDGE('',*,*,#10684,.T.);
#14308=ORIENTED_EDGE('',*,*,#10685,.T.);
#14309=ORIENTED_EDGE('',*,*,#10686,.T.);
#14310=ORIENTED_EDGE('',*,*,#10404,.T.);
#14311=ORIENTED_EDGE('',*,*,#10687,.F.);
#14312=ORIENTED_EDGE('',*,*,#10688,.F.);
#14313=ORIENTED_EDGE('',*,*,#10661,.T.);
#14314=ORIENTED_EDGE('',*,*,#10657,.T.);
#14315=ORIENTED_EDGE('',*,*,#10654,.T.);
#14316=ORIENTED_EDGE('',*,*,#10689,.F.);
#14317=ORIENTED_EDGE('',*,*,#10690,.F.);
#14318=ORIENTED_EDGE('',*,*,#10691,.T.);
#14319=ORIENTED_EDGE('',*,*,#10692,.T.);
#14320=ORIENTED_EDGE('',*,*,#10693,.T.);
#14321=ORIENTED_EDGE('',*,*,#10694,.T.);
#14322=ORIENTED_EDGE('',*,*,#10695,.T.);
#14323=ORIENTED_EDGE('',*,*,#10696,.T.);
#14324=ORIENTED_EDGE('',*,*,#10697,.T.);
#14325=ORIENTED_EDGE('',*,*,#10698,.F.);
#14326=ORIENTED_EDGE('',*,*,#10699,.F.);
#14327=ORIENTED_EDGE('',*,*,#10651,.T.);
#14328=ORIENTED_EDGE('',*,*,#10648,.T.);
#14329=ORIENTED_EDGE('',*,*,#10645,.T.);
#14330=ORIENTED_EDGE('',*,*,#10700,.F.);
#14331=ORIENTED_EDGE('',*,*,#10701,.F.);
#14332=ORIENTED_EDGE('',*,*,#10702,.T.);
#14333=ORIENTED_EDGE('',*,*,#10703,.T.);
#14334=ORIENTED_EDGE('',*,*,#10704,.T.);
#14335=ORIENTED_EDGE('',*,*,#10705,.T.);
#14336=ORIENTED_EDGE('',*,*,#10706,.T.);
#14337=ORIENTED_EDGE('',*,*,#10707,.T.);
#14338=ORIENTED_EDGE('',*,*,#10708,.T.);
#14339=ORIENTED_EDGE('',*,*,#10709,.F.);
#14340=ORIENTED_EDGE('',*,*,#10710,.F.);
#14341=ORIENTED_EDGE('',*,*,#10675,.T.);
#14342=ORIENTED_EDGE('',*,*,#10671,.T.);
#14343=ORIENTED_EDGE('',*,*,#10668,.T.);
#14344=ORIENTED_EDGE('',*,*,#10711,.T.);
#14345=ORIENTED_EDGE('',*,*,#10712,.F.);
#14346=ORIENTED_EDGE('',*,*,#10713,.T.);
#14347=ORIENTED_EDGE('',*,*,#10714,.T.);
#14348=ORIENTED_EDGE('',*,*,#10715,.T.);
#14349=ORIENTED_EDGE('',*,*,#10716,.T.);
#14350=ORIENTED_EDGE('',*,*,#10717,.T.);
#14351=ORIENTED_EDGE('',*,*,#10718,.T.);
#14352=ORIENTED_EDGE('',*,*,#10603,.T.);
#14353=ORIENTED_EDGE('',*,*,#10577,.T.);
#14354=ORIENTED_EDGE('',*,*,#10579,.T.);
#14355=ORIENTED_EDGE('',*,*,#10581,.T.);
#14356=ORIENTED_EDGE('',*,*,#10583,.T.);
#14357=ORIENTED_EDGE('',*,*,#10585,.T.);
#14358=ORIENTED_EDGE('',*,*,#10587,.T.);
#14359=ORIENTED_EDGE('',*,*,#10589,.T.);
#14360=ORIENTED_EDGE('',*,*,#10591,.T.);
#14361=ORIENTED_EDGE('',*,*,#10593,.T.);
#14362=ORIENTED_EDGE('',*,*,#10595,.T.);
#14363=ORIENTED_EDGE('',*,*,#10596,.T.);
#14364=ORIENTED_EDGE('',*,*,#10390,.T.);
#14365=ORIENTED_EDGE('',*,*,#10598,.T.);
#14366=ORIENTED_EDGE('',*,*,#10600,.T.);
#14367=ORIENTED_EDGE('',*,*,#10602,.T.);
#14368=ORIENTED_EDGE('',*,*,#10383,.T.);
#14369=ORIENTED_EDGE('',*,*,#10384,.F.);
#14370=ORIENTED_EDGE('',*,*,#10379,.F.);
#14371=ORIENTED_EDGE('',*,*,#10614,.T.);
#14372=ORIENTED_EDGE('',*,*,#10615,.T.);
#14373=ORIENTED_EDGE('',*,*,#10606,.T.);
#14374=ORIENTED_EDGE('',*,*,#10608,.T.);
#14375=ORIENTED_EDGE('',*,*,#10610,.T.);
#14376=ORIENTED_EDGE('',*,*,#10612,.T.);
#14377=ORIENTED_EDGE('',*,*,#10376,.F.);
#14378=ORIENTED_EDGE('',*,*,#10626,.T.);
#14379=ORIENTED_EDGE('',*,*,#10627,.T.);
#14380=ORIENTED_EDGE('',*,*,#10618,.T.);
#14381=ORIENTED_EDGE('',*,*,#10620,.T.);
#14382=ORIENTED_EDGE('',*,*,#10622,.T.);
#14383=ORIENTED_EDGE('',*,*,#10624,.T.);
#14384=ORIENTED_EDGE('',*,*,#10719,.T.);
#14385=ORIENTED_EDGE('',*,*,#10720,.F.);
#14386=ORIENTED_EDGE('',*,*,#10638,.T.);
#14387=ORIENTED_EDGE('',*,*,#10721,.F.);
#14388=ORIENTED_EDGE('',*,*,#10722,.T.);
#14389=ORIENTED_EDGE('',*,*,#10723,.F.);
#14390=ORIENTED_EDGE('',*,*,#10632,.T.);
#14391=ORIENTED_EDGE('',*,*,#10487,.T.);
#14392=ORIENTED_EDGE('',*,*,#10628,.T.);
#14393=ORIENTED_EDGE('',*,*,#10538,.T.);
#14394=ORIENTED_EDGE('',*,*,#10639,.T.);
#14395=ORIENTED_EDGE('',*,*,#10720,.T.);
#14396=ORIENTED_EDGE('',*,*,#10724,.T.);
#14397=ORIENTED_EDGE('',*,*,#10725,.F.);
#14398=ORIENTED_EDGE('',*,*,#10630,.T.);
#14399=ORIENTED_EDGE('',*,*,#10723,.T.);
#14400=ORIENTED_EDGE('',*,*,#10726,.T.);
#14401=ORIENTED_EDGE('',*,*,#10727,.F.);
#14402=ORIENTED_EDGE('',*,*,#10634,.T.);
#14403=ORIENTED_EDGE('',*,*,#10519,.T.);
#14404=ORIENTED_EDGE('',*,*,#10629,.T.);
#14405=ORIENTED_EDGE('',*,*,#10497,.T.);
#14406=ORIENTED_EDGE('',*,*,#10631,.T.);
#14407=ORIENTED_EDGE('',*,*,#10725,.T.);
#14408=ORIENTED_EDGE('',*,*,#10728,.T.);
#14409=ORIENTED_EDGE('',*,*,#10729,.F.);
#14410=ORIENTED_EDGE('',*,*,#10635,.T.);
#14411=ORIENTED_EDGE('',*,*,#10727,.T.);
#14412=ORIENTED_EDGE('',*,*,#10730,.T.);
#14413=ORIENTED_EDGE('',*,*,#10731,.F.);
#14414=ORIENTED_EDGE('',*,*,#10641,.T.);
#14415=ORIENTED_EDGE('',*,*,#10572,.T.);
#14416=ORIENTED_EDGE('',*,*,#10633,.T.);
#14417=ORIENTED_EDGE('',*,*,#10514,.T.);
#14418=ORIENTED_EDGE('',*,*,#10636,.T.);
#14419=ORIENTED_EDGE('',*,*,#10729,.T.);
#14420=ORIENTED_EDGE('',*,*,#10732,.T.);
#14421=ORIENTED_EDGE('',*,*,#10733,.F.);
#14422=ORIENTED_EDGE('',*,*,#10642,.T.);
#14423=ORIENTED_EDGE('',*,*,#10731,.T.);
#14424=ORIENTED_EDGE('',*,*,#10734,.T.);
#14425=ORIENTED_EDGE('',*,*,#10721,.T.);
#14426=ORIENTED_EDGE('',*,*,#10637,.T.);
#14427=ORIENTED_EDGE('',*,*,#10543,.T.);
#14428=ORIENTED_EDGE('',*,*,#10640,.T.);
#14429=ORIENTED_EDGE('',*,*,#10568,.T.);
#14430=ORIENTED_EDGE('',*,*,#10643,.T.);
#14431=ORIENTED_EDGE('',*,*,#10733,.T.);
#14432=ORIENTED_EDGE('',*,*,#10735,.F.);
#14433=ORIENTED_EDGE('',*,*,#10422,.T.);
#14434=ORIENTED_EDGE('',*,*,#10736,.F.);
#14435=ORIENTED_EDGE('',*,*,#10700,.T.);
#14436=ORIENTED_EDGE('',*,*,#10644,.T.);
#14437=ORIENTED_EDGE('',*,*,#10647,.T.);
#14438=ORIENTED_EDGE('',*,*,#10650,.T.);
#14439=ORIENTED_EDGE('',*,*,#10653,.T.);
#14440=ORIENTED_EDGE('',*,*,#10737,.F.);
#14441=ORIENTED_EDGE('',*,*,#10738,.F.);
#14442=ORIENTED_EDGE('',*,*,#10735,.T.);
#14443=ORIENTED_EDGE('',*,*,#10739,.F.);
#14444=ORIENTED_EDGE('',*,*,#10420,.T.);
#14445=ORIENTED_EDGE('',*,*,#10737,.T.);
#14446=ORIENTED_EDGE('',*,*,#10652,.T.);
#14447=ORIENTED_EDGE('',*,*,#10699,.T.);
#14448=ORIENTED_EDGE('',*,*,#10739,.T.);
#14449=ORIENTED_EDGE('',*,*,#10698,.T.);
#14450=ORIENTED_EDGE('',*,*,#10740,.T.);
#14451=ORIENTED_EDGE('',*,*,#10741,.F.);
#14452=ORIENTED_EDGE('',*,*,#10742,.F.);
#14453=ORIENTED_EDGE('',*,*,#10743,.T.);
#14454=ORIENTED_EDGE('',*,*,#10744,.F.);
#14455=ORIENTED_EDGE('',*,*,#10740,.F.);
#14456=ORIENTED_EDGE('',*,*,#10697,.F.);
#14457=ORIENTED_EDGE('',*,*,#10745,.T.);
#14458=ORIENTED_EDGE('',*,*,#10746,.F.);
#14459=ORIENTED_EDGE('',*,*,#10743,.F.);
#14460=ORIENTED_EDGE('',*,*,#10696,.F.);
#14461=ORIENTED_EDGE('',*,*,#10747,.T.);
#14462=ORIENTED_EDGE('',*,*,#10748,.F.);
#14463=ORIENTED_EDGE('',*,*,#10745,.F.);
#14464=ORIENTED_EDGE('',*,*,#10749,.F.);
#14465=ORIENTED_EDGE('',*,*,#10750,.T.);
#14466=ORIENTED_EDGE('',*,*,#10695,.F.);
#14467=ORIENTED_EDGE('',*,*,#10751,.T.);
#14468=ORIENTED_EDGE('',*,*,#10752,.F.);
#14469=ORIENTED_EDGE('',*,*,#10750,.F.);
#14470=ORIENTED_EDGE('',*,*,#10753,.F.);
#14471=ORIENTED_EDGE('',*,*,#10747,.F.);
#14472=ORIENTED_EDGE('',*,*,#10694,.F.);
#14473=ORIENTED_EDGE('',*,*,#10754,.T.);
#14474=ORIENTED_EDGE('',*,*,#10755,.F.);
#14475=ORIENTED_EDGE('',*,*,#10751,.F.);
#14476=ORIENTED_EDGE('',*,*,#10756,.F.);
#14477=ORIENTED_EDGE('',*,*,#10757,.T.);
#14478=ORIENTED_EDGE('',*,*,#10693,.F.);
#14479=ORIENTED_EDGE('',*,*,#10758,.T.);
#14480=ORIENTED_EDGE('',*,*,#10759,.F.);
#14481=ORIENTED_EDGE('',*,*,#10757,.F.);
#14482=ORIENTED_EDGE('',*,*,#10760,.F.);
#14483=ORIENTED_EDGE('',*,*,#10754,.F.);
#14484=ORIENTED_EDGE('',*,*,#10692,.F.);
#14485=ORIENTED_EDGE('',*,*,#10761,.T.);
#14486=ORIENTED_EDGE('',*,*,#10762,.F.);
#14487=ORIENTED_EDGE('',*,*,#10758,.F.);
#14488=ORIENTED_EDGE('',*,*,#10763,.F.);
#14489=ORIENTED_EDGE('',*,*,#10764,.T.);
#14490=ORIENTED_EDGE('',*,*,#10691,.F.);
#14491=ORIENTED_EDGE('',*,*,#10765,.F.);
#14492=ORIENTED_EDGE('',*,*,#10766,.F.);
#14493=ORIENTED_EDGE('',*,*,#10764,.F.);
#14494=ORIENTED_EDGE('',*,*,#10767,.F.);
#14495=ORIENTED_EDGE('',*,*,#10761,.F.);
#14496=ORIENTED_EDGE('',*,*,#10417,.F.);
#14497=ORIENTED_EDGE('',*,*,#10768,.F.);
#14498=ORIENTED_EDGE('',*,*,#10765,.T.);
#14499=ORIENTED_EDGE('',*,*,#10690,.T.);
#14500=ORIENTED_EDGE('',*,*,#10689,.T.);
#14501=ORIENTED_EDGE('',*,*,#10418,.T.);
#14502=ORIENTED_EDGE('',*,*,#10656,.T.);
#14503=ORIENTED_EDGE('',*,*,#10659,.T.);
#14504=ORIENTED_EDGE('',*,*,#10660,.T.);
#14505=ORIENTED_EDGE('',*,*,#10411,.F.);
#14506=ORIENTED_EDGE('',*,*,#10769,.F.);
#14507=ORIENTED_EDGE('',*,*,#10416,.T.);
#14508=ORIENTED_EDGE('',*,*,#10688,.T.);
#14509=ORIENTED_EDGE('',*,*,#10413,.T.);
#14510=ORIENTED_EDGE('',*,*,#10362,.F.);
#14511=ORIENTED_EDGE('',*,*,#10770,.T.);
#14512=ORIENTED_EDGE('',*,*,#10397,.F.);
#14513=ORIENTED_EDGE('',*,*,#10364,.F.);
#14514=ORIENTED_EDGE('',*,*,#10771,.T.);
#14515=ORIENTED_EDGE('',*,*,#10401,.T.);
#14516=ORIENTED_EDGE('',*,*,#10772,.T.);
#14517=ORIENTED_EDGE('',*,*,#10680,.T.);
#14518=ORIENTED_EDGE('',*,*,#10410,.T.);
#14519=ORIENTED_EDGE('',*,*,#10687,.T.);
#14520=ORIENTED_EDGE('',*,*,#10403,.T.);
#14521=ORIENTED_EDGE('',*,*,#10773,.T.);
#14522=ORIENTED_EDGE('',*,*,#10407,.T.);
#14523=ORIENTED_EDGE('',*,*,#10368,.F.);
#14524=ORIENTED_EDGE('',*,*,#10370,.F.);
#14525=ORIENTED_EDGE('',*,*,#10406,.T.);
#14526=ORIENTED_EDGE('',*,*,#10773,.F.);
#14527=ORIENTED_EDGE('',*,*,#10402,.T.);
#14528=ORIENTED_EDGE('',*,*,#10686,.F.);
#14529=ORIENTED_EDGE('',*,*,#10774,.T.);
#14530=ORIENTED_EDGE('',*,*,#10372,.F.);
#14531=ORIENTED_EDGE('',*,*,#10405,.F.);
#14532=ORIENTED_EDGE('',*,*,#10374,.F.);
#14533=ORIENTED_EDGE('',*,*,#10775,.T.);
#14534=ORIENTED_EDGE('',*,*,#10685,.F.);
#14535=ORIENTED_EDGE('',*,*,#10776,.T.);
#14536=ORIENTED_EDGE('',*,*,#10375,.F.);
#14537=ORIENTED_EDGE('',*,*,#10775,.F.);
#14538=ORIENTED_EDGE('',*,*,#10373,.F.);
#14539=ORIENTED_EDGE('',*,*,#10774,.F.);
#14540=ORIENTED_EDGE('',*,*,#10684,.F.);
#14541=ORIENTED_EDGE('',*,*,#10777,.T.);
#14542=ORIENTED_EDGE('',*,*,#10356,.F.);
#14543=ORIENTED_EDGE('',*,*,#10776,.F.);
#14544=ORIENTED_EDGE('',*,*,#10358,.F.);
#14545=ORIENTED_EDGE('',*,*,#10778,.T.);
#14546=ORIENTED_EDGE('',*,*,#10683,.F.);
#14547=ORIENTED_EDGE('',*,*,#10779,.T.);
#14548=ORIENTED_EDGE('',*,*,#10359,.F.);
#14549=ORIENTED_EDGE('',*,*,#10778,.F.);
#14550=ORIENTED_EDGE('',*,*,#10357,.F.);
#14551=ORIENTED_EDGE('',*,*,#10777,.F.);
#14552=ORIENTED_EDGE('',*,*,#10682,.F.);
#14553=ORIENTED_EDGE('',*,*,#10780,.T.);
#14554=ORIENTED_EDGE('',*,*,#10360,.F.);
#14555=ORIENTED_EDGE('',*,*,#10779,.F.);
#14556=ORIENTED_EDGE('',*,*,#10772,.F.);
#14557=ORIENTED_EDGE('',*,*,#10400,.T.);
#14558=ORIENTED_EDGE('',*,*,#10771,.F.);
#14559=ORIENTED_EDGE('',*,*,#10363,.F.);
#14560=ORIENTED_EDGE('',*,*,#10770,.F.);
#14561=ORIENTED_EDGE('',*,*,#10361,.F.);
#14562=ORIENTED_EDGE('',*,*,#10780,.F.);
#14563=ORIENTED_EDGE('',*,*,#10681,.F.);
#14564=ORIENTED_EDGE('',*,*,#10679,.T.);
#14565=ORIENTED_EDGE('',*,*,#10398,.T.);
#14566=ORIENTED_EDGE('',*,*,#10126,.T.);
#14567=ORIENTED_EDGE('',*,*,#10781,.F.);
#14568=ORIENTED_EDGE('',*,*,#10121,.T.);
#14569=ORIENTED_EDGE('',*,*,#10782,.F.);
#14570=ORIENTED_EDGE('',*,*,#10125,.T.);
#14571=ORIENTED_EDGE('',*,*,#10678,.T.);
#14572=ORIENTED_EDGE('',*,*,#10783,.T.);
#14573=ORIENTED_EDGE('',*,*,#10784,.F.);
#14574=ORIENTED_EDGE('',*,*,#10785,.F.);
#14575=ORIENTED_EDGE('',*,*,#10786,.T.);
#14576=ORIENTED_EDGE('',*,*,#10786,.F.);
#14577=ORIENTED_EDGE('',*,*,#10787,.F.);
#14578=ORIENTED_EDGE('',*,*,#10783,.F.);
#14579=ORIENTED_EDGE('',*,*,#10677,.F.);
#14580=ORIENTED_EDGE('',*,*,#10788,.T.);
#14581=ORIENTED_EDGE('',*,*,#10789,.F.);
#14582=ORIENTED_EDGE('',*,*,#10718,.F.);
#14583=ORIENTED_EDGE('',*,*,#10790,.T.);
#14584=ORIENTED_EDGE('',*,*,#10791,.F.);
#14585=ORIENTED_EDGE('',*,*,#10788,.F.);
#14586=ORIENTED_EDGE('',*,*,#10792,.F.);
#14587=ORIENTED_EDGE('',*,*,#10793,.T.);
#14588=ORIENTED_EDGE('',*,*,#10717,.F.);
#14589=ORIENTED_EDGE('',*,*,#10794,.T.);
#14590=ORIENTED_EDGE('',*,*,#10795,.F.);
#14591=ORIENTED_EDGE('',*,*,#10793,.F.);
#14592=ORIENTED_EDGE('',*,*,#10796,.F.);
#14593=ORIENTED_EDGE('',*,*,#10790,.F.);
#14594=ORIENTED_EDGE('',*,*,#10716,.F.);
#14595=ORIENTED_EDGE('',*,*,#10797,.T.);
#14596=ORIENTED_EDGE('',*,*,#10798,.F.);
#14597=ORIENTED_EDGE('',*,*,#10794,.F.);
#14598=ORIENTED_EDGE('',*,*,#10799,.F.);
#14599=ORIENTED_EDGE('',*,*,#10800,.T.);
#14600=ORIENTED_EDGE('',*,*,#10715,.F.);
#14601=ORIENTED_EDGE('',*,*,#10801,.T.);
#14602=ORIENTED_EDGE('',*,*,#10802,.F.);
#14603=ORIENTED_EDGE('',*,*,#10800,.F.);
#14604=ORIENTED_EDGE('',*,*,#10803,.F.);
#14605=ORIENTED_EDGE('',*,*,#10797,.F.);
#14606=ORIENTED_EDGE('',*,*,#10714,.F.);
#14607=ORIENTED_EDGE('',*,*,#10804,.T.);
#14608=ORIENTED_EDGE('',*,*,#10805,.F.);
#14609=ORIENTED_EDGE('',*,*,#10801,.F.);
#14610=ORIENTED_EDGE('',*,*,#10806,.F.);
#14611=ORIENTED_EDGE('',*,*,#10807,.T.);
#14612=ORIENTED_EDGE('',*,*,#10713,.F.);
#14613=ORIENTED_EDGE('',*,*,#10808,.F.);
#14614=ORIENTED_EDGE('',*,*,#10809,.F.);
#14615=ORIENTED_EDGE('',*,*,#10807,.F.);
#14616=ORIENTED_EDGE('',*,*,#10810,.F.);
#14617=ORIENTED_EDGE('',*,*,#10804,.F.);
#14618=ORIENTED_EDGE('',*,*,#10811,.T.);
#14619=ORIENTED_EDGE('',*,*,#10812,.F.);
#14620=ORIENTED_EDGE('',*,*,#10808,.T.);
#14621=ORIENTED_EDGE('',*,*,#10712,.T.);
#14622=ORIENTED_EDGE('',*,*,#10813,.F.);
#14623=ORIENTED_EDGE('',*,*,#10814,.F.);
#14624=ORIENTED_EDGE('',*,*,#10811,.F.);
#14625=ORIENTED_EDGE('',*,*,#10711,.F.);
#14626=ORIENTED_EDGE('',*,*,#10667,.F.);
#14627=ORIENTED_EDGE('',*,*,#10670,.T.);
#14628=ORIENTED_EDGE('',*,*,#10673,.T.);
#14629=ORIENTED_EDGE('',*,*,#10674,.T.);
#14630=ORIENTED_EDGE('',*,*,#10815,.F.);
#14631=ORIENTED_EDGE('',*,*,#10816,.F.);
#14632=ORIENTED_EDGE('',*,*,#10813,.T.);
#14633=ORIENTED_EDGE('',*,*,#10817,.F.);
#14634=ORIENTED_EDGE('',*,*,#10393,.T.);
#14635=ORIENTED_EDGE('',*,*,#10818,.F.);
#14636=ORIENTED_EDGE('',*,*,#10815,.T.);
#14637=ORIENTED_EDGE('',*,*,#10676,.T.);
#14638=ORIENTED_EDGE('',*,*,#10710,.T.);
#14639=ORIENTED_EDGE('',*,*,#10819,.F.);
#14640=ORIENTED_EDGE('',*,*,#10820,.T.);
#14641=ORIENTED_EDGE('',*,*,#10736,.T.);
#14642=ORIENTED_EDGE('',*,*,#10821,.F.);
#14643=ORIENTED_EDGE('',*,*,#10822,.T.);
#14644=ORIENTED_EDGE('',*,*,#10701,.T.);
#14645=ORIENTED_EDGE('',*,*,#10817,.T.);
#14646=ORIENTED_EDGE('',*,*,#10709,.T.);
#14647=ORIENTED_EDGE('',*,*,#10823,.T.);
#14648=ORIENTED_EDGE('',*,*,#10824,.F.);
#14649=ORIENTED_EDGE('',*,*,#10825,.F.);
#14650=ORIENTED_EDGE('',*,*,#10826,.T.);
#14651=ORIENTED_EDGE('',*,*,#10827,.F.);
#14652=ORIENTED_EDGE('',*,*,#10823,.F.);
#14653=ORIENTED_EDGE('',*,*,#10708,.F.);
#14654=ORIENTED_EDGE('',*,*,#10828,.T.);
#14655=ORIENTED_EDGE('',*,*,#10829,.F.);
#14656=ORIENTED_EDGE('',*,*,#10826,.F.);
#14657=ORIENTED_EDGE('',*,*,#10707,.F.);
#14658=ORIENTED_EDGE('',*,*,#10830,.T.);
#14659=ORIENTED_EDGE('',*,*,#10831,.F.);
#14660=ORIENTED_EDGE('',*,*,#10828,.F.);
#14661=ORIENTED_EDGE('',*,*,#10832,.F.);
#14662=ORIENTED_EDGE('',*,*,#10833,.T.);
#14663=ORIENTED_EDGE('',*,*,#10706,.F.);
#14664=ORIENTED_EDGE('',*,*,#10834,.T.);
#14665=ORIENTED_EDGE('',*,*,#10835,.F.);
#14666=ORIENTED_EDGE('',*,*,#10833,.F.);
#14667=ORIENTED_EDGE('',*,*,#10836,.F.);
#14668=ORIENTED_EDGE('',*,*,#10830,.F.);
#14669=ORIENTED_EDGE('',*,*,#10705,.F.);
#14670=ORIENTED_EDGE('',*,*,#10837,.T.);
#14671=ORIENTED_EDGE('',*,*,#10838,.F.);
#14672=ORIENTED_EDGE('',*,*,#10834,.F.);
#14673=ORIENTED_EDGE('',*,*,#10839,.F.);
#14674=ORIENTED_EDGE('',*,*,#10840,.T.);
#14675=ORIENTED_EDGE('',*,*,#10704,.F.);
#14676=ORIENTED_EDGE('',*,*,#10841,.T.);
#14677=ORIENTED_EDGE('',*,*,#10842,.F.);
#14678=ORIENTED_EDGE('',*,*,#10840,.F.);
#14679=ORIENTED_EDGE('',*,*,#10843,.F.);
#14680=ORIENTED_EDGE('',*,*,#10837,.F.);
#14681=ORIENTED_EDGE('',*,*,#10703,.F.);
#14682=ORIENTED_EDGE('',*,*,#10844,.T.);
#14683=ORIENTED_EDGE('',*,*,#10845,.F.);
#14684=ORIENTED_EDGE('',*,*,#10841,.F.);
#14685=ORIENTED_EDGE('',*,*,#10702,.F.);
#14686=ORIENTED_EDGE('',*,*,#10822,.F.);
#14687=ORIENTED_EDGE('',*,*,#10846,.F.);
#14688=ORIENTED_EDGE('',*,*,#10820,.F.);
#14689=ORIENTED_EDGE('',*,*,#10847,.F.);
#14690=ORIENTED_EDGE('',*,*,#10844,.F.);
#14691=ORIENTED_EDGE('',*,*,#10732,.F.);
#14692=ORIENTED_EDGE('',*,*,#10730,.F.);
#14693=ORIENTED_EDGE('',*,*,#10728,.F.);
#14694=ORIENTED_EDGE('',*,*,#10726,.F.);
#14695=ORIENTED_EDGE('',*,*,#10724,.F.);
#14696=ORIENTED_EDGE('',*,*,#10722,.F.);
#14697=ORIENTED_EDGE('',*,*,#10719,.F.);
#14698=ORIENTED_EDGE('',*,*,#10734,.F.);
#14699=ORIENTED_EDGE('',*,*,#10848,.F.);
#14700=ORIENTED_EDGE('',*,*,#10849,.F.);
#14701=ORIENTED_EDGE('',*,*,#10850,.F.);
#14702=ORIENTED_EDGE('',*,*,#10851,.F.);
#14703=ORIENTED_EDGE('',*,*,#10852,.F.);
#14704=ORIENTED_EDGE('',*,*,#10853,.F.);
#14705=ORIENTED_EDGE('',*,*,#10854,.F.);
#14706=ORIENTED_EDGE('',*,*,#10855,.F.);
#14707=ORIENTED_EDGE('',*,*,#10856,.F.);
#14708=ORIENTED_EDGE('',*,*,#10857,.F.);
#14709=ORIENTED_EDGE('',*,*,#10423,.T.);
#14710=ORIENTED_EDGE('',*,*,#10858,.F.);
#14711=ORIENTED_EDGE('',*,*,#10859,.F.);
#14712=ORIENTED_EDGE('',*,*,#10858,.T.);
#14713=ORIENTED_EDGE('',*,*,#10738,.T.);
#14714=ORIENTED_EDGE('',*,*,#10860,.F.);
#14715=ORIENTED_EDGE('',*,*,#10861,.F.);
#14716=ORIENTED_EDGE('',*,*,#10860,.T.);
#14717=ORIENTED_EDGE('',*,*,#10421,.T.);
#14718=ORIENTED_EDGE('',*,*,#10862,.F.);
#14719=ORIENTED_EDGE('',*,*,#10863,.F.);
#14720=ORIENTED_EDGE('',*,*,#10864,.F.);
#14721=ORIENTED_EDGE('',*,*,#10862,.T.);
#14722=ORIENTED_EDGE('',*,*,#10741,.T.);
#14723=ORIENTED_EDGE('',*,*,#10744,.T.);
#14724=ORIENTED_EDGE('',*,*,#10742,.T.);
#14725=ORIENTED_EDGE('',*,*,#10746,.T.);
#14726=ORIENTED_EDGE('',*,*,#10748,.T.);
#14727=ORIENTED_EDGE('',*,*,#10753,.T.);
#14728=ORIENTED_EDGE('',*,*,#10749,.T.);
#14729=ORIENTED_EDGE('',*,*,#10752,.T.);
#14730=ORIENTED_EDGE('',*,*,#10755,.T.);
#14731=ORIENTED_EDGE('',*,*,#10760,.T.);
#14732=ORIENTED_EDGE('',*,*,#10756,.T.);
#14733=ORIENTED_EDGE('',*,*,#10759,.T.);
#14734=ORIENTED_EDGE('',*,*,#10762,.T.);
#14735=ORIENTED_EDGE('',*,*,#10767,.T.);
#14736=ORIENTED_EDGE('',*,*,#10763,.T.);
#14737=ORIENTED_EDGE('',*,*,#10766,.T.);
#14738=ORIENTED_EDGE('',*,*,#10768,.T.);
#14739=ORIENTED_EDGE('',*,*,#10865,.F.);
#14740=ORIENTED_EDGE('',*,*,#10863,.T.);
#14741=ORIENTED_EDGE('',*,*,#10415,.T.);
#14742=ORIENTED_EDGE('',*,*,#10866,.F.);
#14743=ORIENTED_EDGE('',*,*,#10867,.F.);
#14744=ORIENTED_EDGE('',*,*,#10866,.T.);
#14745=ORIENTED_EDGE('',*,*,#10769,.T.);
#14746=ORIENTED_EDGE('',*,*,#10868,.F.);
#14747=ORIENTED_EDGE('',*,*,#10869,.F.);
#14748=ORIENTED_EDGE('',*,*,#10868,.T.);
#14749=ORIENTED_EDGE('',*,*,#10409,.T.);
#14750=ORIENTED_EDGE('',*,*,#10367,.F.);
#14751=ORIENTED_EDGE('',*,*,#10870,.F.);
#14752=ORIENTED_EDGE('',*,*,#10365,.T.);
#14753=ORIENTED_EDGE('',*,*,#10396,.T.);
#14754=ORIENTED_EDGE('',*,*,#10871,.F.);
#14755=ORIENTED_EDGE('',*,*,#10872,.F.);
#14756=ORIENTED_EDGE('',*,*,#10871,.T.);
#14757=ORIENTED_EDGE('',*,*,#10781,.T.);
#14758=ORIENTED_EDGE('',*,*,#10873,.F.);
#14759=ORIENTED_EDGE('',*,*,#10874,.F.);
#14760=ORIENTED_EDGE('',*,*,#10873,.T.);
#14761=ORIENTED_EDGE('',*,*,#10782,.T.);
#14762=ORIENTED_EDGE('',*,*,#10875,.F.);
#14763=ORIENTED_EDGE('',*,*,#10876,.F.);
#14764=ORIENTED_EDGE('',*,*,#10877,.F.);
#14765=ORIENTED_EDGE('',*,*,#10875,.T.);
#14766=ORIENTED_EDGE('',*,*,#10784,.T.);
#14767=ORIENTED_EDGE('',*,*,#10787,.T.);
#14768=ORIENTED_EDGE('',*,*,#10785,.T.);
#14769=ORIENTED_EDGE('',*,*,#10789,.T.);
#14770=ORIENTED_EDGE('',*,*,#10791,.T.);
#14771=ORIENTED_EDGE('',*,*,#10796,.T.);
#14772=ORIENTED_EDGE('',*,*,#10792,.T.);
#14773=ORIENTED_EDGE('',*,*,#10795,.T.);
#14774=ORIENTED_EDGE('',*,*,#10798,.T.);
#14775=ORIENTED_EDGE('',*,*,#10803,.T.);
#14776=ORIENTED_EDGE('',*,*,#10799,.T.);
#14777=ORIENTED_EDGE('',*,*,#10802,.T.);
#14778=ORIENTED_EDGE('',*,*,#10805,.T.);
#14779=ORIENTED_EDGE('',*,*,#10810,.T.);
#14780=ORIENTED_EDGE('',*,*,#10806,.T.);
#14781=ORIENTED_EDGE('',*,*,#10809,.T.);
#14782=ORIENTED_EDGE('',*,*,#10812,.T.);
#14783=ORIENTED_EDGE('',*,*,#10878,.F.);
#14784=ORIENTED_EDGE('',*,*,#10876,.T.);
#14785=ORIENTED_EDGE('',*,*,#10814,.T.);
#14786=ORIENTED_EDGE('',*,*,#10879,.F.);
#14787=ORIENTED_EDGE('',*,*,#10880,.F.);
#14788=ORIENTED_EDGE('',*,*,#10879,.T.);
#14789=ORIENTED_EDGE('',*,*,#10816,.T.);
#14790=ORIENTED_EDGE('',*,*,#10881,.F.);
#14791=ORIENTED_EDGE('',*,*,#10882,.F.);
#14792=ORIENTED_EDGE('',*,*,#10881,.T.);
#14793=ORIENTED_EDGE('',*,*,#10818,.T.);
#14794=ORIENTED_EDGE('',*,*,#10394,.T.);
#14795=ORIENTED_EDGE('',*,*,#10883,.F.);
#14796=ORIENTED_EDGE('',*,*,#10845,.T.);
#14797=ORIENTED_EDGE('',*,*,#10847,.T.);
#14798=ORIENTED_EDGE('',*,*,#10819,.T.);
#14799=ORIENTED_EDGE('',*,*,#10846,.T.);
#14800=ORIENTED_EDGE('',*,*,#10821,.T.);
#14801=ORIENTED_EDGE('',*,*,#10857,.T.);
#14802=ORIENTED_EDGE('',*,*,#10884,.F.);
#14803=ORIENTED_EDGE('',*,*,#10883,.T.);
#14804=ORIENTED_EDGE('',*,*,#10824,.T.);
#14805=ORIENTED_EDGE('',*,*,#10827,.T.);
#14806=ORIENTED_EDGE('',*,*,#10825,.T.);
#14807=ORIENTED_EDGE('',*,*,#10829,.T.);
#14808=ORIENTED_EDGE('',*,*,#10831,.T.);
#14809=ORIENTED_EDGE('',*,*,#10836,.T.);
#14810=ORIENTED_EDGE('',*,*,#10832,.T.);
#14811=ORIENTED_EDGE('',*,*,#10835,.T.);
#14812=ORIENTED_EDGE('',*,*,#10838,.T.);
#14813=ORIENTED_EDGE('',*,*,#10843,.T.);
#14814=ORIENTED_EDGE('',*,*,#10839,.T.);
#14815=ORIENTED_EDGE('',*,*,#10842,.T.);
#14816=ORIENTED_EDGE('',*,*,#10885,.F.);
#14817=ORIENTED_EDGE('',*,*,#10852,.T.);
#14818=ORIENTED_EDGE('',*,*,#10886,.F.);
#14819=ORIENTED_EDGE('',*,*,#10887,.F.);
#14820=ORIENTED_EDGE('',*,*,#10888,.F.);
#14821=ORIENTED_EDGE('',*,*,#10854,.T.);
#14822=ORIENTED_EDGE('',*,*,#10889,.F.);
#14823=ORIENTED_EDGE('',*,*,#10890,.F.);
#14824=ORIENTED_EDGE('',*,*,#10378,.T.);
#14825=ORIENTED_EDGE('',*,*,#10381,.T.);
#14826=ORIENTED_EDGE('',*,*,#10891,.F.);
#14827=ORIENTED_EDGE('',*,*,#10892,.T.);
#14828=ORIENTED_EDGE('',*,*,#10893,.F.);
#14829=ORIENTED_EDGE('',*,*,#10889,.T.);
#14830=ORIENTED_EDGE('',*,*,#10853,.T.);
#14831=ORIENTED_EDGE('',*,*,#10885,.T.);
#14832=ORIENTED_EDGE('',*,*,#10894,.F.);
#14833=ORIENTED_EDGE('',*,*,#10848,.T.);
#14834=ORIENTED_EDGE('',*,*,#10895,.F.);
#14835=ORIENTED_EDGE('',*,*,#10896,.F.);
#14836=ORIENTED_EDGE('',*,*,#10855,.T.);
#14837=ORIENTED_EDGE('',*,*,#10888,.T.);
#14838=ORIENTED_EDGE('',*,*,#10897,.F.);
#14839=ORIENTED_EDGE('',*,*,#10898,.T.);
#14840=ORIENTED_EDGE('',*,*,#10899,.F.);
#14841=ORIENTED_EDGE('',*,*,#10895,.T.);
#14842=ORIENTED_EDGE('',*,*,#10900,.F.);
#14843=ORIENTED_EDGE('',*,*,#10901,.T.);
#14844=ORIENTED_EDGE('',*,*,#10902,.F.);
#14845=ORIENTED_EDGE('',*,*,#10903,.F.);
#14846=ORIENTED_EDGE('',*,*,#10849,.T.);
#14847=ORIENTED_EDGE('',*,*,#10894,.T.);
#14848=ORIENTED_EDGE('',*,*,#10851,.T.);
#14849=ORIENTED_EDGE('',*,*,#10904,.F.);
#14850=ORIENTED_EDGE('',*,*,#10905,.F.);
#14851=ORIENTED_EDGE('',*,*,#10906,.T.);
#14852=ORIENTED_EDGE('',*,*,#10907,.F.);
#14853=ORIENTED_EDGE('',*,*,#10886,.T.);
#14854=ORIENTED_EDGE('',*,*,#10904,.T.);
#14855=ORIENTED_EDGE('',*,*,#10850,.T.);
#14856=ORIENTED_EDGE('',*,*,#10903,.T.);
#14857=ORIENTED_EDGE('',*,*,#10908,.F.);
#14858=ORIENTED_EDGE('',*,*,#10909,.F.);
#14859=ORIENTED_EDGE('',*,*,#10910,.T.);
#14860=ORIENTED_EDGE('',*,*,#10911,.F.);
#14861=ORIENTED_EDGE('',*,*,#10912,.F.);
#14862=ORIENTED_EDGE('',*,*,#10913,.F.);
#14863=ORIENTED_EDGE('',*,*,#10914,.T.);
#14864=ORIENTED_EDGE('',*,*,#10915,.F.);
#14865=ORIENTED_EDGE('',*,*,#10910,.F.);
#14866=ORIENTED_EDGE('',*,*,#10914,.F.);
#14867=ORIENTED_EDGE('',*,*,#10916,.F.);
#14868=ORIENTED_EDGE('',*,*,#10917,.F.);
#14869=ORIENTED_EDGE('',*,*,#10918,.F.);
#14870=ORIENTED_EDGE('',*,*,#10919,.F.);
#14871=ORIENTED_EDGE('',*,*,#10920,.T.);
#14872=ORIENTED_EDGE('',*,*,#10921,.F.);
#14873=ORIENTED_EDGE('',*,*,#10922,.F.);
#14874=ORIENTED_EDGE('',*,*,#10923,.F.);
#14875=ORIENTED_EDGE('',*,*,#10924,.F.);
#14876=ORIENTED_EDGE('',*,*,#10919,.T.);
#14877=ORIENTED_EDGE('',*,*,#10925,.F.);
#14878=ORIENTED_EDGE('',*,*,#10926,.F.);
#14879=ORIENTED_EDGE('',*,*,#10927,.F.);
#14880=ORIENTED_EDGE('',*,*,#10928,.F.);
#14881=ORIENTED_EDGE('',*,*,#10923,.T.);
#14882=ORIENTED_EDGE('',*,*,#10929,.F.);
#14883=ORIENTED_EDGE('',*,*,#10930,.T.);
#14884=ORIENTED_EDGE('',*,*,#10931,.F.);
#14885=ORIENTED_EDGE('',*,*,#10932,.F.);
#14886=ORIENTED_EDGE('',*,*,#10933,.F.);
#14887=ORIENTED_EDGE('',*,*,#10934,.F.);
#14888=ORIENTED_EDGE('',*,*,#10929,.T.);
#14889=ORIENTED_EDGE('',*,*,#10935,.F.);
#14890=ORIENTED_EDGE('',*,*,#10936,.F.);
#14891=ORIENTED_EDGE('',*,*,#10937,.F.);
#14892=ORIENTED_EDGE('',*,*,#10938,.F.);
#14893=ORIENTED_EDGE('',*,*,#10933,.T.);
#14894=ORIENTED_EDGE('',*,*,#10939,.F.);
#14895=ORIENTED_EDGE('',*,*,#10940,.T.);
#14896=ORIENTED_EDGE('',*,*,#10941,.F.);
#14897=ORIENTED_EDGE('',*,*,#10942,.F.);
#14898=ORIENTED_EDGE('',*,*,#10943,.F.);
#14899=ORIENTED_EDGE('',*,*,#10944,.T.);
#14900=ORIENTED_EDGE('',*,*,#10945,.F.);
#14901=ORIENTED_EDGE('',*,*,#10940,.F.);
#14902=ORIENTED_EDGE('',*,*,#10944,.F.);
#14903=ORIENTED_EDGE('',*,*,#10946,.F.);
#14904=ORIENTED_EDGE('',*,*,#10947,.F.);
#14905=ORIENTED_EDGE('',*,*,#10948,.F.);
#14906=ORIENTED_EDGE('',*,*,#10346,.F.);
#14907=ORIENTED_EDGE('',*,*,#10949,.F.);
#14908=ORIENTED_EDGE('',*,*,#10926,.T.);
#14909=ORIENTED_EDGE('',*,*,#10925,.T.);
#14910=ORIENTED_EDGE('',*,*,#10922,.T.);
#14911=ORIENTED_EDGE('',*,*,#10950,.F.);
#14912=ORIENTED_EDGE('',*,*,#10951,.F.);
#14913=ORIENTED_EDGE('',*,*,#10952,.F.);
#14914=ORIENTED_EDGE('',*,*,#10916,.T.);
#14915=ORIENTED_EDGE('',*,*,#10913,.T.);
#14916=ORIENTED_EDGE('',*,*,#10909,.T.);
#14917=ORIENTED_EDGE('',*,*,#10953,.F.);
#14918=ORIENTED_EDGE('',*,*,#10954,.F.);
#14919=ORIENTED_EDGE('',*,*,#10955,.F.);
#14920=ORIENTED_EDGE('',*,*,#10946,.T.);
#14921=ORIENTED_EDGE('',*,*,#10943,.T.);
#14922=ORIENTED_EDGE('',*,*,#10939,.T.);
#14923=ORIENTED_EDGE('',*,*,#10956,.F.);
#14924=ORIENTED_EDGE('',*,*,#10957,.F.);
#14925=ORIENTED_EDGE('',*,*,#10958,.F.);
#14926=ORIENTED_EDGE('',*,*,#10936,.T.);
#14927=ORIENTED_EDGE('',*,*,#10935,.T.);
#14928=ORIENTED_EDGE('',*,*,#10932,.T.);
#14929=ORIENTED_EDGE('',*,*,#10959,.F.);
#14930=ORIENTED_EDGE('',*,*,#10882,.T.);
#14931=ORIENTED_EDGE('',*,*,#10884,.T.);
#14932=ORIENTED_EDGE('',*,*,#10856,.T.);
#14933=ORIENTED_EDGE('',*,*,#10859,.T.);
#14934=ORIENTED_EDGE('',*,*,#10861,.T.);
#14935=ORIENTED_EDGE('',*,*,#10864,.T.);
#14936=ORIENTED_EDGE('',*,*,#10865,.T.);
#14937=ORIENTED_EDGE('',*,*,#10867,.T.);
#14938=ORIENTED_EDGE('',*,*,#10869,.T.);
#14939=ORIENTED_EDGE('',*,*,#10366,.T.);
#14940=ORIENTED_EDGE('',*,*,#10870,.T.);
#14941=ORIENTED_EDGE('',*,*,#10872,.T.);
#14942=ORIENTED_EDGE('',*,*,#10874,.T.);
#14943=ORIENTED_EDGE('',*,*,#10877,.T.);
#14944=ORIENTED_EDGE('',*,*,#10878,.T.);
#14945=ORIENTED_EDGE('',*,*,#10880,.T.);
#14946=ORIENTED_EDGE('',*,*,#10960,.T.);
#14947=ORIENTED_EDGE('',*,*,#10961,.T.);
#14948=ORIENTED_EDGE('',*,*,#10962,.T.);
#14949=ORIENTED_EDGE('',*,*,#10963,.T.);
#14950=ORIENTED_EDGE('',*,*,#10964,.T.);
#14951=ORIENTED_EDGE('',*,*,#10965,.T.);
#14952=ORIENTED_EDGE('',*,*,#10966,.T.);
#14953=ORIENTED_EDGE('',*,*,#10967,.T.);
#14954=ORIENTED_EDGE('',*,*,#10968,.T.);
#14955=ORIENTED_EDGE('',*,*,#10969,.T.);
#14956=ORIENTED_EDGE('',*,*,#10970,.T.);
#14957=ORIENTED_EDGE('',*,*,#10971,.T.);
#14958=ORIENTED_EDGE('',*,*,#10891,.T.);
#14959=ORIENTED_EDGE('',*,*,#10887,.T.);
#14960=ORIENTED_EDGE('',*,*,#10907,.T.);
#14961=ORIENTED_EDGE('',*,*,#10972,.T.);
#14962=ORIENTED_EDGE('',*,*,#10893,.T.);
#14963=ORIENTED_EDGE('',*,*,#10973,.T.);
#14964=ORIENTED_EDGE('',*,*,#10897,.T.);
#14965=ORIENTED_EDGE('',*,*,#10890,.T.);
#14966=ORIENTED_EDGE('',*,*,#10899,.T.);
#14967=ORIENTED_EDGE('',*,*,#10974,.T.);
#14968=ORIENTED_EDGE('',*,*,#10900,.T.);
#14969=ORIENTED_EDGE('',*,*,#10896,.T.);
#14970=ORIENTED_EDGE('',*,*,#10905,.T.);
#14971=ORIENTED_EDGE('',*,*,#10908,.T.);
#14972=ORIENTED_EDGE('',*,*,#10902,.T.);
#14973=ORIENTED_EDGE('',*,*,#10975,.T.);
#14974=ORIENTED_EDGE('',*,*,#10976,.F.);
#14975=ORIENTED_EDGE('',*,*,#10977,.F.);
#14976=ORIENTED_EDGE('',*,*,#10953,.T.);
#14977=ORIENTED_EDGE('',*,*,#10978,.F.);
#14978=ORIENTED_EDGE('',*,*,#10979,.F.);
#14979=ORIENTED_EDGE('',*,*,#10980,.F.);
#14980=ORIENTED_EDGE('',*,*,#10978,.T.);
#14981=ORIENTED_EDGE('',*,*,#10912,.T.);
#14982=ORIENTED_EDGE('',*,*,#10981,.F.);
#14983=ORIENTED_EDGE('',*,*,#10982,.F.);
#14984=ORIENTED_EDGE('',*,*,#10979,.T.);
#14985=ORIENTED_EDGE('',*,*,#10911,.T.);
#14986=ORIENTED_EDGE('',*,*,#10915,.T.);
#14987=ORIENTED_EDGE('',*,*,#10918,.T.);
#14988=ORIENTED_EDGE('',*,*,#10983,.F.);
#14989=ORIENTED_EDGE('',*,*,#10984,.F.);
#14990=ORIENTED_EDGE('',*,*,#10981,.T.);
#14991=ORIENTED_EDGE('',*,*,#10917,.T.);
#14992=ORIENTED_EDGE('',*,*,#10985,.F.);
#14993=ORIENTED_EDGE('',*,*,#10983,.T.);
#14994=ORIENTED_EDGE('',*,*,#10952,.T.);
#14995=ORIENTED_EDGE('',*,*,#10986,.F.);
#14996=ORIENTED_EDGE('',*,*,#10987,.F.);
#14997=ORIENTED_EDGE('',*,*,#10988,.F.);
#14998=ORIENTED_EDGE('',*,*,#10986,.T.);
#14999=ORIENTED_EDGE('',*,*,#10951,.T.);
#15000=ORIENTED_EDGE('',*,*,#10989,.F.);
#15001=ORIENTED_EDGE('',*,*,#10987,.T.);
#15002=ORIENTED_EDGE('',*,*,#10950,.T.);
#15003=ORIENTED_EDGE('',*,*,#10990,.F.);
#15004=ORIENTED_EDGE('',*,*,#10991,.F.);
#15005=ORIENTED_EDGE('',*,*,#10992,.F.);
#15006=ORIENTED_EDGE('',*,*,#10990,.T.);
#15007=ORIENTED_EDGE('',*,*,#10921,.T.);
#15008=ORIENTED_EDGE('',*,*,#10991,.T.);
#15009=ORIENTED_EDGE('',*,*,#10920,.F.);
#15010=ORIENTED_EDGE('',*,*,#10924,.T.);
#15011=ORIENTED_EDGE('',*,*,#10928,.T.);
#15012=ORIENTED_EDGE('',*,*,#10993,.F.);
#15013=ORIENTED_EDGE('',*,*,#10994,.F.);
#15014=ORIENTED_EDGE('',*,*,#10995,.F.);
#15015=ORIENTED_EDGE('',*,*,#10996,.F.);
#15016=ORIENTED_EDGE('',*,*,#10993,.T.);
#15017=ORIENTED_EDGE('',*,*,#10927,.T.);
#15018=ORIENTED_EDGE('',*,*,#10997,.F.);
#15019=ORIENTED_EDGE('',*,*,#10995,.T.);
#15020=ORIENTED_EDGE('',*,*,#10949,.T.);
#15021=ORIENTED_EDGE('',*,*,#10349,.F.);
#15022=ORIENTED_EDGE('',*,*,#10998,.F.);
#15023=ORIENTED_EDGE('',*,*,#10347,.T.);
#15024=ORIENTED_EDGE('',*,*,#10959,.T.);
#15025=ORIENTED_EDGE('',*,*,#10999,.F.);
#15026=ORIENTED_EDGE('',*,*,#11000,.F.);
#15027=ORIENTED_EDGE('',*,*,#11001,.F.);
#15028=ORIENTED_EDGE('',*,*,#10999,.T.);
#15029=ORIENTED_EDGE('',*,*,#10931,.T.);
#15030=ORIENTED_EDGE('',*,*,#11000,.T.);
#15031=ORIENTED_EDGE('',*,*,#10930,.F.);
#15032=ORIENTED_EDGE('',*,*,#10934,.T.);
#15033=ORIENTED_EDGE('',*,*,#10938,.T.);
#15034=ORIENTED_EDGE('',*,*,#11002,.F.);
#15035=ORIENTED_EDGE('',*,*,#11003,.F.);
#15036=ORIENTED_EDGE('',*,*,#11004,.F.);
#15037=ORIENTED_EDGE('',*,*,#11005,.F.);
#15038=ORIENTED_EDGE('',*,*,#11002,.T.);
#15039=ORIENTED_EDGE('',*,*,#10937,.T.);
#15040=ORIENTED_EDGE('',*,*,#11006,.F.);
#15041=ORIENTED_EDGE('',*,*,#11004,.T.);
#15042=ORIENTED_EDGE('',*,*,#10958,.T.);
#15043=ORIENTED_EDGE('',*,*,#11007,.F.);
#15044=ORIENTED_EDGE('',*,*,#11008,.F.);
#15045=ORIENTED_EDGE('',*,*,#11009,.F.);
#15046=ORIENTED_EDGE('',*,*,#11007,.T.);
#15047=ORIENTED_EDGE('',*,*,#10957,.T.);
#15048=ORIENTED_EDGE('',*,*,#11010,.F.);
#15049=ORIENTED_EDGE('',*,*,#11008,.T.);
#15050=ORIENTED_EDGE('',*,*,#10956,.T.);
#15051=ORIENTED_EDGE('',*,*,#11011,.F.);
#15052=ORIENTED_EDGE('',*,*,#11012,.F.);
#15053=ORIENTED_EDGE('',*,*,#11013,.F.);
#15054=ORIENTED_EDGE('',*,*,#11011,.T.);
#15055=ORIENTED_EDGE('',*,*,#10942,.T.);
#15056=ORIENTED_EDGE('',*,*,#11014,.F.);
#15057=ORIENTED_EDGE('',*,*,#11015,.F.);
#15058=ORIENTED_EDGE('',*,*,#11012,.T.);
#15059=ORIENTED_EDGE('',*,*,#10941,.T.);
#15060=ORIENTED_EDGE('',*,*,#10945,.T.);
#15061=ORIENTED_EDGE('',*,*,#10948,.T.);
#15062=ORIENTED_EDGE('',*,*,#11016,.F.);
#15063=ORIENTED_EDGE('',*,*,#11017,.F.);
#15064=ORIENTED_EDGE('',*,*,#11014,.T.);
#15065=ORIENTED_EDGE('',*,*,#10947,.T.);
#15066=ORIENTED_EDGE('',*,*,#11018,.F.);
#15067=ORIENTED_EDGE('',*,*,#11016,.T.);
#15068=ORIENTED_EDGE('',*,*,#10955,.T.);
#15069=ORIENTED_EDGE('',*,*,#11019,.F.);
#15070=ORIENTED_EDGE('',*,*,#11020,.F.);
#15071=ORIENTED_EDGE('',*,*,#11019,.T.);
#15072=ORIENTED_EDGE('',*,*,#10954,.T.);
#15073=ORIENTED_EDGE('',*,*,#10977,.T.);
#15074=ORIENTED_EDGE('',*,*,#11021,.T.);
#15075=ORIENTED_EDGE('',*,*,#10965,.F.);
#15076=ORIENTED_EDGE('',*,*,#11022,.T.);
#15077=ORIENTED_EDGE('',*,*,#11023,.F.);
#15078=ORIENTED_EDGE('',*,*,#11022,.F.);
#15079=ORIENTED_EDGE('',*,*,#10964,.F.);
#15080=ORIENTED_EDGE('',*,*,#11024,.T.);
#15081=ORIENTED_EDGE('',*,*,#11025,.F.);
#15082=ORIENTED_EDGE('',*,*,#11024,.F.);
#15083=ORIENTED_EDGE('',*,*,#10963,.F.);
#15084=ORIENTED_EDGE('',*,*,#11026,.T.);
#15085=ORIENTED_EDGE('',*,*,#11027,.F.);
#15086=ORIENTED_EDGE('',*,*,#11026,.F.);
#15087=ORIENTED_EDGE('',*,*,#10962,.F.);
#15088=ORIENTED_EDGE('',*,*,#11028,.T.);
#15089=ORIENTED_EDGE('',*,*,#11029,.F.);
#15090=ORIENTED_EDGE('',*,*,#11028,.F.);
#15091=ORIENTED_EDGE('',*,*,#10961,.F.);
#15092=ORIENTED_EDGE('',*,*,#11030,.T.);
#15093=ORIENTED_EDGE('',*,*,#11031,.F.);
#15094=ORIENTED_EDGE('',*,*,#11030,.F.);
#15095=ORIENTED_EDGE('',*,*,#10960,.F.);
#15096=ORIENTED_EDGE('',*,*,#11021,.F.);
#15097=ORIENTED_EDGE('',*,*,#11032,.F.);
#15098=ORIENTED_EDGE('',*,*,#11033,.T.);
#15099=ORIENTED_EDGE('',*,*,#10971,.F.);
#15100=ORIENTED_EDGE('',*,*,#11034,.T.);
#15101=ORIENTED_EDGE('',*,*,#11035,.F.);
#15102=ORIENTED_EDGE('',*,*,#11034,.F.);
#15103=ORIENTED_EDGE('',*,*,#10970,.F.);
#15104=ORIENTED_EDGE('',*,*,#11036,.T.);
#15105=ORIENTED_EDGE('',*,*,#11037,.F.);
#15106=ORIENTED_EDGE('',*,*,#11036,.F.);
#15107=ORIENTED_EDGE('',*,*,#10969,.F.);
#15108=ORIENTED_EDGE('',*,*,#11038,.T.);
#15109=ORIENTED_EDGE('',*,*,#11039,.F.);
#15110=ORIENTED_EDGE('',*,*,#11038,.F.);
#15111=ORIENTED_EDGE('',*,*,#10968,.F.);
#15112=ORIENTED_EDGE('',*,*,#11040,.T.);
#15113=ORIENTED_EDGE('',*,*,#11041,.F.);
#15114=ORIENTED_EDGE('',*,*,#11040,.F.);
#15115=ORIENTED_EDGE('',*,*,#10967,.F.);
#15116=ORIENTED_EDGE('',*,*,#11042,.T.);
#15117=ORIENTED_EDGE('',*,*,#11043,.F.);
#15118=ORIENTED_EDGE('',*,*,#11042,.F.);
#15119=ORIENTED_EDGE('',*,*,#10966,.F.);
#15120=ORIENTED_EDGE('',*,*,#11033,.F.);
#15121=ORIENTED_EDGE('',*,*,#11044,.F.);
#15122=ORIENTED_EDGE('',*,*,#11045,.F.);
#15123=ORIENTED_EDGE('',*,*,#11046,.F.);
#15124=ORIENTED_EDGE('',*,*,#11047,.T.);
#15125=ORIENTED_EDGE('',*,*,#11048,.F.);
#15126=ORIENTED_EDGE('',*,*,#11049,.T.);
#15127=ORIENTED_EDGE('',*,*,#11050,.F.);
#15128=ORIENTED_EDGE('',*,*,#11051,.F.);
#15129=ORIENTED_EDGE('',*,*,#11052,.F.);
#15130=ORIENTED_EDGE('',*,*,#10901,.F.);
#15131=ORIENTED_EDGE('',*,*,#10974,.F.);
#15132=ORIENTED_EDGE('',*,*,#10898,.F.);
#15133=ORIENTED_EDGE('',*,*,#10973,.F.);
#15134=ORIENTED_EDGE('',*,*,#10892,.F.);
#15135=ORIENTED_EDGE('',*,*,#10972,.F.);
#15136=ORIENTED_EDGE('',*,*,#10906,.F.);
#15137=ORIENTED_EDGE('',*,*,#10975,.F.);
#15138=ORIENTED_EDGE('',*,*,#11053,.T.);
#15139=ORIENTED_EDGE('',*,*,#11054,.T.);
#15140=ORIENTED_EDGE('',*,*,#11055,.T.);
#15141=ORIENTED_EDGE('',*,*,#11056,.T.);
#15142=ORIENTED_EDGE('',*,*,#11057,.F.);
#15143=ORIENTED_EDGE('',*,*,#11058,.F.);
#15144=ORIENTED_EDGE('',*,*,#11059,.F.);
#15145=ORIENTED_EDGE('',*,*,#11060,.T.);
#15146=ORIENTED_EDGE('',*,*,#11054,.F.);
#15147=ORIENTED_EDGE('',*,*,#11061,.T.);
#15148=ORIENTED_EDGE('',*,*,#11062,.F.);
#15149=ORIENTED_EDGE('',*,*,#11058,.T.);
#15150=ORIENTED_EDGE('',*,*,#11063,.F.);
#15151=ORIENTED_EDGE('',*,*,#11064,.F.);
#15152=ORIENTED_EDGE('',*,*,#11065,.T.);
#15153=ORIENTED_EDGE('',*,*,#11066,.F.);
#15154=ORIENTED_EDGE('',*,*,#11067,.F.);
#15155=ORIENTED_EDGE('',*,*,#11068,.F.);
#15156=ORIENTED_EDGE('',*,*,#11069,.F.);
#15157=ORIENTED_EDGE('',*,*,#11070,.F.);
#15158=ORIENTED_EDGE('',*,*,#11071,.T.);
#15159=ORIENTED_EDGE('',*,*,#11072,.F.);
#15160=ORIENTED_EDGE('',*,*,#11073,.T.);
#15161=ORIENTED_EDGE('',*,*,#11074,.F.);
#15162=ORIENTED_EDGE('',*,*,#11075,.F.);
#15163=ORIENTED_EDGE('',*,*,#11076,.F.);
#15164=ORIENTED_EDGE('',*,*,#11018,.T.);
#15165=ORIENTED_EDGE('',*,*,#11020,.T.);
#15166=ORIENTED_EDGE('',*,*,#10976,.T.);
#15167=ORIENTED_EDGE('',*,*,#10980,.T.);
#15168=ORIENTED_EDGE('',*,*,#10982,.T.);
#15169=ORIENTED_EDGE('',*,*,#10984,.T.);
#15170=ORIENTED_EDGE('',*,*,#10985,.T.);
#15171=ORIENTED_EDGE('',*,*,#10988,.T.);
#15172=ORIENTED_EDGE('',*,*,#10989,.T.);
#15173=ORIENTED_EDGE('',*,*,#10992,.T.);
#15174=ORIENTED_EDGE('',*,*,#10994,.T.);
#15175=ORIENTED_EDGE('',*,*,#10996,.T.);
#15176=ORIENTED_EDGE('',*,*,#10997,.T.);
#15177=ORIENTED_EDGE('',*,*,#10348,.T.);
#15178=ORIENTED_EDGE('',*,*,#10998,.T.);
#15179=ORIENTED_EDGE('',*,*,#11001,.T.);
#15180=ORIENTED_EDGE('',*,*,#11003,.T.);
#15181=ORIENTED_EDGE('',*,*,#11005,.T.);
#15182=ORIENTED_EDGE('',*,*,#11006,.T.);
#15183=ORIENTED_EDGE('',*,*,#11009,.T.);
#15184=ORIENTED_EDGE('',*,*,#11010,.T.);
#15185=ORIENTED_EDGE('',*,*,#11013,.T.);
#15186=ORIENTED_EDGE('',*,*,#11015,.T.);
#15187=ORIENTED_EDGE('',*,*,#11017,.T.);
#15188=ORIENTED_EDGE('',*,*,#11077,.F.);
#15189=ORIENTED_EDGE('',*,*,#11069,.T.);
#15190=ORIENTED_EDGE('',*,*,#11078,.F.);
#15191=ORIENTED_EDGE('',*,*,#11067,.T.);
#15192=ORIENTED_EDGE('',*,*,#11079,.F.);
#15193=ORIENTED_EDGE('',*,*,#11064,.T.);
#15194=ORIENTED_EDGE('',*,*,#11080,.F.);
#15195=ORIENTED_EDGE('',*,*,#11051,.T.);
#15196=ORIENTED_EDGE('',*,*,#11081,.F.);
#15197=ORIENTED_EDGE('',*,*,#11045,.T.);
#15198=ORIENTED_EDGE('',*,*,#11082,.F.);
#15199=ORIENTED_EDGE('',*,*,#11083,.F.);
#15200=ORIENTED_EDGE('',*,*,#11084,.F.);
#15201=ORIENTED_EDGE('',*,*,#10341,.F.);
#15202=ORIENTED_EDGE('',*,*,#11085,.F.);
#15203=ORIENTED_EDGE('',*,*,#11075,.T.);
#15204=ORIENTED_EDGE('',*,*,#11086,.T.);
#15205=ORIENTED_EDGE('',*,*,#11087,.F.);
#15206=ORIENTED_EDGE('',*,*,#11083,.T.);
#15207=ORIENTED_EDGE('',*,*,#11088,.F.);
#15208=ORIENTED_EDGE('',*,*,#10326,.F.);
#15209=ORIENTED_EDGE('',*,*,#11031,.T.);
#15210=ORIENTED_EDGE('',*,*,#11032,.T.);
#15211=ORIENTED_EDGE('',*,*,#11023,.T.);
#15212=ORIENTED_EDGE('',*,*,#11025,.T.);
#15213=ORIENTED_EDGE('',*,*,#11027,.T.);
#15214=ORIENTED_EDGE('',*,*,#11029,.T.);
#15215=ORIENTED_EDGE('',*,*,#10323,.F.);
#15216=ORIENTED_EDGE('',*,*,#11043,.T.);
#15217=ORIENTED_EDGE('',*,*,#11044,.T.);
#15218=ORIENTED_EDGE('',*,*,#11035,.T.);
#15219=ORIENTED_EDGE('',*,*,#11037,.T.);
#15220=ORIENTED_EDGE('',*,*,#11039,.T.);
#15221=ORIENTED_EDGE('',*,*,#11041,.T.);
#15222=ORIENTED_EDGE('',*,*,#11048,.T.);
#15223=ORIENTED_EDGE('',*,*,#11089,.T.);
#15224=ORIENTED_EDGE('',*,*,#11090,.T.);
#15225=ORIENTED_EDGE('',*,*,#11091,.T.);
#15226=ORIENTED_EDGE('',*,*,#11088,.T.);
#15227=ORIENTED_EDGE('',*,*,#11082,.T.);
#15228=ORIENTED_EDGE('',*,*,#11050,.T.);
#15229=ORIENTED_EDGE('',*,*,#11092,.T.);
#15230=ORIENTED_EDGE('',*,*,#11093,.T.);
#15231=ORIENTED_EDGE('',*,*,#11094,.T.);
#15232=ORIENTED_EDGE('',*,*,#11046,.T.);
#15233=ORIENTED_EDGE('',*,*,#11081,.T.);
#15234=ORIENTED_EDGE('',*,*,#11089,.F.);
#15235=ORIENTED_EDGE('',*,*,#11047,.F.);
#15236=ORIENTED_EDGE('',*,*,#11094,.F.);
#15237=ORIENTED_EDGE('',*,*,#11095,.T.);
#15238=ORIENTED_EDGE('',*,*,#11096,.F.);
#15239=ORIENTED_EDGE('',*,*,#11097,.T.);
#15240=ORIENTED_EDGE('',*,*,#11098,.T.);
#15241=ORIENTED_EDGE('',*,*,#11099,.T.);
#15242=ORIENTED_EDGE('',*,*,#11100,.F.);
#15243=ORIENTED_EDGE('',*,*,#11101,.T.);
#15244=ORIENTED_EDGE('',*,*,#11102,.T.);
#15245=ORIENTED_EDGE('',*,*,#11103,.F.);
#15246=ORIENTED_EDGE('',*,*,#11104,.T.);
#15247=ORIENTED_EDGE('',*,*,#11105,.T.);
#15248=ORIENTED_EDGE('',*,*,#11080,.T.);
#15249=ORIENTED_EDGE('',*,*,#11063,.T.);
#15250=ORIENTED_EDGE('',*,*,#11057,.T.);
#15251=ORIENTED_EDGE('',*,*,#11106,.T.);
#15252=ORIENTED_EDGE('',*,*,#11107,.T.);
#15253=ORIENTED_EDGE('',*,*,#11108,.T.);
#15254=ORIENTED_EDGE('',*,*,#11109,.T.);
#15255=ORIENTED_EDGE('',*,*,#11052,.T.);
#15256=ORIENTED_EDGE('',*,*,#11110,.T.);
#15257=ORIENTED_EDGE('',*,*,#11105,.F.);
#15258=ORIENTED_EDGE('',*,*,#11111,.T.);
#15259=ORIENTED_EDGE('',*,*,#11092,.F.);
#15260=ORIENTED_EDGE('',*,*,#11049,.F.);
#15261=ORIENTED_EDGE('',*,*,#11109,.F.);
#15262=ORIENTED_EDGE('',*,*,#10335,.F.);
#15263=ORIENTED_EDGE('',*,*,#11112,.F.);
#15264=ORIENTED_EDGE('',*,*,#11113,.F.);
#15265=ORIENTED_EDGE('',*,*,#11114,.T.);
#15266=ORIENTED_EDGE('',*,*,#11107,.F.);
#15267=ORIENTED_EDGE('',*,*,#11115,.T.);
#15268=ORIENTED_EDGE('',*,*,#11116,.T.);
#15269=ORIENTED_EDGE('',*,*,#11115,.F.);
#15270=ORIENTED_EDGE('',*,*,#11106,.F.);
#15271=ORIENTED_EDGE('',*,*,#11061,.F.);
#15272=ORIENTED_EDGE('',*,*,#11053,.F.);
#15273=ORIENTED_EDGE('',*,*,#11117,.T.);
#15274=ORIENTED_EDGE('',*,*,#11118,.T.);
#15275=ORIENTED_EDGE('',*,*,#11119,.T.);
#15276=ORIENTED_EDGE('',*,*,#11055,.F.);
#15277=ORIENTED_EDGE('',*,*,#11060,.F.);
#15278=ORIENTED_EDGE('',*,*,#11120,.F.);
#15279=ORIENTED_EDGE('',*,*,#11121,.T.);
#15280=ORIENTED_EDGE('',*,*,#11122,.T.);
#15281=ORIENTED_EDGE('',*,*,#11123,.T.);
#15282=ORIENTED_EDGE('',*,*,#11124,.T.);
#15283=ORIENTED_EDGE('',*,*,#11117,.F.);
#15284=ORIENTED_EDGE('',*,*,#11056,.F.);
#15285=ORIENTED_EDGE('',*,*,#11119,.F.);
#15286=ORIENTED_EDGE('',*,*,#11125,.T.);
#15287=ORIENTED_EDGE('',*,*,#11126,.T.);
#15288=ORIENTED_EDGE('',*,*,#11120,.T.);
#15289=ORIENTED_EDGE('',*,*,#11059,.T.);
#15290=ORIENTED_EDGE('',*,*,#11062,.T.);
#15291=ORIENTED_EDGE('',*,*,#11079,.T.);
#15292=ORIENTED_EDGE('',*,*,#11066,.T.);
#15293=ORIENTED_EDGE('',*,*,#11127,.T.);
#15294=ORIENTED_EDGE('',*,*,#11126,.F.);
#15295=ORIENTED_EDGE('',*,*,#11128,.T.);
#15296=ORIENTED_EDGE('',*,*,#11129,.F.);
#15297=ORIENTED_EDGE('',*,*,#11130,.T.);
#15298=ORIENTED_EDGE('',*,*,#11121,.F.);
#15299=ORIENTED_EDGE('',*,*,#11131,.T.);
#15300=ORIENTED_EDGE('',*,*,#11132,.F.);
#15301=ORIENTED_EDGE('',*,*,#11133,.T.);
#15302=ORIENTED_EDGE('',*,*,#11134,.T.);
#15303=ORIENTED_EDGE('',*,*,#11072,.T.);
#15304=ORIENTED_EDGE('',*,*,#11135,.T.);
#15305=ORIENTED_EDGE('',*,*,#11136,.T.);
#15306=ORIENTED_EDGE('',*,*,#11137,.T.);
#15307=ORIENTED_EDGE('',*,*,#11068,.T.);
#15308=ORIENTED_EDGE('',*,*,#11078,.T.);
#15309=ORIENTED_EDGE('',*,*,#11138,.T.);
#15310=ORIENTED_EDGE('',*,*,#11134,.F.);
#15311=ORIENTED_EDGE('',*,*,#11139,.T.);
#15312=ORIENTED_EDGE('',*,*,#11127,.F.);
#15313=ORIENTED_EDGE('',*,*,#11065,.F.);
#15314=ORIENTED_EDGE('',*,*,#11137,.F.);
#15315=ORIENTED_EDGE('',*,*,#10332,.F.);
#15316=ORIENTED_EDGE('',*,*,#11074,.T.);
#15317=ORIENTED_EDGE('',*,*,#11140,.T.);
#15318=ORIENTED_EDGE('',*,*,#11141,.T.);
#15319=ORIENTED_EDGE('',*,*,#11142,.T.);
#15320=ORIENTED_EDGE('',*,*,#11070,.T.);
#15321=ORIENTED_EDGE('',*,*,#11077,.T.);
#15322=ORIENTED_EDGE('',*,*,#11135,.F.);
#15323=ORIENTED_EDGE('',*,*,#11071,.F.);
#15324=ORIENTED_EDGE('',*,*,#11142,.F.);
#15325=ORIENTED_EDGE('',*,*,#11143,.T.);
#15326=ORIENTED_EDGE('',*,*,#11144,.F.);
#15327=ORIENTED_EDGE('',*,*,#11145,.T.);
#15328=ORIENTED_EDGE('',*,*,#11146,.T.);
#15329=ORIENTED_EDGE('',*,*,#11147,.T.);
#15330=ORIENTED_EDGE('',*,*,#11148,.F.);
#15331=ORIENTED_EDGE('',*,*,#11149,.T.);
#15332=ORIENTED_EDGE('',*,*,#11150,.T.);
#15333=ORIENTED_EDGE('',*,*,#11151,.F.);
#15334=ORIENTED_EDGE('',*,*,#11152,.T.);
#15335=ORIENTED_EDGE('',*,*,#11153,.T.);
#15336=ORIENTED_EDGE('',*,*,#10340,.T.);
#15337=ORIENTED_EDGE('',*,*,#11154,.T.);
#15338=ORIENTED_EDGE('',*,*,#11155,.T.);
#15339=ORIENTED_EDGE('',*,*,#11156,.T.);
#15340=ORIENTED_EDGE('',*,*,#11076,.T.);
#15341=ORIENTED_EDGE('',*,*,#11085,.T.);
#15342=ORIENTED_EDGE('',*,*,#11157,.T.);
#15343=ORIENTED_EDGE('',*,*,#11153,.F.);
#15344=ORIENTED_EDGE('',*,*,#11158,.T.);
#15345=ORIENTED_EDGE('',*,*,#11140,.F.);
#15346=ORIENTED_EDGE('',*,*,#11073,.F.);
#15347=ORIENTED_EDGE('',*,*,#11156,.F.);
#15348=ORIENTED_EDGE('',*,*,#10329,.F.);
#15349=ORIENTED_EDGE('',*,*,#11159,.T.);
#15350=ORIENTED_EDGE('',*,*,#11160,.F.);
#15351=ORIENTED_EDGE('',*,*,#11161,.T.);
#15352=ORIENTED_EDGE('',*,*,#11162,.T.);
#15353=ORIENTED_EDGE('',*,*,#11163,.T.);
#15354=ORIENTED_EDGE('',*,*,#11162,.F.);
#15355=ORIENTED_EDGE('',*,*,#11164,.T.);
#15356=ORIENTED_EDGE('',*,*,#11165,.F.);
#15357=ORIENTED_EDGE('',*,*,#11086,.F.);
#15358=ORIENTED_EDGE('',*,*,#11091,.F.);
#15359=ORIENTED_EDGE('',*,*,#10338,.F.);
#15360=ORIENTED_EDGE('',*,*,#11087,.T.);
#15361=ORIENTED_EDGE('',*,*,#11165,.T.);
#15362=ORIENTED_EDGE('',*,*,#11166,.T.);
#15363=ORIENTED_EDGE('',*,*,#11167,.T.);
#15364=ORIENTED_EDGE('',*,*,#10342,.T.);
#15365=ORIENTED_EDGE('',*,*,#11084,.T.);
#15366=ORIENTED_EDGE('',*,*,#10339,.F.);
#15367=ORIENTED_EDGE('',*,*,#11167,.F.);
#15368=ORIENTED_EDGE('',*,*,#11168,.T.);
#15369=ORIENTED_EDGE('',*,*,#11169,.F.);
#15370=ORIENTED_EDGE('',*,*,#11170,.T.);
#15371=ORIENTED_EDGE('',*,*,#11171,.T.);
#15372=ORIENTED_EDGE('',*,*,#11172,.T.);
#15373=ORIENTED_EDGE('',*,*,#11173,.F.);
#15374=ORIENTED_EDGE('',*,*,#11174,.T.);
#15375=ORIENTED_EDGE('',*,*,#11154,.F.);
#15376=ORIENTED_EDGE('',*,*,#11175,.T.);
#15377=ORIENTED_EDGE('',*,*,#11176,.T.);
#15378=ORIENTED_EDGE('',*,*,#11177,.T.);
#15379=ORIENTED_EDGE('',*,*,#11178,.T.);
#15380=ORIENTED_EDGE('',*,*,#11179,.T.);
#15381=ORIENTED_EDGE('',*,*,#11180,.T.);
#15382=ORIENTED_EDGE('',*,*,#11181,.T.);
#15383=ORIENTED_EDGE('',*,*,#11182,.T.);
#15384=ORIENTED_EDGE('',*,*,#11183,.F.);
#15385=ORIENTED_EDGE('',*,*,#11184,.T.);
#15386=ORIENTED_EDGE('',*,*,#10320,.F.);
#15387=ORIENTED_EDGE('',*,*,#10131,.T.);
#15388=ORIENTED_EDGE('',*,*,#11185,.T.);
#15389=ORIENTED_EDGE('',*,*,#11186,.T.);
#15390=ORIENTED_EDGE('',*,*,#11160,.T.);
#15391=ORIENTED_EDGE('',*,*,#11187,.T.);
#15392=ORIENTED_EDGE('',*,*,#11188,.T.);
#15393=ORIENTED_EDGE('',*,*,#11189,.F.);
#15394=ORIENTED_EDGE('',*,*,#10336,.T.);
#15395=ORIENTED_EDGE('',*,*,#11189,.T.);
#15396=ORIENTED_EDGE('',*,*,#11190,.T.);
#15397=ORIENTED_EDGE('',*,*,#11191,.T.);
#15398=ORIENTED_EDGE('',*,*,#11192,.T.);
#15399=ORIENTED_EDGE('',*,*,#11090,.F.);
#15400=ORIENTED_EDGE('',*,*,#11101,.F.);
#15401=ORIENTED_EDGE('',*,*,#11193,.F.);
#15402=ORIENTED_EDGE('',*,*,#11194,.F.);
#15403=ORIENTED_EDGE('',*,*,#11195,.T.);
#15404=ORIENTED_EDGE('',*,*,#11187,.F.);
#15405=ORIENTED_EDGE('',*,*,#11159,.F.);
#15406=ORIENTED_EDGE('',*,*,#11163,.F.);
#15407=ORIENTED_EDGE('',*,*,#11100,.T.);
#15408=ORIENTED_EDGE('',*,*,#11196,.T.);
#15409=ORIENTED_EDGE('',*,*,#11197,.F.);
#15410=ORIENTED_EDGE('',*,*,#11193,.T.);
#15411=ORIENTED_EDGE('',*,*,#11196,.F.);
#15412=ORIENTED_EDGE('',*,*,#11099,.F.);
#15413=ORIENTED_EDGE('',*,*,#11198,.T.);
#15414=ORIENTED_EDGE('',*,*,#11199,.F.);
#15415=ORIENTED_EDGE('',*,*,#11198,.F.);
#15416=ORIENTED_EDGE('',*,*,#11098,.F.);
#15417=ORIENTED_EDGE('',*,*,#11200,.T.);
#15418=ORIENTED_EDGE('',*,*,#11201,.F.);
#15419=ORIENTED_EDGE('',*,*,#11200,.F.);
#15420=ORIENTED_EDGE('',*,*,#11097,.F.);
#15421=ORIENTED_EDGE('',*,*,#11202,.F.);
#15422=ORIENTED_EDGE('',*,*,#11203,.F.);
#15423=ORIENTED_EDGE('',*,*,#11096,.T.);
#15424=ORIENTED_EDGE('',*,*,#11204,.T.);
#15425=ORIENTED_EDGE('',*,*,#11205,.F.);
#15426=ORIENTED_EDGE('',*,*,#11202,.T.);
#15427=ORIENTED_EDGE('',*,*,#11093,.F.);
#15428=ORIENTED_EDGE('',*,*,#11111,.F.);
#15429=ORIENTED_EDGE('',*,*,#11104,.F.);
#15430=ORIENTED_EDGE('',*,*,#11206,.F.);
#15431=ORIENTED_EDGE('',*,*,#11207,.T.);
#15432=ORIENTED_EDGE('',*,*,#11208,.F.);
#15433=ORIENTED_EDGE('',*,*,#11204,.F.);
#15434=ORIENTED_EDGE('',*,*,#11095,.F.);
#15435=ORIENTED_EDGE('',*,*,#11209,.T.);
#15436=ORIENTED_EDGE('',*,*,#11206,.T.);
#15437=ORIENTED_EDGE('',*,*,#11103,.T.);
#15438=ORIENTED_EDGE('',*,*,#11210,.T.);
#15439=ORIENTED_EDGE('',*,*,#11211,.T.);
#15440=ORIENTED_EDGE('',*,*,#11212,.F.);
#15441=ORIENTED_EDGE('',*,*,#10333,.T.);
#15442=ORIENTED_EDGE('',*,*,#11212,.T.);
#15443=ORIENTED_EDGE('',*,*,#11213,.T.);
#15444=ORIENTED_EDGE('',*,*,#11214,.T.);
#15445=ORIENTED_EDGE('',*,*,#11215,.T.);
#15446=ORIENTED_EDGE('',*,*,#11108,.F.);
#15447=ORIENTED_EDGE('',*,*,#11114,.F.);
#15448=ORIENTED_EDGE('',*,*,#11216,.F.);
#15449=ORIENTED_EDGE('',*,*,#11217,.F.);
#15450=ORIENTED_EDGE('',*,*,#11218,.T.);
#15451=ORIENTED_EDGE('',*,*,#11210,.F.);
#15452=ORIENTED_EDGE('',*,*,#11102,.F.);
#15453=ORIENTED_EDGE('',*,*,#11110,.F.);
#15454=ORIENTED_EDGE('',*,*,#11113,.T.);
#15455=ORIENTED_EDGE('',*,*,#11219,.T.);
#15456=ORIENTED_EDGE('',*,*,#11220,.F.);
#15457=ORIENTED_EDGE('',*,*,#11216,.T.);
#15458=ORIENTED_EDGE('',*,*,#11221,.T.);
#15459=ORIENTED_EDGE('',*,*,#11222,.F.);
#15460=ORIENTED_EDGE('',*,*,#11219,.F.);
#15461=ORIENTED_EDGE('',*,*,#11112,.T.);
#15462=ORIENTED_EDGE('',*,*,#11116,.F.);
#15463=ORIENTED_EDGE('',*,*,#11124,.F.);
#15464=ORIENTED_EDGE('',*,*,#11223,.T.);
#15465=ORIENTED_EDGE('',*,*,#11224,.F.);
#15466=ORIENTED_EDGE('',*,*,#11221,.F.);
#15467=ORIENTED_EDGE('',*,*,#11123,.F.);
#15468=ORIENTED_EDGE('',*,*,#11118,.F.);
#15469=ORIENTED_EDGE('',*,*,#11130,.F.);
#15470=ORIENTED_EDGE('',*,*,#11225,.F.);
#15471=ORIENTED_EDGE('',*,*,#11226,.F.);
#15472=ORIENTED_EDGE('',*,*,#11223,.F.);
#15473=ORIENTED_EDGE('',*,*,#11122,.F.);
#15474=ORIENTED_EDGE('',*,*,#11129,.T.);
#15475=ORIENTED_EDGE('',*,*,#11227,.T.);
#15476=ORIENTED_EDGE('',*,*,#11228,.F.);
#15477=ORIENTED_EDGE('',*,*,#11225,.T.);
#15478=ORIENTED_EDGE('',*,*,#11125,.F.);
#15479=ORIENTED_EDGE('',*,*,#11139,.F.);
#15480=ORIENTED_EDGE('',*,*,#11133,.F.);
#15481=ORIENTED_EDGE('',*,*,#11229,.F.);
#15482=ORIENTED_EDGE('',*,*,#11230,.T.);
#15483=ORIENTED_EDGE('',*,*,#11231,.F.);
#15484=ORIENTED_EDGE('',*,*,#11227,.F.);
#15485=ORIENTED_EDGE('',*,*,#11128,.F.);
#15486=ORIENTED_EDGE('',*,*,#11232,.T.);
#15487=ORIENTED_EDGE('',*,*,#11229,.T.);
#15488=ORIENTED_EDGE('',*,*,#11132,.T.);
#15489=ORIENTED_EDGE('',*,*,#11233,.T.);
#15490=ORIENTED_EDGE('',*,*,#11234,.T.);
#15491=ORIENTED_EDGE('',*,*,#11235,.F.);
#15492=ORIENTED_EDGE('',*,*,#10330,.T.);
#15493=ORIENTED_EDGE('',*,*,#11235,.T.);
#15494=ORIENTED_EDGE('',*,*,#11236,.T.);
#15495=ORIENTED_EDGE('',*,*,#11237,.T.);
#15496=ORIENTED_EDGE('',*,*,#11238,.T.);
#15497=ORIENTED_EDGE('',*,*,#11136,.F.);
#15498=ORIENTED_EDGE('',*,*,#11149,.F.);
#15499=ORIENTED_EDGE('',*,*,#11239,.F.);
#15500=ORIENTED_EDGE('',*,*,#11240,.F.);
#15501=ORIENTED_EDGE('',*,*,#11241,.T.);
#15502=ORIENTED_EDGE('',*,*,#11233,.F.);
#15503=ORIENTED_EDGE('',*,*,#11131,.F.);
#15504=ORIENTED_EDGE('',*,*,#11138,.F.);
#15505=ORIENTED_EDGE('',*,*,#11148,.T.);
#15506=ORIENTED_EDGE('',*,*,#11242,.T.);
#15507=ORIENTED_EDGE('',*,*,#11243,.F.);
#15508=ORIENTED_EDGE('',*,*,#11239,.T.);
#15509=ORIENTED_EDGE('',*,*,#11242,.F.);
#15510=ORIENTED_EDGE('',*,*,#11147,.F.);
#15511=ORIENTED_EDGE('',*,*,#11244,.T.);
#15512=ORIENTED_EDGE('',*,*,#11245,.F.);
#15513=ORIENTED_EDGE('',*,*,#11244,.F.);
#15514=ORIENTED_EDGE('',*,*,#11146,.F.);
#15515=ORIENTED_EDGE('',*,*,#11246,.T.);
#15516=ORIENTED_EDGE('',*,*,#11247,.F.);
#15517=ORIENTED_EDGE('',*,*,#11246,.F.);
#15518=ORIENTED_EDGE('',*,*,#11145,.F.);
#15519=ORIENTED_EDGE('',*,*,#11248,.F.);
#15520=ORIENTED_EDGE('',*,*,#11249,.F.);
#15521=ORIENTED_EDGE('',*,*,#11144,.T.);
#15522=ORIENTED_EDGE('',*,*,#11250,.T.);
#15523=ORIENTED_EDGE('',*,*,#11251,.F.);
#15524=ORIENTED_EDGE('',*,*,#11248,.T.);
#15525=ORIENTED_EDGE('',*,*,#11141,.F.);
#15526=ORIENTED_EDGE('',*,*,#11158,.F.);
#15527=ORIENTED_EDGE('',*,*,#11152,.F.);
#15528=ORIENTED_EDGE('',*,*,#11252,.F.);
#15529=ORIENTED_EDGE('',*,*,#11253,.T.);
#15530=ORIENTED_EDGE('',*,*,#11254,.F.);
#15531=ORIENTED_EDGE('',*,*,#11250,.F.);
#15532=ORIENTED_EDGE('',*,*,#11143,.F.);
#15533=ORIENTED_EDGE('',*,*,#11255,.T.);
#15534=ORIENTED_EDGE('',*,*,#11252,.T.);
#15535=ORIENTED_EDGE('',*,*,#11151,.T.);
#15536=ORIENTED_EDGE('',*,*,#11256,.T.);
#15537=ORIENTED_EDGE('',*,*,#11257,.T.);
#15538=ORIENTED_EDGE('',*,*,#11258,.F.);
#15539=ORIENTED_EDGE('',*,*,#10327,.T.);
#15540=ORIENTED_EDGE('',*,*,#11258,.T.);
#15541=ORIENTED_EDGE('',*,*,#11259,.T.);
#15542=ORIENTED_EDGE('',*,*,#11260,.T.);
#15543=ORIENTED_EDGE('',*,*,#11261,.T.);
#15544=ORIENTED_EDGE('',*,*,#11155,.F.);
#15545=ORIENTED_EDGE('',*,*,#11174,.F.);
#15546=ORIENTED_EDGE('',*,*,#11262,.F.);
#15547=ORIENTED_EDGE('',*,*,#11263,.F.);
#15548=ORIENTED_EDGE('',*,*,#11264,.T.);
#15549=ORIENTED_EDGE('',*,*,#11256,.F.);
#15550=ORIENTED_EDGE('',*,*,#11150,.F.);
#15551=ORIENTED_EDGE('',*,*,#11157,.F.);
#15552=ORIENTED_EDGE('',*,*,#11173,.T.);
#15553=ORIENTED_EDGE('',*,*,#11265,.T.);
#15554=ORIENTED_EDGE('',*,*,#11266,.F.);
#15555=ORIENTED_EDGE('',*,*,#11262,.T.);
#15556=ORIENTED_EDGE('',*,*,#11265,.F.);
#15557=ORIENTED_EDGE('',*,*,#11172,.F.);
#15558=ORIENTED_EDGE('',*,*,#11267,.T.);
#15559=ORIENTED_EDGE('',*,*,#11268,.F.);
#15560=ORIENTED_EDGE('',*,*,#11267,.F.);
#15561=ORIENTED_EDGE('',*,*,#11171,.F.);
#15562=ORIENTED_EDGE('',*,*,#11269,.T.);
#15563=ORIENTED_EDGE('',*,*,#11270,.F.);
#15564=ORIENTED_EDGE('',*,*,#11269,.F.);
#15565=ORIENTED_EDGE('',*,*,#11170,.F.);
#15566=ORIENTED_EDGE('',*,*,#11271,.F.);
#15567=ORIENTED_EDGE('',*,*,#11272,.F.);
#15568=ORIENTED_EDGE('',*,*,#11169,.T.);
#15569=ORIENTED_EDGE('',*,*,#11273,.T.);
#15570=ORIENTED_EDGE('',*,*,#11274,.F.);
#15571=ORIENTED_EDGE('',*,*,#11271,.T.);
#15572=ORIENTED_EDGE('',*,*,#11166,.F.);
#15573=ORIENTED_EDGE('',*,*,#11164,.F.);
#15574=ORIENTED_EDGE('',*,*,#11161,.F.);
#15575=ORIENTED_EDGE('',*,*,#11186,.F.);
#15576=ORIENTED_EDGE('',*,*,#11275,.T.);
#15577=ORIENTED_EDGE('',*,*,#11276,.F.);
#15578=ORIENTED_EDGE('',*,*,#11273,.F.);
#15579=ORIENTED_EDGE('',*,*,#11168,.F.);
#15580=ORIENTED_EDGE('',*,*,#11277,.T.);
#15581=ORIENTED_EDGE('',*,*,#11278,.F.);
#15582=ORIENTED_EDGE('',*,*,#11279,.T.);
#15583=ORIENTED_EDGE('',*,*,#11180,.F.);
#15584=ORIENTED_EDGE('',*,*,#11280,.T.);
#15585=ORIENTED_EDGE('',*,*,#11281,.F.);
#15586=ORIENTED_EDGE('',*,*,#11277,.F.);
#15587=ORIENTED_EDGE('',*,*,#11179,.F.);
#15588=ORIENTED_EDGE('',*,*,#11282,.T.);
#15589=ORIENTED_EDGE('',*,*,#11283,.F.);
#15590=ORIENTED_EDGE('',*,*,#11280,.F.);
#15591=ORIENTED_EDGE('',*,*,#11178,.F.);
#15592=ORIENTED_EDGE('',*,*,#11284,.T.);
#15593=ORIENTED_EDGE('',*,*,#11285,.F.);
#15594=ORIENTED_EDGE('',*,*,#11282,.F.);
#15595=ORIENTED_EDGE('',*,*,#11177,.F.);
#15596=ORIENTED_EDGE('',*,*,#11286,.T.);
#15597=ORIENTED_EDGE('',*,*,#11287,.F.);
#15598=ORIENTED_EDGE('',*,*,#11284,.F.);
#15599=ORIENTED_EDGE('',*,*,#11176,.F.);
#15600=ORIENTED_EDGE('',*,*,#11279,.F.);
#15601=ORIENTED_EDGE('',*,*,#11288,.F.);
#15602=ORIENTED_EDGE('',*,*,#11286,.F.);
#15603=ORIENTED_EDGE('',*,*,#11175,.F.);
#15604=ORIENTED_EDGE('',*,*,#10316,.T.);
#15605=ORIENTED_EDGE('',*,*,#10324,.T.);
#15606=ORIENTED_EDGE('',*,*,#10313,.T.);
#15607=ORIENTED_EDGE('',*,*,#10321,.T.);
#15608=ORIENTED_EDGE('',*,*,#11289,.F.);
#15609=ORIENTED_EDGE('',*,*,#11182,.F.);
#15610=ORIENTED_EDGE('',*,*,#11290,.T.);
#15611=ORIENTED_EDGE('',*,*,#10311,.F.);
#15612=ORIENTED_EDGE('',*,*,#11290,.F.);
#15613=ORIENTED_EDGE('',*,*,#11181,.F.);
#15614=ORIENTED_EDGE('',*,*,#11291,.T.);
#15615=ORIENTED_EDGE('',*,*,#10305,.F.);
#15616=ORIENTED_EDGE('',*,*,#10312,.F.);
#15617=ORIENTED_EDGE('',*,*,#11291,.F.);
#15618=ORIENTED_EDGE('',*,*,#11184,.F.);
#15619=ORIENTED_EDGE('',*,*,#11292,.F.);
#15620=ORIENTED_EDGE('',*,*,#10306,.F.);
#15621=ORIENTED_EDGE('',*,*,#11289,.T.);
#15622=ORIENTED_EDGE('',*,*,#10310,.F.);
#15623=ORIENTED_EDGE('',*,*,#10307,.F.);
#15624=ORIENTED_EDGE('',*,*,#11292,.T.);
#15625=ORIENTED_EDGE('',*,*,#11183,.T.);
#15626=ORIENTED_EDGE('',*,*,#10302,.T.);
#15627=ORIENTED_EDGE('',*,*,#10299,.T.);
#15628=ORIENTED_EDGE('',*,*,#10296,.T.);
#15629=ORIENTED_EDGE('',*,*,#10293,.T.);
#15630=ORIENTED_EDGE('',*,*,#11185,.F.);
#15631=ORIENTED_EDGE('',*,*,#11192,.F.);
#15632=ORIENTED_EDGE('',*,*,#11293,.T.);
#15633=ORIENTED_EDGE('',*,*,#11294,.F.);
#15634=ORIENTED_EDGE('',*,*,#11295,.F.);
#15635=ORIENTED_EDGE('',*,*,#11275,.F.);
#15636=ORIENTED_EDGE('',*,*,#11296,.F.);
#15637=ORIENTED_EDGE('',*,*,#11297,.F.);
#15638=ORIENTED_EDGE('',*,*,#11298,.F.);
#15639=ORIENTED_EDGE('',*,*,#11299,.F.);
#15640=ORIENTED_EDGE('',*,*,#11293,.F.);
#15641=ORIENTED_EDGE('',*,*,#11191,.F.);
#15642=ORIENTED_EDGE('',*,*,#11300,.T.);
#15643=ORIENTED_EDGE('',*,*,#11301,.F.);
#15644=ORIENTED_EDGE('',*,*,#11302,.F.);
#15645=ORIENTED_EDGE('',*,*,#11303,.F.);
#15646=ORIENTED_EDGE('',*,*,#11300,.F.);
#15647=ORIENTED_EDGE('',*,*,#11190,.F.);
#15648=ORIENTED_EDGE('',*,*,#11188,.F.);
#15649=ORIENTED_EDGE('',*,*,#11195,.F.);
#15650=ORIENTED_EDGE('',*,*,#11304,.T.);
#15651=ORIENTED_EDGE('',*,*,#11305,.F.);
#15652=ORIENTED_EDGE('',*,*,#11302,.T.);
#15653=ORIENTED_EDGE('',*,*,#11194,.T.);
#15654=ORIENTED_EDGE('',*,*,#11197,.T.);
#15655=ORIENTED_EDGE('',*,*,#11199,.T.);
#15656=ORIENTED_EDGE('',*,*,#11201,.T.);
#15657=ORIENTED_EDGE('',*,*,#11203,.T.);
#15658=ORIENTED_EDGE('',*,*,#11205,.T.);
#15659=ORIENTED_EDGE('',*,*,#11208,.T.);
#15660=ORIENTED_EDGE('',*,*,#11209,.F.);
#15661=ORIENTED_EDGE('',*,*,#11215,.F.);
#15662=ORIENTED_EDGE('',*,*,#11306,.T.);
#15663=ORIENTED_EDGE('',*,*,#11307,.F.);
#15664=ORIENTED_EDGE('',*,*,#11304,.F.);
#15665=ORIENTED_EDGE('',*,*,#11207,.F.);
#15666=ORIENTED_EDGE('',*,*,#11308,.F.);
#15667=ORIENTED_EDGE('',*,*,#11309,.F.);
#15668=ORIENTED_EDGE('',*,*,#11310,.F.);
#15669=ORIENTED_EDGE('',*,*,#11311,.F.);
#15670=ORIENTED_EDGE('',*,*,#11306,.F.);
#15671=ORIENTED_EDGE('',*,*,#11214,.F.);
#15672=ORIENTED_EDGE('',*,*,#11312,.T.);
#15673=ORIENTED_EDGE('',*,*,#10287,.F.);
#15674=ORIENTED_EDGE('',*,*,#11313,.F.);
#15675=ORIENTED_EDGE('',*,*,#10288,.F.);
#15676=ORIENTED_EDGE('',*,*,#11312,.F.);
#15677=ORIENTED_EDGE('',*,*,#11213,.F.);
#15678=ORIENTED_EDGE('',*,*,#11211,.F.);
#15679=ORIENTED_EDGE('',*,*,#11218,.F.);
#15680=ORIENTED_EDGE('',*,*,#11228,.T.);
#15681=ORIENTED_EDGE('',*,*,#11231,.T.);
#15682=ORIENTED_EDGE('',*,*,#11314,.T.);
#15683=ORIENTED_EDGE('',*,*,#10282,.F.);
#15684=ORIENTED_EDGE('',*,*,#11313,.T.);
#15685=ORIENTED_EDGE('',*,*,#11217,.T.);
#15686=ORIENTED_EDGE('',*,*,#11220,.T.);
#15687=ORIENTED_EDGE('',*,*,#11222,.T.);
#15688=ORIENTED_EDGE('',*,*,#11224,.T.);
#15689=ORIENTED_EDGE('',*,*,#11226,.T.);
#15690=ORIENTED_EDGE('',*,*,#11232,.F.);
#15691=ORIENTED_EDGE('',*,*,#11238,.F.);
#15692=ORIENTED_EDGE('',*,*,#11315,.T.);
#15693=ORIENTED_EDGE('',*,*,#10283,.F.);
#15694=ORIENTED_EDGE('',*,*,#11314,.F.);
#15695=ORIENTED_EDGE('',*,*,#11230,.F.);
#15696=ORIENTED_EDGE('',*,*,#11315,.F.);
#15697=ORIENTED_EDGE('',*,*,#11237,.F.);
#15698=ORIENTED_EDGE('',*,*,#11316,.T.);
#15699=ORIENTED_EDGE('',*,*,#11317,.F.);
#15700=ORIENTED_EDGE('',*,*,#11318,.F.);
#15701=ORIENTED_EDGE('',*,*,#11319,.F.);
#15702=ORIENTED_EDGE('',*,*,#11320,.F.);
#15703=ORIENTED_EDGE('',*,*,#10284,.F.);
#15704=ORIENTED_EDGE('',*,*,#11321,.F.);
#15705=ORIENTED_EDGE('',*,*,#11322,.F.);
#15706=ORIENTED_EDGE('',*,*,#11316,.F.);
#15707=ORIENTED_EDGE('',*,*,#11236,.F.);
#15708=ORIENTED_EDGE('',*,*,#11234,.F.);
#15709=ORIENTED_EDGE('',*,*,#11241,.F.);
#15710=ORIENTED_EDGE('',*,*,#11251,.T.);
#15711=ORIENTED_EDGE('',*,*,#11254,.T.);
#15712=ORIENTED_EDGE('',*,*,#11323,.T.);
#15713=ORIENTED_EDGE('',*,*,#11324,.F.);
#15714=ORIENTED_EDGE('',*,*,#11321,.T.);
#15715=ORIENTED_EDGE('',*,*,#11240,.T.);
#15716=ORIENTED_EDGE('',*,*,#11243,.T.);
#15717=ORIENTED_EDGE('',*,*,#11245,.T.);
#15718=ORIENTED_EDGE('',*,*,#11247,.T.);
#15719=ORIENTED_EDGE('',*,*,#11249,.T.);
#15720=ORIENTED_EDGE('',*,*,#11255,.F.);
#15721=ORIENTED_EDGE('',*,*,#11261,.F.);
#15722=ORIENTED_EDGE('',*,*,#11325,.T.);
#15723=ORIENTED_EDGE('',*,*,#11326,.F.);
#15724=ORIENTED_EDGE('',*,*,#11323,.F.);
#15725=ORIENTED_EDGE('',*,*,#11253,.F.);
#15726=ORIENTED_EDGE('',*,*,#11325,.F.);
#15727=ORIENTED_EDGE('',*,*,#11260,.F.);
#15728=ORIENTED_EDGE('',*,*,#11327,.T.);
#15729=ORIENTED_EDGE('',*,*,#11328,.F.);
#15730=ORIENTED_EDGE('',*,*,#11329,.F.);
#15731=ORIENTED_EDGE('',*,*,#11330,.F.);
#15732=ORIENTED_EDGE('',*,*,#11331,.F.);
#15733=ORIENTED_EDGE('',*,*,#11332,.F.);
#15734=ORIENTED_EDGE('',*,*,#11333,.F.);
#15735=ORIENTED_EDGE('',*,*,#11334,.F.);
#15736=ORIENTED_EDGE('',*,*,#11327,.F.);
#15737=ORIENTED_EDGE('',*,*,#11259,.F.);
#15738=ORIENTED_EDGE('',*,*,#11257,.F.);
#15739=ORIENTED_EDGE('',*,*,#11264,.F.);
#15740=ORIENTED_EDGE('',*,*,#11274,.T.);
#15741=ORIENTED_EDGE('',*,*,#11276,.T.);
#15742=ORIENTED_EDGE('',*,*,#11295,.T.);
#15743=ORIENTED_EDGE('',*,*,#11335,.F.);
#15744=ORIENTED_EDGE('',*,*,#11333,.T.);
#15745=ORIENTED_EDGE('',*,*,#11263,.T.);
#15746=ORIENTED_EDGE('',*,*,#11266,.T.);
#15747=ORIENTED_EDGE('',*,*,#11268,.T.);
#15748=ORIENTED_EDGE('',*,*,#11270,.T.);
#15749=ORIENTED_EDGE('',*,*,#11272,.T.);
#15750=ORIENTED_EDGE('',*,*,#10290,.F.);
#15751=ORIENTED_EDGE('',*,*,#11287,.T.);
#15752=ORIENTED_EDGE('',*,*,#11288,.T.);
#15753=ORIENTED_EDGE('',*,*,#11278,.T.);
#15754=ORIENTED_EDGE('',*,*,#11281,.T.);
#15755=ORIENTED_EDGE('',*,*,#11283,.T.);
#15756=ORIENTED_EDGE('',*,*,#11285,.T.);
#15757=ORIENTED_EDGE('',*,*,#11336,.T.);
#15758=ORIENTED_EDGE('',*,*,#11337,.T.);
#15759=ORIENTED_EDGE('',*,*,#11338,.T.);
#15760=ORIENTED_EDGE('',*,*,#11339,.T.);
#15761=ORIENTED_EDGE('',*,*,#11340,.T.);
#15762=ORIENTED_EDGE('',*,*,#11341,.T.);
#15763=ORIENTED_EDGE('',*,*,#11298,.T.);
#15764=ORIENTED_EDGE('',*,*,#11342,.F.);
#15765=ORIENTED_EDGE('',*,*,#10254,.F.);
#15766=ORIENTED_EDGE('',*,*,#11343,.T.);
#15767=ORIENTED_EDGE('',*,*,#11344,.F.);
#15768=ORIENTED_EDGE('',*,*,#10255,.F.);
#15769=ORIENTED_EDGE('',*,*,#11342,.T.);
#15770=ORIENTED_EDGE('',*,*,#11297,.T.);
#15771=ORIENTED_EDGE('',*,*,#11296,.T.);
#15772=ORIENTED_EDGE('',*,*,#11345,.F.);
#15773=ORIENTED_EDGE('',*,*,#10256,.F.);
#15774=ORIENTED_EDGE('',*,*,#11344,.T.);
#15775=ORIENTED_EDGE('',*,*,#11345,.T.);
#15776=ORIENTED_EDGE('',*,*,#11301,.T.);
#15777=ORIENTED_EDGE('',*,*,#11303,.T.);
#15778=ORIENTED_EDGE('',*,*,#11305,.T.);
#15779=ORIENTED_EDGE('',*,*,#11307,.T.);
#15780=ORIENTED_EDGE('',*,*,#11311,.T.);
#15781=ORIENTED_EDGE('',*,*,#11346,.F.);
#15782=ORIENTED_EDGE('',*,*,#10262,.F.);
#15783=ORIENTED_EDGE('',*,*,#10257,.F.);
#15784=ORIENTED_EDGE('',*,*,#11310,.T.);
#15785=ORIENTED_EDGE('',*,*,#11347,.F.);
#15786=ORIENTED_EDGE('',*,*,#10263,.F.);
#15787=ORIENTED_EDGE('',*,*,#11346,.T.);
#15788=ORIENTED_EDGE('',*,*,#11348,.F.);
#15789=ORIENTED_EDGE('',*,*,#10264,.F.);
#15790=ORIENTED_EDGE('',*,*,#11347,.T.);
#15791=ORIENTED_EDGE('',*,*,#11309,.T.);
#15792=ORIENTED_EDGE('',*,*,#11308,.T.);
#15793=ORIENTED_EDGE('',*,*,#10286,.F.);
#15794=ORIENTED_EDGE('',*,*,#10265,.F.);
#15795=ORIENTED_EDGE('',*,*,#11348,.T.);
#15796=ORIENTED_EDGE('',*,*,#11320,.T.);
#15797=ORIENTED_EDGE('',*,*,#11349,.F.);
#15798=ORIENTED_EDGE('',*,*,#10267,.F.);
#15799=ORIENTED_EDGE('',*,*,#10285,.T.);
#15800=ORIENTED_EDGE('',*,*,#11350,.F.);
#15801=ORIENTED_EDGE('',*,*,#10268,.F.);
#15802=ORIENTED_EDGE('',*,*,#11349,.T.);
#15803=ORIENTED_EDGE('',*,*,#11319,.T.);
#15804=ORIENTED_EDGE('',*,*,#11318,.T.);
#15805=ORIENTED_EDGE('',*,*,#11351,.F.);
#15806=ORIENTED_EDGE('',*,*,#10269,.F.);
#15807=ORIENTED_EDGE('',*,*,#11350,.T.);
#15808=ORIENTED_EDGE('',*,*,#11351,.T.);
#15809=ORIENTED_EDGE('',*,*,#11317,.T.);
#15810=ORIENTED_EDGE('',*,*,#11322,.T.);
#15811=ORIENTED_EDGE('',*,*,#11324,.T.);
#15812=ORIENTED_EDGE('',*,*,#11326,.T.);
#15813=ORIENTED_EDGE('',*,*,#11332,.T.);
#15814=ORIENTED_EDGE('',*,*,#11352,.F.);
#15815=ORIENTED_EDGE('',*,*,#10249,.F.);
#15816=ORIENTED_EDGE('',*,*,#11331,.T.);
#15817=ORIENTED_EDGE('',*,*,#11353,.F.);
#15818=ORIENTED_EDGE('',*,*,#10250,.F.);
#15819=ORIENTED_EDGE('',*,*,#11352,.T.);
#15820=ORIENTED_EDGE('',*,*,#11354,.F.);
#15821=ORIENTED_EDGE('',*,*,#10251,.F.);
#15822=ORIENTED_EDGE('',*,*,#11353,.T.);
#15823=ORIENTED_EDGE('',*,*,#11330,.T.);
#15824=ORIENTED_EDGE('',*,*,#11329,.T.);
#15825=ORIENTED_EDGE('',*,*,#11355,.F.);
#15826=ORIENTED_EDGE('',*,*,#10252,.F.);
#15827=ORIENTED_EDGE('',*,*,#11354,.T.);
#15828=ORIENTED_EDGE('',*,*,#11334,.T.);
#15829=ORIENTED_EDGE('',*,*,#11335,.T.);
#15830=ORIENTED_EDGE('',*,*,#11294,.T.);
#15831=ORIENTED_EDGE('',*,*,#11299,.T.);
#15832=ORIENTED_EDGE('',*,*,#11343,.F.);
#15833=ORIENTED_EDGE('',*,*,#10253,.F.);
#15834=ORIENTED_EDGE('',*,*,#11355,.T.);
#15835=ORIENTED_EDGE('',*,*,#11328,.T.);
#15836=ORIENTED_EDGE('',*,*,#11356,.F.);
#15837=ORIENTED_EDGE('',*,*,#11357,.F.);
#15838=ORIENTED_EDGE('',*,*,#11358,.F.);
#15839=ORIENTED_EDGE('',*,*,#11359,.F.);
#15840=ORIENTED_EDGE('',*,*,#11360,.F.);
#15841=ORIENTED_EDGE('',*,*,#11361,.F.);
#15842=ORIENTED_EDGE('',*,*,#11362,.F.);
#15843=ORIENTED_EDGE('',*,*,#11363,.F.);
#15844=ORIENTED_EDGE('',*,*,#10318,.F.);
#15845=ORIENTED_EDGE('',*,*,#11360,.T.);
#15846=ORIENTED_EDGE('',*,*,#11364,.F.);
#15847=ORIENTED_EDGE('',*,*,#10278,.T.);
#15848=ORIENTED_EDGE('',*,*,#11365,.F.);
#15849=ORIENTED_EDGE('',*,*,#10280,.T.);
#15850=ORIENTED_EDGE('',*,*,#11366,.F.);
#15851=ORIENTED_EDGE('',*,*,#11367,.F.);
#15852=ORIENTED_EDGE('',*,*,#11368,.F.);
#15853=ORIENTED_EDGE('',*,*,#11369,.F.);
#15854=ORIENTED_EDGE('',*,*,#11370,.F.);
#15855=ORIENTED_EDGE('',*,*,#11371,.F.);
#15856=ORIENTED_EDGE('',*,*,#11372,.T.);
#15857=ORIENTED_EDGE('',*,*,#11373,.F.);
#15858=ORIENTED_EDGE('',*,*,#11374,.F.);
#15859=ORIENTED_EDGE('',*,*,#11367,.T.);
#15860=ORIENTED_EDGE('',*,*,#11375,.F.);
#15861=ORIENTED_EDGE('',*,*,#10315,.T.);
#15862=ORIENTED_EDGE('',*,*,#11376,.T.);
#15863=ORIENTED_EDGE('',*,*,#11377,.T.);
#15864=ORIENTED_EDGE('',*,*,#11378,.T.);
#15865=ORIENTED_EDGE('',*,*,#11379,.T.);
#15866=ORIENTED_EDGE('',*,*,#11380,.T.);
#15867=ORIENTED_EDGE('',*,*,#11381,.T.);
#15868=ORIENTED_EDGE('',*,*,#10201,.T.);
#15869=ORIENTED_EDGE('',*,*,#10242,.T.);
#15870=ORIENTED_EDGE('',*,*,#10248,.T.);
#15871=ORIENTED_EDGE('',*,*,#11382,.T.);
#15872=ORIENTED_EDGE('',*,*,#11383,.T.);
#15873=ORIENTED_EDGE('',*,*,#11384,.T.);
#15874=ORIENTED_EDGE('',*,*,#11385,.T.);
#15875=ORIENTED_EDGE('',*,*,#11340,.F.);
#15876=ORIENTED_EDGE('',*,*,#11385,.F.);
#15877=ORIENTED_EDGE('',*,*,#11386,.T.);
#15878=ORIENTED_EDGE('',*,*,#11387,.T.);
#15879=ORIENTED_EDGE('',*,*,#11341,.F.);
#15880=ORIENTED_EDGE('',*,*,#11387,.F.);
#15881=ORIENTED_EDGE('',*,*,#11388,.T.);
#15882=ORIENTED_EDGE('',*,*,#11389,.T.);
#15883=ORIENTED_EDGE('',*,*,#11336,.F.);
#15884=ORIENTED_EDGE('',*,*,#11389,.F.);
#15885=ORIENTED_EDGE('',*,*,#11390,.T.);
#15886=ORIENTED_EDGE('',*,*,#11391,.T.);
#15887=ORIENTED_EDGE('',*,*,#11337,.F.);
#15888=ORIENTED_EDGE('',*,*,#11391,.F.);
#15889=ORIENTED_EDGE('',*,*,#11392,.T.);
#15890=ORIENTED_EDGE('',*,*,#11393,.T.);
#15891=ORIENTED_EDGE('',*,*,#11338,.F.);
#15892=ORIENTED_EDGE('',*,*,#11393,.F.);
#15893=ORIENTED_EDGE('',*,*,#11394,.T.);
#15894=ORIENTED_EDGE('',*,*,#11383,.F.);
#15895=ORIENTED_EDGE('',*,*,#11339,.F.);
#15896=ORIENTED_EDGE('',*,*,#11382,.F.);
#15897=ORIENTED_EDGE('',*,*,#10247,.T.);
#15898=ORIENTED_EDGE('',*,*,#11395,.F.);
#15899=ORIENTED_EDGE('',*,*,#11396,.T.);
#15900=ORIENTED_EDGE('',*,*,#11397,.F.);
#15901=ORIENTED_EDGE('',*,*,#10202,.T.);
#15902=ORIENTED_EDGE('',*,*,#11371,.T.);
#15903=ORIENTED_EDGE('',*,*,#11398,.F.);
#15904=ORIENTED_EDGE('',*,*,#10235,.T.);
#15905=ORIENTED_EDGE('',*,*,#11399,.F.);
#15906=ORIENTED_EDGE('',*,*,#10234,.F.);
#15907=ORIENTED_EDGE('',*,*,#10303,.T.);
#15908=ORIENTED_EDGE('',*,*,#10231,.T.);
#15909=ORIENTED_EDGE('',*,*,#10300,.T.);
#15910=ORIENTED_EDGE('',*,*,#10228,.T.);
#15911=ORIENTED_EDGE('',*,*,#10297,.T.);
#15912=ORIENTED_EDGE('',*,*,#10225,.T.);
#15913=ORIENTED_EDGE('',*,*,#10294,.T.);
#15914=ORIENTED_EDGE('',*,*,#10222,.T.);
#15915=ORIENTED_EDGE('',*,*,#10291,.T.);
#15916=ORIENTED_EDGE('',*,*,#11400,.T.);
#15917=ORIENTED_EDGE('',*,*,#11401,.F.);
#15918=ORIENTED_EDGE('',*,*,#11402,.T.);
#15919=ORIENTED_EDGE('',*,*,#11401,.T.);
#15920=ORIENTED_EDGE('',*,*,#11403,.T.);
#15921=ORIENTED_EDGE('',*,*,#10277,.F.);
#15922=ORIENTED_EDGE('',*,*,#10273,.F.);
#15923=ORIENTED_EDGE('',*,*,#11404,.T.);
#15924=ORIENTED_EDGE('',*,*,#11405,.T.);
#15925=ORIENTED_EDGE('',*,*,#11406,.T.);
#15926=ORIENTED_EDGE('',*,*,#11407,.T.);
#15927=ORIENTED_EDGE('',*,*,#11408,.T.);
#15928=ORIENTED_EDGE('',*,*,#11409,.T.);
#15929=ORIENTED_EDGE('',*,*,#11410,.T.);
#15930=ORIENTED_EDGE('',*,*,#11411,.T.);
#15931=ORIENTED_EDGE('',*,*,#11412,.T.);
#15932=ORIENTED_EDGE('',*,*,#11413,.T.);
#15933=ORIENTED_EDGE('',*,*,#11414,.T.);
#15934=ORIENTED_EDGE('',*,*,#11415,.T.);
#15935=ORIENTED_EDGE('',*,*,#11416,.T.);
#15936=ORIENTED_EDGE('',*,*,#11417,.T.);
#15937=ORIENTED_EDGE('',*,*,#11418,.T.);
#15938=ORIENTED_EDGE('',*,*,#11419,.T.);
#15939=ORIENTED_EDGE('',*,*,#11420,.T.);
#15940=ORIENTED_EDGE('',*,*,#11421,.T.);
#15941=ORIENTED_EDGE('',*,*,#11422,.F.);
#15942=ORIENTED_EDGE('',*,*,#11370,.T.);
#15943=ORIENTED_EDGE('',*,*,#11423,.F.);
#15944=ORIENTED_EDGE('',*,*,#11423,.T.);
#15945=ORIENTED_EDGE('',*,*,#11369,.T.);
#15946=ORIENTED_EDGE('',*,*,#11424,.F.);
#15947=ORIENTED_EDGE('',*,*,#11425,.F.);
#15948=ORIENTED_EDGE('',*,*,#11426,.F.);
#15949=ORIENTED_EDGE('',*,*,#11424,.T.);
#15950=ORIENTED_EDGE('',*,*,#11375,.T.);
#15951=ORIENTED_EDGE('',*,*,#11427,.F.);
#15952=ORIENTED_EDGE('',*,*,#11359,.T.);
#15953=ORIENTED_EDGE('',*,*,#11428,.F.);
#15954=ORIENTED_EDGE('',*,*,#11428,.T.);
#15955=ORIENTED_EDGE('',*,*,#11358,.T.);
#15956=ORIENTED_EDGE('',*,*,#11429,.F.);
#15957=ORIENTED_EDGE('',*,*,#11430,.F.);
#15958=ORIENTED_EDGE('',*,*,#11431,.F.);
#15959=ORIENTED_EDGE('',*,*,#11429,.T.);
#15960=ORIENTED_EDGE('',*,*,#11357,.T.);
#15961=ORIENTED_EDGE('',*,*,#10209,.T.);
#15962=ORIENTED_EDGE('',*,*,#11432,.F.);
#15963=ORIENTED_EDGE('',*,*,#11356,.T.);
#15964=ORIENTED_EDGE('',*,*,#11433,.F.);
#15965=ORIENTED_EDGE('',*,*,#11434,.F.);
#15966=ORIENTED_EDGE('',*,*,#11363,.T.);
#15967=ORIENTED_EDGE('',*,*,#11435,.F.);
#15968=ORIENTED_EDGE('',*,*,#11435,.T.);
#15969=ORIENTED_EDGE('',*,*,#11362,.T.);
#15970=ORIENTED_EDGE('',*,*,#11436,.F.);
#15971=ORIENTED_EDGE('',*,*,#11437,.F.);
#15972=ORIENTED_EDGE('',*,*,#11438,.F.);
#15973=ORIENTED_EDGE('',*,*,#11436,.T.);
#15974=ORIENTED_EDGE('',*,*,#11361,.T.);
#15975=ORIENTED_EDGE('',*,*,#11439,.F.);
#15976=ORIENTED_EDGE('',*,*,#11374,.T.);
#15977=ORIENTED_EDGE('',*,*,#11440,.F.);
#15978=ORIENTED_EDGE('',*,*,#11440,.T.);
#15979=ORIENTED_EDGE('',*,*,#11373,.T.);
#15980=ORIENTED_EDGE('',*,*,#11441,.F.);
#15981=ORIENTED_EDGE('',*,*,#11442,.F.);
#15982=ORIENTED_EDGE('',*,*,#11443,.F.);
#15983=ORIENTED_EDGE('',*,*,#11441,.T.);
#15984=ORIENTED_EDGE('',*,*,#11372,.F.);
#15985=ORIENTED_EDGE('',*,*,#11444,.T.);
#15986=ORIENTED_EDGE('',*,*,#11445,.F.);
#15987=ORIENTED_EDGE('',*,*,#11446,.T.);
#15988=ORIENTED_EDGE('',*,*,#11380,.F.);
#15989=ORIENTED_EDGE('',*,*,#11447,.T.);
#15990=ORIENTED_EDGE('',*,*,#11448,.F.);
#15991=ORIENTED_EDGE('',*,*,#11444,.F.);
#15992=ORIENTED_EDGE('',*,*,#11379,.F.);
#15993=ORIENTED_EDGE('',*,*,#11449,.T.);
#15994=ORIENTED_EDGE('',*,*,#11450,.F.);
#15995=ORIENTED_EDGE('',*,*,#11447,.F.);
#15996=ORIENTED_EDGE('',*,*,#11378,.F.);
#15997=ORIENTED_EDGE('',*,*,#11451,.T.);
#15998=ORIENTED_EDGE('',*,*,#11452,.F.);
#15999=ORIENTED_EDGE('',*,*,#11449,.F.);
#16000=ORIENTED_EDGE('',*,*,#11377,.F.);
#16001=ORIENTED_EDGE('',*,*,#11453,.T.);
#16002=ORIENTED_EDGE('',*,*,#11454,.F.);
#16003=ORIENTED_EDGE('',*,*,#11451,.F.);
#16004=ORIENTED_EDGE('',*,*,#11376,.F.);
#16005=ORIENTED_EDGE('',*,*,#11446,.F.);
#16006=ORIENTED_EDGE('',*,*,#11455,.F.);
#16007=ORIENTED_EDGE('',*,*,#11453,.F.);
#16008=ORIENTED_EDGE('',*,*,#11381,.F.);
#16009=ORIENTED_EDGE('',*,*,#11456,.F.);
#16010=ORIENTED_EDGE('',*,*,#10203,.T.);
#16011=ORIENTED_EDGE('',*,*,#11397,.T.);
#16012=ORIENTED_EDGE('',*,*,#11457,.T.);
#16013=ORIENTED_EDGE('',*,*,#11458,.F.);
#16014=ORIENTED_EDGE('',*,*,#11459,.T.);
#16015=ORIENTED_EDGE('',*,*,#11460,.F.);
#16016=ORIENTED_EDGE('',*,*,#11458,.T.);
#16017=ORIENTED_EDGE('',*,*,#11459,.F.);
#16018=ORIENTED_EDGE('',*,*,#11457,.F.);
#16019=ORIENTED_EDGE('',*,*,#11396,.F.);
#16020=ORIENTED_EDGE('',*,*,#11461,.F.);
#16021=ORIENTED_EDGE('',*,*,#11462,.F.);
#16022=ORIENTED_EDGE('',*,*,#11463,.F.);
#16023=ORIENTED_EDGE('',*,*,#11392,.F.);
#16024=ORIENTED_EDGE('',*,*,#11390,.F.);
#16025=ORIENTED_EDGE('',*,*,#11388,.F.);
#16026=ORIENTED_EDGE('',*,*,#11386,.F.);
#16027=ORIENTED_EDGE('',*,*,#11384,.F.);
#16028=ORIENTED_EDGE('',*,*,#11394,.F.);
#16029=ORIENTED_EDGE('',*,*,#11464,.F.);
#16030=ORIENTED_EDGE('',*,*,#11465,.F.);
#16031=ORIENTED_EDGE('',*,*,#11462,.T.);
#16032=ORIENTED_EDGE('',*,*,#11466,.F.);
#16033=ORIENTED_EDGE('',*,*,#11467,.F.);
#16034=ORIENTED_EDGE('',*,*,#11464,.T.);
#16035=ORIENTED_EDGE('',*,*,#11461,.T.);
#16036=ORIENTED_EDGE('',*,*,#11395,.T.);
#16037=ORIENTED_EDGE('',*,*,#10246,.T.);
#16038=ORIENTED_EDGE('',*,*,#11468,.T.);
#16039=ORIENTED_EDGE('',*,*,#11469,.T.);
#16040=ORIENTED_EDGE('',*,*,#11470,.T.);
#16041=ORIENTED_EDGE('',*,*,#11471,.T.);
#16042=ORIENTED_EDGE('',*,*,#11472,.T.);
#16043=ORIENTED_EDGE('',*,*,#11473,.T.);
#16044=ORIENTED_EDGE('',*,*,#11474,.T.);
#16045=ORIENTED_EDGE('',*,*,#11475,.T.);
#16046=ORIENTED_EDGE('',*,*,#11476,.T.);
#16047=ORIENTED_EDGE('',*,*,#11477,.T.);
#16048=ORIENTED_EDGE('',*,*,#11478,.T.);
#16049=ORIENTED_EDGE('',*,*,#11479,.T.);
#16050=ORIENTED_EDGE('',*,*,#11480,.T.);
#16051=ORIENTED_EDGE('',*,*,#11481,.T.);
#16052=ORIENTED_EDGE('',*,*,#11482,.T.);
#16053=ORIENTED_EDGE('',*,*,#11483,.T.);
#16054=ORIENTED_EDGE('',*,*,#11484,.T.);
#16055=ORIENTED_EDGE('',*,*,#11485,.T.);
#16056=ORIENTED_EDGE('',*,*,#11486,.T.);
#16057=ORIENTED_EDGE('',*,*,#11487,.T.);
#16058=ORIENTED_EDGE('',*,*,#10259,.T.);
#16059=ORIENTED_EDGE('',*,*,#10219,.T.);
#16060=ORIENTED_EDGE('',*,*,#10260,.F.);
#16061=ORIENTED_EDGE('',*,*,#11487,.F.);
#16062=ORIENTED_EDGE('',*,*,#11488,.T.);
#16063=ORIENTED_EDGE('',*,*,#11489,.T.);
#16064=ORIENTED_EDGE('',*,*,#10272,.F.);
#16065=ORIENTED_EDGE('',*,*,#11403,.F.);
#16066=ORIENTED_EDGE('',*,*,#11400,.F.);
#16067=ORIENTED_EDGE('',*,*,#11402,.F.);
#16068=ORIENTED_EDGE('',*,*,#10261,.F.);
#16069=ORIENTED_EDGE('',*,*,#11489,.F.);
#16070=ORIENTED_EDGE('',*,*,#11490,.T.);
#16071=ORIENTED_EDGE('',*,*,#10217,.F.);
#16072=ORIENTED_EDGE('',*,*,#11491,.T.);
#16073=ORIENTED_EDGE('',*,*,#11492,.T.);
#16074=ORIENTED_EDGE('',*,*,#11493,.T.);
#16075=ORIENTED_EDGE('',*,*,#11494,.T.);
#16076=ORIENTED_EDGE('',*,*,#11495,.T.);
#16077=ORIENTED_EDGE('',*,*,#11496,.T.);
#16078=ORIENTED_EDGE('',*,*,#11497,.T.);
#16079=ORIENTED_EDGE('',*,*,#11498,.T.);
#16080=ORIENTED_EDGE('',*,*,#11499,.T.);
#16081=ORIENTED_EDGE('',*,*,#11500,.T.);
#16082=ORIENTED_EDGE('',*,*,#11501,.T.);
#16083=ORIENTED_EDGE('',*,*,#11502,.T.);
#16084=ORIENTED_EDGE('',*,*,#11503,.T.);
#16085=ORIENTED_EDGE('',*,*,#11409,.F.);
#16086=ORIENTED_EDGE('',*,*,#11504,.T.);
#16087=ORIENTED_EDGE('',*,*,#11505,.F.);
#16088=ORIENTED_EDGE('',*,*,#11504,.F.);
#16089=ORIENTED_EDGE('',*,*,#11408,.F.);
#16090=ORIENTED_EDGE('',*,*,#11506,.T.);
#16091=ORIENTED_EDGE('',*,*,#11507,.F.);
#16092=ORIENTED_EDGE('',*,*,#11506,.F.);
#16093=ORIENTED_EDGE('',*,*,#11407,.F.);
#16094=ORIENTED_EDGE('',*,*,#11508,.T.);
#16095=ORIENTED_EDGE('',*,*,#11509,.F.);
#16096=ORIENTED_EDGE('',*,*,#11508,.F.);
#16097=ORIENTED_EDGE('',*,*,#11406,.F.);
#16098=ORIENTED_EDGE('',*,*,#11510,.T.);
#16099=ORIENTED_EDGE('',*,*,#11511,.F.);
#16100=ORIENTED_EDGE('',*,*,#11510,.F.);
#16101=ORIENTED_EDGE('',*,*,#11405,.F.);
#16102=ORIENTED_EDGE('',*,*,#11512,.T.);
#16103=ORIENTED_EDGE('',*,*,#11513,.F.);
#16104=ORIENTED_EDGE('',*,*,#11512,.F.);
#16105=ORIENTED_EDGE('',*,*,#11404,.F.);
#16106=ORIENTED_EDGE('',*,*,#11503,.F.);
#16107=ORIENTED_EDGE('',*,*,#11514,.F.);
#16108=ORIENTED_EDGE('',*,*,#11515,.T.);
#16109=ORIENTED_EDGE('',*,*,#11516,.F.);
#16110=ORIENTED_EDGE('',*,*,#11517,.T.);
#16111=ORIENTED_EDGE('',*,*,#11518,.F.);
#16112=ORIENTED_EDGE('',*,*,#11519,.T.);
#16113=ORIENTED_EDGE('',*,*,#11515,.F.);
#16114=ORIENTED_EDGE('',*,*,#11520,.T.);
#16115=ORIENTED_EDGE('',*,*,#11521,.T.);
#16116=ORIENTED_EDGE('',*,*,#11522,.T.);
#16117=ORIENTED_EDGE('',*,*,#11523,.F.);
#16118=ORIENTED_EDGE('',*,*,#11524,.T.);
#16119=ORIENTED_EDGE('',*,*,#11518,.T.);
#16120=ORIENTED_EDGE('',*,*,#11525,.T.);
#16121=ORIENTED_EDGE('',*,*,#11526,.T.);
#16122=ORIENTED_EDGE('',*,*,#11527,.T.);
#16123=ORIENTED_EDGE('',*,*,#11414,.F.);
#16124=ORIENTED_EDGE('',*,*,#11527,.F.);
#16125=ORIENTED_EDGE('',*,*,#11528,.T.);
#16126=ORIENTED_EDGE('',*,*,#11529,.T.);
#16127=ORIENTED_EDGE('',*,*,#11415,.F.);
#16128=ORIENTED_EDGE('',*,*,#11529,.F.);
#16129=ORIENTED_EDGE('',*,*,#11530,.T.);
#16130=ORIENTED_EDGE('',*,*,#11531,.T.);
#16131=ORIENTED_EDGE('',*,*,#11410,.F.);
#16132=ORIENTED_EDGE('',*,*,#11531,.F.);
#16133=ORIENTED_EDGE('',*,*,#11532,.T.);
#16134=ORIENTED_EDGE('',*,*,#11533,.T.);
#16135=ORIENTED_EDGE('',*,*,#11411,.F.);
#16136=ORIENTED_EDGE('',*,*,#11533,.F.);
#16137=ORIENTED_EDGE('',*,*,#11534,.T.);
#16138=ORIENTED_EDGE('',*,*,#11535,.T.);
#16139=ORIENTED_EDGE('',*,*,#11412,.F.);
#16140=ORIENTED_EDGE('',*,*,#11535,.F.);
#16141=ORIENTED_EDGE('',*,*,#11536,.T.);
#16142=ORIENTED_EDGE('',*,*,#11525,.F.);
#16143=ORIENTED_EDGE('',*,*,#11413,.F.);
#16144=ORIENTED_EDGE('',*,*,#11537,.F.);
#16145=ORIENTED_EDGE('',*,*,#11538,.T.);
#16146=ORIENTED_EDGE('',*,*,#11539,.F.);
#16147=ORIENTED_EDGE('',*,*,#11540,.F.);
#16148=ORIENTED_EDGE('',*,*,#11539,.T.);
#16149=ORIENTED_EDGE('',*,*,#11541,.T.);
#16150=ORIENTED_EDGE('',*,*,#11542,.F.);
#16151=ORIENTED_EDGE('',*,*,#11543,.T.);
#16152=ORIENTED_EDGE('',*,*,#11544,.F.);
#16153=ORIENTED_EDGE('',*,*,#11545,.T.);
#16154=ORIENTED_EDGE('',*,*,#11546,.F.);
#16155=ORIENTED_EDGE('',*,*,#11547,.T.);
#16156=ORIENTED_EDGE('',*,*,#11420,.F.);
#16157=ORIENTED_EDGE('',*,*,#11548,.T.);
#16158=ORIENTED_EDGE('',*,*,#11549,.F.);
#16159=ORIENTED_EDGE('',*,*,#11545,.F.);
#16160=ORIENTED_EDGE('',*,*,#11419,.F.);
#16161=ORIENTED_EDGE('',*,*,#11550,.T.);
#16162=ORIENTED_EDGE('',*,*,#11551,.F.);
#16163=ORIENTED_EDGE('',*,*,#11548,.F.);
#16164=ORIENTED_EDGE('',*,*,#11418,.F.);
#16165=ORIENTED_EDGE('',*,*,#11552,.T.);
#16166=ORIENTED_EDGE('',*,*,#11553,.F.);
#16167=ORIENTED_EDGE('',*,*,#11550,.F.);
#16168=ORIENTED_EDGE('',*,*,#11417,.F.);
#16169=ORIENTED_EDGE('',*,*,#11554,.T.);
#16170=ORIENTED_EDGE('',*,*,#11555,.F.);
#16171=ORIENTED_EDGE('',*,*,#11552,.F.);
#16172=ORIENTED_EDGE('',*,*,#11416,.F.);
#16173=ORIENTED_EDGE('',*,*,#11547,.F.);
#16174=ORIENTED_EDGE('',*,*,#11556,.F.);
#16175=ORIENTED_EDGE('',*,*,#11554,.F.);
#16176=ORIENTED_EDGE('',*,*,#11421,.F.);
#16177=ORIENTED_EDGE('',*,*,#11557,.T.);
#16178=ORIENTED_EDGE('',*,*,#11558,.F.);
#16179=ORIENTED_EDGE('',*,*,#10212,.T.);
#16180=ORIENTED_EDGE('',*,*,#11559,.F.);
#16181=ORIENTED_EDGE('',*,*,#10208,.T.);
#16182=ORIENTED_EDGE('',*,*,#11560,.F.);
#16183=ORIENTED_EDGE('',*,*,#11561,.F.);
#16184=ORIENTED_EDGE('',*,*,#10214,.T.);
#16185=ORIENTED_EDGE('',*,*,#11562,.F.);
#16186=ORIENTED_EDGE('',*,*,#11563,.F.);
#16187=ORIENTED_EDGE('',*,*,#10236,.T.);
#16188=ORIENTED_EDGE('',*,*,#11398,.T.);
#16189=ORIENTED_EDGE('',*,*,#11422,.T.);
#16190=ORIENTED_EDGE('',*,*,#11425,.T.);
#16191=ORIENTED_EDGE('',*,*,#11426,.T.);
#16192=ORIENTED_EDGE('',*,*,#11366,.T.);
#16193=ORIENTED_EDGE('',*,*,#10279,.T.);
#16194=ORIENTED_EDGE('',*,*,#11364,.T.);
#16195=ORIENTED_EDGE('',*,*,#11427,.T.);
#16196=ORIENTED_EDGE('',*,*,#11430,.T.);
#16197=ORIENTED_EDGE('',*,*,#11431,.T.);
#16198=ORIENTED_EDGE('',*,*,#11432,.T.);
#16199=ORIENTED_EDGE('',*,*,#11442,.T.);
#16200=ORIENTED_EDGE('',*,*,#11443,.T.);
#16201=ORIENTED_EDGE('',*,*,#11399,.T.);
#16202=ORIENTED_EDGE('',*,*,#10238,.T.);
#16203=ORIENTED_EDGE('',*,*,#11564,.F.);
#16204=ORIENTED_EDGE('',*,*,#11565,.F.);
#16205=ORIENTED_EDGE('',*,*,#11466,.T.);
#16206=ORIENTED_EDGE('',*,*,#10245,.T.);
#16207=ORIENTED_EDGE('',*,*,#11566,.F.);
#16208=ORIENTED_EDGE('',*,*,#11567,.F.);
#16209=ORIENTED_EDGE('',*,*,#11568,.F.);
#16210=ORIENTED_EDGE('',*,*,#10210,.T.);
#16211=ORIENTED_EDGE('',*,*,#11433,.T.);
#16212=ORIENTED_EDGE('',*,*,#11434,.T.);
#16213=ORIENTED_EDGE('',*,*,#11437,.T.);
#16214=ORIENTED_EDGE('',*,*,#11438,.T.);
#16215=ORIENTED_EDGE('',*,*,#11365,.T.);
#16216=ORIENTED_EDGE('',*,*,#10281,.T.);
#16217=ORIENTED_EDGE('',*,*,#11368,.T.);
#16218=ORIENTED_EDGE('',*,*,#11439,.T.);
#16219=ORIENTED_EDGE('',*,*,#11569,.F.);
#16220=ORIENTED_EDGE('',*,*,#11570,.F.);
#16221=ORIENTED_EDGE('',*,*,#11566,.T.);
#16222=ORIENTED_EDGE('',*,*,#10244,.T.);
#16223=ORIENTED_EDGE('',*,*,#10240,.T.);
#16224=ORIENTED_EDGE('',*,*,#11571,.F.);
#16225=ORIENTED_EDGE('',*,*,#11572,.F.);
#16226=ORIENTED_EDGE('',*,*,#11573,.F.);
#16227=ORIENTED_EDGE('',*,*,#11569,.T.);
#16228=ORIENTED_EDGE('',*,*,#11574,.F.);
#16229=ORIENTED_EDGE('',*,*,#11575,.F.);
#16230=ORIENTED_EDGE('',*,*,#11572,.T.);
#16231=ORIENTED_EDGE('',*,*,#11571,.T.);
#16232=ORIENTED_EDGE('',*,*,#10239,.T.);
#16233=ORIENTED_EDGE('',*,*,#11576,.F.);
#16234=ORIENTED_EDGE('',*,*,#11454,.T.);
#16235=ORIENTED_EDGE('',*,*,#11455,.T.);
#16236=ORIENTED_EDGE('',*,*,#11445,.T.);
#16237=ORIENTED_EDGE('',*,*,#11448,.T.);
#16238=ORIENTED_EDGE('',*,*,#11450,.T.);
#16239=ORIENTED_EDGE('',*,*,#11452,.T.);
#16240=ORIENTED_EDGE('',*,*,#11577,.F.);
#16241=ORIENTED_EDGE('',*,*,#11578,.F.);
#16242=ORIENTED_EDGE('',*,*,#11574,.T.);
#16243=ORIENTED_EDGE('',*,*,#10199,.T.);
#16244=ORIENTED_EDGE('',*,*,#11579,.F.);
#16245=ORIENTED_EDGE('',*,*,#11577,.T.);
#16246=ORIENTED_EDGE('',*,*,#11576,.T.);
#16247=ORIENTED_EDGE('',*,*,#10243,.T.);
#16248=ORIENTED_EDGE('',*,*,#10196,.T.);
#16249=ORIENTED_EDGE('',*,*,#11580,.F.);
#16250=ORIENTED_EDGE('',*,*,#11581,.F.);
#16251=ORIENTED_EDGE('',*,*,#10205,.T.);
#16252=ORIENTED_EDGE('',*,*,#11582,.F.);
#16253=ORIENTED_EDGE('',*,*,#11583,.F.);
#16254=ORIENTED_EDGE('',*,*,#10192,.T.);
#16255=ORIENTED_EDGE('',*,*,#11584,.F.);
#16256=ORIENTED_EDGE('',*,*,#11585,.F.);
#16257=ORIENTED_EDGE('',*,*,#10198,.T.);
#16258=ORIENTED_EDGE('',*,*,#11586,.F.);
#16259=ORIENTED_EDGE('',*,*,#11587,.F.);
#16260=ORIENTED_EDGE('',*,*,#10194,.T.);
#16261=ORIENTED_EDGE('',*,*,#11588,.F.);
#16262=ORIENTED_EDGE('',*,*,#11589,.T.);
#16263=ORIENTED_EDGE('',*,*,#11590,.F.);
#16264=ORIENTED_EDGE('',*,*,#11524,.F.);
#16265=ORIENTED_EDGE('',*,*,#11591,.F.);
#16266=ORIENTED_EDGE('',*,*,#11541,.F.);
#16267=ORIENTED_EDGE('',*,*,#11538,.F.);
#16268=ORIENTED_EDGE('',*,*,#11592,.F.);
#16269=ORIENTED_EDGE('',*,*,#11589,.F.);
#16270=ORIENTED_EDGE('',*,*,#11593,.F.);
#16271=ORIENTED_EDGE('',*,*,#11519,.F.);
#16272=ORIENTED_EDGE('',*,*,#11594,.F.);
#16273=ORIENTED_EDGE('',*,*,#11595,.F.);
#16274=ORIENTED_EDGE('',*,*,#11537,.T.);
#16275=ORIENTED_EDGE('',*,*,#11596,.F.);
#16276=ORIENTED_EDGE('',*,*,#11597,.F.);
#16277=ORIENTED_EDGE('',*,*,#11598,.T.);
#16278=ORIENTED_EDGE('',*,*,#11599,.F.);
#16279=ORIENTED_EDGE('',*,*,#11600,.F.);
#16280=ORIENTED_EDGE('',*,*,#11601,.F.);
#16281=ORIENTED_EDGE('',*,*,#11602,.T.);
#16282=ORIENTED_EDGE('',*,*,#11603,.F.);
#16283=ORIENTED_EDGE('',*,*,#11557,.F.);
#16284=ORIENTED_EDGE('',*,*,#11604,.F.);
#16285=ORIENTED_EDGE('',*,*,#11605,.T.);
#16286=ORIENTED_EDGE('',*,*,#11606,.F.);
#16287=ORIENTED_EDGE('',*,*,#11607,.F.);
#16288=ORIENTED_EDGE('',*,*,#11608,.T.);
#16289=ORIENTED_EDGE('',*,*,#11608,.F.);
#16290=ORIENTED_EDGE('',*,*,#11602,.F.);
#16291=ORIENTED_EDGE('',*,*,#11609,.F.);
#16292=ORIENTED_EDGE('',*,*,#11610,.F.);
#16293=ORIENTED_EDGE('',*,*,#11609,.T.);
#16294=ORIENTED_EDGE('',*,*,#11601,.T.);
#16295=ORIENTED_EDGE('',*,*,#11611,.F.);
#16296=ORIENTED_EDGE('',*,*,#11612,.T.);
#16297=ORIENTED_EDGE('',*,*,#11613,.F.);
#16298=ORIENTED_EDGE('',*,*,#11583,.T.);
#16299=ORIENTED_EDGE('',*,*,#11582,.T.);
#16300=ORIENTED_EDGE('',*,*,#10204,.T.);
#16301=ORIENTED_EDGE('',*,*,#11456,.T.);
#16302=ORIENTED_EDGE('',*,*,#11460,.T.);
#16303=ORIENTED_EDGE('',*,*,#11463,.T.);
#16304=ORIENTED_EDGE('',*,*,#11465,.T.);
#16305=ORIENTED_EDGE('',*,*,#11467,.T.);
#16306=ORIENTED_EDGE('',*,*,#11565,.T.);
#16307=ORIENTED_EDGE('',*,*,#11564,.T.);
#16308=ORIENTED_EDGE('',*,*,#10237,.T.);
#16309=ORIENTED_EDGE('',*,*,#11563,.T.);
#16310=ORIENTED_EDGE('',*,*,#11562,.T.);
#16311=ORIENTED_EDGE('',*,*,#10213,.T.);
#16312=ORIENTED_EDGE('',*,*,#11558,.T.);
#16313=ORIENTED_EDGE('',*,*,#11603,.T.);
#16314=ORIENTED_EDGE('',*,*,#11607,.T.);
#16315=ORIENTED_EDGE('',*,*,#11614,.F.);
#16316=ORIENTED_EDGE('',*,*,#11615,.F.);
#16317=ORIENTED_EDGE('',*,*,#11616,.F.);
#16318=ORIENTED_EDGE('',*,*,#11596,.T.);
#16319=ORIENTED_EDGE('',*,*,#11617,.T.);
#16320=ORIENTED_EDGE('',*,*,#11516,.T.);
#16321=ORIENTED_EDGE('',*,*,#11593,.T.);
#16322=ORIENTED_EDGE('',*,*,#11588,.T.);
#16323=ORIENTED_EDGE('',*,*,#10193,.T.);
#16324=ORIENTED_EDGE('',*,*,#11587,.T.);
#16325=ORIENTED_EDGE('',*,*,#11586,.T.);
#16326=ORIENTED_EDGE('',*,*,#10197,.T.);
#16327=ORIENTED_EDGE('',*,*,#11618,.T.);
#16328=ORIENTED_EDGE('',*,*,#11619,.F.);
#16329=ORIENTED_EDGE('',*,*,#11620,.T.);
#16330=ORIENTED_EDGE('',*,*,#11472,.F.);
#16331=ORIENTED_EDGE('',*,*,#11621,.T.);
#16332=ORIENTED_EDGE('',*,*,#11622,.F.);
#16333=ORIENTED_EDGE('',*,*,#11618,.F.);
#16334=ORIENTED_EDGE('',*,*,#11471,.F.);
#16335=ORIENTED_EDGE('',*,*,#11623,.T.);
#16336=ORIENTED_EDGE('',*,*,#11624,.F.);
#16337=ORIENTED_EDGE('',*,*,#11621,.F.);
#16338=ORIENTED_EDGE('',*,*,#11470,.F.);
#16339=ORIENTED_EDGE('',*,*,#11625,.T.);
#16340=ORIENTED_EDGE('',*,*,#11626,.F.);
#16341=ORIENTED_EDGE('',*,*,#11623,.F.);
#16342=ORIENTED_EDGE('',*,*,#11469,.F.);
#16343=ORIENTED_EDGE('',*,*,#11627,.T.);
#16344=ORIENTED_EDGE('',*,*,#11628,.F.);
#16345=ORIENTED_EDGE('',*,*,#11625,.F.);
#16346=ORIENTED_EDGE('',*,*,#11468,.F.);
#16347=ORIENTED_EDGE('',*,*,#11620,.F.);
#16348=ORIENTED_EDGE('',*,*,#11629,.F.);
#16349=ORIENTED_EDGE('',*,*,#11627,.F.);
#16350=ORIENTED_EDGE('',*,*,#11473,.F.);
#16351=ORIENTED_EDGE('',*,*,#11630,.F.);
#16352=ORIENTED_EDGE('',*,*,#11631,.F.);
#16353=ORIENTED_EDGE('',*,*,#11615,.T.);
#16354=ORIENTED_EDGE('',*,*,#11632,.T.);
#16355=ORIENTED_EDGE('',*,*,#11633,.F.);
#16356=ORIENTED_EDGE('',*,*,#11634,.T.);
#16357=ORIENTED_EDGE('',*,*,#11635,.F.);
#16358=ORIENTED_EDGE('',*,*,#11605,.F.);
#16359=ORIENTED_EDGE('',*,*,#11632,.F.);
#16360=ORIENTED_EDGE('',*,*,#11636,.T.);
#16361=ORIENTED_EDGE('',*,*,#11637,.T.);
#16362=ORIENTED_EDGE('',*,*,#11638,.T.);
#16363=ORIENTED_EDGE('',*,*,#11639,.F.);
#16364=ORIENTED_EDGE('',*,*,#11599,.T.);
#16365=ORIENTED_EDGE('',*,*,#11635,.T.);
#16366=ORIENTED_EDGE('',*,*,#11640,.T.);
#16367=ORIENTED_EDGE('',*,*,#11641,.T.);
#16368=ORIENTED_EDGE('',*,*,#11642,.T.);
#16369=ORIENTED_EDGE('',*,*,#11478,.F.);
#16370=ORIENTED_EDGE('',*,*,#11642,.F.);
#16371=ORIENTED_EDGE('',*,*,#11643,.T.);
#16372=ORIENTED_EDGE('',*,*,#11644,.T.);
#16373=ORIENTED_EDGE('',*,*,#11479,.F.);
#16374=ORIENTED_EDGE('',*,*,#11644,.F.);
#16375=ORIENTED_EDGE('',*,*,#11645,.T.);
#16376=ORIENTED_EDGE('',*,*,#11646,.T.);
#16377=ORIENTED_EDGE('',*,*,#11474,.F.);
#16378=ORIENTED_EDGE('',*,*,#11646,.F.);
#16379=ORIENTED_EDGE('',*,*,#11647,.T.);
#16380=ORIENTED_EDGE('',*,*,#11648,.T.);
#16381=ORIENTED_EDGE('',*,*,#11475,.F.);
#16382=ORIENTED_EDGE('',*,*,#11648,.F.);
#16383=ORIENTED_EDGE('',*,*,#11649,.T.);
#16384=ORIENTED_EDGE('',*,*,#11650,.T.);
#16385=ORIENTED_EDGE('',*,*,#11476,.F.);
#16386=ORIENTED_EDGE('',*,*,#11650,.F.);
#16387=ORIENTED_EDGE('',*,*,#11651,.T.);
#16388=ORIENTED_EDGE('',*,*,#11640,.F.);
#16389=ORIENTED_EDGE('',*,*,#11477,.F.);
#16390=ORIENTED_EDGE('',*,*,#11652,.T.);
#16391=ORIENTED_EDGE('',*,*,#11482,.F.);
#16392=ORIENTED_EDGE('',*,*,#11653,.T.);
#16393=ORIENTED_EDGE('',*,*,#11654,.F.);
#16394=ORIENTED_EDGE('',*,*,#11653,.F.);
#16395=ORIENTED_EDGE('',*,*,#11481,.F.);
#16396=ORIENTED_EDGE('',*,*,#11655,.T.);
#16397=ORIENTED_EDGE('',*,*,#11656,.F.);
#16398=ORIENTED_EDGE('',*,*,#11655,.F.);
#16399=ORIENTED_EDGE('',*,*,#11480,.F.);
#16400=ORIENTED_EDGE('',*,*,#11657,.T.);
#16401=ORIENTED_EDGE('',*,*,#11658,.F.);
#16402=ORIENTED_EDGE('',*,*,#11657,.F.);
#16403=ORIENTED_EDGE('',*,*,#11485,.F.);
#16404=ORIENTED_EDGE('',*,*,#11659,.T.);
#16405=ORIENTED_EDGE('',*,*,#11660,.F.);
#16406=ORIENTED_EDGE('',*,*,#11659,.F.);
#16407=ORIENTED_EDGE('',*,*,#11484,.F.);
#16408=ORIENTED_EDGE('',*,*,#11661,.T.);
#16409=ORIENTED_EDGE('',*,*,#11662,.F.);
#16410=ORIENTED_EDGE('',*,*,#11661,.F.);
#16411=ORIENTED_EDGE('',*,*,#11483,.F.);
#16412=ORIENTED_EDGE('',*,*,#11652,.F.);
#16413=ORIENTED_EDGE('',*,*,#11663,.F.);
#16414=ORIENTED_EDGE('',*,*,#10190,.F.);
#16415=ORIENTED_EDGE('',*,*,#10232,.T.);
#16416=ORIENTED_EDGE('',*,*,#11664,.T.);
#16417=ORIENTED_EDGE('',*,*,#11665,.T.);
#16418=ORIENTED_EDGE('',*,*,#11666,.T.);
#16419=ORIENTED_EDGE('',*,*,#11667,.T.);
#16420=ORIENTED_EDGE('',*,*,#11668,.T.);
#16421=ORIENTED_EDGE('',*,*,#11669,.T.);
#16422=ORIENTED_EDGE('',*,*,#10185,.F.);
#16423=ORIENTED_EDGE('',*,*,#11488,.F.);
#16424=ORIENTED_EDGE('',*,*,#11486,.F.);
#16425=ORIENTED_EDGE('',*,*,#10218,.F.);
#16426=ORIENTED_EDGE('',*,*,#11490,.F.);
#16427=ORIENTED_EDGE('',*,*,#10220,.F.);
#16428=ORIENTED_EDGE('',*,*,#10223,.F.);
#16429=ORIENTED_EDGE('',*,*,#10226,.F.);
#16430=ORIENTED_EDGE('',*,*,#10229,.F.);
#16431=ORIENTED_EDGE('',*,*,#11670,.F.);
#16432=ORIENTED_EDGE('',*,*,#11671,.F.);
#16433=ORIENTED_EDGE('',*,*,#11672,.F.);
#16434=ORIENTED_EDGE('',*,*,#11673,.F.);
#16435=ORIENTED_EDGE('',*,*,#11674,.F.);
#16436=ORIENTED_EDGE('',*,*,#11675,.F.);
#16437=ORIENTED_EDGE('',*,*,#11676,.T.);
#16438=ORIENTED_EDGE('',*,*,#11677,.F.);
#16439=ORIENTED_EDGE('',*,*,#11670,.T.);
#16440=ORIENTED_EDGE('',*,*,#11678,.F.);
#16441=ORIENTED_EDGE('',*,*,#11679,.F.);
#16442=ORIENTED_EDGE('',*,*,#11676,.F.);
#16443=ORIENTED_EDGE('',*,*,#11680,.F.);
#16444=ORIENTED_EDGE('',*,*,#11681,.F.);
#16445=ORIENTED_EDGE('',*,*,#11682,.F.);
#16446=ORIENTED_EDGE('',*,*,#11683,.F.);
#16447=ORIENTED_EDGE('',*,*,#11684,.T.);
#16448=ORIENTED_EDGE('',*,*,#11685,.F.);
#16449=ORIENTED_EDGE('',*,*,#11682,.T.);
#16450=ORIENTED_EDGE('',*,*,#11686,.F.);
#16451=ORIENTED_EDGE('',*,*,#11687,.T.);
#16452=ORIENTED_EDGE('',*,*,#11496,.F.);
#16453=ORIENTED_EDGE('',*,*,#11688,.T.);
#16454=ORIENTED_EDGE('',*,*,#11689,.F.);
#16455=ORIENTED_EDGE('',*,*,#11688,.F.);
#16456=ORIENTED_EDGE('',*,*,#11495,.F.);
#16457=ORIENTED_EDGE('',*,*,#11690,.T.);
#16458=ORIENTED_EDGE('',*,*,#11691,.F.);
#16459=ORIENTED_EDGE('',*,*,#11690,.F.);
#16460=ORIENTED_EDGE('',*,*,#11494,.F.);
#16461=ORIENTED_EDGE('',*,*,#11692,.T.);
#16462=ORIENTED_EDGE('',*,*,#11693,.F.);
#16463=ORIENTED_EDGE('',*,*,#11692,.F.);
#16464=ORIENTED_EDGE('',*,*,#11493,.F.);
#16465=ORIENTED_EDGE('',*,*,#11694,.T.);
#16466=ORIENTED_EDGE('',*,*,#11695,.F.);
#16467=ORIENTED_EDGE('',*,*,#11694,.F.);
#16468=ORIENTED_EDGE('',*,*,#11492,.F.);
#16469=ORIENTED_EDGE('',*,*,#11696,.T.);
#16470=ORIENTED_EDGE('',*,*,#11697,.F.);
#16471=ORIENTED_EDGE('',*,*,#11696,.F.);
#16472=ORIENTED_EDGE('',*,*,#11491,.F.);
#16473=ORIENTED_EDGE('',*,*,#11687,.F.);
#16474=ORIENTED_EDGE('',*,*,#11698,.F.);
#16475=ORIENTED_EDGE('',*,*,#11699,.F.);
#16476=ORIENTED_EDGE('',*,*,#11700,.F.);
#16477=ORIENTED_EDGE('',*,*,#11701,.T.);
#16478=ORIENTED_EDGE('',*,*,#11502,.F.);
#16479=ORIENTED_EDGE('',*,*,#11702,.T.);
#16480=ORIENTED_EDGE('',*,*,#11703,.F.);
#16481=ORIENTED_EDGE('',*,*,#11702,.F.);
#16482=ORIENTED_EDGE('',*,*,#11501,.F.);
#16483=ORIENTED_EDGE('',*,*,#11704,.T.);
#16484=ORIENTED_EDGE('',*,*,#11705,.F.);
#16485=ORIENTED_EDGE('',*,*,#11704,.F.);
#16486=ORIENTED_EDGE('',*,*,#11500,.F.);
#16487=ORIENTED_EDGE('',*,*,#11706,.T.);
#16488=ORIENTED_EDGE('',*,*,#11707,.F.);
#16489=ORIENTED_EDGE('',*,*,#11706,.F.);
#16490=ORIENTED_EDGE('',*,*,#11499,.F.);
#16491=ORIENTED_EDGE('',*,*,#11708,.T.);
#16492=ORIENTED_EDGE('',*,*,#11709,.F.);
#16493=ORIENTED_EDGE('',*,*,#11710,.F.);
#16494=ORIENTED_EDGE('',*,*,#11711,.F.);
#16495=ORIENTED_EDGE('',*,*,#11708,.F.);
#16496=ORIENTED_EDGE('',*,*,#11498,.F.);
#16497=ORIENTED_EDGE('',*,*,#11712,.T.);
#16498=ORIENTED_EDGE('',*,*,#11713,.F.);
#16499=ORIENTED_EDGE('',*,*,#11712,.F.);
#16500=ORIENTED_EDGE('',*,*,#11497,.F.);
#16501=ORIENTED_EDGE('',*,*,#11701,.F.);
#16502=ORIENTED_EDGE('',*,*,#11714,.F.);
#16503=ORIENTED_EDGE('',*,*,#10182,.F.);
#16504=ORIENTED_EDGE('',*,*,#11513,.T.);
#16505=ORIENTED_EDGE('',*,*,#11514,.T.);
#16506=ORIENTED_EDGE('',*,*,#11505,.T.);
#16507=ORIENTED_EDGE('',*,*,#11507,.T.);
#16508=ORIENTED_EDGE('',*,*,#11509,.T.);
#16509=ORIENTED_EDGE('',*,*,#11511,.T.);
#16510=ORIENTED_EDGE('',*,*,#11542,.T.);
#16511=ORIENTED_EDGE('',*,*,#11591,.T.);
#16512=ORIENTED_EDGE('',*,*,#11523,.T.);
#16513=ORIENTED_EDGE('',*,*,#11715,.T.);
#16514=ORIENTED_EDGE('',*,*,#11598,.F.);
#16515=ORIENTED_EDGE('',*,*,#11716,.F.);
#16516=ORIENTED_EDGE('',*,*,#11717,.T.);
#16517=ORIENTED_EDGE('',*,*,#11521,.F.);
#16518=ORIENTED_EDGE('',*,*,#11520,.F.);
#16519=ORIENTED_EDGE('',*,*,#11517,.F.);
#16520=ORIENTED_EDGE('',*,*,#11617,.F.);
#16521=ORIENTED_EDGE('',*,*,#11534,.F.);
#16522=ORIENTED_EDGE('',*,*,#11532,.F.);
#16523=ORIENTED_EDGE('',*,*,#11530,.F.);
#16524=ORIENTED_EDGE('',*,*,#11528,.F.);
#16525=ORIENTED_EDGE('',*,*,#11526,.F.);
#16526=ORIENTED_EDGE('',*,*,#11536,.F.);
#16527=ORIENTED_EDGE('',*,*,#11718,.F.);
#16528=ORIENTED_EDGE('',*,*,#11719,.F.);
#16529=ORIENTED_EDGE('',*,*,#11720,.F.);
#16530=ORIENTED_EDGE('',*,*,#11718,.T.);
#16531=ORIENTED_EDGE('',*,*,#11721,.F.);
#16532=ORIENTED_EDGE('',*,*,#11594,.T.);
#16533=ORIENTED_EDGE('',*,*,#11540,.T.);
#16534=ORIENTED_EDGE('',*,*,#11544,.T.);
#16535=ORIENTED_EDGE('',*,*,#11722,.T.);
#16536=ORIENTED_EDGE('',*,*,#11723,.F.);
#16537=ORIENTED_EDGE('',*,*,#11555,.T.);
#16538=ORIENTED_EDGE('',*,*,#11556,.T.);
#16539=ORIENTED_EDGE('',*,*,#11546,.T.);
#16540=ORIENTED_EDGE('',*,*,#11549,.T.);
#16541=ORIENTED_EDGE('',*,*,#11551,.T.);
#16542=ORIENTED_EDGE('',*,*,#11553,.T.);
#16543=ORIENTED_EDGE('',*,*,#11724,.T.);
#16544=ORIENTED_EDGE('',*,*,#11725,.F.);
#16545=ORIENTED_EDGE('',*,*,#11726,.T.);
#16546=ORIENTED_EDGE('',*,*,#11633,.T.);
#16547=ORIENTED_EDGE('',*,*,#11604,.T.);
#16548=ORIENTED_EDGE('',*,*,#11559,.T.);
#16549=ORIENTED_EDGE('',*,*,#10211,.T.);
#16550=ORIENTED_EDGE('',*,*,#11561,.T.);
#16551=ORIENTED_EDGE('',*,*,#11560,.T.);
#16552=ORIENTED_EDGE('',*,*,#10207,.T.);
#16553=ORIENTED_EDGE('',*,*,#11568,.T.);
#16554=ORIENTED_EDGE('',*,*,#11567,.T.);
#16555=ORIENTED_EDGE('',*,*,#11570,.T.);
#16556=ORIENTED_EDGE('',*,*,#11573,.T.);
#16557=ORIENTED_EDGE('',*,*,#11575,.T.);
#16558=ORIENTED_EDGE('',*,*,#11578,.T.);
#16559=ORIENTED_EDGE('',*,*,#11579,.T.);
#16560=ORIENTED_EDGE('',*,*,#10206,.T.);
#16561=ORIENTED_EDGE('',*,*,#11581,.T.);
#16562=ORIENTED_EDGE('',*,*,#11580,.T.);
#16563=ORIENTED_EDGE('',*,*,#10195,.T.);
#16564=ORIENTED_EDGE('',*,*,#11585,.T.);
#16565=ORIENTED_EDGE('',*,*,#11584,.T.);
#16566=ORIENTED_EDGE('',*,*,#10191,.T.);
#16567=ORIENTED_EDGE('',*,*,#11590,.T.);
#16568=ORIENTED_EDGE('',*,*,#11592,.T.);
#16569=ORIENTED_EDGE('',*,*,#11595,.T.);
#16570=ORIENTED_EDGE('',*,*,#11721,.T.);
#16571=ORIENTED_EDGE('',*,*,#11720,.T.);
#16572=ORIENTED_EDGE('',*,*,#11725,.T.);
#16573=ORIENTED_EDGE('',*,*,#11727,.F.);
#16574=ORIENTED_EDGE('',*,*,#11728,.T.);
#16575=ORIENTED_EDGE('',*,*,#11729,.F.);
#16576=ORIENTED_EDGE('',*,*,#11684,.F.);
#16577=ORIENTED_EDGE('',*,*,#11730,.F.);
#16578=ORIENTED_EDGE('',*,*,#11731,.F.);
#16579=ORIENTED_EDGE('',*,*,#11732,.F.);
#16580=ORIENTED_EDGE('',*,*,#11733,.T.);
#16581=ORIENTED_EDGE('',*,*,#11716,.T.);
#16582=ORIENTED_EDGE('',*,*,#11597,.T.);
#16583=ORIENTED_EDGE('',*,*,#11734,.F.);
#16584=ORIENTED_EDGE('',*,*,#11735,.F.);
#16585=ORIENTED_EDGE('',*,*,#11734,.T.);
#16586=ORIENTED_EDGE('',*,*,#11616,.T.);
#16587=ORIENTED_EDGE('',*,*,#11736,.F.);
#16588=ORIENTED_EDGE('',*,*,#11611,.T.);
#16589=ORIENTED_EDGE('',*,*,#11600,.T.);
#16590=ORIENTED_EDGE('',*,*,#11639,.T.);
#16591=ORIENTED_EDGE('',*,*,#11737,.T.);
#16592=ORIENTED_EDGE('',*,*,#11630,.T.);
#16593=ORIENTED_EDGE('',*,*,#11614,.T.);
#16594=ORIENTED_EDGE('',*,*,#11606,.T.);
#16595=ORIENTED_EDGE('',*,*,#11610,.T.);
#16596=ORIENTED_EDGE('',*,*,#11613,.T.);
#16597=ORIENTED_EDGE('',*,*,#11738,.T.);
#16598=ORIENTED_EDGE('',*,*,#11739,.F.);
#16599=ORIENTED_EDGE('',*,*,#11628,.T.);
#16600=ORIENTED_EDGE('',*,*,#11629,.T.);
#16601=ORIENTED_EDGE('',*,*,#11619,.T.);
#16602=ORIENTED_EDGE('',*,*,#11622,.T.);
#16603=ORIENTED_EDGE('',*,*,#11624,.T.);
#16604=ORIENTED_EDGE('',*,*,#11626,.T.);
#16605=ORIENTED_EDGE('',*,*,#11740,.F.);
#16606=ORIENTED_EDGE('',*,*,#11736,.T.);
#16607=ORIENTED_EDGE('',*,*,#11631,.T.);
#16608=ORIENTED_EDGE('',*,*,#11739,.T.);
#16609=ORIENTED_EDGE('',*,*,#11741,.T.);
#16610=ORIENTED_EDGE('',*,*,#11728,.F.);
#16611=ORIENTED_EDGE('',*,*,#11742,.F.);
#16612=ORIENTED_EDGE('',*,*,#11743,.T.);
#16613=ORIENTED_EDGE('',*,*,#11637,.F.);
#16614=ORIENTED_EDGE('',*,*,#11636,.F.);
#16615=ORIENTED_EDGE('',*,*,#11634,.F.);
#16616=ORIENTED_EDGE('',*,*,#11726,.F.);
#16617=ORIENTED_EDGE('',*,*,#11649,.F.);
#16618=ORIENTED_EDGE('',*,*,#11647,.F.);
#16619=ORIENTED_EDGE('',*,*,#11645,.F.);
#16620=ORIENTED_EDGE('',*,*,#11643,.F.);
#16621=ORIENTED_EDGE('',*,*,#11641,.F.);
#16622=ORIENTED_EDGE('',*,*,#11651,.F.);
#16623=ORIENTED_EDGE('',*,*,#10169,.F.);
#16624=ORIENTED_EDGE('',*,*,#11662,.T.);
#16625=ORIENTED_EDGE('',*,*,#11663,.T.);
#16626=ORIENTED_EDGE('',*,*,#11654,.T.);
#16627=ORIENTED_EDGE('',*,*,#11656,.T.);
#16628=ORIENTED_EDGE('',*,*,#11658,.T.);
#16629=ORIENTED_EDGE('',*,*,#11660,.T.);
#16630=ORIENTED_EDGE('',*,*,#11744,.T.);
#16631=ORIENTED_EDGE('',*,*,#11669,.F.);
#16632=ORIENTED_EDGE('',*,*,#11745,.T.);
#16633=ORIENTED_EDGE('',*,*,#11746,.F.);
#16634=ORIENTED_EDGE('',*,*,#11745,.F.);
#16635=ORIENTED_EDGE('',*,*,#11668,.F.);
#16636=ORIENTED_EDGE('',*,*,#11747,.T.);
#16637=ORIENTED_EDGE('',*,*,#11748,.F.);
#16638=ORIENTED_EDGE('',*,*,#11747,.F.);
#16639=ORIENTED_EDGE('',*,*,#11667,.F.);
#16640=ORIENTED_EDGE('',*,*,#11749,.T.);
#16641=ORIENTED_EDGE('',*,*,#11750,.F.);
#16642=ORIENTED_EDGE('',*,*,#11749,.F.);
#16643=ORIENTED_EDGE('',*,*,#11666,.F.);
#16644=ORIENTED_EDGE('',*,*,#11751,.T.);
#16645=ORIENTED_EDGE('',*,*,#11752,.F.);
#16646=ORIENTED_EDGE('',*,*,#11751,.F.);
#16647=ORIENTED_EDGE('',*,*,#11665,.F.);
#16648=ORIENTED_EDGE('',*,*,#11753,.T.);
#16649=ORIENTED_EDGE('',*,*,#11754,.F.);
#16650=ORIENTED_EDGE('',*,*,#11753,.F.);
#16651=ORIENTED_EDGE('',*,*,#11664,.F.);
#16652=ORIENTED_EDGE('',*,*,#11744,.F.);
#16653=ORIENTED_EDGE('',*,*,#11755,.F.);
#16654=ORIENTED_EDGE('',*,*,#11730,.T.);
#16655=ORIENTED_EDGE('',*,*,#11686,.T.);
#16656=ORIENTED_EDGE('',*,*,#11681,.T.);
#16657=ORIENTED_EDGE('',*,*,#11756,.F.);
#16658=ORIENTED_EDGE('',*,*,#11680,.T.);
#16659=ORIENTED_EDGE('',*,*,#11678,.T.);
#16660=ORIENTED_EDGE('',*,*,#11675,.T.);
#16661=ORIENTED_EDGE('',*,*,#11757,.F.);
#16662=ORIENTED_EDGE('',*,*,#11758,.F.);
#16663=ORIENTED_EDGE('',*,*,#11759,.F.);
#16664=ORIENTED_EDGE('',*,*,#11674,.T.);
#16665=ORIENTED_EDGE('',*,*,#11760,.F.);
#16666=ORIENTED_EDGE('',*,*,#11761,.F.);
#16667=ORIENTED_EDGE('',*,*,#11760,.T.);
#16668=ORIENTED_EDGE('',*,*,#11673,.T.);
#16669=ORIENTED_EDGE('',*,*,#11762,.F.);
#16670=ORIENTED_EDGE('',*,*,#11763,.F.);
#16671=ORIENTED_EDGE('',*,*,#11762,.T.);
#16672=ORIENTED_EDGE('',*,*,#11672,.T.);
#16673=ORIENTED_EDGE('',*,*,#11764,.F.);
#16674=ORIENTED_EDGE('',*,*,#11679,.T.);
#16675=ORIENTED_EDGE('',*,*,#11765,.F.);
#16676=ORIENTED_EDGE('',*,*,#11671,.T.);
#16677=ORIENTED_EDGE('',*,*,#11677,.T.);
#16678=ORIENTED_EDGE('',*,*,#11729,.T.);
#16679=ORIENTED_EDGE('',*,*,#11766,.F.);
#16680=ORIENTED_EDGE('',*,*,#11683,.T.);
#16681=ORIENTED_EDGE('',*,*,#11685,.T.);
#16682=ORIENTED_EDGE('',*,*,#10168,.F.);
#16683=ORIENTED_EDGE('',*,*,#11697,.T.);
#16684=ORIENTED_EDGE('',*,*,#11698,.T.);
#16685=ORIENTED_EDGE('',*,*,#11689,.T.);
#16686=ORIENTED_EDGE('',*,*,#11691,.T.);
#16687=ORIENTED_EDGE('',*,*,#11693,.T.);
#16688=ORIENTED_EDGE('',*,*,#11695,.T.);
#16689=ORIENTED_EDGE('',*,*,#11711,.T.);
#16690=ORIENTED_EDGE('',*,*,#11767,.T.);
#16691=ORIENTED_EDGE('',*,*,#11703,.T.);
#16692=ORIENTED_EDGE('',*,*,#11705,.T.);
#16693=ORIENTED_EDGE('',*,*,#11707,.T.);
#16694=ORIENTED_EDGE('',*,*,#11714,.T.);
#16695=ORIENTED_EDGE('',*,*,#11700,.T.);
#16696=ORIENTED_EDGE('',*,*,#11768,.T.);
#16697=ORIENTED_EDGE('',*,*,#10174,.T.);
#16698=ORIENTED_EDGE('',*,*,#11769,.T.);
#16699=ORIENTED_EDGE('',*,*,#11709,.T.);
#16700=ORIENTED_EDGE('',*,*,#11713,.T.);
#16701=ORIENTED_EDGE('',*,*,#11770,.F.);
#16702=ORIENTED_EDGE('',*,*,#11771,.T.);
#16703=ORIENTED_EDGE('',*,*,#11772,.F.);
#16704=ORIENTED_EDGE('',*,*,#11773,.T.);
#16705=ORIENTED_EDGE('',*,*,#11774,.F.);
#16706=ORIENTED_EDGE('',*,*,#10183,.F.);
#16707=ORIENTED_EDGE('',*,*,#10180,.F.);
#16708=ORIENTED_EDGE('',*,*,#11717,.F.);
#16709=ORIENTED_EDGE('',*,*,#11733,.F.);
#16710=ORIENTED_EDGE('',*,*,#11775,.F.);
#16711=ORIENTED_EDGE('',*,*,#11776,.F.);
#16712=ORIENTED_EDGE('',*,*,#11722,.F.);
#16713=ORIENTED_EDGE('',*,*,#11543,.F.);
#16714=ORIENTED_EDGE('',*,*,#11715,.F.);
#16715=ORIENTED_EDGE('',*,*,#11522,.F.);
#16716=ORIENTED_EDGE('',*,*,#11777,.T.);
#16717=ORIENTED_EDGE('',*,*,#11778,.T.);
#16718=ORIENTED_EDGE('',*,*,#11719,.T.);
#16719=ORIENTED_EDGE('',*,*,#11723,.T.);
#16720=ORIENTED_EDGE('',*,*,#11776,.T.);
#16721=ORIENTED_EDGE('',*,*,#11779,.F.);
#16722=ORIENTED_EDGE('',*,*,#11780,.F.);
#16723=ORIENTED_EDGE('',*,*,#11724,.F.);
#16724=ORIENTED_EDGE('',*,*,#11778,.F.);
#16725=ORIENTED_EDGE('',*,*,#11781,.T.);
#16726=ORIENTED_EDGE('',*,*,#11782,.F.);
#16727=ORIENTED_EDGE('',*,*,#11783,.T.);
#16728=ORIENTED_EDGE('',*,*,#11742,.T.);
#16729=ORIENTED_EDGE('',*,*,#11727,.T.);
#16730=ORIENTED_EDGE('',*,*,#11780,.T.);
#16731=ORIENTED_EDGE('',*,*,#11784,.T.);
#16732=ORIENTED_EDGE('',*,*,#11732,.T.);
#16733=ORIENTED_EDGE('',*,*,#11735,.T.);
#16734=ORIENTED_EDGE('',*,*,#11740,.T.);
#16735=ORIENTED_EDGE('',*,*,#11785,.F.);
#16736=ORIENTED_EDGE('',*,*,#11731,.T.);
#16737=ORIENTED_EDGE('',*,*,#11786,.F.);
#16738=ORIENTED_EDGE('',*,*,#11743,.F.);
#16739=ORIENTED_EDGE('',*,*,#11783,.F.);
#16740=ORIENTED_EDGE('',*,*,#11787,.F.);
#16741=ORIENTED_EDGE('',*,*,#11741,.F.);
#16742=ORIENTED_EDGE('',*,*,#11738,.F.);
#16743=ORIENTED_EDGE('',*,*,#11612,.F.);
#16744=ORIENTED_EDGE('',*,*,#11737,.F.);
#16745=ORIENTED_EDGE('',*,*,#11638,.F.);
#16746=ORIENTED_EDGE('',*,*,#11788,.F.);
#16747=ORIENTED_EDGE('',*,*,#11789,.T.);
#16748=ORIENTED_EDGE('',*,*,#11790,.F.);
#16749=ORIENTED_EDGE('',*,*,#11791,.T.);
#16750=ORIENTED_EDGE('',*,*,#11792,.F.);
#16751=ORIENTED_EDGE('',*,*,#10163,.F.);
#16752=ORIENTED_EDGE('',*,*,#10158,.T.);
#16753=ORIENTED_EDGE('',*,*,#11793,.T.);
#16754=ORIENTED_EDGE('',*,*,#11794,.T.);
#16755=ORIENTED_EDGE('',*,*,#10162,.F.);
#16756=ORIENTED_EDGE('',*,*,#11795,.F.);
#16757=ORIENTED_EDGE('',*,*,#11796,.F.);
#16758=ORIENTED_EDGE('',*,*,#11797,.F.);
#16759=ORIENTED_EDGE('',*,*,#11798,.F.);
#16760=ORIENTED_EDGE('',*,*,#11799,.F.);
#16761=ORIENTED_EDGE('',*,*,#11800,.F.);
#16762=ORIENTED_EDGE('',*,*,#11801,.T.);
#16763=ORIENTED_EDGE('',*,*,#10156,.F.);
#16764=ORIENTED_EDGE('',*,*,#11794,.F.);
#16765=ORIENTED_EDGE('',*,*,#10188,.F.);
#16766=ORIENTED_EDGE('',*,*,#11801,.F.);
#16767=ORIENTED_EDGE('',*,*,#11802,.F.);
#16768=ORIENTED_EDGE('',*,*,#11793,.F.);
#16769=ORIENTED_EDGE('',*,*,#10157,.F.);
#16770=ORIENTED_EDGE('',*,*,#10161,.F.);
#16771=ORIENTED_EDGE('',*,*,#10152,.F.);
#16772=ORIENTED_EDGE('',*,*,#11803,.F.);
#16773=ORIENTED_EDGE('',*,*,#11795,.T.);
#16774=ORIENTED_EDGE('',*,*,#10150,.F.);
#16775=ORIENTED_EDGE('',*,*,#11754,.T.);
#16776=ORIENTED_EDGE('',*,*,#11755,.T.);
#16777=ORIENTED_EDGE('',*,*,#11746,.T.);
#16778=ORIENTED_EDGE('',*,*,#11748,.T.);
#16779=ORIENTED_EDGE('',*,*,#11750,.T.);
#16780=ORIENTED_EDGE('',*,*,#11752,.T.);
#16781=ORIENTED_EDGE('',*,*,#11804,.F.);
#16782=ORIENTED_EDGE('',*,*,#11805,.F.);
#16783=ORIENTED_EDGE('',*,*,#11806,.F.);
#16784=ORIENTED_EDGE('',*,*,#11807,.F.);
#16785=ORIENTED_EDGE('',*,*,#11808,.F.);
#16786=ORIENTED_EDGE('',*,*,#11809,.F.);
#16787=ORIENTED_EDGE('',*,*,#11806,.T.);
#16788=ORIENTED_EDGE('',*,*,#11756,.T.);
#16789=ORIENTED_EDGE('',*,*,#11810,.T.);
#16790=ORIENTED_EDGE('',*,*,#11811,.F.);
#16791=ORIENTED_EDGE('',*,*,#11812,.F.);
#16792=ORIENTED_EDGE('',*,*,#11813,.F.);
#16793=ORIENTED_EDGE('',*,*,#11814,.F.);
#16794=ORIENTED_EDGE('',*,*,#11810,.F.);
#16795=ORIENTED_EDGE('',*,*,#11812,.T.);
#16796=ORIENTED_EDGE('',*,*,#11757,.T.);
#16797=ORIENTED_EDGE('',*,*,#11815,.F.);
#16798=ORIENTED_EDGE('',*,*,#11816,.F.);
#16799=ORIENTED_EDGE('',*,*,#11817,.F.);
#16800=ORIENTED_EDGE('',*,*,#11815,.T.);
#16801=ORIENTED_EDGE('',*,*,#11818,.F.);
#16802=ORIENTED_EDGE('',*,*,#11819,.F.);
#16803=ORIENTED_EDGE('',*,*,#11820,.F.);
#16804=ORIENTED_EDGE('',*,*,#11821,.F.);
#16805=ORIENTED_EDGE('',*,*,#11818,.T.);
#16806=ORIENTED_EDGE('',*,*,#11759,.T.);
#16807=ORIENTED_EDGE('',*,*,#11822,.F.);
#16808=ORIENTED_EDGE('',*,*,#11823,.F.);
#16809=ORIENTED_EDGE('',*,*,#11824,.F.);
#16810=ORIENTED_EDGE('',*,*,#11825,.F.);
#16811=ORIENTED_EDGE('',*,*,#11826,.F.);
#16812=ORIENTED_EDGE('',*,*,#11827,.F.);
#16813=ORIENTED_EDGE('',*,*,#11820,.T.);
#16814=ORIENTED_EDGE('',*,*,#11758,.T.);
#16815=ORIENTED_EDGE('',*,*,#11761,.T.);
#16816=ORIENTED_EDGE('',*,*,#11763,.T.);
#16817=ORIENTED_EDGE('',*,*,#11828,.F.);
#16818=ORIENTED_EDGE('',*,*,#11829,.F.);
#16819=ORIENTED_EDGE('',*,*,#11830,.F.);
#16820=ORIENTED_EDGE('',*,*,#11831,.F.);
#16821=ORIENTED_EDGE('',*,*,#10187,.T.);
#16822=ORIENTED_EDGE('',*,*,#11828,.T.);
#16823=ORIENTED_EDGE('',*,*,#11764,.T.);
#16824=ORIENTED_EDGE('',*,*,#11832,.F.);
#16825=ORIENTED_EDGE('',*,*,#11833,.F.);
#16826=ORIENTED_EDGE('',*,*,#11834,.F.);
#16827=ORIENTED_EDGE('',*,*,#11835,.F.);
#16828=ORIENTED_EDGE('',*,*,#11832,.T.);
#16829=ORIENTED_EDGE('',*,*,#11836,.F.);
#16830=ORIENTED_EDGE('',*,*,#11837,.T.);
#16831=ORIENTED_EDGE('',*,*,#11838,.F.);
#16832=ORIENTED_EDGE('',*,*,#11836,.T.);
#16833=ORIENTED_EDGE('',*,*,#11765,.T.);
#16834=ORIENTED_EDGE('',*,*,#11839,.F.);
#16835=ORIENTED_EDGE('',*,*,#11840,.F.);
#16836=ORIENTED_EDGE('',*,*,#11837,.F.);
#16837=ORIENTED_EDGE('',*,*,#11841,.F.);
#16838=ORIENTED_EDGE('',*,*,#11842,.T.);
#16839=ORIENTED_EDGE('',*,*,#11843,.F.);
#16840=ORIENTED_EDGE('',*,*,#11841,.T.);
#16841=ORIENTED_EDGE('',*,*,#11766,.T.);
#16842=ORIENTED_EDGE('',*,*,#11844,.F.);
#16843=ORIENTED_EDGE('',*,*,#11845,.F.);
#16844=ORIENTED_EDGE('',*,*,#11842,.F.);
#16845=ORIENTED_EDGE('',*,*,#11846,.F.);
#16846=ORIENTED_EDGE('',*,*,#11847,.F.);
#16847=ORIENTED_EDGE('',*,*,#11848,.F.);
#16848=ORIENTED_EDGE('',*,*,#11849,.T.);
#16849=ORIENTED_EDGE('',*,*,#11850,.T.);
#16850=ORIENTED_EDGE('',*,*,#10172,.T.);
#16851=ORIENTED_EDGE('',*,*,#11851,.T.);
#16852=ORIENTED_EDGE('',*,*,#11852,.T.);
#16853=ORIENTED_EDGE('',*,*,#11853,.F.);
#16854=ORIENTED_EDGE('',*,*,#11789,.F.);
#16855=ORIENTED_EDGE('',*,*,#11854,.F.);
#16856=ORIENTED_EDGE('',*,*,#10175,.F.);
#16857=ORIENTED_EDGE('',*,*,#11768,.F.);
#16858=ORIENTED_EDGE('',*,*,#11699,.T.);
#16859=ORIENTED_EDGE('',*,*,#11767,.F.);
#16860=ORIENTED_EDGE('',*,*,#11710,.T.);
#16861=ORIENTED_EDGE('',*,*,#11769,.F.);
#16862=ORIENTED_EDGE('',*,*,#10173,.F.);
#16863=ORIENTED_EDGE('',*,*,#11850,.F.);
#16864=ORIENTED_EDGE('',*,*,#11855,.T.);
#16865=ORIENTED_EDGE('',*,*,#11856,.F.);
#16866=ORIENTED_EDGE('',*,*,#11771,.F.);
#16867=ORIENTED_EDGE('',*,*,#11857,.F.);
#16868=ORIENTED_EDGE('',*,*,#11858,.T.);
#16869=ORIENTED_EDGE('',*,*,#11859,.F.);
#16870=ORIENTED_EDGE('',*,*,#11773,.F.);
#16871=ORIENTED_EDGE('',*,*,#11860,.F.);
#16872=ORIENTED_EDGE('',*,*,#11861,.T.);
#16873=ORIENTED_EDGE('',*,*,#11862,.F.);
#16874=ORIENTED_EDGE('',*,*,#10178,.T.);
#16875=ORIENTED_EDGE('',*,*,#11863,.F.);
#16876=ORIENTED_EDGE('',*,*,#11804,.T.);
#16877=ORIENTED_EDGE('',*,*,#11864,.F.);
#16878=ORIENTED_EDGE('',*,*,#11865,.T.);
#16879=ORIENTED_EDGE('',*,*,#11857,.T.);
#16880=ORIENTED_EDGE('',*,*,#11770,.T.);
#16881=ORIENTED_EDGE('',*,*,#11856,.T.);
#16882=ORIENTED_EDGE('',*,*,#11866,.T.);
#16883=ORIENTED_EDGE('',*,*,#11860,.T.);
#16884=ORIENTED_EDGE('',*,*,#11772,.T.);
#16885=ORIENTED_EDGE('',*,*,#11859,.T.);
#16886=ORIENTED_EDGE('',*,*,#11805,.T.);
#16887=ORIENTED_EDGE('',*,*,#11863,.T.);
#16888=ORIENTED_EDGE('',*,*,#10184,.T.);
#16889=ORIENTED_EDGE('',*,*,#11774,.T.);
#16890=ORIENTED_EDGE('',*,*,#10179,.T.);
#16891=ORIENTED_EDGE('',*,*,#11862,.T.);
#16892=ORIENTED_EDGE('',*,*,#11867,.T.);
#16893=ORIENTED_EDGE('',*,*,#11868,.F.);
#16894=ORIENTED_EDGE('',*,*,#11775,.T.);
#16895=ORIENTED_EDGE('',*,*,#11786,.T.);
#16896=ORIENTED_EDGE('',*,*,#11868,.T.);
#16897=ORIENTED_EDGE('',*,*,#11869,.T.);
#16898=ORIENTED_EDGE('',*,*,#11779,.T.);
#16899=ORIENTED_EDGE('',*,*,#11784,.F.);
#16900=ORIENTED_EDGE('',*,*,#11781,.F.);
#16901=ORIENTED_EDGE('',*,*,#11777,.F.);
#16902=ORIENTED_EDGE('',*,*,#11870,.T.);
#16903=ORIENTED_EDGE('',*,*,#11871,.T.);
#16904=ORIENTED_EDGE('',*,*,#11872,.F.);
#16905=ORIENTED_EDGE('',*,*,#11782,.T.);
#16906=ORIENTED_EDGE('',*,*,#11873,.T.);
#16907=ORIENTED_EDGE('',*,*,#11874,.F.);
#16908=ORIENTED_EDGE('',*,*,#11846,.T.);
#16909=ORIENTED_EDGE('',*,*,#11785,.T.);
#16910=ORIENTED_EDGE('',*,*,#11787,.T.);
#16911=ORIENTED_EDGE('',*,*,#11872,.T.);
#16912=ORIENTED_EDGE('',*,*,#11790,.T.);
#16913=ORIENTED_EDGE('',*,*,#11875,.T.);
#16914=ORIENTED_EDGE('',*,*,#10176,.T.);
#16915=ORIENTED_EDGE('',*,*,#11854,.T.);
#16916=ORIENTED_EDGE('',*,*,#11788,.T.);
#16917=ORIENTED_EDGE('',*,*,#11853,.T.);
#16918=ORIENTED_EDGE('',*,*,#11876,.T.);
#16919=ORIENTED_EDGE('',*,*,#11877,.F.);
#16920=ORIENTED_EDGE('',*,*,#11847,.T.);
#16921=ORIENTED_EDGE('',*,*,#11874,.T.);
#16922=ORIENTED_EDGE('',*,*,#11878,.T.);
#16923=ORIENTED_EDGE('',*,*,#11879,.T.);
#16924=ORIENTED_EDGE('',*,*,#11880,.T.);
#16925=ORIENTED_EDGE('',*,*,#11851,.F.);
#16926=ORIENTED_EDGE('',*,*,#10171,.F.);
#16927=ORIENTED_EDGE('',*,*,#10177,.F.);
#16928=ORIENTED_EDGE('',*,*,#11875,.F.);
#16929=ORIENTED_EDGE('',*,*,#11791,.F.);
#16930=ORIENTED_EDGE('',*,*,#11879,.F.);
#16931=ORIENTED_EDGE('',*,*,#11881,.F.);
#16932=ORIENTED_EDGE('',*,*,#11797,.T.);
#16933=ORIENTED_EDGE('',*,*,#11796,.T.);
#16934=ORIENTED_EDGE('',*,*,#11803,.T.);
#16935=ORIENTED_EDGE('',*,*,#10155,.F.);
#16936=ORIENTED_EDGE('',*,*,#11882,.T.);
#16937=ORIENTED_EDGE('',*,*,#11881,.T.);
#16938=ORIENTED_EDGE('',*,*,#11883,.T.);
#16939=ORIENTED_EDGE('',*,*,#11884,.F.);
#16940=ORIENTED_EDGE('',*,*,#11798,.T.);
#16941=ORIENTED_EDGE('',*,*,#11885,.F.);
#16942=ORIENTED_EDGE('',*,*,#11799,.T.);
#16943=ORIENTED_EDGE('',*,*,#11884,.T.);
#16944=ORIENTED_EDGE('',*,*,#11886,.T.);
#16945=ORIENTED_EDGE('',*,*,#10164,.F.);
#16946=ORIENTED_EDGE('',*,*,#11792,.T.);
#16947=ORIENTED_EDGE('',*,*,#11802,.T.);
#16948=ORIENTED_EDGE('',*,*,#11800,.T.);
#16949=ORIENTED_EDGE('',*,*,#11885,.T.);
#16950=ORIENTED_EDGE('',*,*,#11887,.T.);
#16951=ORIENTED_EDGE('',*,*,#11888,.T.);
#16952=ORIENTED_EDGE('',*,*,#11889,.F.);
#16953=ORIENTED_EDGE('',*,*,#11890,.T.);
#16954=ORIENTED_EDGE('',*,*,#11864,.T.);
#16955=ORIENTED_EDGE('',*,*,#11809,.T.);
#16956=ORIENTED_EDGE('',*,*,#11891,.F.);
#16957=ORIENTED_EDGE('',*,*,#10140,.T.);
#16958=ORIENTED_EDGE('',*,*,#11892,.T.);
#16959=ORIENTED_EDGE('',*,*,#11893,.F.);
#16960=ORIENTED_EDGE('',*,*,#11894,.T.);
#16961=ORIENTED_EDGE('',*,*,#11889,.T.);
#16962=ORIENTED_EDGE('',*,*,#11895,.T.);
#16963=ORIENTED_EDGE('',*,*,#11891,.T.);
#16964=ORIENTED_EDGE('',*,*,#11808,.T.);
#16965=ORIENTED_EDGE('',*,*,#11896,.F.);
#16966=ORIENTED_EDGE('',*,*,#11807,.T.);
#16967=ORIENTED_EDGE('',*,*,#11811,.T.);
#16968=ORIENTED_EDGE('',*,*,#11814,.T.);
#16969=ORIENTED_EDGE('',*,*,#11897,.F.);
#16970=ORIENTED_EDGE('',*,*,#11813,.T.);
#16971=ORIENTED_EDGE('',*,*,#11816,.T.);
#16972=ORIENTED_EDGE('',*,*,#11817,.T.);
#16973=ORIENTED_EDGE('',*,*,#11898,.F.);
#16974=ORIENTED_EDGE('',*,*,#11827,.T.);
#16975=ORIENTED_EDGE('',*,*,#11899,.F.);
#16976=ORIENTED_EDGE('',*,*,#10151,.T.);
#16977=ORIENTED_EDGE('',*,*,#10148,.T.);
#16978=ORIENTED_EDGE('',*,*,#11900,.F.);
#16979=ORIENTED_EDGE('',*,*,#11819,.T.);
#16980=ORIENTED_EDGE('',*,*,#11821,.T.);
#16981=ORIENTED_EDGE('',*,*,#11901,.F.);
#16982=ORIENTED_EDGE('',*,*,#11902,.F.);
#16983=ORIENTED_EDGE('',*,*,#11826,.T.);
#16984=ORIENTED_EDGE('',*,*,#11903,.F.);
#16985=ORIENTED_EDGE('',*,*,#11904,.F.);
#16986=ORIENTED_EDGE('',*,*,#11903,.T.);
#16987=ORIENTED_EDGE('',*,*,#11825,.T.);
#16988=ORIENTED_EDGE('',*,*,#11905,.F.);
#16989=ORIENTED_EDGE('',*,*,#10137,.T.);
#16990=ORIENTED_EDGE('',*,*,#11906,.F.);
#16991=ORIENTED_EDGE('',*,*,#11905,.T.);
#16992=ORIENTED_EDGE('',*,*,#11824,.T.);
#16993=ORIENTED_EDGE('',*,*,#11907,.F.);
#16994=ORIENTED_EDGE('',*,*,#11908,.F.);
#16995=ORIENTED_EDGE('',*,*,#11909,.F.);
#16996=ORIENTED_EDGE('',*,*,#11910,.F.);
#16997=ORIENTED_EDGE('',*,*,#11823,.T.);
#16998=ORIENTED_EDGE('',*,*,#11911,.F.);
#16999=ORIENTED_EDGE('',*,*,#11912,.F.);
#17000=ORIENTED_EDGE('',*,*,#11822,.T.);
#17001=ORIENTED_EDGE('',*,*,#11913,.F.);
#17002=ORIENTED_EDGE('',*,*,#11914,.F.);
#17003=ORIENTED_EDGE('',*,*,#11913,.T.);
#17004=ORIENTED_EDGE('',*,*,#11831,.T.);
#17005=ORIENTED_EDGE('',*,*,#11915,.F.);
#17006=ORIENTED_EDGE('',*,*,#10143,.T.);
#17007=ORIENTED_EDGE('',*,*,#11916,.F.);
#17008=ORIENTED_EDGE('',*,*,#11915,.T.);
#17009=ORIENTED_EDGE('',*,*,#11830,.T.);
#17010=ORIENTED_EDGE('',*,*,#11917,.F.);
#17011=ORIENTED_EDGE('',*,*,#11829,.T.);
#17012=ORIENTED_EDGE('',*,*,#11833,.T.);
#17013=ORIENTED_EDGE('',*,*,#11835,.T.);
#17014=ORIENTED_EDGE('',*,*,#11918,.F.);
#17015=ORIENTED_EDGE('',*,*,#11840,.T.);
#17016=ORIENTED_EDGE('',*,*,#11919,.F.);
#17017=ORIENTED_EDGE('',*,*,#11834,.T.);
#17018=ORIENTED_EDGE('',*,*,#11838,.T.);
#17019=ORIENTED_EDGE('',*,*,#11845,.T.);
#17020=ORIENTED_EDGE('',*,*,#11920,.F.);
#17021=ORIENTED_EDGE('',*,*,#11839,.T.);
#17022=ORIENTED_EDGE('',*,*,#11843,.T.);
#17023=ORIENTED_EDGE('',*,*,#11921,.T.);
#17024=ORIENTED_EDGE('',*,*,#11922,.F.);
#17025=ORIENTED_EDGE('',*,*,#11848,.T.);
#17026=ORIENTED_EDGE('',*,*,#11877,.T.);
#17027=ORIENTED_EDGE('',*,*,#11923,.T.);
#17028=ORIENTED_EDGE('',*,*,#11924,.F.);
#17029=ORIENTED_EDGE('',*,*,#10146,.T.);
#17030=ORIENTED_EDGE('',*,*,#11925,.T.);
#17031=ORIENTED_EDGE('',*,*,#11926,.F.);
#17032=ORIENTED_EDGE('',*,*,#11844,.T.);
#17033=ORIENTED_EDGE('',*,*,#11922,.T.);
#17034=ORIENTED_EDGE('',*,*,#11927,.T.);
#17035=ORIENTED_EDGE('',*,*,#11924,.T.);
#17036=ORIENTED_EDGE('',*,*,#11928,.T.);
#17037=ORIENTED_EDGE('',*,*,#11929,.F.);
#17038=ORIENTED_EDGE('',*,*,#11880,.F.);
#17039=ORIENTED_EDGE('',*,*,#11878,.F.);
#17040=ORIENTED_EDGE('',*,*,#11873,.F.);
#17041=ORIENTED_EDGE('',*,*,#11871,.F.);
#17042=ORIENTED_EDGE('',*,*,#11870,.F.);
#17043=ORIENTED_EDGE('',*,*,#11869,.F.);
#17044=ORIENTED_EDGE('',*,*,#11867,.F.);
#17045=ORIENTED_EDGE('',*,*,#11861,.F.);
#17046=ORIENTED_EDGE('',*,*,#11858,.F.);
#17047=ORIENTED_EDGE('',*,*,#11866,.F.);
#17048=ORIENTED_EDGE('',*,*,#11855,.F.);
#17049=ORIENTED_EDGE('',*,*,#11865,.F.);
#17050=ORIENTED_EDGE('',*,*,#11890,.F.);
#17051=ORIENTED_EDGE('',*,*,#11894,.F.);
#17052=ORIENTED_EDGE('',*,*,#11930,.F.);
#17053=ORIENTED_EDGE('',*,*,#11931,.F.);
#17054=ORIENTED_EDGE('',*,*,#11932,.F.);
#17055=ORIENTED_EDGE('',*,*,#11928,.F.);
#17056=ORIENTED_EDGE('',*,*,#11923,.F.);
#17057=ORIENTED_EDGE('',*,*,#11876,.F.);
#17058=ORIENTED_EDGE('',*,*,#11852,.F.);
#17059=ORIENTED_EDGE('',*,*,#11849,.F.);
#17060=ORIENTED_EDGE('',*,*,#10166,.F.);
#17061=ORIENTED_EDGE('',*,*,#10154,.F.);
#17062=ORIENTED_EDGE('',*,*,#10160,.F.);
#17063=ORIENTED_EDGE('',*,*,#10165,.F.);
#17064=ORIENTED_EDGE('',*,*,#11887,.F.);
#17065=ORIENTED_EDGE('',*,*,#11886,.F.);
#17066=ORIENTED_EDGE('',*,*,#11883,.F.);
#17067=ORIENTED_EDGE('',*,*,#11882,.F.);
#17068=ORIENTED_EDGE('',*,*,#11933,.T.);
#17069=ORIENTED_EDGE('',*,*,#11934,.F.);
#17070=ORIENTED_EDGE('',*,*,#11930,.T.);
#17071=ORIENTED_EDGE('',*,*,#11893,.T.);
#17072=ORIENTED_EDGE('',*,*,#11933,.F.);
#17073=ORIENTED_EDGE('',*,*,#11892,.F.);
#17074=ORIENTED_EDGE('',*,*,#11888,.F.);
#17075=ORIENTED_EDGE('',*,*,#11895,.F.);
#17076=ORIENTED_EDGE('',*,*,#11935,.F.);
#17077=ORIENTED_EDGE('',*,*,#11936,.F.);
#17078=ORIENTED_EDGE('',*,*,#11898,.T.);
#17079=ORIENTED_EDGE('',*,*,#11900,.T.);
#17080=ORIENTED_EDGE('',*,*,#10147,.T.);
#17081=ORIENTED_EDGE('',*,*,#11899,.T.);
#17082=ORIENTED_EDGE('',*,*,#11902,.T.);
#17083=ORIENTED_EDGE('',*,*,#11937,.F.);
#17084=ORIENTED_EDGE('',*,*,#11938,.F.);
#17085=ORIENTED_EDGE('',*,*,#11935,.T.);
#17086=ORIENTED_EDGE('',*,*,#11896,.T.);
#17087=ORIENTED_EDGE('',*,*,#11897,.T.);
#17088=ORIENTED_EDGE('',*,*,#11904,.T.);
#17089=ORIENTED_EDGE('',*,*,#11906,.T.);
#17090=ORIENTED_EDGE('',*,*,#11939,.F.);
#17091=ORIENTED_EDGE('',*,*,#11940,.F.);
#17092=ORIENTED_EDGE('',*,*,#11937,.T.);
#17093=ORIENTED_EDGE('',*,*,#11901,.T.);
#17094=ORIENTED_EDGE('',*,*,#11907,.T.);
#17095=ORIENTED_EDGE('',*,*,#11910,.T.);
#17096=ORIENTED_EDGE('',*,*,#11941,.F.);
#17097=ORIENTED_EDGE('',*,*,#11942,.F.);
#17098=ORIENTED_EDGE('',*,*,#11939,.T.);
#17099=ORIENTED_EDGE('',*,*,#11943,.F.);
#17100=ORIENTED_EDGE('',*,*,#11944,.F.);
#17101=ORIENTED_EDGE('',*,*,#11941,.T.);
#17102=ORIENTED_EDGE('',*,*,#11909,.T.);
#17103=ORIENTED_EDGE('',*,*,#11945,.F.);
#17104=ORIENTED_EDGE('',*,*,#11946,.F.);
#17105=ORIENTED_EDGE('',*,*,#11943,.T.);
#17106=ORIENTED_EDGE('',*,*,#11908,.T.);
#17107=ORIENTED_EDGE('',*,*,#11912,.T.);
#17108=ORIENTED_EDGE('',*,*,#11914,.T.);
#17109=ORIENTED_EDGE('',*,*,#11916,.T.);
#17110=ORIENTED_EDGE('',*,*,#11947,.F.);
#17111=ORIENTED_EDGE('',*,*,#11948,.F.);
#17112=ORIENTED_EDGE('',*,*,#11945,.T.);
#17113=ORIENTED_EDGE('',*,*,#11911,.T.);
#17114=ORIENTED_EDGE('',*,*,#11949,.T.);
#17115=ORIENTED_EDGE('',*,*,#11950,.F.);
#17116=ORIENTED_EDGE('',*,*,#11947,.T.);
#17117=ORIENTED_EDGE('',*,*,#11917,.T.);
#17118=ORIENTED_EDGE('',*,*,#11918,.T.);
#17119=ORIENTED_EDGE('',*,*,#11919,.T.);
#17120=ORIENTED_EDGE('',*,*,#11920,.T.);
#17121=ORIENTED_EDGE('',*,*,#11926,.T.);
#17122=ORIENTED_EDGE('',*,*,#11949,.F.);
#17123=ORIENTED_EDGE('',*,*,#11925,.F.);
#17124=ORIENTED_EDGE('',*,*,#11921,.F.);
#17125=ORIENTED_EDGE('',*,*,#11927,.F.);
#17126=ORIENTED_EDGE('',*,*,#11951,.F.);
#17127=ORIENTED_EDGE('',*,*,#11952,.F.);
#17128=ORIENTED_EDGE('',*,*,#11951,.T.);
#17129=ORIENTED_EDGE('',*,*,#11929,.T.);
#17130=ORIENTED_EDGE('',*,*,#11932,.T.);
#17131=ORIENTED_EDGE('',*,*,#11953,.F.);
#17132=ORIENTED_EDGE('',*,*,#11952,.T.);
#17133=ORIENTED_EDGE('',*,*,#11953,.T.);
#17134=ORIENTED_EDGE('',*,*,#11931,.T.);
#17135=ORIENTED_EDGE('',*,*,#11934,.T.);
#17136=ORIENTED_EDGE('',*,*,#11936,.T.);
#17137=ORIENTED_EDGE('',*,*,#11938,.T.);
#17138=ORIENTED_EDGE('',*,*,#11940,.T.);
#17139=ORIENTED_EDGE('',*,*,#11942,.T.);
#17140=ORIENTED_EDGE('',*,*,#11944,.T.);
#17141=ORIENTED_EDGE('',*,*,#11946,.T.);
#17142=ORIENTED_EDGE('',*,*,#11948,.T.);
#17143=ORIENTED_EDGE('',*,*,#11950,.T.);
#17144=ORIENTED_EDGE('',*,*,#10135,.T.);
#17145=ORIENTED_EDGE('',*,*,#10138,.T.);
#17146=ORIENTED_EDGE('',*,*,#10141,.T.);
#17147=ORIENTED_EDGE('',*,*,#10144,.T.);
#17256=TOROIDAL_SURFACE('',#18853,29.0000000000007,5.00000000000101);
#17257=TOROIDAL_SURFACE('',#18858,27.0000000000009,4.99999999999874);
#17258=TOROIDAL_SURFACE('',#18864,45.5,4.00000000000009);
#17259=TOROIDAL_SURFACE('',#18870,35.0000000000004,3.99999999999933);
#17260=TOROIDAL_SURFACE('',#18905,25.3774921629995,19.9999999999997);
#17520=ADVANCED_FACE('',(#5076),#17256,.F.);
#17521=ADVANCED_FACE('',(#5077),#17257,.T.);
#17522=ADVANCED_FACE('',(#5078),#17258,.F.);
#17523=ADVANCED_FACE('',(#5079),#17259,.F.);
#17524=ADVANCED_FACE('',(#5080),#4674,.F.);
#17525=ADVANCED_FACE('',(#5081),#129,.T.);
#17526=ADVANCED_FACE('',(#5082),#130,.F.);
#17527=ADVANCED_FACE('',(#5083),#131,.T.);
#17528=ADVANCED_FACE('',(#5084),#132,.T.);
#17529=ADVANCED_FACE('',(#5085,#996),#423,.F.);
#17530=ADVANCED_FACE('',(#5086,#997),#424,.F.);
#17531=ADVANCED_FACE('',(#5087),#133,.T.);
#17532=ADVANCED_FACE('',(#5088),#134,.F.);
#17533=ADVANCED_FACE('',(#5089,#998),#425,.F.);
#17534=ADVANCED_FACE('',(#5090),#135,.F.);
#17535=ADVANCED_FACE('',(#5091),#426,.T.);
#17536=ADVANCED_FACE('',(#5092),#427,.T.);
#17537=ADVANCED_FACE('',(#5093),#428,.F.);
#17538=ADVANCED_FACE('',(#5094),#429,.F.);
#17539=ADVANCED_FACE('',(#5095),#430,.F.);
#17540=ADVANCED_FACE('',(#5096),#431,.F.);
#17541=ADVANCED_FACE('',(#5097),#432,.F.);
#17542=ADVANCED_FACE('',(#5098),#433,.F.);
#17543=ADVANCED_FACE('',(#5099),#434,.T.);
#17544=ADVANCED_FACE('',(#5100),#435,.T.);
#17545=ADVANCED_FACE('',(#5101),#188,.T.);
#17546=ADVANCED_FACE('',(#5102),#189,.T.);
#17547=ADVANCED_FACE('',(#5103),#17260,.T.);
#17548=ADVANCED_FACE('',(#5104),#4675,.F.);
#17549=ADVANCED_FACE('',(#5105),#4676,.F.);
#17550=ADVANCED_FACE('',(#5106),#4677,.F.);
#17551=ADVANCED_FACE('',(#5107),#4678,.F.);
#17552=ADVANCED_FACE('',(#5108),#4679,.T.);
#17553=ADVANCED_FACE('',(#5109),#4680,.T.);
#17554=ADVANCED_FACE('',(#5110),#136,.T.);
#17555=ADVANCED_FACE('',(#5111),#4681,.T.);
#17556=ADVANCED_FACE('',(#5112),#4682,.T.);
#17557=ADVANCED_FACE('',(#5113),#4683,.T.);
#17558=ADVANCED_FACE('',(#5114),#4684,.T.);
#17559=ADVANCED_FACE('',(#5115),#4685,.T.);
#17560=ADVANCED_FACE('',(#5116),#4686,.T.);
#17561=ADVANCED_FACE('',(#5117),#4687,.F.);
#17562=ADVANCED_FACE('',(#5118),#4688,.F.);
#17563=ADVANCED_FACE('',(#5119),#4689,.F.);
#17564=ADVANCED_FACE('',(#5120),#4690,.F.);
#17565=ADVANCED_FACE('',(#5121),#4691,.F.);
#17566=ADVANCED_FACE('',(#5122),#4692,.T.);
#17567=ADVANCED_FACE('',(#5123),#4693,.F.);
#17568=ADVANCED_FACE('',(#5124),#4694,.F.);
#17569=ADVANCED_FACE('',(#5125),#4695,.F.);
#17570=ADVANCED_FACE('',(#5126),#4696,.F.);
#17571=ADVANCED_FACE('',(#5127),#4697,.T.);
#17572=ADVANCED_FACE('',(#5128),#4698,.F.);
#17573=ADVANCED_FACE('',(#5129),#4699,.F.);
#17574=ADVANCED_FACE('',(#5130),#4700,.F.);
#17575=ADVANCED_FACE('',(#5131,#999),#137,.T.);
#17576=ADVANCED_FACE('',(#5132),#4701,.T.);
#17577=ADVANCED_FACE('',(#5133),#4702,.F.);
#17578=ADVANCED_FACE('',(#5134),#4703,.T.);
#17579=ADVANCED_FACE('',(#5135),#138,.T.);
#17580=ADVANCED_FACE('',(#5136),#4704,.F.);
#17581=ADVANCED_FACE('',(#5137),#4705,.F.);
#17582=ADVANCED_FACE('',(#5138),#4706,.F.);
#17583=ADVANCED_FACE('',(#5139),#4707,.F.);
#17584=ADVANCED_FACE('',(#5140),#4708,.T.);
#17585=ADVANCED_FACE('',(#5141),#4709,.F.);
#17586=ADVANCED_FACE('',(#5142),#4710,.F.);
#17587=ADVANCED_FACE('',(#5143),#139,.T.);
#17588=ADVANCED_FACE('',(#5144),#4711,.T.);
#17589=ADVANCED_FACE('',(#5145),#4712,.T.);
#17590=ADVANCED_FACE('',(#5146),#4713,.T.);
#17591=ADVANCED_FACE('',(#5147),#4714,.T.);
#17592=ADVANCED_FACE('',(#5148),#4715,.T.);
#17593=ADVANCED_FACE('',(#5149),#4716,.T.);
#17594=ADVANCED_FACE('',(#5150),#4717,.T.);
#17595=ADVANCED_FACE('',(#5151),#4718,.F.);
#17596=ADVANCED_FACE('',(#5152),#140,.T.);
#17597=ADVANCED_FACE('',(#5153),#141,.F.);
#17598=ADVANCED_FACE('',(#5154),#4719,.F.);
#17599=ADVANCED_FACE('',(#5155),#142,.T.);
#17600=ADVANCED_FACE('',(#5156),#4720,.T.);
#17601=ADVANCED_FACE('',(#5157),#4721,.T.);
#17602=ADVANCED_FACE('',(#5158),#143,.F.);
#17603=ADVANCED_FACE('',(#5159),#4722,.F.);
#17604=ADVANCED_FACE('',(#5160),#4723,.F.);
#17605=ADVANCED_FACE('',(#5161),#144,.F.);
#17606=ADVANCED_FACE('',(#5162),#190,.T.);
#17607=ADVANCED_FACE('',(#5163),#191,.T.);
#17608=ADVANCED_FACE('',(#5164),#192,.T.);
#17609=ADVANCED_FACE('',(#5165),#193,.F.);
#17610=ADVANCED_FACE('',(#5166),#194,.F.);
#17611=ADVANCED_FACE('',(#5167),#195,.T.);
#17612=ADVANCED_FACE('',(#5168),#196,.T.);
#17613=ADVANCED_FACE('',(#5169),#197,.T.);
#17614=ADVANCED_FACE('',(#5170),#198,.T.);
#17615=ADVANCED_FACE('',(#5171),#199,.T.);
#17616=ADVANCED_FACE('',(#5172),#200,.T.);
#17617=ADVANCED_FACE('',(#5173),#436,.T.);
#17618=ADVANCED_FACE('',(#5174),#437,.T.);
#17619=ADVANCED_FACE('',(#5175),#438,.T.);
#17620=ADVANCED_FACE('',(#5176),#439,.T.);
#17621=ADVANCED_FACE('',(#5177),#440,.T.);
#17622=ADVANCED_FACE('',(#5178),#441,.T.);
#17623=ADVANCED_FACE('',(#5179),#442,.T.);
#17624=ADVANCED_FACE('',(#5180),#443,.T.);
#17625=ADVANCED_FACE('',(#5181),#444,.T.);
#17626=ADVANCED_FACE('',(#5182),#445,.T.);
#17627=ADVANCED_FACE('',(#5183),#446,.T.);
#17628=ADVANCED_FACE('',(#5184),#447,.T.);
#17629=ADVANCED_FACE('',(#5185),#448,.T.);
#17630=ADVANCED_FACE('',(#5186),#449,.F.);
#17631=ADVANCED_FACE('',(#5187),#4724,.F.);
#17632=ADVANCED_FACE('',(#5188),#450,.F.);
#17633=ADVANCED_FACE('',(#5189),#451,.T.);
#17634=ADVANCED_FACE('',(#5190),#452,.T.);
#17635=ADVANCED_FACE('',(#5191),#453,.T.);
#17636=ADVANCED_FACE('',(#5192),#454,.T.);
#17637=ADVANCED_FACE('',(#5193),#455,.T.);
#17638=ADVANCED_FACE('',(#5194),#456,.T.);
#17639=ADVANCED_FACE('',(#5195),#457,.F.);
#17640=ADVANCED_FACE('',(#5196),#4725,.F.);
#17641=ADVANCED_FACE('',(#5197),#458,.F.);
#17642=ADVANCED_FACE('',(#5198),#459,.T.);
#17643=ADVANCED_FACE('',(#5199),#460,.T.);
#17644=ADVANCED_FACE('',(#5200),#461,.T.);
#17645=ADVANCED_FACE('',(#5201),#462,.T.);
#17646=ADVANCED_FACE('',(#5202),#463,.T.);
#17647=ADVANCED_FACE('',(#5203),#464,.T.);
#17648=ADVANCED_FACE('',(#5204),#465,.F.);
#17649=ADVANCED_FACE('',(#5205),#4726,.F.);
#17650=ADVANCED_FACE('',(#5206),#466,.F.);
#17651=ADVANCED_FACE('',(#5207),#467,.T.);
#17652=ADVANCED_FACE('',(#5208),#468,.T.);
#17653=ADVANCED_FACE('',(#5209),#469,.T.);
#17654=ADVANCED_FACE('',(#5210),#470,.T.);
#17655=ADVANCED_FACE('',(#5211),#471,.T.);
#17656=ADVANCED_FACE('',(#5212),#472,.T.);
#17657=ADVANCED_FACE('',(#5213),#473,.T.);
#17658=ADVANCED_FACE('',(#5214),#474,.F.);
#17659=ADVANCED_FACE('',(#5215),#4727,.F.);
#17660=ADVANCED_FACE('',(#5216),#475,.F.);
#17661=ADVANCED_FACE('',(#5217),#4728,.F.);
#17662=ADVANCED_FACE('',(#5218),#476,.F.);
#17663=ADVANCED_FACE('',(#5219),#4729,.F.);
#17664=ADVANCED_FACE('',(#5220),#4730,.F.);
#17665=ADVANCED_FACE('',(#5221),#4731,.F.);
#17666=ADVANCED_FACE('',(#5222),#477,.F.);
#17667=ADVANCED_FACE('',(#5223),#4732,.F.);
#17668=ADVANCED_FACE('',(#5224),#4733,.F.);
#17669=ADVANCED_FACE('',(#5225),#4734,.F.);
#17670=ADVANCED_FACE('',(#5226),#478,.F.);
#17671=ADVANCED_FACE('',(#5227),#4735,.F.);
#17672=ADVANCED_FACE('',(#5228),#4736,.F.);
#17673=ADVANCED_FACE('',(#5229),#479,.F.);
#17674=ADVANCED_FACE('',(#5230),#4737,.F.);
#17675=ADVANCED_FACE('',(#5231),#4738,.F.);
#17676=ADVANCED_FACE('',(#5232),#480,.F.);
#17677=ADVANCED_FACE('',(#5233),#481,.F.);
#17678=ADVANCED_FACE('',(#5234),#482,.F.);
#17679=ADVANCED_FACE('',(#5235),#483,.F.);
#17680=ADVANCED_FACE('',(#5236),#484,.F.);
#17681=ADVANCED_FACE('',(#5237),#485,.F.);
#17682=ADVANCED_FACE('',(#5238),#486,.F.);
#17683=ADVANCED_FACE('',(#5239),#487,.F.);
#17684=ADVANCED_FACE('',(#5240),#488,.F.);
#17685=ADVANCED_FACE('',(#5241),#489,.F.);
#17686=ADVANCED_FACE('',(#5242),#490,.F.);
#17687=ADVANCED_FACE('',(#5243),#491,.F.);
#17688=ADVANCED_FACE('',(#5244),#4739,.T.);
#17689=ADVANCED_FACE('',(#5245),#4740,.T.);
#17690=ADVANCED_FACE('',(#5246,#1000),#492,.F.);
#17691=ADVANCED_FACE('',(#5247),#4741,.T.);
#17692=ADVANCED_FACE('',(#5248,#1001),#493,.T.);
#17693=ADVANCED_FACE('',(#5249,#1002),#494,.T.);
#17694=ADVANCED_FACE('',(#5250),#4742,.T.);
#17695=ADVANCED_FACE('',(#5251,#1003),#495,.T.);
#17696=ADVANCED_FACE('',(#5252),#496,.T.);
#17697=ADVANCED_FACE('',(#5253),#4743,.T.);
#17698=ADVANCED_FACE('',(#5254),#497,.T.);
#17699=ADVANCED_FACE('',(#5255),#498,.T.);
#17700=ADVANCED_FACE('',(#5256),#4744,.T.);
#17701=ADVANCED_FACE('',(#5257),#499,.T.);
#17702=ADVANCED_FACE('',(#5258),#500,.T.);
#17703=ADVANCED_FACE('',(#5259),#4745,.T.);
#17704=ADVANCED_FACE('',(#5260),#501,.T.);
#17705=ADVANCED_FACE('',(#5261),#502,.T.);
#17706=ADVANCED_FACE('',(#5262),#4746,.T.);
#17707=ADVANCED_FACE('',(#5263),#503,.T.);
#17708=ADVANCED_FACE('',(#5264,#1004),#504,.T.);
#17709=ADVANCED_FACE('',(#5265,#1005),#505,.F.);
#17710=ADVANCED_FACE('',(#5266,#1006),#95,.T.);
#17711=ADVANCED_FACE('',(#5267,#1007),#96,.T.);
#17712=ADVANCED_FACE('',(#5268),#4747,.T.);
#17713=ADVANCED_FACE('',(#5269),#506,.T.);
#17714=ADVANCED_FACE('',(#5270),#4748,.T.);
#17715=ADVANCED_FACE('',(#5271),#507,.T.);
#17716=ADVANCED_FACE('',(#5272),#4749,.T.);
#17717=ADVANCED_FACE('',(#5273),#508,.T.);
#17718=ADVANCED_FACE('',(#5274),#4750,.T.);
#17719=ADVANCED_FACE('',(#5275),#509,.T.);
#17720=ADVANCED_FACE('',(#5276),#201,.T.);
#17721=ADVANCED_FACE('',(#5277),#202,.T.);
#17722=ADVANCED_FACE('',(#5278),#203,.T.);
#17723=ADVANCED_FACE('',(#5279),#204,.T.);
#17724=ADVANCED_FACE('',(#5280),#510,.T.);
#17725=ADVANCED_FACE('',(#5281),#205,.F.);
#17726=ADVANCED_FACE('',(#5282),#206,.F.);
#17727=ADVANCED_FACE('',(#5283),#511,.T.);
#17728=ADVANCED_FACE('',(#5284),#207,.F.);
#17729=ADVANCED_FACE('',(#5285),#208,.F.);
#17730=ADVANCED_FACE('',(#5286),#512,.T.);
#17731=ADVANCED_FACE('',(#5287),#209,.F.);
#17732=ADVANCED_FACE('',(#5288),#210,.F.);
#17733=ADVANCED_FACE('',(#5289),#513,.T.);
#17734=ADVANCED_FACE('',(#5290),#211,.F.);
#17735=ADVANCED_FACE('',(#5291),#212,.T.);
#17736=ADVANCED_FACE('',(#5292),#213,.T.);
#17737=ADVANCED_FACE('',(#5293),#214,.T.);
#17738=ADVANCED_FACE('',(#5294),#215,.T.);
#17739=ADVANCED_FACE('',(#5295),#514,.T.);
#17740=ADVANCED_FACE('',(#5296),#216,.T.);
#17741=ADVANCED_FACE('',(#5297),#217,.T.);
#17742=ADVANCED_FACE('',(#5298),#515,.T.);
#17743=ADVANCED_FACE('',(#5299),#218,.F.);
#17744=ADVANCED_FACE('',(#5300),#219,.F.);
#17745=ADVANCED_FACE('',(#5301),#516,.T.);
#17746=ADVANCED_FACE('',(#5302),#220,.F.);
#17747=ADVANCED_FACE('',(#5303),#221,.F.);
#17748=ADVANCED_FACE('',(#5304),#517,.T.);
#17749=ADVANCED_FACE('',(#5305),#222,.F.);
#17750=ADVANCED_FACE('',(#5306),#223,.F.);
#17751=ADVANCED_FACE('',(#5307),#224,.F.);
#17752=ADVANCED_FACE('',(#5308),#225,.T.);
#17753=ADVANCED_FACE('',(#5309),#226,.T.);
#17754=ADVANCED_FACE('',(#5310),#227,.T.);
#17755=ADVANCED_FACE('',(#5311),#145,.T.);
#17756=ADVANCED_FACE('',(#5312),#518,.F.);
#17757=ADVANCED_FACE('',(#5313),#248,.F.);
#17758=ADVANCED_FACE('',(#5314),#249,.F.);
#17759=ADVANCED_FACE('',(#5315),#519,.F.);
#17760=ADVANCED_FACE('',(#5316),#250,.F.);
#17761=ADVANCED_FACE('',(#5317),#251,.F.);
#17762=ADVANCED_FACE('',(#5318),#520,.F.);
#17763=ADVANCED_FACE('',(#5319),#252,.F.);
#17764=ADVANCED_FACE('',(#5320),#253,.F.);
#17765=ADVANCED_FACE('',(#5321),#521,.F.);
#17766=ADVANCED_FACE('',(#5322),#254,.F.);
#17767=ADVANCED_FACE('',(#5323),#228,.T.);
#17768=ADVANCED_FACE('',(#5324),#255,.F.);
#17769=ADVANCED_FACE('',(#5325),#229,.T.);
#17770=ADVANCED_FACE('',(#5326),#230,.T.);
#17771=ADVANCED_FACE('',(#5327),#522,.T.);
#17772=ADVANCED_FACE('',(#5328),#231,.T.);
#17773=ADVANCED_FACE('',(#5329),#232,.T.);
#17774=ADVANCED_FACE('',(#5330),#523,.T.);
#17775=ADVANCED_FACE('',(#5331),#233,.F.);
#17776=ADVANCED_FACE('',(#5332),#234,.F.);
#17777=ADVANCED_FACE('',(#5333),#524,.T.);
#17778=ADVANCED_FACE('',(#5334),#235,.F.);
#17779=ADVANCED_FACE('',(#5335),#236,.F.);
#17780=ADVANCED_FACE('',(#5336),#525,.T.);
#17781=ADVANCED_FACE('',(#5337),#237,.F.);
#17782=ADVANCED_FACE('',(#5338),#238,.F.);
#17783=ADVANCED_FACE('',(#5339),#239,.F.);
#17784=ADVANCED_FACE('',(#5340,#1008),#526,.F.);
#17785=ADVANCED_FACE('',(#5341),#146,.T.);
#17786=ADVANCED_FACE('',(#5342),#147,.T.);
#17787=ADVANCED_FACE('',(#5343),#148,.T.);
#17788=ADVANCED_FACE('',(#5344),#149,.T.);
#17789=ADVANCED_FACE('',(#5345),#150,.T.);
#17790=ADVANCED_FACE('',(#5346),#151,.T.);
#17791=ADVANCED_FACE('',(#5347),#152,.T.);
#17792=ADVANCED_FACE('',(#5348),#153,.T.);
#17793=ADVANCED_FACE('',(#5349),#154,.T.);
#17794=ADVANCED_FACE('',(#5350),#155,.T.);
#17795=ADVANCED_FACE('',(#5351),#156,.T.);
#17796=ADVANCED_FACE('',(#5352),#157,.T.);
#17797=ADVANCED_FACE('',(#5353),#158,.T.);
#17798=ADVANCED_FACE('',(#5354),#159,.T.);
#17799=ADVANCED_FACE('',(#5355),#160,.T.);
#17800=ADVANCED_FACE('',(#5356),#527,.T.);
#17801=ADVANCED_FACE('',(#5357,#1009,#1010),#528,.T.);
#17802=ADVANCED_FACE('',(#5358),#4751,.T.);
#17803=ADVANCED_FACE('',(#5359),#529,.T.);
#17804=ADVANCED_FACE('',(#5360),#4752,.T.);
#17805=ADVANCED_FACE('',(#5361),#4753,.T.);
#17806=ADVANCED_FACE('',(#5362),#4754,.T.);
#17807=ADVANCED_FACE('',(#5363),#530,.T.);
#17808=ADVANCED_FACE('',(#5364),#256,.F.);
#17809=ADVANCED_FACE('',(#5365),#257,.F.);
#17810=ADVANCED_FACE('',(#5366),#258,.F.);
#17811=ADVANCED_FACE('',(#5367),#259,.T.);
#17812=ADVANCED_FACE('',(#5368),#260,.T.);
#17813=ADVANCED_FACE('',(#5369),#261,.T.);
#17814=ADVANCED_FACE('',(#5370),#262,.T.);
#17815=ADVANCED_FACE('',(#5371),#263,.T.);
#17816=ADVANCED_FACE('',(#5372),#264,.T.);
#17817=ADVANCED_FACE('',(#5373),#265,.F.);
#17818=ADVANCED_FACE('',(#5374),#266,.F.);
#17819=ADVANCED_FACE('',(#5375),#267,.F.);
#17820=ADVANCED_FACE('',(#5376,#1011),#531,.T.);
#17821=ADVANCED_FACE('',(#5377),#532,.F.);
#17822=ADVANCED_FACE('',(#5378),#533,.F.);
#17823=ADVANCED_FACE('',(#5379),#4755,.T.);
#17824=ADVANCED_FACE('',(#5380),#4756,.T.);
#17825=ADVANCED_FACE('',(#5381),#4757,.T.);
#17826=ADVANCED_FACE('',(#5382),#4758,.T.);
#17827=ADVANCED_FACE('',(#5383),#161,.T.);
#17828=ADVANCED_FACE('',(#5384),#534,.T.);
#17829=ADVANCED_FACE('',(#5385),#535,.T.);
#17830=ADVANCED_FACE('',(#5386),#536,.T.);
#17831=ADVANCED_FACE('',(#5387),#162,.T.);
#17832=ADVANCED_FACE('',(#5388),#163,.T.);
#17833=ADVANCED_FACE('',(#5389),#164,.T.);
#17834=ADVANCED_FACE('',(#5390),#537,.T.);
#17835=ADVANCED_FACE('',(#5391),#538,.T.);
#17836=ADVANCED_FACE('',(#5392),#539,.T.);
#17837=ADVANCED_FACE('',(#5393),#165,.T.);
#17838=ADVANCED_FACE('',(#5394),#166,.T.);
#17839=ADVANCED_FACE('',(#5395),#540,.T.);
#17840=ADVANCED_FACE('',(#5396),#541,.T.);
#17841=ADVANCED_FACE('',(#5397),#542,.T.);
#17842=ADVANCED_FACE('',(#5398),#167,.T.);
#17843=ADVANCED_FACE('',(#5399),#168,.T.);
#17844=ADVANCED_FACE('',(#5400),#169,.T.);
#17845=ADVANCED_FACE('',(#5401),#543,.T.);
#17846=ADVANCED_FACE('',(#5402),#544,.T.);
#17847=ADVANCED_FACE('',(#5403),#545,.T.);
#17848=ADVANCED_FACE('',(#5404),#170,.T.);
#17849=ADVANCED_FACE('',(#5405),#171,.T.);
#17850=ADVANCED_FACE('',(#5406),#546,.F.);
#17851=ADVANCED_FACE('',(#5407),#547,.F.);
#17852=ADVANCED_FACE('',(#5408),#548,.F.);
#17853=ADVANCED_FACE('',(#5409),#549,.F.);
#17854=ADVANCED_FACE('',(#5410),#550,.F.);
#17855=ADVANCED_FACE('',(#5411),#551,.F.);
#17856=ADVANCED_FACE('',(#5412),#552,.F.);
#17857=ADVANCED_FACE('',(#5413),#553,.F.);
#17858=ADVANCED_FACE('',(#5414),#554,.F.);
#17859=ADVANCED_FACE('',(#5415),#555,.F.);
#17860=ADVANCED_FACE('',(#5416),#556,.F.);
#17861=ADVANCED_FACE('',(#5417),#557,.F.);
#17862=ADVANCED_FACE('',(#5418),#4759,.T.);
#17863=ADVANCED_FACE('',(#5419),#4760,.T.);
#17864=ADVANCED_FACE('',(#5420,#1012),#558,.F.);
#17865=ADVANCED_FACE('',(#5421),#559,.F.);
#17866=ADVANCED_FACE('',(#5422),#4761,.T.);
#17867=ADVANCED_FACE('',(#5423),#4762,.T.);
#17868=ADVANCED_FACE('',(#5424),#4763,.T.);
#17869=ADVANCED_FACE('',(#5425),#4764,.T.);
#17870=ADVANCED_FACE('',(#5426,#1013),#560,.T.);
#17871=ADVANCED_FACE('',(#5427),#4765,.T.);
#17872=ADVANCED_FACE('',(#5428,#1014),#561,.T.);
#17873=ADVANCED_FACE('',(#5429,#1015),#562,.T.);
#17874=ADVANCED_FACE('',(#5430),#563,.T.);
#17875=ADVANCED_FACE('',(#5431),#564,.T.);
#17876=ADVANCED_FACE('',(#5432),#565,.F.);
#17877=ADVANCED_FACE('',(#5433),#4766,.F.);
#17878=ADVANCED_FACE('',(#5434),#566,.T.);
#17879=ADVANCED_FACE('',(#5435,#1016),#567,.F.);
#17880=ADVANCED_FACE('',(#5436),#568,.F.);
#17881=ADVANCED_FACE('',(#5437),#569,.F.);
#17882=ADVANCED_FACE('',(#5438),#570,.F.);
#17883=ADVANCED_FACE('',(#5439),#571,.F.);
#17884=ADVANCED_FACE('',(#5440),#572,.T.);
#17885=ADVANCED_FACE('',(#5441),#573,.F.);
#17886=ADVANCED_FACE('',(#5442),#4767,.F.);
#17887=ADVANCED_FACE('',(#5443),#574,.T.);
#17888=ADVANCED_FACE('',(#5444,#1017),#575,.F.);
#17889=ADVANCED_FACE('',(#5445),#576,.T.);
#17890=ADVANCED_FACE('',(#5446),#577,.F.);
#17891=ADVANCED_FACE('',(#5447),#4768,.F.);
#17892=ADVANCED_FACE('',(#5448),#578,.T.);
#17893=ADVANCED_FACE('',(#5449,#1018),#579,.F.);
#17894=ADVANCED_FACE('',(#5450),#4769,.F.);
#17895=ADVANCED_FACE('',(#5451,#1019),#580,.F.);
#17896=ADVANCED_FACE('',(#5452),#581,.T.);
#17897=ADVANCED_FACE('',(#5453),#582,.F.);
#17898=ADVANCED_FACE('',(#5454),#583,.F.);
#17899=ADVANCED_FACE('',(#5455),#584,.F.);
#17900=ADVANCED_FACE('',(#5456,#1020),#585,.T.);
#17901=ADVANCED_FACE('',(#5457,#1021),#586,.T.);
#17902=ADVANCED_FACE('',(#5458),#4770,.T.);
#17903=ADVANCED_FACE('',(#5459),#587,.F.);
#17904=ADVANCED_FACE('',(#5460),#4771,.T.);
#17905=ADVANCED_FACE('',(#5461),#588,.F.);
#17906=ADVANCED_FACE('',(#5462),#589,.F.);
#17907=ADVANCED_FACE('',(#5463),#590,.F.);
#17908=ADVANCED_FACE('',(#5464),#4772,.T.);
#17909=ADVANCED_FACE('',(#5465),#591,.F.);
#17910=ADVANCED_FACE('',(#5466,#1022),#592,.T.);
#17911=ADVANCED_FACE('',(#5467),#4773,.T.);
#17912=ADVANCED_FACE('',(#5468),#593,.F.);
#17913=ADVANCED_FACE('',(#5469),#4774,.T.);
#17914=ADVANCED_FACE('',(#5470),#594,.F.);
#17915=ADVANCED_FACE('',(#5471),#595,.F.);
#17916=ADVANCED_FACE('',(#5472),#596,.F.);
#17917=ADVANCED_FACE('',(#5473),#4775,.T.);
#17918=ADVANCED_FACE('',(#5474),#597,.F.);
#17919=ADVANCED_FACE('',(#5475,#1023),#598,.T.);
#17920=ADVANCED_FACE('',(#5476),#4776,.T.);
#17921=ADVANCED_FACE('',(#5477),#599,.F.);
#17922=ADVANCED_FACE('',(#5478),#4777,.T.);
#17923=ADVANCED_FACE('',(#5479),#600,.F.);
#17924=ADVANCED_FACE('',(#5480),#601,.F.);
#17925=ADVANCED_FACE('',(#5481),#602,.F.);
#17926=ADVANCED_FACE('',(#5482),#4778,.T.);
#17927=ADVANCED_FACE('',(#5483),#603,.F.);
#17928=ADVANCED_FACE('',(#5484,#1024),#604,.T.);
#17929=ADVANCED_FACE('',(#5485),#4779,.T.);
#17930=ADVANCED_FACE('',(#5486),#605,.F.);
#17931=ADVANCED_FACE('',(#5487),#4780,.T.);
#17932=ADVANCED_FACE('',(#5488),#606,.F.);
#17933=ADVANCED_FACE('',(#5489),#607,.F.);
#17934=ADVANCED_FACE('',(#5490),#608,.F.);
#17935=ADVANCED_FACE('',(#5491),#4781,.T.);
#17936=ADVANCED_FACE('',(#5492),#609,.F.);
#17937=ADVANCED_FACE('',(#5493),#610,.F.);
#17938=ADVANCED_FACE('',(#5494),#611,.F.);
#17939=ADVANCED_FACE('',(#5495),#612,.F.);
#17940=ADVANCED_FACE('',(#5496),#613,.F.);
#17941=ADVANCED_FACE('',(#5497),#614,.F.);
#17942=ADVANCED_FACE('',(#5498),#615,.F.);
#17943=ADVANCED_FACE('',(#5499,#1025),#616,.T.);
#17944=ADVANCED_FACE('',(#5500,#1026),#617,.T.);
#17945=ADVANCED_FACE('',(#5501),#618,.F.);
#17946=ADVANCED_FACE('',(#5502),#619,.F.);
#17947=ADVANCED_FACE('',(#5503),#620,.F.);
#17948=ADVANCED_FACE('',(#5504),#621,.T.);
#17949=ADVANCED_FACE('',(#5505),#622,.F.);
#17950=ADVANCED_FACE('',(#5506),#623,.F.);
#17951=ADVANCED_FACE('',(#5507),#624,.F.);
#17952=ADVANCED_FACE('',(#5508),#625,.F.);
#17953=ADVANCED_FACE('',(#5509),#626,.F.);
#17954=ADVANCED_FACE('',(#5510),#627,.F.);
#17955=ADVANCED_FACE('',(#5511),#628,.F.);
#17956=ADVANCED_FACE('',(#5512),#629,.T.);
#17957=ADVANCED_FACE('',(#5513),#630,.F.);
#17958=ADVANCED_FACE('',(#5514),#631,.F.);
#17959=ADVANCED_FACE('',(#5515),#632,.F.);
#17960=ADVANCED_FACE('',(#5516),#633,.T.);
#17961=ADVANCED_FACE('',(#5517),#634,.F.);
#17962=ADVANCED_FACE('',(#5518),#635,.F.);
#17963=ADVANCED_FACE('',(#5519),#636,.F.);
#17964=ADVANCED_FACE('',(#5520),#637,.T.);
#17965=ADVANCED_FACE('',(#5521),#638,.F.);
#17966=ADVANCED_FACE('',(#5522),#639,.F.);
#17967=ADVANCED_FACE('',(#5523),#640,.F.);
#17968=ADVANCED_FACE('',(#5524),#641,.T.);
#17969=ADVANCED_FACE('',(#5525,#1027),#642,.T.);
#17970=ADVANCED_FACE('',(#5526),#643,.T.);
#17971=ADVANCED_FACE('',(#5527),#644,.T.);
#17972=ADVANCED_FACE('',(#5528),#4782,.T.);
#17973=ADVANCED_FACE('',(#5529),#645,.T.);
#17974=ADVANCED_FACE('',(#5530),#4783,.T.);
#17975=ADVANCED_FACE('',(#5531),#646,.T.);
#17976=ADVANCED_FACE('',(#5532),#4784,.T.);
#17977=ADVANCED_FACE('',(#5533),#647,.T.);
#17978=ADVANCED_FACE('',(#5534),#648,.T.);
#17979=ADVANCED_FACE('',(#5535),#4785,.T.);
#17980=ADVANCED_FACE('',(#5536),#649,.T.);
#17981=ADVANCED_FACE('',(#5537),#4786,.T.);
#17982=ADVANCED_FACE('',(#5538),#650,.T.);
#17983=ADVANCED_FACE('',(#5539),#4787,.T.);
#17984=ADVANCED_FACE('',(#5540),#651,.T.);
#17985=ADVANCED_FACE('',(#5541),#4788,.T.);
#17986=ADVANCED_FACE('',(#5542,#1028),#652,.F.);
#17987=ADVANCED_FACE('',(#5543),#653,.T.);
#17988=ADVANCED_FACE('',(#5544),#654,.T.);
#17989=ADVANCED_FACE('',(#5545,#1029),#655,.T.);
#17990=ADVANCED_FACE('',(#5546),#656,.T.);
#17991=ADVANCED_FACE('',(#5547),#4789,.T.);
#17992=ADVANCED_FACE('',(#5548),#657,.F.);
#17993=ADVANCED_FACE('',(#5549),#658,.F.);
#17994=ADVANCED_FACE('',(#5550),#659,.F.);
#17995=ADVANCED_FACE('',(#5551),#660,.F.);
#17996=ADVANCED_FACE('',(#5552),#661,.F.);
#17997=ADVANCED_FACE('',(#5553),#662,.F.);
#17998=ADVANCED_FACE('',(#5554),#4790,.F.);
#17999=ADVANCED_FACE('',(#5555),#663,.T.);
#18000=ADVANCED_FACE('',(#5556,#1030),#664,.T.);
#18001=ADVANCED_FACE('',(#5557,#1031),#665,.T.);
#18002=ADVANCED_FACE('',(#5558,#1032),#666,.T.);
#18003=ADVANCED_FACE('',(#5559,#1033),#667,.T.);
#18004=ADVANCED_FACE('',(#5560,#1034),#668,.T.);
#18005=ADVANCED_FACE('',(#5561),#4791,.T.);
#18006=ADVANCED_FACE('',(#5562),#669,.T.);
#18007=ADVANCED_FACE('',(#5563),#670,.F.);
#18008=ADVANCED_FACE('',(#5564),#671,.T.);
#18009=ADVANCED_FACE('',(#5565),#672,.T.);
#18010=ADVANCED_FACE('',(#5566),#673,.T.);
#18011=ADVANCED_FACE('',(#5567),#674,.T.);
#18012=ADVANCED_FACE('',(#5568),#675,.T.);
#18013=ADVANCED_FACE('',(#5569),#676,.T.);
#18014=ADVANCED_FACE('',(#5570),#677,.T.);
#18015=ADVANCED_FACE('',(#5571),#678,.T.);
#18016=ADVANCED_FACE('',(#5572),#679,.T.);
#18017=ADVANCED_FACE('',(#5573),#680,.T.);
#18018=ADVANCED_FACE('',(#5574),#681,.T.);
#18019=ADVANCED_FACE('',(#5575),#682,.T.);
#18020=ADVANCED_FACE('',(#5576),#683,.T.);
#18021=ADVANCED_FACE('',(#5577),#684,.T.);
#18022=ADVANCED_FACE('',(#5578),#685,.T.);
#18023=ADVANCED_FACE('',(#5579),#686,.F.);
#18024=ADVANCED_FACE('',(#5580),#687,.F.);
#18025=ADVANCED_FACE('',(#5581),#688,.F.);
#18026=ADVANCED_FACE('',(#5582),#689,.F.);
#18027=ADVANCED_FACE('',(#5583),#690,.F.);
#18028=ADVANCED_FACE('',(#5584),#691,.F.);
#18029=ADVANCED_FACE('',(#5585),#692,.T.);
#18030=ADVANCED_FACE('',(#5586),#4792,.T.);
#18031=ADVANCED_FACE('',(#5587,#1035),#693,.F.);
#18032=ADVANCED_FACE('',(#5588),#4793,.T.);
#18033=ADVANCED_FACE('',(#5589),#694,.T.);
#18034=ADVANCED_FACE('',(#5590),#695,.T.);
#18035=ADVANCED_FACE('',(#5591),#696,.T.);
#18036=ADVANCED_FACE('',(#5592),#697,.T.);
#18037=ADVANCED_FACE('',(#5593),#698,.T.);
#18038=ADVANCED_FACE('',(#5594,#1036),#699,.F.);
#18039=ADVANCED_FACE('',(#5595),#700,.F.);
#18040=ADVANCED_FACE('',(#5596),#701,.F.);
#18041=ADVANCED_FACE('',(#5597),#702,.F.);
#18042=ADVANCED_FACE('',(#5598),#703,.F.);
#18043=ADVANCED_FACE('',(#5599),#704,.F.);
#18044=ADVANCED_FACE('',(#5600),#705,.F.);
#18045=ADVANCED_FACE('',(#5601),#706,.F.);
#18046=ADVANCED_FACE('',(#5602),#707,.F.);
#18047=ADVANCED_FACE('',(#5603),#708,.F.);
#18048=ADVANCED_FACE('',(#5604),#709,.T.);
#18049=ADVANCED_FACE('',(#5605),#4794,.F.);
#18050=ADVANCED_FACE('',(#5606),#710,.T.);
#18051=ADVANCED_FACE('',(#5607),#711,.F.);
#18052=ADVANCED_FACE('',(#5608),#712,.F.);
#18053=ADVANCED_FACE('',(#5609),#713,.F.);
#18054=ADVANCED_FACE('',(#5610),#714,.F.);
#18055=ADVANCED_FACE('',(#5611),#715,.F.);
#18056=ADVANCED_FACE('',(#5612),#716,.F.);
#18057=ADVANCED_FACE('',(#5613),#4795,.F.);
#18058=ADVANCED_FACE('',(#5614),#717,.T.);
#18059=ADVANCED_FACE('',(#5615),#718,.F.);
#18060=ADVANCED_FACE('',(#5616),#719,.F.);
#18061=ADVANCED_FACE('',(#5617),#720,.F.);
#18062=ADVANCED_FACE('',(#5618),#721,.F.);
#18063=ADVANCED_FACE('',(#5619),#722,.F.);
#18064=ADVANCED_FACE('',(#5620),#723,.F.);
#18065=ADVANCED_FACE('',(#5621),#4796,.T.);
#18066=ADVANCED_FACE('',(#5622),#4797,.T.);
#18067=ADVANCED_FACE('',(#5623),#4798,.T.);
#18068=ADVANCED_FACE('',(#5624),#724,.T.);
#18069=ADVANCED_FACE('',(#5625),#4799,.T.);
#18070=ADVANCED_FACE('',(#5626,#1037),#725,.T.);
#18071=ADVANCED_FACE('',(#5627),#4800,.T.);
#18072=ADVANCED_FACE('',(#5628),#726,.T.);
#18073=ADVANCED_FACE('',(#5629),#4801,.T.);
#18074=ADVANCED_FACE('',(#5630),#4802,.T.);
#18075=ADVANCED_FACE('',(#5631),#4803,.T.);
#18076=ADVANCED_FACE('',(#5632),#727,.F.);
#18077=ADVANCED_FACE('',(#5633),#728,.T.);
#18078=ADVANCED_FACE('',(#5634),#240,.T.);
#18079=ADVANCED_FACE('',(#5635),#729,.F.);
#18080=ADVANCED_FACE('',(#5636),#730,.T.);
#18081=ADVANCED_FACE('',(#5637),#4804,.F.);
#18082=ADVANCED_FACE('',(#5638),#731,.T.);
#18083=ADVANCED_FACE('',(#5639),#4805,.T.);
#18084=ADVANCED_FACE('',(#5640),#732,.F.);
#18085=ADVANCED_FACE('',(#5641),#733,.F.);
#18086=ADVANCED_FACE('',(#5642),#734,.F.);
#18087=ADVANCED_FACE('',(#5643),#735,.F.);
#18088=ADVANCED_FACE('',(#5644),#736,.F.);
#18089=ADVANCED_FACE('',(#5645),#737,.F.);
#18090=ADVANCED_FACE('',(#5646),#241,.T.);
#18091=ADVANCED_FACE('',(#5647),#738,.T.);
#18092=ADVANCED_FACE('',(#5648),#4806,.F.);
#18093=ADVANCED_FACE('',(#5649),#739,.T.);
#18094=ADVANCED_FACE('',(#5650),#740,.F.);
#18095=ADVANCED_FACE('',(#5651),#741,.F.);
#18096=ADVANCED_FACE('',(#5652),#742,.F.);
#18097=ADVANCED_FACE('',(#5653),#743,.F.);
#18098=ADVANCED_FACE('',(#5654),#744,.F.);
#18099=ADVANCED_FACE('',(#5655),#745,.F.);
#18100=ADVANCED_FACE('',(#5656),#746,.F.);
#18101=ADVANCED_FACE('',(#5657),#747,.F.);
#18102=ADVANCED_FACE('',(#5658),#748,.F.);
#18103=ADVANCED_FACE('',(#5659),#749,.F.);
#18104=ADVANCED_FACE('',(#5660),#750,.F.);
#18105=ADVANCED_FACE('',(#5661),#751,.F.);
#18106=ADVANCED_FACE('',(#5662,#1038),#752,.T.);
#18107=ADVANCED_FACE('',(#5663),#753,.F.);
#18108=ADVANCED_FACE('',(#5664,#1039,#1040,#1041,#1042,#1043),#754,.F.);
#18109=ADVANCED_FACE('',(#5665),#755,.T.);
#18110=ADVANCED_FACE('',(#5666),#756,.T.);
#18111=ADVANCED_FACE('',(#5667),#757,.F.);
#18112=ADVANCED_FACE('',(#5668),#758,.T.);
#18113=ADVANCED_FACE('',(#5669),#759,.F.);
#18114=ADVANCED_FACE('',(#5670),#760,.F.);
#18115=ADVANCED_FACE('',(#5671),#761,.F.);
#18116=ADVANCED_FACE('',(#5672),#762,.F.);
#18117=ADVANCED_FACE('',(#5673),#763,.F.);
#18118=ADVANCED_FACE('',(#5674),#764,.F.);
#18119=ADVANCED_FACE('',(#5675),#765,.F.);
#18120=ADVANCED_FACE('',(#5676),#766,.F.);
#18121=ADVANCED_FACE('',(#5677),#767,.F.);
#18122=ADVANCED_FACE('',(#5678),#768,.F.);
#18123=ADVANCED_FACE('',(#5679),#769,.F.);
#18124=ADVANCED_FACE('',(#5680),#770,.F.);
#18125=ADVANCED_FACE('',(#5681,#1044),#771,.T.);
#18126=ADVANCED_FACE('',(#5682),#4807,.T.);
#18127=ADVANCED_FACE('',(#5683,#1045),#772,.F.);
#18128=ADVANCED_FACE('',(#5684),#242,.T.);
#18129=ADVANCED_FACE('',(#5685,#1046),#773,.T.);
#18130=ADVANCED_FACE('',(#5686),#4808,.T.);
#18131=ADVANCED_FACE('',(#5687),#243,.T.);
#18132=ADVANCED_FACE('',(#5688),#774,.F.);
#18133=ADVANCED_FACE('',(#5689),#4809,.T.);
#18134=ADVANCED_FACE('',(#5690),#775,.T.);
#18135=ADVANCED_FACE('',(#5691),#4810,.T.);
#18136=ADVANCED_FACE('',(#5692,#1047),#776,.T.);
#18137=ADVANCED_FACE('',(#5693),#4811,.T.);
#18138=ADVANCED_FACE('',(#5694,#1048),#777,.F.);
#18139=ADVANCED_FACE('',(#5695,#1049),#778,.T.);
#18140=ADVANCED_FACE('',(#5696),#779,.F.);
#18141=ADVANCED_FACE('',(#5697),#780,.F.);
#18142=ADVANCED_FACE('',(#5698),#781,.F.);
#18143=ADVANCED_FACE('',(#5699),#782,.F.);
#18144=ADVANCED_FACE('',(#5700),#783,.F.);
#18145=ADVANCED_FACE('',(#5701),#784,.F.);
#18146=ADVANCED_FACE('',(#5702),#785,.T.);
#18147=ADVANCED_FACE('',(#5703),#786,.T.);
#18148=ADVANCED_FACE('',(#5704),#787,.T.);
#18149=ADVANCED_FACE('',(#5705),#788,.T.);
#18150=ADVANCED_FACE('',(#5706),#789,.T.);
#18151=ADVANCED_FACE('',(#5707),#790,.T.);
#18152=ADVANCED_FACE('',(#5708),#791,.T.);
#18153=ADVANCED_FACE('',(#5709,#1050),#792,.T.);
#18154=ADVANCED_FACE('',(#5710),#793,.T.);
#18155=ADVANCED_FACE('',(#5711),#794,.T.);
#18156=ADVANCED_FACE('',(#5712),#795,.F.);
#18157=ADVANCED_FACE('',(#5713),#796,.F.);
#18158=ADVANCED_FACE('',(#5714),#797,.T.);
#18159=ADVANCED_FACE('',(#5715),#798,.F.);
#18160=ADVANCED_FACE('',(#5716),#4812,.T.);
#18161=ADVANCED_FACE('',(#5717),#799,.F.);
#18162=ADVANCED_FACE('',(#5718),#4813,.T.);
#18163=ADVANCED_FACE('',(#5719),#800,.T.);
#18164=ADVANCED_FACE('',(#5720),#801,.F.);
#18165=ADVANCED_FACE('',(#5721),#802,.F.);
#18166=ADVANCED_FACE('',(#5722),#803,.F.);
#18167=ADVANCED_FACE('',(#5723),#804,.T.);
#18168=ADVANCED_FACE('',(#5724),#4814,.F.);
#18169=ADVANCED_FACE('',(#5725,#1051),#805,.F.);
#18170=ADVANCED_FACE('',(#5726),#4815,.F.);
#18171=ADVANCED_FACE('',(#5727),#806,.T.);
#18172=ADVANCED_FACE('',(#5728,#1052),#807,.T.);
#18173=ADVANCED_FACE('',(#5729),#808,.F.);
#18174=ADVANCED_FACE('',(#5730),#809,.T.);
#18175=ADVANCED_FACE('',(#5731),#810,.F.);
#18176=ADVANCED_FACE('',(#5732),#811,.T.);
#18177=ADVANCED_FACE('',(#5733),#812,.T.);
#18178=ADVANCED_FACE('',(#5734),#813,.T.);
#18179=ADVANCED_FACE('',(#5735,#1053),#814,.T.);
#18180=ADVANCED_FACE('',(#5736),#815,.T.);
#18181=ADVANCED_FACE('',(#5737),#816,.T.);
#18182=ADVANCED_FACE('',(#5738),#817,.T.);
#18183=ADVANCED_FACE('',(#5739),#818,.F.);
#18184=ADVANCED_FACE('',(#5740),#819,.T.);
#18185=ADVANCED_FACE('',(#5741),#820,.F.);
#18186=ADVANCED_FACE('',(#5742),#821,.T.);
#18187=ADVANCED_FACE('',(#5743),#4816,.F.);
#18188=ADVANCED_FACE('',(#5744),#4817,.F.);
#18189=ADVANCED_FACE('',(#5745),#4818,.F.);
#18190=ADVANCED_FACE('',(#5746),#822,.T.);
#18191=ADVANCED_FACE('',(#5747),#823,.T.);
#18192=ADVANCED_FACE('',(#5748),#824,.T.);
#18193=ADVANCED_FACE('',(#5749),#825,.F.);
#18194=ADVANCED_FACE('',(#5750),#826,.T.);
#18195=ADVANCED_FACE('',(#5751),#827,.T.);
#18196=ADVANCED_FACE('',(#5752),#828,.T.);
#18197=ADVANCED_FACE('',(#5753),#4819,.F.);
#18198=ADVANCED_FACE('',(#5754),#172,.T.);
#18199=ADVANCED_FACE('',(#5755),#173,.T.);
#18200=ADVANCED_FACE('',(#5756),#174,.T.);
#18201=ADVANCED_FACE('',(#5757),#175,.T.);
#18202=ADVANCED_FACE('',(#5758,#1054),#829,.T.);
#18203=ADVANCED_FACE('',(#5759),#830,.T.);
#18204=ADVANCED_FACE('',(#5760),#831,.T.);
#18205=ADVANCED_FACE('',(#5761),#832,.T.);
#18206=ADVANCED_FACE('',(#5762),#833,.T.);
#18207=ADVANCED_FACE('',(#5763),#834,.T.);
#18208=ADVANCED_FACE('',(#5764),#835,.T.);
#18209=ADVANCED_FACE('',(#5765,#1055),#836,.T.);
#18210=ADVANCED_FACE('',(#5766),#837,.T.);
#18211=ADVANCED_FACE('',(#5767),#838,.T.);
#18212=ADVANCED_FACE('',(#5768),#839,.T.);
#18213=ADVANCED_FACE('',(#5769,#1056),#840,.T.);
#18214=ADVANCED_FACE('',(#5770),#841,.T.);
#18215=ADVANCED_FACE('',(#5771),#842,.T.);
#18216=ADVANCED_FACE('',(#5772),#843,.T.);
#18217=ADVANCED_FACE('',(#5773),#844,.T.);
#18218=ADVANCED_FACE('',(#5774,#1057),#845,.T.);
#18219=ADVANCED_FACE('',(#5775),#846,.T.);
#18220=ADVANCED_FACE('',(#5776),#847,.T.);
#18221=ADVANCED_FACE('',(#5777,#1058,#1059),#848,.F.);
#18222=ADVANCED_FACE('',(#5778),#849,.T.);
#18223=ADVANCED_FACE('',(#5779),#850,.F.);
#18224=ADVANCED_FACE('',(#5780),#851,.T.);
#18225=ADVANCED_FACE('',(#5781),#852,.T.);
#18226=ADVANCED_FACE('',(#5782),#853,.T.);
#18227=ADVANCED_FACE('',(#5783),#854,.T.);
#18228=ADVANCED_FACE('',(#5784),#855,.T.);
#18229=ADVANCED_FACE('',(#5785),#856,.T.);
#18230=ADVANCED_FACE('',(#5786),#857,.T.);
#18231=ADVANCED_FACE('',(#5787),#858,.F.);
#18232=ADVANCED_FACE('',(#5788),#859,.T.);
#18233=ADVANCED_FACE('',(#5789,#1060,#1061,#1062,#1063),#860,.T.);
#18265=CLOSED_SHELL('',(#17520,#17521,#17522,#17523,#17524,#17525,#17526,
#17527,#17528,#17529,#17530));
#18266=CLOSED_SHELL('',(#17531,#17532,#17533));
#18267=CLOSED_SHELL('',(#17534,#17535));
#18268=CLOSED_SHELL('',(#17536,#17537,#17538,#17539,#17540,#17541,#17542,
#17543,#17544));
#18269=CLOSED_SHELL('',(#17545,#17546,#17547,#17548,#17549,#17550,#17551,
#17552,#17553,#17554,#17555,#17556,#17557,#17558,#17559,#17560,#17561,#17562,
#17563,#17564,#17565,#17566,#17567,#17568,#17569,#17570,#17571,#17572,#17573,
#17574,#17575,#17576,#17577,#17578,#17579,#17580,#17581,#17582,#17583,#17584,
#17585,#17586,#17587,#17588,#17589,#17590,#17591,#17592,#17593,#17594,#17595,
#17596,#17597,#17598,#17599,#17600,#17601,#17602,#17603,#17604,#17605,#17606,
#17607,#17608,#17609,#17610,#17611,#17612,#17613,#17614,#17615,#17616,#17617,
#17618,#17619,#17620,#17621,#17622,#17623,#17624,#17625,#17626,#17627,#17628,
#17629,#17630,#17631,#17632,#17633,#17634,#17635,#17636,#17637,#17638,#17639,
#17640,#17641,#17642,#17643,#17644,#17645,#17646,#17647,#17648,#17649,#17650,
#17651,#17652,#17653,#17654,#17655,#17656,#17657,#17658,#17659,#17660,#17661,
#17662,#17663,#17664,#17665,#17666,#17667,#17668,#17669,#17670,#17671,#17672,
#17673,#17674,#17675,#17676,#17677,#17678,#17679,#17680,#17681,#17682,#17683,
#17684,#17685,#17686,#17687,#17688,#17689,#17690,#17691,#17692,#17693,#17694,
#17695,#17696,#17697,#17698,#17699,#17700,#17701,#17702,#17703,#17704,#17705,
#17706,#17707,#17708,#17709,#17710,#17711,#17712,#17713,#17714,#17715,#17716,
#17717,#17718,#17719,#17720,#17721,#17722,#17723,#17724,#17725,#17726,#17727,
#17728,#17729,#17730,#17731,#17732,#17733,#17734,#17735,#17736,#17737,#17738,
#17739,#17740,#17741,#17742,#17743,#17744,#17745,#17746,#17747,#17748,#17749,
#17750,#17751,#17752,#17753,#17754,#17755,#17756,#17757,#17758,#17759,#17760,
#17761,#17762,#17763,#17764,#17765,#17766,#17767,#17768,#17769,#17770,#17771,
#17772,#17773,#17774,#17775,#17776,#17777,#17778,#17779,#17780,#17781,#17782,
#17783,#17784,#17785,#17786,#17787,#17788,#17789,#17790,#17791,#17792,#17793,
#17794,#17795,#17796,#17797,#17798,#17799,#17800,#17801,#17802,#17803,#17804,
#17805,#17806,#17807,#17808,#17809,#17810,#17811,#17812,#17813,#17814,#17815,
#17816,#17817,#17818,#17819,#17820,#17821,#17822,#17823,#17824,#17825,#17826,
#17827,#17828,#17829,#17830,#17831,#17832,#17833,#17834,#17835,#17836,#17837,
#17838,#17839,#17840,#17841,#17842,#17843,#17844,#17845,#17846,#17847,#17848,
#17849,#17850,#17851,#17852,#17853,#17854,#17855,#17856,#17857,#17858,#17859,
#17860,#17861,#17862,#17863,#17864,#17865,#17866,#17867,#17868,#17869,#17870,
#17871,#17872,#17873,#17874,#17875,#17876,#17877,#17878,#17879,#17880,#17881,
#17882,#17883,#17884,#17885,#17886,#17887,#17888,#17889,#17890,#17891,#17892,
#17893,#17894,#17895,#17896,#17897,#17898,#17899,#17900,#17901,#17902,#17903,
#17904,#17905,#17906,#17907,#17908,#17909,#17910,#17911,#17912,#17913,#17914,
#17915,#17916,#17917,#17918,#17919,#17920,#17921,#17922,#17923,#17924,#17925,
#17926,#17927,#17928,#17929,#17930,#17931,#17932,#17933,#17934,#17935,#17936,
#17937,#17938,#17939,#17940,#17941,#17942,#17943,#17944,#17945,#17946,#17947,
#17948,#17949,#17950,#17951,#17952,#17953,#17954,#17955,#17956,#17957,#17958,
#17959,#17960,#17961,#17962,#17963,#17964,#17965,#17966,#17967,#17968,#17969,
#17970,#17971,#17972,#17973,#17974,#17975,#17976,#17977,#17978,#17979,#17980,
#17981,#17982,#17983,#17984,#17985,#17986,#17987,#17988,#17989,#17990,#17991,
#17992,#17993,#17994,#17995,#17996,#17997,#17998,#17999,#18000,#18001,#18002,
#18003,#18004,#18005,#18006,#18007,#18008,#18009,#18010,#18011,#18012,#18013,
#18014,#18015,#18016,#18017,#18018,#18019,#18020,#18021,#18022,#18023,#18024,
#18025,#18026,#18027,#18028,#18029,#18030,#18031,#18032,#18033,#18034,#18035,
#18036,#18037,#18038,#18039,#18040,#18041,#18042,#18043,#18044,#18045,#18046,
#18047,#18048,#18049,#18050,#18051,#18052,#18053,#18054,#18055,#18056,#18057,
#18058,#18059,#18060,#18061,#18062,#18063,#18064,#18065,#18066,#18067,#18068,
#18069,#18070,#18071,#18072,#18073,#18074,#18075,#18076,#18077,#18078,#18079,
#18080,#18081,#18082,#18083,#18084,#18085,#18086,#18087,#18088,#18089,#18090,
#18091,#18092,#18093,#18094,#18095,#18096,#18097,#18098,#18099,#18100,#18101,
#18102,#18103,#18104,#18105,#18106,#18107,#18108,#18109,#18110,#18111,#18112,
#18113,#18114,#18115,#18116,#18117,#18118,#18119,#18120,#18121,#18122,#18123,
#18124,#18125,#18126,#18127,#18128,#18129,#18130,#18131,#18132,#18133,#18134,
#18135,#18136,#18137,#18138,#18139,#18140,#18141,#18142,#18143,#18144,#18145,
#18146,#18147,#18148,#18149,#18150,#18151,#18152,#18153,#18154,#18155,#18156,
#18157,#18158,#18159,#18160,#18161,#18162,#18163,#18164,#18165,#18166,#18167,
#18168,#18169,#18170,#18171,#18172,#18173,#18174,#18175,#18176,#18177,#18178,
#18179,#18180,#18181,#18182,#18183,#18184,#18185,#18186,#18187,#18188,#18189,
#18190,#18191,#18192,#18193,#18194,#18195,#18196,#18197,#18198,#18199,#18200,
#18201,#18202,#18203,#18204,#18205,#18206,#18207,#18208,#18209,#18210,#18211,
#18212,#18213,#18214,#18215,#18216,#18217,#18218,#18219,#18220,#18221,#18222,
#18223,#18224,#18225,#18226,#18227,#18228,#18229,#18230,#18231,#18232,#18233));
#18852=AXIS2_PLACEMENT_3D('',#30602,#21398,#21399);
#18853=AXIS2_PLACEMENT_3D('',#30603,#21400,#21401);
#18854=AXIS2_PLACEMENT_3D('',#30605,#21402,#21403);
#18855=AXIS2_PLACEMENT_3D('',#30607,#21404,#21405);
#18856=AXIS2_PLACEMENT_3D('',#30609,#21406,#21407);
#18857=AXIS2_PLACEMENT_3D('',#30610,#21408,#21409);
#18858=AXIS2_PLACEMENT_3D('',#30611,#21410,#21411);
#18859=AXIS2_PLACEMENT_3D('',#30614,#21412,#21413);
#18860=AXIS2_PLACEMENT_3D('',#30616,#21414,#21415);
#18861=AXIS2_PLACEMENT_3D('',#30618,#21416,#21417);
#18862=AXIS2_PLACEMENT_3D('',#30619,#21418,#21419);
#18863=AXIS2_PLACEMENT_3D('',#30620,#21420,#21421);
#18864=AXIS2_PLACEMENT_3D('',#30621,#21422,#21423);
#18865=AXIS2_PLACEMENT_3D('',#30624,#21424,#21425);
#18866=AXIS2_PLACEMENT_3D('',#30626,#21426,#21427);
#18867=AXIS2_PLACEMENT_3D('',#30628,#21428,#21429);
#18868=AXIS2_PLACEMENT_3D('',#30629,#21430,#21431);
#18869=AXIS2_PLACEMENT_3D('',#30630,#21432,#21433);
#18870=AXIS2_PLACEMENT_3D('',#30631,#21434,#21435);
#18871=AXIS2_PLACEMENT_3D('',#30634,#21436,#21437);
#18872=AXIS2_PLACEMENT_3D('',#30636,#21438,#21439);
#18873=AXIS2_PLACEMENT_3D('',#30638,#21440,#21441);
#18874=AXIS2_PLACEMENT_3D('',#30639,#21442,#21443);
#18875=AXIS2_PLACEMENT_3D('',#30640,#21444,#21445);
#18876=AXIS2_PLACEMENT_3D('',#30641,#21446,#21447);
#18877=AXIS2_PLACEMENT_3D('',#30643,#21448,#21449);
#18878=AXIS2_PLACEMENT_3D('',#30646,#21451,#21452);
#18879=AXIS2_PLACEMENT_3D('',#30647,#21453,#21454);
#18880=AXIS2_PLACEMENT_3D('',#30649,#21456,#21457);
#18881=AXIS2_PLACEMENT_3D('',#30652,#21459,#21460);
#18882=AXIS2_PLACEMENT_3D('',#30653,#21461,#21462);
#18883=AXIS2_PLACEMENT_3D('',#30655,#21464,#21465);
#18884=AXIS2_PLACEMENT_3D('',#30657,#21467,#21468);
#18885=AXIS2_PLACEMENT_3D('',#30658,#21469,#21470);
#18886=AXIS2_PLACEMENT_3D('',#30659,#21471,#21472);
#18887=AXIS2_PLACEMENT_3D('',#30662,#21473,#21474);
#18888=AXIS2_PLACEMENT_3D('',#30663,#21475,#21476);
#18889=AXIS2_PLACEMENT_3D('',#30666,#21478,#21479);
#18890=AXIS2_PLACEMENT_3D('',#30667,#21480,#21481);
#18891=AXIS2_PLACEMENT_3D('',#30670,#21483,#21484);
#18892=AXIS2_PLACEMENT_3D('',#30671,#21485,#21486);
#18893=AXIS2_PLACEMENT_3D('',#30672,#21487,#21488);
#18894=AXIS2_PLACEMENT_3D('',#30676,#21490,#21491);
#18895=AXIS2_PLACEMENT_3D('',#30677,#21492,#21493);
#18896=AXIS2_PLACEMENT_3D('',#30678,#21494,#21495);
#18897=AXIS2_PLACEMENT_3D('',#30691,#21502,#21503);
#18898=AXIS2_PLACEMENT_3D('',#30697,#21507,#21508);
#18899=AXIS2_PLACEMENT_3D('',#30701,#21511,#21512);
#18900=AXIS2_PLACEMENT_3D('',#30707,#21516,#21517);
#18901=AXIS2_PLACEMENT_3D('',#30711,#21520,#21521);
#18902=AXIS2_PLACEMENT_3D('',#30715,#21524,#21525);
#18903=AXIS2_PLACEMENT_3D('',#30719,#21528,#21529);
#18904=AXIS2_PLACEMENT_3D('',#30721,#21531,#21532);
#18905=AXIS2_PLACEMENT_3D('',#30788,#21536,#21537);
#18906=AXIS2_PLACEMENT_3D('',#30790,#21538,#21539);
#18907=AXIS2_PLACEMENT_3D('',#30792,#21540,#21541);
#18908=AXIS2_PLACEMENT_3D('',#30794,#21542,#21543);
#18909=AXIS2_PLACEMENT_3D('',#30795,#21544,#21545);
#18910=AXIS2_PLACEMENT_3D('',#30796,#21546,#21547);
#18911=AXIS2_PLACEMENT_3D('',#30798,#21548,#21549);
#18912=AXIS2_PLACEMENT_3D('',#30801,#21551,#21552);
#18913=AXIS2_PLACEMENT_3D('',#30802,#21553,#21554);
#18914=AXIS2_PLACEMENT_3D('',#30804,#21555,#21556);
#18915=AXIS2_PLACEMENT_3D('',#30807,#21558,#21559);
#18916=AXIS2_PLACEMENT_3D('',#30808,#21560,#21561);
#18917=AXIS2_PLACEMENT_3D('',#30810,#21562,#21563);
#18918=AXIS2_PLACEMENT_3D('',#30813,#21565,#21566);
#18919=AXIS2_PLACEMENT_3D('',#30814,#21567,#21568);
#18920=AXIS2_PLACEMENT_3D('',#30816,#21569,#21570);
#18921=AXIS2_PLACEMENT_3D('',#30819,#21572,#21573);
#18922=AXIS2_PLACEMENT_3D('',#30820,#21574,#21575);
#18923=AXIS2_PLACEMENT_3D('',#30823,#21576,#21577);
#18924=AXIS2_PLACEMENT_3D('',#30825,#21578,#21579);
#18925=AXIS2_PLACEMENT_3D('',#30828,#21581,#21582);
#18926=AXIS2_PLACEMENT_3D('',#30829,#21583,#21584);
#18927=AXIS2_PLACEMENT_3D('',#30830,#21585,#21586);
#18928=AXIS2_PLACEMENT_3D('',#30833,#21587,#21588);
#18929=AXIS2_PLACEMENT_3D('',#30840,#21589,#21590);
#18930=AXIS2_PLACEMENT_3D('',#30845,#21591,#21592);
#18931=AXIS2_PLACEMENT_3D('',#30848,#21593,#21594);
#18932=AXIS2_PLACEMENT_3D('',#30859,#21595,#21596);
#18933=AXIS2_PLACEMENT_3D('',#30865,#21597,#21598);
#18934=AXIS2_PLACEMENT_3D('',#30867,#21599,#21600);
#18935=AXIS2_PLACEMENT_3D('',#30874,#21601,#21602);
#18936=AXIS2_PLACEMENT_3D('',#30876,#21603,#21604);
#18937=AXIS2_PLACEMENT_3D('',#30882,#21605,#21606);
#18938=AXIS2_PLACEMENT_3D('',#30883,#21607,#21608);
#18939=AXIS2_PLACEMENT_3D('',#30885,#21609,#21610);
#18940=AXIS2_PLACEMENT_3D('',#30888,#21612,#21613);
#18941=AXIS2_PLACEMENT_3D('',#30889,#21614,#21615);
#18942=AXIS2_PLACEMENT_3D('',#30891,#21616,#21617);
#18943=AXIS2_PLACEMENT_3D('',#30902,#21619,#21620);
#18944=AXIS2_PLACEMENT_3D('',#30911,#21621,#21622);
#18945=AXIS2_PLACEMENT_3D('',#30920,#21623,#21624);
#18946=AXIS2_PLACEMENT_3D('',#30927,#21625,#21626);
#18947=AXIS2_PLACEMENT_3D('',#30930,#21627,#21628);
#18948=AXIS2_PLACEMENT_3D('',#30932,#21629,#21630);
#18949=AXIS2_PLACEMENT_3D('',#30934,#21631,#21632);
#18950=AXIS2_PLACEMENT_3D('',#30937,#21634,#21635);
#18951=AXIS2_PLACEMENT_3D('',#30939,#21636,#21637);
#18952=AXIS2_PLACEMENT_3D('',#30940,#21638,#21639);
#18953=AXIS2_PLACEMENT_3D('',#30941,#21640,#21641);
#18954=AXIS2_PLACEMENT_3D('',#30943,#21642,#21643);
#18955=AXIS2_PLACEMENT_3D('',#30946,#21645,#21646);
#18956=AXIS2_PLACEMENT_3D('',#30947,#21647,#21648);
#18957=AXIS2_PLACEMENT_3D('',#30949,#21649,#21650);
#18958=AXIS2_PLACEMENT_3D('',#30952,#21652,#21653);
#18959=AXIS2_PLACEMENT_3D('',#30953,#21654,#21655);
#18960=AXIS2_PLACEMENT_3D('',#30996,#21658,#21659);
#18961=AXIS2_PLACEMENT_3D('',#31039,#21662,#21663);
#18962=AXIS2_PLACEMENT_3D('',#31042,#21664,#21665);
#18963=AXIS2_PLACEMENT_3D('',#31060,#21667,#21668);
#18964=AXIS2_PLACEMENT_3D('',#31080,#21670,#21671);
#18965=AXIS2_PLACEMENT_3D('',#31104,#21673,#21674);
#18966=AXIS2_PLACEMENT_3D('',#31106,#21676,#21677);
#18967=AXIS2_PLACEMENT_3D('',#31149,#21680,#21681);
#18968=AXIS2_PLACEMENT_3D('',#31152,#21682,#21683);
#18969=AXIS2_PLACEMENT_3D('',#31154,#21684,#21685);
#18970=AXIS2_PLACEMENT_3D('',#31158,#21687,#21688);
#18971=AXIS2_PLACEMENT_3D('',#31160,#21690,#21691);
#18972=AXIS2_PLACEMENT_3D('',#31162,#21692,#21693);
#18973=AXIS2_PLACEMENT_3D('',#31165,#21695,#21696);
#18974=AXIS2_PLACEMENT_3D('',#31166,#21697,#21698);
#18975=AXIS2_PLACEMENT_3D('',#31168,#21699,#21700);
#18976=AXIS2_PLACEMENT_3D('',#31171,#21702,#21703);
#18977=AXIS2_PLACEMENT_3D('',#31172,#21704,#21705);
#18978=AXIS2_PLACEMENT_3D('',#31174,#21706,#21707);
#18979=AXIS2_PLACEMENT_3D('',#31177,#21709,#21710);
#18980=AXIS2_PLACEMENT_3D('',#31178,#21711,#21712);
#18981=AXIS2_PLACEMENT_3D('',#31180,#21713,#21714);
#18982=AXIS2_PLACEMENT_3D('',#31183,#21716,#21717);
#18983=AXIS2_PLACEMENT_3D('',#31184,#21718,#21719);
#18984=AXIS2_PLACEMENT_3D('',#31186,#21720,#21721);
#18985=AXIS2_PLACEMENT_3D('',#31189,#21723,#21724);
#18986=AXIS2_PLACEMENT_3D('',#31190,#21725,#21726);
#18987=AXIS2_PLACEMENT_3D('',#31193,#21727,#21728);
#18988=AXIS2_PLACEMENT_3D('',#31216,#21731,#21732);
#18989=AXIS2_PLACEMENT_3D('',#31219,#21733,#21734);
#18990=AXIS2_PLACEMENT_3D('',#31244,#21737,#21738);
#18991=AXIS2_PLACEMENT_3D('',#31246,#21739,#21740);
#18992=AXIS2_PLACEMENT_3D('',#31250,#21742,#21743);
#18993=AXIS2_PLACEMENT_3D('',#31265,#21745,#21746);
#18994=AXIS2_PLACEMENT_3D('',#31268,#21747,#21748);
#18995=AXIS2_PLACEMENT_3D('',#31274,#21749,#21750);
#18996=AXIS2_PLACEMENT_3D('',#31280,#21751,#21752);
#18997=AXIS2_PLACEMENT_3D('',#31286,#21753,#21754);
#18998=AXIS2_PLACEMENT_3D('',#31292,#21755,#21756);
#18999=AXIS2_PLACEMENT_3D('',#31306,#21758,#21759);
#19000=AXIS2_PLACEMENT_3D('',#31312,#21760,#21761);
#19001=AXIS2_PLACEMENT_3D('',#31318,#21762,#21763);
#19002=AXIS2_PLACEMENT_3D('',#31324,#21764,#21765);
#19003=AXIS2_PLACEMENT_3D('',#31360,#21766,#21767);
#19004=AXIS2_PLACEMENT_3D('',#31363,#21768,#21769);
#19005=AXIS2_PLACEMENT_3D('',#31365,#21770,#21771);
#19006=AXIS2_PLACEMENT_3D('',#31368,#21773,#21774);
#19007=AXIS2_PLACEMENT_3D('',#31369,#21775,#21776);
#19008=AXIS2_PLACEMENT_3D('',#31370,#21777,#21778);
#19009=AXIS2_PLACEMENT_3D('',#31371,#21779,#21780);
#19010=AXIS2_PLACEMENT_3D('',#31374,#21781,#21782);
#19011=AXIS2_PLACEMENT_3D('',#31378,#21784,#21785);
#19012=AXIS2_PLACEMENT_3D('',#31380,#21787,#21788);
#19013=AXIS2_PLACEMENT_3D('',#31383,#21789,#21790);
#19014=AXIS2_PLACEMENT_3D('',#31387,#21792,#21793);
#19015=AXIS2_PLACEMENT_3D('',#31392,#21796,#21797);
#19016=AXIS2_PLACEMENT_3D('',#31394,#21799,#21800);
#19017=AXIS2_PLACEMENT_3D('',#31397,#21802,#21803);
#19018=AXIS2_PLACEMENT_3D('',#31398,#21804,#21805);
#19019=AXIS2_PLACEMENT_3D('',#31400,#21806,#21807);
#19020=AXIS2_PLACEMENT_3D('',#31403,#21809,#21810);
#19021=AXIS2_PLACEMENT_3D('',#31404,#21811,#21812);
#19022=AXIS2_PLACEMENT_3D('',#31406,#21813,#21814);
#19023=AXIS2_PLACEMENT_3D('',#31409,#21816,#21817);
#19024=AXIS2_PLACEMENT_3D('',#31410,#21818,#21819);
#19025=AXIS2_PLACEMENT_3D('',#31412,#21820,#21821);
#19026=AXIS2_PLACEMENT_3D('',#31415,#21823,#21824);
#19027=AXIS2_PLACEMENT_3D('',#31416,#21825,#21826);
#19028=AXIS2_PLACEMENT_3D('',#31418,#21827,#21828);
#19029=AXIS2_PLACEMENT_3D('',#31421,#21830,#21831);
#19030=AXIS2_PLACEMENT_3D('',#31422,#21832,#21833);
#19031=AXIS2_PLACEMENT_3D('',#31424,#21834,#21835);
#19032=AXIS2_PLACEMENT_3D('',#31428,#21837,#21838);
#19033=AXIS2_PLACEMENT_3D('',#31432,#21840,#21841);
#19034=AXIS2_PLACEMENT_3D('',#31435,#21843,#21844);
#19035=AXIS2_PLACEMENT_3D('',#31437,#21845,#21846);
#19036=AXIS2_PLACEMENT_3D('',#31440,#21848,#21849);
#19037=AXIS2_PLACEMENT_3D('',#31441,#21850,#21851);
#19038=AXIS2_PLACEMENT_3D('',#31443,#21852,#21853);
#19039=AXIS2_PLACEMENT_3D('',#31446,#21855,#21856);
#19040=AXIS2_PLACEMENT_3D('',#31447,#21857,#21858);
#19041=AXIS2_PLACEMENT_3D('',#31449,#21859,#21860);
#19042=AXIS2_PLACEMENT_3D('',#31452,#21862,#21863);
#19043=AXIS2_PLACEMENT_3D('',#31453,#21864,#21865);
#19044=AXIS2_PLACEMENT_3D('',#31456,#21867,#21868);
#19045=AXIS2_PLACEMENT_3D('',#31457,#21869,#21870);
#19046=AXIS2_PLACEMENT_3D('',#31459,#21871,#21872);
#19047=AXIS2_PLACEMENT_3D('',#31462,#21874,#21875);
#19048=AXIS2_PLACEMENT_3D('',#31463,#21876,#21877);
#19049=AXIS2_PLACEMENT_3D('',#31465,#21878,#21879);
#19050=AXIS2_PLACEMENT_3D('',#31468,#21881,#21882);
#19051=AXIS2_PLACEMENT_3D('',#31469,#21883,#21884);
#19052=AXIS2_PLACEMENT_3D('',#31471,#21885,#21886);
#19053=AXIS2_PLACEMENT_3D('',#31474,#21888,#21889);
#19054=AXIS2_PLACEMENT_3D('',#31475,#21890,#21891);
#19055=AXIS2_PLACEMENT_3D('',#31477,#21892,#21893);
#19056=AXIS2_PLACEMENT_3D('',#31480,#21895,#21896);
#19057=AXIS2_PLACEMENT_3D('',#31481,#21897,#21898);
#19058=AXIS2_PLACEMENT_3D('',#31483,#21899,#21900);
#19059=AXIS2_PLACEMENT_3D('',#31486,#21902,#21903);
#19060=AXIS2_PLACEMENT_3D('',#31487,#21904,#21905);
#19061=AXIS2_PLACEMENT_3D('',#31489,#21906,#21907);
#19062=AXIS2_PLACEMENT_3D('',#31492,#21909,#21910);
#19063=AXIS2_PLACEMENT_3D('',#31493,#21911,#21912);
#19064=AXIS2_PLACEMENT_3D('',#31496,#21913,#21914);
#19065=AXIS2_PLACEMENT_3D('',#31500,#21916,#21917);
#19066=AXIS2_PLACEMENT_3D('',#31502,#21919,#21920);
#19067=AXIS2_PLACEMENT_3D('',#31506,#21922,#21923);
#19068=AXIS2_PLACEMENT_3D('',#31507,#21924,#21925);
#19069=AXIS2_PLACEMENT_3D('',#31508,#21926,#21927);
#19070=AXIS2_PLACEMENT_3D('',#31511,#21928,#21929);
#19071=AXIS2_PLACEMENT_3D('',#31515,#21931,#21932);
#19072=AXIS2_PLACEMENT_3D('',#31517,#21934,#21935);
#19073=AXIS2_PLACEMENT_3D('',#31520,#21936,#21937);
#19074=AXIS2_PLACEMENT_3D('',#31521,#21938,#21939);
#19075=AXIS2_PLACEMENT_3D('',#31523,#21941,#21942);
#19076=AXIS2_PLACEMENT_3D('',#31526,#21943,#21944);
#19077=AXIS2_PLACEMENT_3D('',#31527,#21945,#21946);
#19078=AXIS2_PLACEMENT_3D('',#31529,#21948,#21949);
#19079=AXIS2_PLACEMENT_3D('',#31550,#21950,#21951);
#19080=AXIS2_PLACEMENT_3D('',#31577,#21952,#21953);
#19081=AXIS2_PLACEMENT_3D('',#31595,#21955,#21956);
#19082=AXIS2_PLACEMENT_3D('',#31613,#21958,#21959);
#19083=AXIS2_PLACEMENT_3D('',#31638,#21960,#21961);
#19084=AXIS2_PLACEMENT_3D('',#31645,#21962,#21963);
#19085=AXIS2_PLACEMENT_3D('',#31647,#21964,#21965);
#19086=AXIS2_PLACEMENT_3D('',#31650,#21967,#21968);
#19087=AXIS2_PLACEMENT_3D('',#31651,#21969,#21970);
#19088=AXIS2_PLACEMENT_3D('',#31653,#21971,#21972);
#19089=AXIS2_PLACEMENT_3D('',#31656,#21974,#21975);
#19090=AXIS2_PLACEMENT_3D('',#31657,#21976,#21977);
#19091=AXIS2_PLACEMENT_3D('',#31660,#21979,#21980);
#19092=AXIS2_PLACEMENT_3D('',#31661,#21981,#21982);
#19093=AXIS2_PLACEMENT_3D('',#31663,#21983,#21984);
#19094=AXIS2_PLACEMENT_3D('',#31667,#21986,#21987);
#19095=AXIS2_PLACEMENT_3D('',#31668,#21988,#21989);
#19096=AXIS2_PLACEMENT_3D('',#31669,#21990,#21991);
#19097=AXIS2_PLACEMENT_3D('',#31672,#21992,#21993);
#19098=AXIS2_PLACEMENT_3D('',#31676,#21995,#21996);
#19099=AXIS2_PLACEMENT_3D('',#31678,#21998,#21999);
#19100=AXIS2_PLACEMENT_3D('',#31691,#22001,#22002);
#19101=AXIS2_PLACEMENT_3D('',#31708,#22003,#22004);
#19102=AXIS2_PLACEMENT_3D('',#31840,#22009,#22010);
#19103=AXIS2_PLACEMENT_3D('',#31916,#22013,#22014);
#19104=AXIS2_PLACEMENT_3D('',#31990,#22017,#22018);
#19105=AXIS2_PLACEMENT_3D('',#32011,#22019,#22020);
#19106=AXIS2_PLACEMENT_3D('',#32022,#22021,#22022);
#19107=AXIS2_PLACEMENT_3D('',#32035,#22029,#22030);
#19108=AXIS2_PLACEMENT_3D('',#32048,#22037,#22038);
#19109=AXIS2_PLACEMENT_3D('',#32061,#22045,#22046);
#19110=AXIS2_PLACEMENT_3D('',#32074,#22053,#22054);
#19111=AXIS2_PLACEMENT_3D('',#32077,#22055,#22056);
#19112=AXIS2_PLACEMENT_3D('',#32081,#22058,#22059);
#19113=AXIS2_PLACEMENT_3D('',#32083,#22060,#22061);
#19114=AXIS2_PLACEMENT_3D('',#32085,#22062,#22063);
#19115=AXIS2_PLACEMENT_3D('',#32088,#22065,#22066);
#19116=AXIS2_PLACEMENT_3D('',#32090,#22067,#22068);
#19117=AXIS2_PLACEMENT_3D('',#32094,#22070,#22071);
#19118=AXIS2_PLACEMENT_3D('',#32096,#22072,#22073);
#19119=AXIS2_PLACEMENT_3D('',#32098,#22074,#22075);
#19120=AXIS2_PLACEMENT_3D('',#32102,#22077,#22078);
#19121=AXIS2_PLACEMENT_3D('',#32103,#22079,#22080);
#19122=AXIS2_PLACEMENT_3D('',#32104,#22081,#22082);
#19123=AXIS2_PLACEMENT_3D('',#32117,#22089,#22090);
#19124=AXIS2_PLACEMENT_3D('',#32130,#22097,#22098);
#19125=AXIS2_PLACEMENT_3D('',#32136,#22102,#22103);
#19126=AXIS2_PLACEMENT_3D('',#32140,#22106,#22107);
#19127=AXIS2_PLACEMENT_3D('',#32144,#22110,#22111);
#19128=AXIS2_PLACEMENT_3D('',#32148,#22114,#22115);
#19129=AXIS2_PLACEMENT_3D('',#32152,#22118,#22119);
#19130=AXIS2_PLACEMENT_3D('',#32154,#22121,#22122);
#19131=AXIS2_PLACEMENT_3D('',#32164,#22127,#22128);
#19132=AXIS2_PLACEMENT_3D('',#32165,#22129,#22130);
#19133=AXIS2_PLACEMENT_3D('',#32169,#22132,#22133);
#19134=AXIS2_PLACEMENT_3D('',#32170,#22134,#22135);
#19135=AXIS2_PLACEMENT_3D('',#32171,#22136,#22137);
#19136=AXIS2_PLACEMENT_3D('',#32178,#22141,#22142);
#19137=AXIS2_PLACEMENT_3D('',#32179,#22143,#22144);
#19138=AXIS2_PLACEMENT_3D('',#32185,#22148,#22149);
#19139=AXIS2_PLACEMENT_3D('',#32189,#22152,#22153);
#19140=AXIS2_PLACEMENT_3D('',#32193,#22156,#22157);
#19141=AXIS2_PLACEMENT_3D('',#32197,#22160,#22161);
#19142=AXIS2_PLACEMENT_3D('',#32201,#22164,#22165);
#19143=AXIS2_PLACEMENT_3D('',#32203,#22167,#22168);
#19144=AXIS2_PLACEMENT_3D('',#32213,#22173,#22174);
#19145=AXIS2_PLACEMENT_3D('',#32214,#22175,#22176);
#19146=AXIS2_PLACEMENT_3D('',#32218,#22178,#22179);
#19147=AXIS2_PLACEMENT_3D('',#32219,#22180,#22181);
#19148=AXIS2_PLACEMENT_3D('',#32220,#22182,#22183);
#19149=AXIS2_PLACEMENT_3D('',#32227,#22187,#22188);
#19150=AXIS2_PLACEMENT_3D('',#32228,#22189,#22190);
#19151=AXIS2_PLACEMENT_3D('',#32234,#22194,#22195);
#19152=AXIS2_PLACEMENT_3D('',#32238,#22198,#22199);
#19153=AXIS2_PLACEMENT_3D('',#32242,#22202,#22203);
#19154=AXIS2_PLACEMENT_3D('',#32246,#22206,#22207);
#19155=AXIS2_PLACEMENT_3D('',#32250,#22210,#22211);
#19156=AXIS2_PLACEMENT_3D('',#32252,#22213,#22214);
#19157=AXIS2_PLACEMENT_3D('',#32262,#22219,#22220);
#19158=AXIS2_PLACEMENT_3D('',#32263,#22221,#22222);
#19159=AXIS2_PLACEMENT_3D('',#32267,#22224,#22225);
#19160=AXIS2_PLACEMENT_3D('',#32268,#22226,#22227);
#19161=AXIS2_PLACEMENT_3D('',#32269,#22228,#22229);
#19162=AXIS2_PLACEMENT_3D('',#32276,#22233,#22234);
#19163=AXIS2_PLACEMENT_3D('',#32277,#22235,#22236);
#19164=AXIS2_PLACEMENT_3D('',#32284,#22240,#22241);
#19165=AXIS2_PLACEMENT_3D('',#32289,#22245,#22246);
#19166=AXIS2_PLACEMENT_3D('',#32295,#22250,#22251);
#19167=AXIS2_PLACEMENT_3D('',#32299,#22254,#22255);
#19168=AXIS2_PLACEMENT_3D('',#32303,#22258,#22259);
#19169=AXIS2_PLACEMENT_3D('',#32307,#22262,#22263);
#19170=AXIS2_PLACEMENT_3D('',#32311,#22266,#22267);
#19171=AXIS2_PLACEMENT_3D('',#32313,#22269,#22270);
#19172=AXIS2_PLACEMENT_3D('',#32320,#22274,#22275);
#19173=AXIS2_PLACEMENT_3D('',#32321,#22276,#22277);
#19174=AXIS2_PLACEMENT_3D('',#32324,#22279,#22280);
#19175=AXIS2_PLACEMENT_3D('',#32325,#22281,#22282);
#19176=AXIS2_PLACEMENT_3D('',#32330,#22285,#22286);
#19177=AXIS2_PLACEMENT_3D('',#32331,#22287,#22288);
#19178=AXIS2_PLACEMENT_3D('',#32336,#22291,#22292);
#19179=AXIS2_PLACEMENT_3D('',#32337,#22293,#22294);
#19180=AXIS2_PLACEMENT_3D('',#32341,#22297,#22298);
#19181=AXIS2_PLACEMENT_3D('',#32344,#22300,#22301);
#19182=AXIS2_PLACEMENT_3D('',#32345,#22302,#22303);
#19183=AXIS2_PLACEMENT_3D('',#32348,#22305,#22306);
#19184=AXIS2_PLACEMENT_3D('',#32349,#22307,#22308);
#19185=AXIS2_PLACEMENT_3D('',#32352,#22310,#22311);
#19186=AXIS2_PLACEMENT_3D('',#32353,#22312,#22313);
#19187=AXIS2_PLACEMENT_3D('',#32357,#22316,#22317);
#19188=AXIS2_PLACEMENT_3D('',#32360,#22319,#22320);
#19189=AXIS2_PLACEMENT_3D('',#32361,#22321,#22322);
#19190=AXIS2_PLACEMENT_3D('',#32364,#22324,#22325);
#19191=AXIS2_PLACEMENT_3D('',#32365,#22326,#22327);
#19192=AXIS2_PLACEMENT_3D('',#32368,#22329,#22330);
#19193=AXIS2_PLACEMENT_3D('',#32369,#22331,#22332);
#19194=AXIS2_PLACEMENT_3D('',#32373,#22335,#22336);
#19195=AXIS2_PLACEMENT_3D('',#32374,#22337,#22338);
#19196=AXIS2_PLACEMENT_3D('',#32375,#22339,#22340);
#19197=AXIS2_PLACEMENT_3D('',#32378,#22342,#22343);
#19198=AXIS2_PLACEMENT_3D('',#32379,#22344,#22345);
#19199=AXIS2_PLACEMENT_3D('',#32383,#22348,#22349);
#19200=AXIS2_PLACEMENT_3D('',#32386,#22351,#22352);
#19201=AXIS2_PLACEMENT_3D('',#32387,#22353,#22354);
#19202=AXIS2_PLACEMENT_3D('',#32388,#22355,#22356);
#19203=AXIS2_PLACEMENT_3D('',#32389,#22357,#22358);
#19204=AXIS2_PLACEMENT_3D('',#32394,#22361,#22362);
#19205=AXIS2_PLACEMENT_3D('',#32395,#22363,#22364);
#19206=AXIS2_PLACEMENT_3D('',#32398,#22366,#22367);
#19207=AXIS2_PLACEMENT_3D('',#32399,#22368,#22369);
#19208=AXIS2_PLACEMENT_3D('',#32402,#22371,#22372);
#19209=AXIS2_PLACEMENT_3D('',#32403,#22373,#22374);
#19210=AXIS2_PLACEMENT_3D('',#32406,#22376,#22377);
#19211=AXIS2_PLACEMENT_3D('',#32407,#22378,#22379);
#19212=AXIS2_PLACEMENT_3D('',#32410,#22381,#22382);
#19213=AXIS2_PLACEMENT_3D('',#32411,#22383,#22384);
#19214=AXIS2_PLACEMENT_3D('',#32412,#22385,#22386);
#19215=AXIS2_PLACEMENT_3D('',#32413,#22387,#22388);
#19216=AXIS2_PLACEMENT_3D('',#32418,#22391,#22392);
#19217=AXIS2_PLACEMENT_3D('',#32419,#22393,#22394);
#19218=AXIS2_PLACEMENT_3D('',#32422,#22396,#22397);
#19219=AXIS2_PLACEMENT_3D('',#32423,#22398,#22399);
#19220=AXIS2_PLACEMENT_3D('',#32426,#22401,#22402);
#19221=AXIS2_PLACEMENT_3D('',#32427,#22403,#22404);
#19222=AXIS2_PLACEMENT_3D('',#32430,#22406,#22407);
#19223=AXIS2_PLACEMENT_3D('',#32431,#22408,#22409);
#19224=AXIS2_PLACEMENT_3D('',#32434,#22411,#22412);
#19225=AXIS2_PLACEMENT_3D('',#32435,#22413,#22414);
#19226=AXIS2_PLACEMENT_3D('',#32436,#22415,#22416);
#19227=AXIS2_PLACEMENT_3D('',#32437,#22417,#22418);
#19228=AXIS2_PLACEMENT_3D('',#32439,#22420,#22421);
#19229=AXIS2_PLACEMENT_3D('',#32441,#22423,#22424);
#19230=AXIS2_PLACEMENT_3D('',#32444,#22425,#22426);
#19231=AXIS2_PLACEMENT_3D('',#32447,#22429,#22430);
#19232=AXIS2_PLACEMENT_3D('',#32449,#22432,#22433);
#19233=AXIS2_PLACEMENT_3D('',#32453,#22435,#22436);
#19234=AXIS2_PLACEMENT_3D('',#32455,#22438,#22439);
#19235=AXIS2_PLACEMENT_3D('',#32459,#22441,#22442);
#19236=AXIS2_PLACEMENT_3D('',#32461,#22444,#22445);
#19237=AXIS2_PLACEMENT_3D('',#32463,#22447,#22448);
#19238=AXIS2_PLACEMENT_3D('',#32467,#22450,#22451);
#19239=AXIS2_PLACEMENT_3D('',#32469,#22453,#22454);
#19240=AXIS2_PLACEMENT_3D('',#32488,#22457,#22458);
#19241=AXIS2_PLACEMENT_3D('',#32490,#22459,#22460);
#19242=AXIS2_PLACEMENT_3D('',#32499,#22462,#22463);
#19243=AXIS2_PLACEMENT_3D('',#32515,#22465,#22466);
#19244=AXIS2_PLACEMENT_3D('',#32526,#22469,#22470);
#19245=AXIS2_PLACEMENT_3D('',#32528,#22471,#22472);
#19246=AXIS2_PLACEMENT_3D('',#32537,#22474,#22475);
#19247=AXIS2_PLACEMENT_3D('',#32545,#22477,#22478);
#19248=AXIS2_PLACEMENT_3D('',#32549,#22481,#22482);
#19249=AXIS2_PLACEMENT_3D('',#32551,#22483,#22484);
#19250=AXIS2_PLACEMENT_3D('',#32553,#22486,#22487);
#19251=AXIS2_PLACEMENT_3D('',#32555,#22489,#22490);
#19252=AXIS2_PLACEMENT_3D('',#32578,#22493,#22494);
#19253=AXIS2_PLACEMENT_3D('',#32580,#22495,#22496);
#19254=AXIS2_PLACEMENT_3D('',#32589,#22498,#22499);
#19255=AXIS2_PLACEMENT_3D('',#32605,#22501,#22502);
#19256=AXIS2_PLACEMENT_3D('',#32626,#22503,#22504);
#19257=AXIS2_PLACEMENT_3D('',#32668,#22505,#22506);
#19258=AXIS2_PLACEMENT_3D('',#32682,#22507,#22508);
#19259=AXIS2_PLACEMENT_3D('',#32733,#22509,#22510);
#19260=AXIS2_PLACEMENT_3D('',#32744,#22511,#22512);
#19261=AXIS2_PLACEMENT_3D('',#32795,#22513,#22514);
#19262=AXIS2_PLACEMENT_3D('',#32831,#22515,#22516);
#19263=AXIS2_PLACEMENT_3D('',#32881,#22517,#22518);
#19264=AXIS2_PLACEMENT_3D('',#32882,#22519,#22520);
#19265=AXIS2_PLACEMENT_3D('',#32883,#22521,#22522);
#19266=AXIS2_PLACEMENT_3D('',#32884,#22523,#22524);
#19267=AXIS2_PLACEMENT_3D('',#32887,#22525,#22526);
#19268=AXIS2_PLACEMENT_3D('',#32890,#22529,#22530);
#19269=AXIS2_PLACEMENT_3D('',#32894,#22533,#22534);
#19270=AXIS2_PLACEMENT_3D('',#32896,#22535,#22536);
#19271=AXIS2_PLACEMENT_3D('',#32898,#22538,#22539);
#19272=AXIS2_PLACEMENT_3D('',#32902,#22542,#22543);
#19273=AXIS2_PLACEMENT_3D('',#32904,#22544,#22545);
#19274=AXIS2_PLACEMENT_3D('',#32906,#22547,#22548);
#19275=AXIS2_PLACEMENT_3D('',#32910,#22551,#22552);
#19276=AXIS2_PLACEMENT_3D('',#32912,#22553,#22554);
#19277=AXIS2_PLACEMENT_3D('',#32914,#22556,#22557);
#19278=AXIS2_PLACEMENT_3D('',#33033,#22563,#22564);
#19279=AXIS2_PLACEMENT_3D('',#33036,#22565,#22566);
#19280=AXIS2_PLACEMENT_3D('',#33083,#22569,#22570);
#19281=AXIS2_PLACEMENT_3D('',#33086,#22571,#22572);
#19282=AXIS2_PLACEMENT_3D('',#33135,#22575,#22576);
#19283=AXIS2_PLACEMENT_3D('',#33138,#22577,#22578);
#19284=AXIS2_PLACEMENT_3D('',#33187,#22581,#22582);
#19285=AXIS2_PLACEMENT_3D('',#33190,#22583,#22584);
#19286=AXIS2_PLACEMENT_3D('',#33326,#22585,#22586);
#19287=AXIS2_PLACEMENT_3D('',#33389,#22587,#22588);
#19288=AXIS2_PLACEMENT_3D('',#33390,#22589,#22590);
#19289=AXIS2_PLACEMENT_3D('',#33416,#22592,#22593);
#19290=AXIS2_PLACEMENT_3D('',#33441,#22596,#22597);
#19291=AXIS2_PLACEMENT_3D('',#33542,#22600,#22601);
#19292=AXIS2_PLACEMENT_3D('',#33554,#22602,#22603);
#19293=AXIS2_PLACEMENT_3D('',#33557,#22604,#22605);
#19294=AXIS2_PLACEMENT_3D('',#33714,#22608,#22609);
#19295=AXIS2_PLACEMENT_3D('',#33717,#22610,#22611);
#19296=AXIS2_PLACEMENT_3D('',#33874,#22614,#22615);
#19297=AXIS2_PLACEMENT_3D('',#33877,#22616,#22617);
#19298=AXIS2_PLACEMENT_3D('',#34034,#22620,#22621);
#19299=AXIS2_PLACEMENT_3D('',#34037,#22622,#22623);
#19300=AXIS2_PLACEMENT_3D('',#35987,#22626,#22627);
#19301=AXIS2_PLACEMENT_3D('',#35988,#22628,#22629);
#19302=AXIS2_PLACEMENT_3D('',#35991,#22630,#22631);
#19303=AXIS2_PLACEMENT_3D('',#36058,#22632,#22633);
#19304=AXIS2_PLACEMENT_3D('',#36061,#22634,#22635);
#19305=AXIS2_PLACEMENT_3D('',#36062,#22636,#22637);
#19306=AXIS2_PLACEMENT_3D('',#36105,#22640,#22641);
#19307=AXIS2_PLACEMENT_3D('',#36108,#22642,#22643);
#19308=AXIS2_PLACEMENT_3D('',#36157,#22646,#22647);
#19309=AXIS2_PLACEMENT_3D('',#36160,#22648,#22649);
#19310=AXIS2_PLACEMENT_3D('',#36229,#22652,#22653);
#19311=AXIS2_PLACEMENT_3D('',#36234,#22655,#22656);
#19312=AXIS2_PLACEMENT_3D('',#36238,#22658,#22659);
#19313=AXIS2_PLACEMENT_3D('',#36242,#22661,#22662);
#19314=AXIS2_PLACEMENT_3D('',#36245,#22664,#22665);
#19315=AXIS2_PLACEMENT_3D('',#36246,#22666,#22667);
#19316=AXIS2_PLACEMENT_3D('',#36249,#22668,#22669);
#19317=AXIS2_PLACEMENT_3D('',#36252,#22672,#22673);
#19318=AXIS2_PLACEMENT_3D('',#36254,#22674,#22675);
#19319=AXIS2_PLACEMENT_3D('',#36256,#22677,#22678);
#19320=AXIS2_PLACEMENT_3D('',#36258,#22679,#22680);
#19321=AXIS2_PLACEMENT_3D('',#36260,#22682,#22683);
#19322=AXIS2_PLACEMENT_3D('',#36263,#22685,#22686);
#19323=AXIS2_PLACEMENT_3D('',#36264,#22687,#22688);
#19324=AXIS2_PLACEMENT_3D('',#36266,#22689,#22690);
#19325=AXIS2_PLACEMENT_3D('',#36268,#22692,#22693);
#19326=AXIS2_PLACEMENT_3D('',#36270,#22694,#22695);
#19327=AXIS2_PLACEMENT_3D('',#36272,#22697,#22698);
#19328=AXIS2_PLACEMENT_3D('',#36273,#22699,#22700);
#19329=AXIS2_PLACEMENT_3D('',#36274,#22701,#22702);
#19330=AXIS2_PLACEMENT_3D('',#36276,#22703,#22704);
#19331=AXIS2_PLACEMENT_3D('',#36278,#22706,#22707);
#19332=AXIS2_PLACEMENT_3D('',#36280,#22708,#22709);
#19333=AXIS2_PLACEMENT_3D('',#36282,#22711,#22712);
#19334=AXIS2_PLACEMENT_3D('',#36284,#22713,#22714);
#19335=AXIS2_PLACEMENT_3D('',#36289,#22715,#22716);
#19336=AXIS2_PLACEMENT_3D('',#36292,#22718,#22719);
#19337=AXIS2_PLACEMENT_3D('',#36293,#22720,#22721);
#19338=AXIS2_PLACEMENT_3D('',#36295,#22722,#22723);
#19339=AXIS2_PLACEMENT_3D('',#36297,#22725,#22726);
#19340=AXIS2_PLACEMENT_3D('',#36299,#22727,#22728);
#19341=AXIS2_PLACEMENT_3D('',#36301,#22730,#22731);
#19342=AXIS2_PLACEMENT_3D('',#36303,#22732,#22733);
#19343=AXIS2_PLACEMENT_3D('',#36305,#22735,#22736);
#19344=AXIS2_PLACEMENT_3D('',#36306,#22737,#22738);
#19345=AXIS2_PLACEMENT_3D('',#36307,#22739,#22740);
#19346=AXIS2_PLACEMENT_3D('',#36313,#22744,#22745);
#19347=AXIS2_PLACEMENT_3D('',#36319,#22749,#22750);
#19348=AXIS2_PLACEMENT_3D('',#36328,#22751,#22752);
#19349=AXIS2_PLACEMENT_3D('',#36335,#22753,#22754);
#19350=AXIS2_PLACEMENT_3D('',#36341,#22758,#22759);
#19351=AXIS2_PLACEMENT_3D('',#36350,#22760,#22761);
#19352=AXIS2_PLACEMENT_3D('',#36357,#22762,#22763);
#19353=AXIS2_PLACEMENT_3D('',#36366,#22764,#22765);
#19354=AXIS2_PLACEMENT_3D('',#36375,#22767,#22768);
#19355=AXIS2_PLACEMENT_3D('',#36386,#22770,#22771);
#19356=AXIS2_PLACEMENT_3D('',#36393,#22772,#22773);
#19357=AXIS2_PLACEMENT_3D('',#36454,#22776,#22777);
#19358=AXIS2_PLACEMENT_3D('',#36518,#22778,#22779);
#19359=AXIS2_PLACEMENT_3D('',#36613,#22781,#22782);
#19360=AXIS2_PLACEMENT_3D('',#36666,#22784,#22785);
#19361=AXIS2_PLACEMENT_3D('',#36761,#22787,#22788);
#19362=AXIS2_PLACEMENT_3D('',#36832,#22789,#22790);
#19363=AXIS2_PLACEMENT_3D('',#36885,#22792,#22793);
#19364=AXIS2_PLACEMENT_3D('',#36981,#22795,#22796);
#19365=AXIS2_PLACEMENT_3D('',#37031,#22797,#22798);
#19366=AXIS2_PLACEMENT_3D('',#37047,#22799,#22800);
#19367=AXIS2_PLACEMENT_3D('',#37098,#22801,#22802);
#19368=AXIS2_PLACEMENT_3D('',#37102,#22804,#22805);
#19369=AXIS2_PLACEMENT_3D('',#37166,#22806,#22807);
#19370=AXIS2_PLACEMENT_3D('',#37261,#22809,#22810);
#19371=AXIS2_PLACEMENT_3D('',#37262,#22811,#22812);
#19372=AXIS2_PLACEMENT_3D('',#37263,#22813,#22814);
#19373=AXIS2_PLACEMENT_3D('',#37265,#22815,#22816);
#19374=AXIS2_PLACEMENT_3D('',#37267,#22817,#22818);
#19375=AXIS2_PLACEMENT_3D('',#37268,#22819,#22820);
#19376=AXIS2_PLACEMENT_3D('',#37270,#22821,#22822);
#19377=AXIS2_PLACEMENT_3D('',#37272,#22823,#22824);
#19378=AXIS2_PLACEMENT_3D('',#37273,#22825,#22826);
#19379=AXIS2_PLACEMENT_3D('',#37275,#22827,#22828);
#19380=AXIS2_PLACEMENT_3D('',#37277,#22829,#22830);
#19381=AXIS2_PLACEMENT_3D('',#37278,#22831,#22832);
#19382=AXIS2_PLACEMENT_3D('',#37279,#22833,#22834);
#19383=AXIS2_PLACEMENT_3D('',#37280,#22835,#22836);
#19384=AXIS2_PLACEMENT_3D('',#37293,#22843,#22844);
#19385=AXIS2_PLACEMENT_3D('',#37306,#22851,#22852);
#19386=AXIS2_PLACEMENT_3D('',#37308,#22854,#22855);
#19387=AXIS2_PLACEMENT_3D('',#37310,#22857,#22858);
#19388=AXIS2_PLACEMENT_3D('',#37312,#22860,#22861);
#19389=AXIS2_PLACEMENT_3D('',#37314,#22863,#22864);
#19390=AXIS2_PLACEMENT_3D('',#37317,#22865,#22866);
#19391=AXIS2_PLACEMENT_3D('',#37323,#22868,#22869);
#19392=AXIS2_PLACEMENT_3D('',#37327,#22872,#22873);
#19393=AXIS2_PLACEMENT_3D('',#37331,#22876,#22877);
#19394=AXIS2_PLACEMENT_3D('',#37338,#22879,#22880);
#19395=AXIS2_PLACEMENT_3D('',#37340,#22881,#22882);
#19396=AXIS2_PLACEMENT_3D('',#37342,#22884,#22885);
#19397=AXIS2_PLACEMENT_3D('',#37345,#22887,#22888);
#19398=AXIS2_PLACEMENT_3D('',#37346,#22889,#22890);
#19399=AXIS2_PLACEMENT_3D('',#37348,#22891,#22892);
#19400=AXIS2_PLACEMENT_3D('',#37353,#22893,#22894);
#19401=AXIS2_PLACEMENT_3D('',#37357,#22897,#22898);
#19402=AXIS2_PLACEMENT_3D('',#37361,#22901,#22902);
#19403=AXIS2_PLACEMENT_3D('',#37368,#22904,#22905);
#19404=AXIS2_PLACEMENT_3D('',#37369,#22906,#22907);
#19405=AXIS2_PLACEMENT_3D('',#37370,#22908,#22909);
#19406=AXIS2_PLACEMENT_3D('',#37372,#22910,#22911);
#19407=AXIS2_PLACEMENT_3D('',#37377,#22912,#22913);
#19408=AXIS2_PLACEMENT_3D('',#37381,#22916,#22917);
#19409=AXIS2_PLACEMENT_3D('',#37385,#22920,#22921);
#19410=AXIS2_PLACEMENT_3D('',#37392,#22923,#22924);
#19411=AXIS2_PLACEMENT_3D('',#37394,#22925,#22926);
#19412=AXIS2_PLACEMENT_3D('',#37396,#22928,#22929);
#19413=AXIS2_PLACEMENT_3D('',#37399,#22931,#22932);
#19414=AXIS2_PLACEMENT_3D('',#37400,#22933,#22934);
#19415=AXIS2_PLACEMENT_3D('',#37402,#22935,#22936);
#19416=AXIS2_PLACEMENT_3D('',#37407,#22937,#22938);
#19417=AXIS2_PLACEMENT_3D('',#37411,#22941,#22942);
#19418=AXIS2_PLACEMENT_3D('',#37415,#22945,#22946);
#19419=AXIS2_PLACEMENT_3D('',#37422,#22948,#22949);
#19420=AXIS2_PLACEMENT_3D('',#37424,#22950,#22951);
#19421=AXIS2_PLACEMENT_3D('',#37426,#22953,#22954);
#19422=AXIS2_PLACEMENT_3D('',#37427,#22955,#22956);
#19423=AXIS2_PLACEMENT_3D('',#37428,#22957,#22958);
#19424=AXIS2_PLACEMENT_3D('',#37434,#22962,#22963);
#19425=AXIS2_PLACEMENT_3D('',#37438,#22966,#22967);
#19426=AXIS2_PLACEMENT_3D('',#37442,#22970,#22971);
#19427=AXIS2_PLACEMENT_3D('',#37446,#22974,#22975);
#19428=AXIS2_PLACEMENT_3D('',#37450,#22978,#22979);
#19429=AXIS2_PLACEMENT_3D('',#37452,#22981,#22982);
#19430=AXIS2_PLACEMENT_3D('',#37458,#22986,#22987);
#19431=AXIS2_PLACEMENT_3D('',#37462,#22990,#22991);
#19432=AXIS2_PLACEMENT_3D('',#37466,#22994,#22995);
#19433=AXIS2_PLACEMENT_3D('',#37470,#22998,#22999);
#19434=AXIS2_PLACEMENT_3D('',#37474,#23002,#23003);
#19435=AXIS2_PLACEMENT_3D('',#37476,#23005,#23006);
#19436=AXIS2_PLACEMENT_3D('',#37479,#23007,#23008);
#19437=AXIS2_PLACEMENT_3D('',#37483,#23010,#23011);
#19438=AXIS2_PLACEMENT_3D('',#37485,#23013,#23014);
#19439=AXIS2_PLACEMENT_3D('',#37488,#23015,#23016);
#19440=AXIS2_PLACEMENT_3D('',#37492,#23018,#23019);
#19441=AXIS2_PLACEMENT_3D('',#37494,#23021,#23022);
#19442=AXIS2_PLACEMENT_3D('',#37503,#23027,#23028);
#19443=AXIS2_PLACEMENT_3D('',#37508,#23030,#23031);
#19444=AXIS2_PLACEMENT_3D('',#37513,#23035,#23036);
#19445=AXIS2_PLACEMENT_3D('',#37518,#23039,#23040);
#19446=AXIS2_PLACEMENT_3D('',#37519,#23041,#23042);
#19447=AXIS2_PLACEMENT_3D('',#37522,#23043,#23044);
#19448=AXIS2_PLACEMENT_3D('',#37526,#23046,#23047);
#19449=AXIS2_PLACEMENT_3D('',#37528,#23049,#23050);
#19450=AXIS2_PLACEMENT_3D('',#37531,#23051,#23052);
#19451=AXIS2_PLACEMENT_3D('',#37535,#23054,#23055);
#19452=AXIS2_PLACEMENT_3D('',#37537,#23057,#23058);
#19453=AXIS2_PLACEMENT_3D('',#37540,#23059,#23060);
#19454=AXIS2_PLACEMENT_3D('',#37544,#23062,#23063);
#19455=AXIS2_PLACEMENT_3D('',#37546,#23065,#23066);
#19456=AXIS2_PLACEMENT_3D('',#37555,#23073,#23074);
#19457=AXIS2_PLACEMENT_3D('',#37558,#23077,#23078);
#19458=AXIS2_PLACEMENT_3D('',#37561,#23079,#23080);
#19459=AXIS2_PLACEMENT_3D('',#37564,#23083,#23084);
#19460=AXIS2_PLACEMENT_3D('',#37565,#23085,#23086);
#19461=AXIS2_PLACEMENT_3D('',#37566,#23087,#23088);
#19462=AXIS2_PLACEMENT_3D('',#37572,#23092,#23093);
#19463=AXIS2_PLACEMENT_3D('',#37578,#23097,#23098);
#19464=AXIS2_PLACEMENT_3D('',#37582,#23100,#23101);
#19465=AXIS2_PLACEMENT_3D('',#37590,#23105,#23106);
#19466=AXIS2_PLACEMENT_3D('',#37592,#23108,#23109);
#19467=AXIS2_PLACEMENT_3D('',#37597,#23111,#23112);
#19468=AXIS2_PLACEMENT_3D('',#37600,#23114,#23115);
#19469=AXIS2_PLACEMENT_3D('',#37601,#23116,#23117);
#19470=AXIS2_PLACEMENT_3D('',#37609,#23122,#23123);
#19471=AXIS2_PLACEMENT_3D('',#37612,#23126,#23127);
#19472=AXIS2_PLACEMENT_3D('',#37617,#23129,#23130);
#19473=AXIS2_PLACEMENT_3D('',#37620,#23133,#23134);
#19474=AXIS2_PLACEMENT_3D('',#37624,#23137,#23138);
#19475=AXIS2_PLACEMENT_3D('',#37632,#23143,#23144);
#19476=AXIS2_PLACEMENT_3D('',#37638,#23148,#23149);
#19477=AXIS2_PLACEMENT_3D('',#37644,#23153,#23154);
#19478=AXIS2_PLACEMENT_3D('',#37648,#23156,#23157);
#19479=AXIS2_PLACEMENT_3D('',#37650,#23159,#23160);
#19480=AXIS2_PLACEMENT_3D('',#37655,#23162,#23163);
#19481=AXIS2_PLACEMENT_3D('',#37658,#23165,#23166);
#19482=AXIS2_PLACEMENT_3D('',#37659,#23167,#23168);
#19483=AXIS2_PLACEMENT_3D('',#37665,#23172,#23173);
#19484=AXIS2_PLACEMENT_3D('',#37668,#23176,#23177);
#19485=AXIS2_PLACEMENT_3D('',#37674,#23181,#23182);
#19486=AXIS2_PLACEMENT_3D('',#37678,#23184,#23185);
#19487=AXIS2_PLACEMENT_3D('',#37686,#23189,#23190);
#19488=AXIS2_PLACEMENT_3D('',#37688,#23192,#23193);
#19489=AXIS2_PLACEMENT_3D('',#37693,#23195,#23196);
#19490=AXIS2_PLACEMENT_3D('',#37696,#23198,#23199);
#19491=AXIS2_PLACEMENT_3D('',#37697,#23200,#23201);
#19492=AXIS2_PLACEMENT_3D('',#37703,#23205,#23206);
#19493=AXIS2_PLACEMENT_3D('',#37706,#23209,#23210);
#19494=AXIS2_PLACEMENT_3D('',#37711,#23212,#23213);
#19495=AXIS2_PLACEMENT_3D('',#37714,#23215,#23216);
#19496=AXIS2_PLACEMENT_3D('',#37715,#23217,#23218);
#19497=AXIS2_PLACEMENT_3D('',#37720,#23222,#23223);
#19498=AXIS2_PLACEMENT_3D('',#37724,#23226,#23227);
#19499=AXIS2_PLACEMENT_3D('',#37728,#23229,#23230);
#19500=AXIS2_PLACEMENT_3D('',#37736,#23234,#23235);
#19501=AXIS2_PLACEMENT_3D('',#37738,#23237,#23238);
#19502=AXIS2_PLACEMENT_3D('',#37751,#23245,#23246);
#19503=AXIS2_PLACEMENT_3D('',#37760,#23251,#23252);
#19504=AXIS2_PLACEMENT_3D('',#37761,#23253,#23254);
#19505=AXIS2_PLACEMENT_3D('',#37770,#23259,#23260);
#19506=AXIS2_PLACEMENT_3D('',#37771,#23261,#23262);
#19507=AXIS2_PLACEMENT_3D('',#37775,#23264,#23265);
#19508=AXIS2_PLACEMENT_3D('',#37777,#23267,#23268);
#19509=AXIS2_PLACEMENT_3D('',#37783,#23272,#23273);
#19510=AXIS2_PLACEMENT_3D('',#37786,#23275,#23276);
#19511=AXIS2_PLACEMENT_3D('',#37787,#23277,#23278);
#19512=AXIS2_PLACEMENT_3D('',#37791,#23281,#23282);
#19513=AXIS2_PLACEMENT_3D('',#37795,#23285,#23286);
#19514=AXIS2_PLACEMENT_3D('',#37799,#23289,#23290);
#19515=AXIS2_PLACEMENT_3D('',#37802,#23292,#23293);
#19516=AXIS2_PLACEMENT_3D('',#37803,#23294,#23295);
#19517=AXIS2_PLACEMENT_3D('',#37809,#23299,#23300);
#19518=AXIS2_PLACEMENT_3D('',#37816,#23304,#23305);
#19519=AXIS2_PLACEMENT_3D('',#37817,#23306,#23307);
#19520=AXIS2_PLACEMENT_3D('',#37821,#23309,#23310);
#19521=AXIS2_PLACEMENT_3D('',#37823,#23312,#23313);
#19522=AXIS2_PLACEMENT_3D('',#37829,#23317,#23318);
#19523=AXIS2_PLACEMENT_3D('',#37832,#23320,#23321);
#19524=AXIS2_PLACEMENT_3D('',#37833,#23322,#23323);
#19525=AXIS2_PLACEMENT_3D('',#37837,#23326,#23327);
#19526=AXIS2_PLACEMENT_3D('',#37841,#23330,#23331);
#19527=AXIS2_PLACEMENT_3D('',#37845,#23334,#23335);
#19528=AXIS2_PLACEMENT_3D('',#37848,#23337,#23338);
#19529=AXIS2_PLACEMENT_3D('',#37849,#23339,#23340);
#19530=AXIS2_PLACEMENT_3D('',#37855,#23344,#23345);
#19531=AXIS2_PLACEMENT_3D('',#37862,#23349,#23350);
#19532=AXIS2_PLACEMENT_3D('',#37863,#23351,#23352);
#19533=AXIS2_PLACEMENT_3D('',#37867,#23354,#23355);
#19534=AXIS2_PLACEMENT_3D('',#37869,#23357,#23358);
#19535=AXIS2_PLACEMENT_3D('',#37875,#23362,#23363);
#19536=AXIS2_PLACEMENT_3D('',#37878,#23365,#23366);
#19537=AXIS2_PLACEMENT_3D('',#37879,#23367,#23368);
#19538=AXIS2_PLACEMENT_3D('',#37883,#23371,#23372);
#19539=AXIS2_PLACEMENT_3D('',#37887,#23375,#23376);
#19540=AXIS2_PLACEMENT_3D('',#37891,#23379,#23380);
#19541=AXIS2_PLACEMENT_3D('',#37894,#23382,#23383);
#19542=AXIS2_PLACEMENT_3D('',#37895,#23384,#23385);
#19543=AXIS2_PLACEMENT_3D('',#37901,#23389,#23390);
#19544=AXIS2_PLACEMENT_3D('',#37908,#23394,#23395);
#19545=AXIS2_PLACEMENT_3D('',#37909,#23396,#23397);
#19546=AXIS2_PLACEMENT_3D('',#37913,#23399,#23400);
#19547=AXIS2_PLACEMENT_3D('',#37915,#23402,#23403);
#19548=AXIS2_PLACEMENT_3D('',#37921,#23407,#23408);
#19549=AXIS2_PLACEMENT_3D('',#37924,#23410,#23411);
#19550=AXIS2_PLACEMENT_3D('',#37925,#23412,#23413);
#19551=AXIS2_PLACEMENT_3D('',#37929,#23416,#23417);
#19552=AXIS2_PLACEMENT_3D('',#37933,#23420,#23421);
#19553=AXIS2_PLACEMENT_3D('',#37937,#23424,#23425);
#19554=AXIS2_PLACEMENT_3D('',#37940,#23427,#23428);
#19555=AXIS2_PLACEMENT_3D('',#37941,#23429,#23430);
#19556=AXIS2_PLACEMENT_3D('',#37945,#23433,#23434);
#19557=AXIS2_PLACEMENT_3D('',#37951,#23438,#23439);
#19558=AXIS2_PLACEMENT_3D('',#37955,#23442,#23443);
#19559=AXIS2_PLACEMENT_3D('',#37959,#23446,#23447);
#19560=AXIS2_PLACEMENT_3D('',#37963,#23450,#23451);
#19561=AXIS2_PLACEMENT_3D('',#37967,#23454,#23455);
#19562=AXIS2_PLACEMENT_3D('',#37969,#23457,#23458);
#19563=AXIS2_PLACEMENT_3D('',#37970,#23459,#23460);
#19564=AXIS2_PLACEMENT_3D('',#37971,#23461,#23462);
#19565=AXIS2_PLACEMENT_3D('',#37974,#23465,#23466);
#19566=AXIS2_PLACEMENT_3D('',#37976,#23468,#23469);
#19567=AXIS2_PLACEMENT_3D('',#37978,#23471,#23472);
#19568=AXIS2_PLACEMENT_3D('',#37979,#23473,#23474);
#19569=AXIS2_PLACEMENT_3D('',#37980,#23475,#23476);
#19570=AXIS2_PLACEMENT_3D('',#37981,#23477,#23478);
#19571=AXIS2_PLACEMENT_3D('',#37982,#23479,#23480);
#19572=AXIS2_PLACEMENT_3D('',#37983,#23481,#23482);
#19573=AXIS2_PLACEMENT_3D('',#37989,#23486,#23487);
#19574=AXIS2_PLACEMENT_3D('',#37994,#23489,#23490);
#19575=AXIS2_PLACEMENT_3D('',#37997,#23492,#23493);
#19576=AXIS2_PLACEMENT_3D('',#38000,#23495,#23496);
#19577=AXIS2_PLACEMENT_3D('',#38001,#23497,#23498);
#19578=AXIS2_PLACEMENT_3D('',#38005,#23501,#23502);
#19579=AXIS2_PLACEMENT_3D('',#38008,#23504,#23505);
#19580=AXIS2_PLACEMENT_3D('',#38009,#23506,#23507);
#19581=AXIS2_PLACEMENT_3D('',#38013,#23510,#23511);
#19582=AXIS2_PLACEMENT_3D('',#38017,#23513,#23514);
#19583=AXIS2_PLACEMENT_3D('',#38020,#23516,#23517);
#19584=AXIS2_PLACEMENT_3D('',#38022,#23519,#23520);
#19585=AXIS2_PLACEMENT_3D('',#38024,#23522,#23523);
#19586=AXIS2_PLACEMENT_3D('',#38026,#23525,#23526);
#19587=AXIS2_PLACEMENT_3D('',#38028,#23528,#23529);
#19588=AXIS2_PLACEMENT_3D('',#38032,#23531,#23532);
#19589=AXIS2_PLACEMENT_3D('',#38036,#23534,#23535);
#19590=AXIS2_PLACEMENT_3D('',#38038,#23537,#23538);
#19591=AXIS2_PLACEMENT_3D('',#38042,#23541,#23542);
#19592=AXIS2_PLACEMENT_3D('',#38045,#23544,#23545);
#19593=AXIS2_PLACEMENT_3D('',#38046,#23546,#23547);
#19594=AXIS2_PLACEMENT_3D('',#38050,#23550,#23551);
#19595=AXIS2_PLACEMENT_3D('',#38054,#23553,#23554);
#19596=AXIS2_PLACEMENT_3D('',#38058,#23556,#23557);
#19597=AXIS2_PLACEMENT_3D('',#38061,#23559,#23560);
#19598=AXIS2_PLACEMENT_3D('',#38062,#23561,#23562);
#19599=AXIS2_PLACEMENT_3D('',#38066,#23565,#23566);
#19600=AXIS2_PLACEMENT_3D('',#38067,#23567,#23568);
#19601=AXIS2_PLACEMENT_3D('',#38068,#23569,#23570);
#19602=AXIS2_PLACEMENT_3D('',#38069,#23571,#23572);
#19603=AXIS2_PLACEMENT_3D('',#38082,#23579,#23580);
#19604=AXIS2_PLACEMENT_3D('',#38085,#23583,#23584);
#19605=AXIS2_PLACEMENT_3D('',#38087,#23586,#23587);
#19606=AXIS2_PLACEMENT_3D('',#38089,#23589,#23590);
#19607=AXIS2_PLACEMENT_3D('',#38091,#23592,#23593);
#19608=AXIS2_PLACEMENT_3D('',#38093,#23595,#23596);
#19609=AXIS2_PLACEMENT_3D('',#38095,#23598,#23599);
#19610=AXIS2_PLACEMENT_3D('',#38096,#23600,#23601);
#19611=AXIS2_PLACEMENT_3D('',#38098,#23603,#23604);
#19612=AXIS2_PLACEMENT_3D('',#38100,#23606,#23607);
#19613=AXIS2_PLACEMENT_3D('',#38102,#23609,#23610);
#19614=AXIS2_PLACEMENT_3D('',#38104,#23612,#23613);
#19615=AXIS2_PLACEMENT_3D('',#38106,#23615,#23616);
#19616=AXIS2_PLACEMENT_3D('',#38108,#23618,#23619);
#19617=AXIS2_PLACEMENT_3D('',#38110,#23621,#23622);
#19618=AXIS2_PLACEMENT_3D('',#38111,#23623,#23624);
#19619=AXIS2_PLACEMENT_3D('',#38128,#23633,#23634);
#19620=AXIS2_PLACEMENT_3D('',#38129,#23635,#23636);
#19621=AXIS2_PLACEMENT_3D('',#38130,#23637,#23638);
#19622=AXIS2_PLACEMENT_3D('',#38131,#23639,#23640);
#19623=AXIS2_PLACEMENT_3D('',#38133,#23641,#23642);
#19624=AXIS2_PLACEMENT_3D('',#38136,#23644,#23645);
#19625=AXIS2_PLACEMENT_3D('',#38137,#23646,#23647);
#19626=AXIS2_PLACEMENT_3D('',#38151,#23655,#23656);
#19627=AXIS2_PLACEMENT_3D('',#38164,#23663,#23664);
#19628=AXIS2_PLACEMENT_3D('',#38175,#23665,#23666);
#19629=AXIS2_PLACEMENT_3D('',#38181,#23670,#23671);
#19630=AXIS2_PLACEMENT_3D('',#38185,#23674,#23675);
#19631=AXIS2_PLACEMENT_3D('',#38189,#23678,#23679);
#19632=AXIS2_PLACEMENT_3D('',#38193,#23682,#23683);
#19633=AXIS2_PLACEMENT_3D('',#38197,#23686,#23687);
#19634=AXIS2_PLACEMENT_3D('',#38199,#23689,#23690);
#19635=AXIS2_PLACEMENT_3D('',#38203,#23692,#23693);
#19636=AXIS2_PLACEMENT_3D('',#38205,#23695,#23696);
#19637=AXIS2_PLACEMENT_3D('',#38206,#23697,#23698);
#19638=AXIS2_PLACEMENT_3D('',#38207,#23699,#23700);
#19639=AXIS2_PLACEMENT_3D('',#38208,#23701,#23702);
#19640=AXIS2_PLACEMENT_3D('',#38209,#23703,#23704);
#19641=AXIS2_PLACEMENT_3D('',#38210,#23705,#23706);
#19642=AXIS2_PLACEMENT_3D('',#38211,#23707,#23708);
#19643=AXIS2_PLACEMENT_3D('',#38212,#23709,#23710);
#19644=AXIS2_PLACEMENT_3D('',#38213,#23711,#23712);
#19645=AXIS2_PLACEMENT_3D('',#38216,#23713,#23714);
#19646=AXIS2_PLACEMENT_3D('',#38217,#23715,#23716);
#19647=AXIS2_PLACEMENT_3D('',#38218,#23717,#23718);
#19648=AXIS2_PLACEMENT_3D('',#38221,#23721,#23722);
#19649=AXIS2_PLACEMENT_3D('',#38234,#23729,#23730);
#19650=AXIS2_PLACEMENT_3D('',#38247,#23737,#23738);
#19651=AXIS2_PLACEMENT_3D('',#38260,#23745,#23746);
#19652=AXIS2_PLACEMENT_3D('',#38262,#23747,#23748);
#19653=AXIS2_PLACEMENT_3D('',#38264,#23750,#23751);
#19654=AXIS2_PLACEMENT_3D('',#38268,#23754,#23755);
#19655=AXIS2_PLACEMENT_3D('',#38269,#23756,#23757);
#19656=AXIS2_PLACEMENT_3D('',#38270,#23758,#23759);
#19657=AXIS2_PLACEMENT_3D('',#38272,#23760,#23761);
#19658=AXIS2_PLACEMENT_3D('',#38274,#23763,#23764);
#19659=AXIS2_PLACEMENT_3D('',#38278,#23767,#23768);
#19660=AXIS2_PLACEMENT_3D('',#38279,#23769,#23770);
#19661=AXIS2_PLACEMENT_3D('',#38280,#23771,#23772);
#19662=AXIS2_PLACEMENT_3D('',#38281,#23773,#23774);
#19663=AXIS2_PLACEMENT_3D('',#38282,#23775,#23776);
#19664=AXIS2_PLACEMENT_3D('',#38283,#23777,#23778);
#19665=AXIS2_PLACEMENT_3D('',#38285,#23779,#23780);
#19666=AXIS2_PLACEMENT_3D('',#38287,#23782,#23783);
#19667=AXIS2_PLACEMENT_3D('',#38291,#23786,#23787);
#19668=AXIS2_PLACEMENT_3D('',#38292,#23788,#23789);
#19669=AXIS2_PLACEMENT_3D('',#38293,#23790,#23791);
#19670=AXIS2_PLACEMENT_3D('',#38295,#23792,#23793);
#19671=AXIS2_PLACEMENT_3D('',#38297,#23795,#23796);
#19672=AXIS2_PLACEMENT_3D('',#38301,#23799,#23800);
#19673=AXIS2_PLACEMENT_3D('',#38302,#23801,#23802);
#19674=AXIS2_PLACEMENT_3D('',#38303,#23803,#23804);
#19675=AXIS2_PLACEMENT_3D('',#38309,#23808,#23809);
#19676=AXIS2_PLACEMENT_3D('',#38313,#23812,#23813);
#19677=AXIS2_PLACEMENT_3D('',#38317,#23816,#23817);
#19678=AXIS2_PLACEMENT_3D('',#38321,#23820,#23821);
#19679=AXIS2_PLACEMENT_3D('',#38325,#23824,#23825);
#19680=AXIS2_PLACEMENT_3D('',#38327,#23827,#23828);
#19681=AXIS2_PLACEMENT_3D('',#38329,#23829,#23830);
#19682=AXIS2_PLACEMENT_3D('',#38333,#23833,#23834);
#19683=AXIS2_PLACEMENT_3D('',#38335,#23835,#23836);
#19684=AXIS2_PLACEMENT_3D('',#38342,#23837,#23838);
#19685=AXIS2_PLACEMENT_3D('',#38346,#23840,#23841);
#19686=AXIS2_PLACEMENT_3D('',#38348,#23843,#23844);
#19687=AXIS2_PLACEMENT_3D('',#38357,#23846,#23847);
#19688=AXIS2_PLACEMENT_3D('',#38359,#23848,#23849);
#19689=AXIS2_PLACEMENT_3D('',#38360,#23850,#23851);
#19690=AXIS2_PLACEMENT_3D('',#38361,#23852,#23853);
#19691=AXIS2_PLACEMENT_3D('',#38374,#23860,#23861);
#19692=AXIS2_PLACEMENT_3D('',#38387,#23868,#23869);
#19693=AXIS2_PLACEMENT_3D('',#38400,#23876,#23877);
#19694=AXIS2_PLACEMENT_3D('',#38404,#23880,#23881);
#19695=AXIS2_PLACEMENT_3D('',#38408,#23884,#23885);
#19696=AXIS2_PLACEMENT_3D('',#38410,#23887,#23888);
#19697=AXIS2_PLACEMENT_3D('',#38423,#23895,#23896);
#19698=AXIS2_PLACEMENT_3D('',#38436,#23903,#23904);
#19699=AXIS2_PLACEMENT_3D('',#38442,#23908,#23909);
#19700=AXIS2_PLACEMENT_3D('',#38446,#23912,#23913);
#19701=AXIS2_PLACEMENT_3D('',#38450,#23916,#23917);
#19702=AXIS2_PLACEMENT_3D('',#38454,#23920,#23921);
#19703=AXIS2_PLACEMENT_3D('',#38458,#23924,#23925);
#19704=AXIS2_PLACEMENT_3D('',#38460,#23927,#23928);
#19705=AXIS2_PLACEMENT_3D('',#38465,#23930,#23931);
#19706=AXIS2_PLACEMENT_3D('',#38467,#23933,#23934);
#19707=AXIS2_PLACEMENT_3D('',#38471,#23936,#23937);
#19708=AXIS2_PLACEMENT_3D('',#38472,#23938,#23939);
#19709=AXIS2_PLACEMENT_3D('',#38473,#23940,#23941);
#19710=AXIS2_PLACEMENT_3D('',#38479,#23944,#23945);
#19711=AXIS2_PLACEMENT_3D('',#38481,#23947,#23948);
#19712=AXIS2_PLACEMENT_3D('',#38487,#23952,#23953);
#19713=AXIS2_PLACEMENT_3D('',#38491,#23956,#23957);
#19714=AXIS2_PLACEMENT_3D('',#38495,#23960,#23961);
#19715=AXIS2_PLACEMENT_3D('',#38499,#23964,#23965);
#19716=AXIS2_PLACEMENT_3D('',#38503,#23968,#23969);
#19717=AXIS2_PLACEMENT_3D('',#38505,#23971,#23972);
#19718=AXIS2_PLACEMENT_3D('',#38510,#23974,#23975);
#19719=AXIS2_PLACEMENT_3D('',#38513,#23977,#23978);
#19720=AXIS2_PLACEMENT_3D('',#38514,#23979,#23980);
#19721=AXIS2_PLACEMENT_3D('',#38518,#23982,#23983);
#19722=AXIS2_PLACEMENT_3D('',#38522,#23986,#23987);
#19723=AXIS2_PLACEMENT_3D('',#38528,#23991,#23992);
#19724=AXIS2_PLACEMENT_3D('',#38532,#23995,#23996);
#19725=AXIS2_PLACEMENT_3D('',#38536,#23999,#24000);
#19726=AXIS2_PLACEMENT_3D('',#38540,#24003,#24004);
#19727=AXIS2_PLACEMENT_3D('',#38544,#24007,#24008);
#19728=AXIS2_PLACEMENT_3D('',#38546,#24010,#24011);
#19729=AXIS2_PLACEMENT_3D('',#38562,#24013,#24014);
#19730=AXIS2_PLACEMENT_3D('',#38589,#24015,#24016);
#19731=AXIS2_PLACEMENT_3D('',#38602,#24017,#24018);
#19732=AXIS2_PLACEMENT_3D('',#38614,#24019,#24020);
#19733=AXIS2_PLACEMENT_3D('',#38618,#24022,#24023);
#19734=AXIS2_PLACEMENT_3D('',#38620,#24025,#24026);
#19735=AXIS2_PLACEMENT_3D('',#38622,#24027,#24028);
#19736=AXIS2_PLACEMENT_3D('',#38629,#24029,#24030);
#19737=AXIS2_PLACEMENT_3D('',#38632,#24031,#24032);
#19738=AXIS2_PLACEMENT_3D('',#38635,#24035,#24036);
#19739=AXIS2_PLACEMENT_3D('',#38644,#24038,#24039);
#19740=AXIS2_PLACEMENT_3D('',#38645,#24040,#24041);
#19741=AXIS2_PLACEMENT_3D('',#38646,#24042,#24043);
#19742=AXIS2_PLACEMENT_3D('',#38673,#24044,#24045);
#19743=AXIS2_PLACEMENT_3D('',#38700,#24046,#24047);
#19744=AXIS2_PLACEMENT_3D('',#38716,#24049,#24050);
#19745=AXIS2_PLACEMENT_3D('',#38720,#24054,#24055);
#19746=AXIS2_PLACEMENT_3D('',#38723,#24057,#24058);
#19747=AXIS2_PLACEMENT_3D('',#38843,#24059,#24060);
#19748=AXIS2_PLACEMENT_3D('',#38852,#24064,#24065);
#19749=AXIS2_PLACEMENT_3D('',#38856,#24068,#24069);
#19750=AXIS2_PLACEMENT_3D('',#38857,#24070,#24071);
#19751=AXIS2_PLACEMENT_3D('',#38861,#24073,#24074);
#19752=AXIS2_PLACEMENT_3D('',#38863,#24076,#24077);
#19753=AXIS2_PLACEMENT_3D('',#38866,#24079,#24080);
#19754=AXIS2_PLACEMENT_3D('',#38867,#24081,#24082);
#19755=AXIS2_PLACEMENT_3D('',#38869,#24083,#24084);
#19756=AXIS2_PLACEMENT_3D('',#38873,#24087,#24088);
#19757=AXIS2_PLACEMENT_3D('',#38877,#24090,#24091);
#19758=AXIS2_PLACEMENT_3D('',#38880,#24094,#24095);
#19759=AXIS2_PLACEMENT_3D('',#38886,#24099,#24100);
#19760=AXIS2_PLACEMENT_3D('',#38890,#24103,#24104);
#19761=AXIS2_PLACEMENT_3D('',#38894,#24107,#24108);
#19762=AXIS2_PLACEMENT_3D('',#38898,#24111,#24112);
#19763=AXIS2_PLACEMENT_3D('',#38902,#24115,#24116);
#19764=AXIS2_PLACEMENT_3D('',#38978,#24118,#24119);
#19765=AXIS2_PLACEMENT_3D('',#38982,#24121,#24122);
#19766=AXIS2_PLACEMENT_3D('',#38984,#24124,#24125);
#19767=AXIS2_PLACEMENT_3D('',#38987,#24127,#24128);
#19768=AXIS2_PLACEMENT_3D('',#38988,#24129,#24130);
#19769=AXIS2_PLACEMENT_3D('',#38993,#24133,#24134);
#19770=AXIS2_PLACEMENT_3D('',#38994,#24135,#24136);
#19771=AXIS2_PLACEMENT_3D('',#39000,#24140,#24141);
#19772=AXIS2_PLACEMENT_3D('',#39004,#24144,#24145);
#19773=AXIS2_PLACEMENT_3D('',#39008,#24148,#24149);
#19774=AXIS2_PLACEMENT_3D('',#39012,#24152,#24153);
#19775=AXIS2_PLACEMENT_3D('',#39016,#24156,#24157);
#19776=AXIS2_PLACEMENT_3D('',#39018,#24159,#24160);
#19777=AXIS2_PLACEMENT_3D('',#39024,#24164,#24165);
#19778=AXIS2_PLACEMENT_3D('',#39028,#24168,#24169);
#19779=AXIS2_PLACEMENT_3D('',#39032,#24172,#24173);
#19780=AXIS2_PLACEMENT_3D('',#39036,#24176,#24177);
#19781=AXIS2_PLACEMENT_3D('',#39040,#24180,#24181);
#19782=AXIS2_PLACEMENT_3D('',#39042,#24183,#24184);
#19783=AXIS2_PLACEMENT_3D('',#39043,#24185,#24186);
#19784=AXIS2_PLACEMENT_3D('',#39056,#24193,#24194);
#19785=AXIS2_PLACEMENT_3D('',#39057,#24195,#24196);
#19786=AXIS2_PLACEMENT_3D('',#39070,#24203,#24204);
#19787=AXIS2_PLACEMENT_3D('',#39076,#24208,#24209);
#19788=AXIS2_PLACEMENT_3D('',#39086,#24215,#24216);
#19789=AXIS2_PLACEMENT_3D('',#39092,#24220,#24221);
#19790=AXIS2_PLACEMENT_3D('',#39098,#24225,#24226);
#19791=AXIS2_PLACEMENT_3D('',#39102,#24229,#24230);
#19792=AXIS2_PLACEMENT_3D('',#39106,#24233,#24234);
#19793=AXIS2_PLACEMENT_3D('',#39110,#24237,#24238);
#19794=AXIS2_PLACEMENT_3D('',#39114,#24241,#24242);
#19795=AXIS2_PLACEMENT_3D('',#39116,#24244,#24245);
#19796=AXIS2_PLACEMENT_3D('',#39119,#24246,#24247);
#19797=AXIS2_PLACEMENT_3D('',#39126,#24252,#24253);
#19798=AXIS2_PLACEMENT_3D('',#39130,#24256,#24257);
#19799=AXIS2_PLACEMENT_3D('',#39134,#24260,#24261);
#19800=AXIS2_PLACEMENT_3D('',#39140,#24264,#24265);
#19801=AXIS2_PLACEMENT_3D('',#39142,#24267,#24268);
#19802=AXIS2_PLACEMENT_3D('',#39146,#24271,#24272);
#19803=AXIS2_PLACEMENT_3D('',#39148,#24274,#24275);
#19804=AXIS2_PLACEMENT_3D('',#39149,#24276,#24277);
#19805=AXIS2_PLACEMENT_3D('',#39151,#24279,#24280);
#19806=AXIS2_PLACEMENT_3D('',#39153,#24281,#24282);
#19807=AXIS2_PLACEMENT_3D('',#39231,#24284,#24285);
#19808=AXIS2_PLACEMENT_3D('',#39232,#24286,#24287);
#19809=AXIS2_PLACEMENT_3D('',#39236,#24290,#24291);
#19810=AXIS2_PLACEMENT_3D('',#39237,#24292,#24293);
#19811=AXIS2_PLACEMENT_3D('',#39241,#24295,#24296);
#19812=AXIS2_PLACEMENT_3D('',#39317,#24298,#24299);
#19813=AXIS2_PLACEMENT_3D('',#39323,#24303,#24304);
#19814=AXIS2_PLACEMENT_3D('',#39326,#24305,#24306);
#19815=AXIS2_PLACEMENT_3D('',#39329,#24309,#24310);
#19816=AXIS2_PLACEMENT_3D('',#39333,#24313,#24314);
#19817=AXIS2_PLACEMENT_3D('',#39335,#24316,#24317);
#19818=AXIS2_PLACEMENT_3D('',#39338,#24319,#24320);
#19819=AXIS2_PLACEMENT_3D('',#39339,#24321,#24322);
#19820=AXIS2_PLACEMENT_3D('',#39341,#24323,#24324);
#19821=AXIS2_PLACEMENT_3D('',#39343,#24326,#24327);
#19822=AXIS2_PLACEMENT_3D('',#39345,#24328,#24329);
#19823=AXIS2_PLACEMENT_3D('',#39347,#24331,#24332);
#19824=AXIS2_PLACEMENT_3D('',#39348,#24333,#24334);
#19825=AXIS2_PLACEMENT_3D('',#39354,#24338,#24339);
#19826=AXIS2_PLACEMENT_3D('',#39358,#24342,#24343);
#19827=AXIS2_PLACEMENT_3D('',#39362,#24346,#24347);
#19828=AXIS2_PLACEMENT_3D('',#39366,#24350,#24351);
#19829=AXIS2_PLACEMENT_3D('',#39370,#24354,#24355);
#19830=AXIS2_PLACEMENT_3D('',#39372,#24357,#24358);
#19831=AXIS2_PLACEMENT_3D('',#39374,#24360,#24361);
#19832=AXIS2_PLACEMENT_3D('',#39376,#24363,#24364);
#19833=AXIS2_PLACEMENT_3D('',#39382,#24368,#24369);
#19834=AXIS2_PLACEMENT_3D('',#39386,#24372,#24373);
#19835=AXIS2_PLACEMENT_3D('',#39390,#24376,#24377);
#19836=AXIS2_PLACEMENT_3D('',#39392,#24379,#24380);
#19837=AXIS2_PLACEMENT_3D('',#39394,#24382,#24383);
#19838=AXIS2_PLACEMENT_3D('',#39395,#24384,#24385);
#19839=AXIS2_PLACEMENT_3D('',#39397,#24387,#24388);
#19840=AXIS2_PLACEMENT_3D('',#39400,#24391,#24392);
#19841=AXIS2_PLACEMENT_3D('',#39404,#24394,#24395);
#19842=AXIS2_PLACEMENT_3D('',#39405,#24396,#24397);
#19843=AXIS2_PLACEMENT_3D('',#39409,#24399,#24400);
#19844=AXIS2_PLACEMENT_3D('',#39410,#24401,#24402);
#19845=AXIS2_PLACEMENT_3D('',#39412,#24404,#24405);
#19846=AXIS2_PLACEMENT_3D('',#39416,#24408,#24409);
#19847=AXIS2_PLACEMENT_3D('',#39419,#24410,#24411);
#19848=AXIS2_PLACEMENT_3D('',#39421,#24413,#24414);
#19849=AXIS2_PLACEMENT_3D('',#39422,#24415,#24416);
#19850=AXIS2_PLACEMENT_3D('',#39426,#24419,#24420);
#19851=AXIS2_PLACEMENT_3D('',#39429,#24421,#24422);
#19852=AXIS2_PLACEMENT_3D('',#39431,#24424,#24425);
#19853=AXIS2_PLACEMENT_3D('',#39432,#24426,#24427);
#19854=AXIS2_PLACEMENT_3D('',#39435,#24430,#24431);
#19855=AXIS2_PLACEMENT_3D('',#39437,#24433,#24434);
#19856=AXIS2_PLACEMENT_3D('',#39441,#24436,#24437);
#19857=AXIS2_PLACEMENT_3D('',#39442,#24438,#24439);
#19858=AXIS2_PLACEMENT_3D('',#39446,#24441,#24442);
#19859=AXIS2_PLACEMENT_3D('',#39447,#24443,#24444);
#19860=AXIS2_PLACEMENT_3D('',#39449,#24445,#24446);
#19861=AXIS2_PLACEMENT_3D('',#39450,#24447,#24448);
#19862=AXIS2_PLACEMENT_3D('',#39451,#24449,#24450);
#19863=AXIS2_PLACEMENT_3D('',#39453,#24451,#24452);
#19864=AXIS2_PLACEMENT_3D('',#39455,#24453,#24454);
#19865=AXIS2_PLACEMENT_3D('',#39464,#24455,#24456);
#19866=AXIS2_PLACEMENT_3D('',#39466,#24457,#24458);
#19867=AXIS2_PLACEMENT_3D('',#39468,#24459,#24460);
#19868=AXIS2_PLACEMENT_3D('',#39470,#24461,#24462);
#19869=AXIS2_PLACEMENT_3D('',#39472,#24463,#24464);
#19870=AXIS2_PLACEMENT_3D('',#39473,#24465,#24466);
#19871=AXIS2_PLACEMENT_3D('',#39474,#24467,#24468);
#19872=AXIS2_PLACEMENT_3D('',#39483,#24469,#24470);
#19873=AXIS2_PLACEMENT_3D('',#39484,#24471,#24472);
#19874=AXIS2_PLACEMENT_3D('',#39485,#24473,#24474);
#19875=AXIS2_PLACEMENT_3D('',#39486,#24475,#24476);
#19876=AXIS2_PLACEMENT_3D('',#39498,#24483,#24484);
#19877=AXIS2_PLACEMENT_3D('',#39502,#24487,#24488);
#19878=AXIS2_PLACEMENT_3D('',#39508,#24492,#24493);
#19879=AXIS2_PLACEMENT_3D('',#39512,#24496,#24497);
#19880=AXIS2_PLACEMENT_3D('',#39518,#24501,#24502);
#19881=AXIS2_PLACEMENT_3D('',#39522,#24505,#24506);
#19882=AXIS2_PLACEMENT_3D('',#39542,#24517,#24518);
#19883=AXIS2_PLACEMENT_3D('',#39546,#24521,#24522);
#19884=AXIS2_PLACEMENT_3D('',#39552,#24526,#24527);
#19885=AXIS2_PLACEMENT_3D('',#39556,#24530,#24531);
#19886=AXIS2_PLACEMENT_3D('',#39562,#24535,#24536);
#19887=AXIS2_PLACEMENT_3D('',#39566,#24539,#24540);
#19888=AXIS2_PLACEMENT_3D('',#39576,#24546,#24547);
#19889=AXIS2_PLACEMENT_3D('',#39582,#24551,#24552);
#19890=AXIS2_PLACEMENT_3D('',#39584,#24553,#24554);
#19891=AXIS2_PLACEMENT_3D('',#39587,#24557,#24558);
#19892=AXIS2_PLACEMENT_3D('',#39590,#24559,#24560);
#19893=AXIS2_PLACEMENT_3D('',#39593,#24563,#24564);
#19894=AXIS2_PLACEMENT_3D('',#39596,#24565,#24566);
#19895=AXIS2_PLACEMENT_3D('',#39599,#24569,#24570);
#19896=AXIS2_PLACEMENT_3D('',#39608,#24577,#24578);
#19897=AXIS2_PLACEMENT_3D('',#39612,#24581,#24582);
#19898=AXIS2_PLACEMENT_3D('',#39614,#24584,#24585);
#19899=AXIS2_PLACEMENT_3D('',#39616,#24587,#24588);
#19900=AXIS2_PLACEMENT_3D('',#39620,#24591,#24592);
#19901=AXIS2_PLACEMENT_3D('',#39624,#24595,#24596);
#19902=AXIS2_PLACEMENT_3D('',#39632,#24602,#24603);
#19903=AXIS2_PLACEMENT_3D('',#39633,#24604,#24605);
#19904=AXIS2_PLACEMENT_3D('',#39634,#24606,#24607);
#19905=AXIS2_PLACEMENT_3D('',#39640,#24608,#24609);
#19906=AXIS2_PLACEMENT_3D('',#39641,#24610,#24611);
#19907=AXIS2_PLACEMENT_3D('',#39643,#24612,#24613);
#19908=AXIS2_PLACEMENT_3D('',#39648,#24614,#24615);
#19909=AXIS2_PLACEMENT_3D('',#39654,#24616,#24617);
#19910=AXIS2_PLACEMENT_3D('',#39655,#24618,#24619);
#19911=AXIS2_PLACEMENT_3D('',#39656,#24620,#24621);
#19912=AXIS2_PLACEMENT_3D('',#39657,#24622,#24623);
#19913=AXIS2_PLACEMENT_3D('',#39665,#24628,#24629);
#19914=AXIS2_PLACEMENT_3D('',#39671,#24633,#24634);
#19915=AXIS2_PLACEMENT_3D('',#39675,#24637,#24638);
#19916=AXIS2_PLACEMENT_3D('',#39677,#24640,#24641);
#19917=AXIS2_PLACEMENT_3D('',#39679,#24643,#24644);
#19918=AXIS2_PLACEMENT_3D('',#39682,#24647,#24648);
#19919=AXIS2_PLACEMENT_3D('',#39688,#24652,#24653);
#19920=AXIS2_PLACEMENT_3D('',#39692,#24656,#24657);
#19921=AXIS2_PLACEMENT_3D('',#39696,#24660,#24661);
#19922=AXIS2_PLACEMENT_3D('',#39702,#24665,#24666);
#19923=AXIS2_PLACEMENT_3D('',#39708,#24670,#24671);
#19924=AXIS2_PLACEMENT_3D('',#39712,#24674,#24675);
#19925=AXIS2_PLACEMENT_3D('',#39716,#24678,#24679);
#19926=AXIS2_PLACEMENT_3D('',#39718,#24681,#24682);
#19927=AXIS2_PLACEMENT_3D('',#39720,#24684,#24685);
#19928=AXIS2_PLACEMENT_3D('',#39722,#24687,#24688);
#19929=AXIS2_PLACEMENT_3D('',#39730,#24693,#24694);
#19930=AXIS2_PLACEMENT_3D('',#39734,#24697,#24698);
#19931=AXIS2_PLACEMENT_3D('',#39740,#24702,#24703);
#19932=AXIS2_PLACEMENT_3D('',#39746,#24707,#24708);
#19933=AXIS2_PLACEMENT_3D('',#39750,#24711,#24712);
#19934=AXIS2_PLACEMENT_3D('',#39754,#24715,#24716);
#19935=AXIS2_PLACEMENT_3D('',#39758,#24719,#24720);
#19936=AXIS2_PLACEMENT_3D('',#39762,#24723,#24724);
#19937=AXIS2_PLACEMENT_3D('',#39766,#24727,#24728);
#19938=AXIS2_PLACEMENT_3D('',#39770,#24731,#24732);
#19939=AXIS2_PLACEMENT_3D('',#39774,#24735,#24736);
#19940=AXIS2_PLACEMENT_3D('',#39778,#24739,#24740);
#19941=AXIS2_PLACEMENT_3D('',#39782,#24743,#24744);
#19942=AXIS2_PLACEMENT_3D('',#39786,#24747,#24748);
#19943=AXIS2_PLACEMENT_3D('',#39788,#24750,#24751);
#21398=DIRECTION('axis',(0.,0.,1.));
#21399=DIRECTION('refdir',(1.,0.,0.));
#21400=DIRECTION('center_axis',(-3.54454368418083E-15,1.14635476884388E-13,
1.));
#21401=DIRECTION('ref_axis',(1.,0.,4.17966315152979E-15));
#21402=DIRECTION('center_axis',(9.64418253237272E-27,-1.07981213846331E-13,
-1.));
#21403=DIRECTION('ref_axis',(-8.4885105576653E-14,1.,-1.07981213846331E-13));
#21404=DIRECTION('center_axis',(-1.30614473484947E-16,1.,-1.14635476884388E-13));
#21405=DIRECTION('ref_axis',(-1.,-1.30614473485306E-16,-3.13474736364734E-15));
#21406=DIRECTION('center_axis',(1.00515054169548E-26,-1.1518563880486E-13,
-1.));
#21407=DIRECTION('ref_axis',(-8.54871728961371E-14,1.,-1.1518563880486E-13));
#21408=DIRECTION('center_axis',(1.00515054169548E-26,-1.1518563880486E-13,
-1.));
#21409=DIRECTION('ref_axis',(-8.54871728961371E-14,1.,-1.1518563880486E-13));
#21410=DIRECTION('center_axis',(-9.8017643219864E-16,1.15516038958398E-13,
1.));
#21411=DIRECTION('ref_axis',(1.,0.,8.88178419700135E-16));
#21412=DIRECTION('center_axis',(-1.00515054169548E-26,1.1518563880486E-13,
1.));
#21413=DIRECTION('ref_axis',(8.72635297355373E-14,-1.,1.1518563880486E-13));
#21414=DIRECTION('center_axis',(1.38777878078018E-16,-1.,1.15516038958398E-13));
#21415=DIRECTION('ref_axis',(-1.,-1.38777878078146E-16,-1.11022302462517E-15));
#21416=DIRECTION('center_axis',(-1.00515054169548E-26,1.1518563880486E-13,
1.));
#21417=DIRECTION('ref_axis',(-8.72635297355373E-14,1.,-1.1518563880486E-13));
#21418=DIRECTION('center_axis',(-1.00515054169548E-26,1.1518563880486E-13,
1.));
#21419=DIRECTION('ref_axis',(-8.72635297355373E-14,1.,-1.1518563880486E-13));
#21420=DIRECTION('center_axis',(-1.00515054169548E-26,1.1518563880486E-13,
1.));
#21421=DIRECTION('ref_axis',(8.72635297355373E-14,-1.,1.1518563880486E-13));
#21422=DIRECTION('center_axis',(7.85454768979583E-16,1.15103843509475E-13,
1.));
#21423=DIRECTION('ref_axis',(1.,0.,-5.74175948088969E-16));
#21424=DIRECTION('center_axis',(-1.00515054169548E-26,1.1518563880486E-13,
1.));
#21425=DIRECTION('ref_axis',(-8.72635297355373E-14,1.,-1.1518563880486E-13));
#21426=DIRECTION('center_axis',(-1.34572487833435E-16,1.,-1.15103843509475E-13));
#21427=DIRECTION('ref_axis',(-1.,-1.34572487833352E-16,7.17719935111211E-16));
#21428=DIRECTION('center_axis',(-1.00515054169548E-26,1.1518563880486E-13,
1.));
#21429=DIRECTION('ref_axis',(-8.72635297355373E-14,1.,-1.1518563880486E-13));
#21430=DIRECTION('center_axis',(-1.00515054169548E-26,1.1518563880486E-13,
1.));
#21431=DIRECTION('ref_axis',(-8.72635297355373E-14,1.,-1.1518563880486E-13));
#21432=DIRECTION('center_axis',(-1.00515054169548E-26,1.1518563880486E-13,
1.));
#21433=DIRECTION('ref_axis',(-8.72635297355373E-14,1.,-1.1518563880486E-13));
#21434=DIRECTION('center_axis',(2.09517191469308E-15,1.14089507593872E-13,
1.));
#21435=DIRECTION('ref_axis',(1.,0.,-2.18628534080032E-15));
#21436=DIRECTION('center_axis',(-1.00515054169548E-26,1.1518563880486E-13,
1.));
#21437=DIRECTION('ref_axis',(8.72635297355373E-14,-1.,1.1518563880486E-13));
#21438=DIRECTION('center_axis',(-1.13869028166891E-16,1.,-1.14089507593872E-13));
#21439=DIRECTION('ref_axis',(-1.,-1.13869028166684E-16,1.82190445066694E-15));
#21440=DIRECTION('center_axis',(1.00515054169548E-26,-1.1518563880486E-13,
-1.));
#21441=DIRECTION('ref_axis',(8.72635297355373E-14,-1.,1.1518563880486E-13));
#21442=DIRECTION('center_axis',(1.00515054169548E-26,-1.1518563880486E-13,
-1.));
#21443=DIRECTION('ref_axis',(8.72635297355373E-14,-1.,1.1518563880486E-13));
#21444=DIRECTION('center_axis',(-1.00515054169548E-26,1.1518563880486E-13,
1.));
#21445=DIRECTION('ref_axis',(8.72635297355373E-14,-1.,1.1518563880486E-13));
#21446=DIRECTION('center_axis',(-1.00515054169548E-26,1.1518563880486E-13,
1.));
#21447=DIRECTION('ref_axis',(-8.72635297355373E-14,1.,-1.1518563880486E-13));
#21448=DIRECTION('center_axis',(2.90839696048352E-15,1.12070336644323E-13,
1.));
#21449=DIRECTION('ref_axis',(1.,8.67992546525122E-14,-3.22973970800046E-15));
#21450=DIRECTION('',(-1.00515054169548E-26,1.1518563880486E-13,1.));
#21451=DIRECTION('center_axis',(-8.92186509493858E-16,1.14732495036932E-13,
1.));
#21452=DIRECTION('ref_axis',(8.6535488860372E-14,-1.,1.14978733604816E-13));
#21453=DIRECTION('center_axis',(1.00515054169548E-26,-1.1518563880486E-13,
-1.));
#21454=DIRECTION('ref_axis',(8.72635297355373E-14,-1.,1.1518563880486E-13));
#21455=DIRECTION('',(8.21476117669779E-14,-0.94269689858097,0.333650352024124));
#21456=DIRECTION('center_axis',(-1.00515054169548E-26,1.1518563880486E-13,
1.));
#21457=DIRECTION('ref_axis',(-8.72635297355373E-14,1.,-1.1518563880486E-13));
#21458=DIRECTION('',(4.00335205749406E-14,-0.458122847290751,0.888888888888941));
#21459=DIRECTION('center_axis',(-1.00489519728121E-26,1.15107923193136E-13,
1.));
#21460=DIRECTION('ref_axis',(-8.71826535283427E-14,1.,-1.15107923193136E-13));
#21461=DIRECTION('center_axis',(1.00515054169548E-26,-1.1518563880486E-13,
-1.));
#21462=DIRECTION('ref_axis',(8.72635297355373E-14,-1.,1.1518563880486E-13));
#21463=DIRECTION('',(7.26903855506451E-14,-0.834169119969402,0.551508730021088));
#21464=DIRECTION('center_axis',(1.00515054169548E-26,-1.1518563880486E-13,
-1.));
#21465=DIRECTION('ref_axis',(8.72635297355373E-14,-1.,1.1518563880486E-13));
#21466=DIRECTION('',(8.70424333714333E-14,-0.998868137724432,0.0475651494155674));
#21467=DIRECTION('center_axis',(-1.00515054169548E-26,1.1518563880486E-13,
1.));
#21468=DIRECTION('ref_axis',(-8.72635297355373E-14,1.,-1.1518563880486E-13));
#21469=DIRECTION('center_axis',(1.00515054169548E-26,-1.1518563880486E-13,
-1.));
#21470=DIRECTION('ref_axis',(8.72635297355373E-14,-1.,1.1518563880486E-13));
#21471=DIRECTION('center_axis',(-8.72635297355373E-14,1.,-1.1518563880486E-13));
#21472=DIRECTION('ref_axis',(1.0285184916872E-26,-1.1518563880486E-13,-1.));
#21473=DIRECTION('center_axis',(8.72635297355373E-14,-1.,1.1518563880486E-13));
#21474=DIRECTION('ref_axis',(-1.86517468136924E-14,-1.15185638804862E-13,
-1.));
#21475=DIRECTION('center_axis',(8.72635297355373E-14,-1.,1.1518563880486E-13));
#21476=DIRECTION('ref_axis',(-1.86517468136924E-14,-1.15185638804862E-13,
-1.));
#21477=DIRECTION('',(8.55449136515341E-14,-0.980580675690943,-0.196116135138071));
#21478=DIRECTION('center_axis',(-9.43689570926916E-14,1.,1.83186799062301E-13));
#21479=DIRECTION('ref_axis',(6.03740488023232E-15,-1.77635683939193E-13,
1.));
#21480=DIRECTION('center_axis',(8.72635297355373E-14,-1.,1.1518563880486E-13));
#21481=DIRECTION('ref_axis',(-1.06184991926244E-26,1.1518563880486E-13,
1.));
#21482=DIRECTION('',(7.81056416479254E-14,-0.894427190999967,-0.447213595499855));
#21483=DIRECTION('center_axis',(8.88178419730948E-14,-1.,7.10542735786571E-13));
#21484=DIRECTION('ref_axis',(7.57155095484643E-15,7.10542735786545E-13,
1.));
#21485=DIRECTION('center_axis',(8.72635297355373E-14,-1.,1.1518563880486E-13));
#21486=DIRECTION('ref_axis',(-1.00515054169548E-26,1.1518563880486E-13,
1.));
#21487=DIRECTION('center_axis',(8.72635297355373E-14,-1.,1.1518563880486E-13));
#21488=DIRECTION('ref_axis',(-9.82963828734632E-27,1.1518563880486E-13,
1.));
#21489=DIRECTION('',(7.81056416599154E-14,-0.894427191137758,-0.447213595224274));
#21490=DIRECTION('center_axis',(-8.72635297355373E-14,1.,-1.1518563880486E-13));
#21491=DIRECTION('ref_axis',(-9.82963828734632E-27,1.1518563880486E-13,
1.));
#21492=DIRECTION('center_axis',(-8.72635297355373E-14,1.,-1.1518563880486E-13));
#21493=DIRECTION('ref_axis',(1.00515054169548E-26,-1.1518563880486E-13,
-1.));
#21494=DIRECTION('center_axis',(1.,8.72635297355373E-14,0.));
#21495=DIRECTION('ref_axis',(8.72635297355373E-14,-1.,1.1518563880486E-13));
#21496=DIRECTION('',(4.36317648660981E-14,-0.499999999980857,-0.866025403795491));
#21497=DIRECTION('',(-4.36317648660809E-14,0.49999999998066,-0.866025403795605));
#21498=DIRECTION('',(-8.72635297355373E-14,1.,-1.1518563880486E-13));
#21499=DIRECTION('',(-4.36317648660983E-14,0.499999999980859,0.86602540379549));
#21500=DIRECTION('',(4.36317648660808E-14,-0.499999999980657,0.866025403795606));
#21501=DIRECTION('',(8.72635297355373E-14,-1.,1.1518563880486E-13));
#21502=DIRECTION('center_axis',(7.55724335758485E-14,-0.866025403795606,
-0.499999999980658));
#21503=DIRECTION('ref_axis',(4.36317648660808E-14,-0.499999999980658,0.866025403795606));
#21504=DIRECTION('',(1.,8.72635297355373E-14,0.));
#21505=DIRECTION('',(-1.,-8.72635297355373E-14,0.));
#21506=DIRECTION('',(4.36317648660808E-14,-0.499999999980658,0.866025403795606));
#21507=DIRECTION('center_axis',(7.55724335758385E-14,-0.86602540379549,
0.499999999980858));
#21508=DIRECTION('ref_axis',(-4.36317648660983E-14,0.499999999980858,0.86602540379549));
#21509=DIRECTION('',(-1.,-8.72635297355373E-14,0.));
#21510=DIRECTION('',(-4.36317648660983E-14,0.499999999980858,0.86602540379549));
#21511=DIRECTION('center_axis',(-1.00515054169548E-26,1.1518563880486E-13,
1.));
#21512=DIRECTION('ref_axis',(-8.72635297355373E-14,1.,-1.1518563880486E-13));
#21513=DIRECTION('',(-1.,-8.72635297355373E-14,0.));
#21514=DIRECTION('',(0.133254699246628,0.991081825647454,-1.14158393195087E-13));
#21515=DIRECTION('',(-8.72635297355373E-14,1.,-1.1518563880486E-13));
#21516=DIRECTION('center_axis',(-7.55724335758485E-14,0.866025403795606,
0.499999999980658));
#21517=DIRECTION('ref_axis',(-4.36317648660808E-14,0.499999999980658,-0.866025403795606));
#21518=DIRECTION('',(-1.,-8.72635297355373E-14,0.));
#21519=DIRECTION('',(0.0670754893014342,0.498873951679673,-0.864075030926412));
#21520=DIRECTION('center_axis',(-7.55724335758385E-14,0.86602540379549,
-0.499999999980858));
#21521=DIRECTION('ref_axis',(4.36317648660983E-14,-0.499999999980858,-0.86602540379549));
#21522=DIRECTION('',(-1.,-8.72635297355373E-14,0.));
#21523=DIRECTION('',(-0.0670754893014346,-0.498873951679872,-0.864075030926297));
#21524=DIRECTION('center_axis',(1.00515054169548E-26,-1.1518563880486E-13,
-1.));
#21525=DIRECTION('ref_axis',(8.72635297355373E-14,-1.,1.1518563880486E-13));
#21526=DIRECTION('',(-0.133254699246661,-0.99108182564745,1.14158393195087E-13));
#21527=DIRECTION('',(8.72635297355373E-14,-1.,1.1518563880486E-13));
#21528=DIRECTION('center_axis',(-1.,-8.72635297355373E-14,0.));
#21529=DIRECTION('ref_axis',(-8.72635297355373E-14,1.,-1.1518563880486E-13));
#21530=DIRECTION('',(1.00515054169548E-26,-1.1518563880486E-13,-1.));
#21531=DIRECTION('center_axis',(-0.991081825647454,0.133254699246628,-1.53490276564824E-14));
#21532=DIRECTION('ref_axis',(0.133254699246628,0.991081825647454,-1.14158393195087E-13));
#21533=DIRECTION('',(-0.585068654159542,-0.386550578869277,-0.712932899995342));
#21534=DIRECTION('',(-0.35948002755914,-0.539309464528629,-0.761524399645818));
#21535=DIRECTION('',(-0.379976420578218,-0.590823050535381,-0.711720480779239));
#21536=DIRECTION('center_axis',(4.08987016959577E-16,-1.15239837533439E-13,
-1.));
#21537=DIRECTION('ref_axis',(-1.,0.,-3.13169680337459E-16));
#21538=DIRECTION('center_axis',(1.00515054169548E-26,-1.1518563880486E-13,
-1.));
#21539=DIRECTION('ref_axis',(8.72635297355373E-14,-1.,1.1518563880486E-13));
#21540=DIRECTION('center_axis',(-1.22464679914813E-16,-1.,1.15239837533439E-13));
#21541=DIRECTION('ref_axis',(1.,-1.22464679914768E-16,3.91462100421824E-16));
#21542=DIRECTION('center_axis',(1.00515054169548E-26,-1.1518563880486E-13,
-1.));
#21543=DIRECTION('ref_axis',(-8.72635297355373E-14,1.,-1.1518563880486E-13));
#21544=DIRECTION('center_axis',(1.00515054169548E-26,-1.1518563880486E-13,
-1.));
#21545=DIRECTION('ref_axis',(-8.72635297355373E-14,1.,-1.1518563880486E-13));
#21546=DIRECTION('center_axis',(-8.72635297355373E-14,1.,-1.1518563880486E-13));
#21547=DIRECTION('ref_axis',(4.48527684827171E-30,-1.1518563880486E-13,
-1.));
#21548=DIRECTION('center_axis',(-8.72635297355373E-14,1.,-1.1518563880486E-13));
#21549=DIRECTION('ref_axis',(4.48527684827171E-30,-1.1518563880486E-13,
-1.));
#21550=DIRECTION('',(-8.72635297355373E-14,1.,-1.1518563880486E-13));
#21551=DIRECTION('center_axis',(8.72635297355373E-14,-1.,1.1518563880486E-13));
#21552=DIRECTION('ref_axis',(4.48527684827171E-30,-1.1518563880486E-13,
-1.));
#21553=DIRECTION('center_axis',(-8.72635297355373E-14,1.,-1.1518563880486E-13));
#21554=DIRECTION('ref_axis',(4.48527684826454E-30,-1.1518563880486E-13,
-1.));
#21555=DIRECTION('center_axis',(-8.72635297355373E-14,1.,-1.1518563880486E-13));
#21556=DIRECTION('ref_axis',(4.48527684826454E-30,-1.1518563880486E-13,
-1.));
#21557=DIRECTION('',(-8.72635297355373E-14,1.,-1.1518563880486E-13));
#21558=DIRECTION('center_axis',(8.72635297355373E-14,-1.,1.1518563880486E-13));
#21559=DIRECTION('ref_axis',(4.48527684826023E-30,-1.1518563880486E-13,
-1.));
#21560=DIRECTION('center_axis',(-8.72635297355373E-14,1.,-1.1518563880486E-13));
#21561=DIRECTION('ref_axis',(4.48527684827171E-30,-1.1518563880486E-13,
-1.));
#21562=DIRECTION('center_axis',(-8.72635297355373E-14,1.,-1.1518563880486E-13));
#21563=DIRECTION('ref_axis',(4.48527684827171E-30,-1.1518563880486E-13,
-1.));
#21564=DIRECTION('',(-8.72635297355373E-14,1.,-1.1518563880486E-13));
#21565=DIRECTION('center_axis',(8.72635297355373E-14,-1.,1.1518563880486E-13));
#21566=DIRECTION('ref_axis',(4.48527684827171E-30,-1.1518563880486E-13,
-1.));
#21567=DIRECTION('center_axis',(-8.72635297355373E-14,1.,-1.1518563880486E-13));
#21568=DIRECTION('ref_axis',(4.48527684826454E-30,-1.1518563880486E-13,
-1.));
#21569=DIRECTION('center_axis',(-8.72635297355373E-14,1.,-1.1518563880486E-13));
#21570=DIRECTION('ref_axis',(4.48527684826454E-30,-1.1518563880486E-13,
-1.));
#21571=DIRECTION('',(-8.72635297355373E-14,1.,-1.1518563880486E-13));
#21572=DIRECTION('center_axis',(8.72635297355373E-14,-1.,1.1518563880486E-13));
#21573=DIRECTION('ref_axis',(4.48527684826023E-30,-1.1518563880486E-13,
-1.));
#21574=DIRECTION('center_axis',(1.,8.72635297355373E-14,0.));
#21575=DIRECTION('ref_axis',(8.72635297355373E-14,-1.,1.1498738469332E-13));
#21576=DIRECTION('center_axis',(1.,8.72635297355373E-14,0.));
#21577=DIRECTION('ref_axis',(8.72635297355373E-14,-1.,1.1498738469332E-13));
#21578=DIRECTION('center_axis',(0.988934829411352,0.148350608954393,-5.96763239577493E-15));
#21579=DIRECTION('ref_axis',(0.148350608954393,-0.988934829411352,-6.02957470936365E-12));
#21580=DIRECTION('',(-1.,-8.72635297355373E-14,0.));
#21581=DIRECTION('center_axis',(1.,8.72635297355373E-14,0.));
#21582=DIRECTION('ref_axis',(8.72635297355373E-14,-1.,1.1498738469332E-13));
#21583=DIRECTION('center_axis',(0.988934829411352,0.148350608954393,-5.96763239577493E-15));
#21584=DIRECTION('ref_axis',(0.148350608954393,-0.988934829411352,-6.02957470936365E-12));
#21585=DIRECTION('center_axis',(1.00515054169548E-26,-1.1518563880486E-13,
-1.));
#21586=DIRECTION('ref_axis',(8.73039014818873E-14,-1.,1.1518563880486E-13));
#21587=DIRECTION('center_axis',(1.00515054169548E-26,-1.1518563880486E-13,
-1.));
#21588=DIRECTION('ref_axis',(8.73039014818873E-14,-1.,1.1518563880486E-13));
#21589=DIRECTION('center_axis',(-1.00515054169548E-26,1.1518563880486E-13,
1.));
#21590=DIRECTION('ref_axis',(8.73039014818873E-14,-1.,1.1518563880486E-13));
#21591=DIRECTION('center_axis',(1.00515054169548E-26,-1.1518563880486E-13,
-1.));
#21592=DIRECTION('ref_axis',(8.72635297355373E-14,-1.,1.1518563880486E-13));
#21593=DIRECTION('center_axis',(1.00515054169548E-26,-1.1518563880486E-13,
-1.));
#21594=DIRECTION('ref_axis',(8.72635297355373E-14,-1.,1.1518563880486E-13));
#21595=DIRECTION('center_axis',(1.00515054169548E-26,-1.1518563880486E-13,
-1.));
#21596=DIRECTION('ref_axis',(8.72635297355373E-14,-1.,1.1518563880486E-13));
#21597=DIRECTION('center_axis',(-1.00515054169548E-26,1.1518563880486E-13,
1.));
#21598=DIRECTION('ref_axis',(8.72635297355373E-14,-1.,1.1518563880486E-13));
#21599=DIRECTION('center_axis',(-1.00515054169548E-26,1.1518563880486E-13,
1.));
#21600=DIRECTION('ref_axis',(8.72635297355373E-14,-1.,1.1518563880486E-13));
#21601=DIRECTION('center_axis',(1.00515054169548E-26,-1.1518563880486E-13,
-1.));
#21602=DIRECTION('ref_axis',(8.72092802013795E-14,-1.,1.1518563880486E-13));
#21603=DIRECTION('center_axis',(1.00515054169548E-26,-1.1518563880486E-13,
-1.));
#21604=DIRECTION('ref_axis',(8.72092802013795E-14,-1.,1.1518563880486E-13));
#21605=DIRECTION('center_axis',(-1.00515054169548E-26,1.1518563880486E-13,
1.));
#21606=DIRECTION('ref_axis',(8.72092802013795E-14,-1.,1.1518563880486E-13));
#21607=DIRECTION('center_axis',(1.00515054169548E-26,-1.1518563880486E-13,
-1.));
#21608=DIRECTION('ref_axis',(8.72318090776909E-14,-1.,1.1518563880486E-13));
#21609=DIRECTION('center_axis',(-1.00515054169548E-26,1.1518563880486E-13,
1.));
#21610=DIRECTION('ref_axis',(8.72318090776909E-14,-1.,1.1518563880486E-13));
#21611=DIRECTION('',(-1.00515054169548E-26,1.1518563880486E-13,1.));
#21612=DIRECTION('center_axis',(1.00515054169548E-26,-1.1518563880486E-13,
-1.));
#21613=DIRECTION('ref_axis',(8.72318090776909E-14,-1.,1.1518563880486E-13));
#21614=DIRECTION('center_axis',(1.,8.72635297355373E-14,0.));
#21615=DIRECTION('ref_axis',(8.72635297355373E-14,-1.,1.1498738469332E-13));
#21616=DIRECTION('center_axis',(-1.,-8.72635297355373E-14,0.));
#21617=DIRECTION('ref_axis',(8.72635297355373E-14,-1.,1.1498738469332E-13));
#21618=DIRECTION('',(-1.,-8.72635297355373E-14,0.));
#21619=DIRECTION('center_axis',(-1.,-8.72635297355373E-14,0.));
#21620=DIRECTION('ref_axis',(8.72635297355373E-14,-1.,1.1498738469332E-13));
#21621=DIRECTION('center_axis',(-1.,-8.72635297355373E-14,0.));
#21622=DIRECTION('ref_axis',(8.72635297355373E-14,-1.,1.16969925808722E-13));
#21623=DIRECTION('center_axis',(-1.,-8.72635297355373E-14,0.));
#21624=DIRECTION('ref_axis',(8.72635297355373E-14,-1.,1.18952466924124E-13));
#21625=DIRECTION('center_axis',(1.,8.72635297355373E-14,0.));
#21626=DIRECTION('ref_axis',(8.72635297355373E-14,-1.,1.1498738469332E-13));
#21627=DIRECTION('center_axis',(1.,8.72635297355373E-14,0.));
#21628=DIRECTION('ref_axis',(8.72635297355373E-14,-1.,1.1498738469332E-13));
#21629=DIRECTION('center_axis',(0.991081825647456,-0.133254699246617,2.83668489712038E-13));
#21630=DIRECTION('ref_axis',(0.133254699246616,0.991081825647456,-1.1265578716007E-10));
#21631=DIRECTION('center_axis',(-1.,-8.72635297355373E-14,0.));
#21632=DIRECTION('ref_axis',(8.72635297355373E-14,-1.,1.1498738469332E-13));
#21633=DIRECTION('',(-1.,-8.72635297355373E-14,0.));
#21634=DIRECTION('center_axis',(1.,8.72635297355373E-14,0.));
#21635=DIRECTION('ref_axis',(8.72635297355373E-14,-1.,1.1498738469332E-13));
#21636=DIRECTION('center_axis',(-1.,-8.72635297355373E-14,0.));
#21637=DIRECTION('ref_axis',(8.72635297355373E-14,-1.,1.1498738469332E-13));
#21638=DIRECTION('center_axis',(0.991081825647462,-0.133254699246573,-3.75601193874917E-13));
#21639=DIRECTION('ref_axis',(0.133254699246573,0.991081825647462,4.6681475548608E-11));
#21640=DIRECTION('center_axis',(1.00515054169548E-26,-1.1518563880486E-13,
-1.));
#21641=DIRECTION('ref_axis',(8.72635297355373E-14,-1.,1.1518563880486E-13));
#21642=DIRECTION('center_axis',(-1.00515054169548E-26,1.1518563880486E-13,
1.));
#21643=DIRECTION('ref_axis',(8.72635297355373E-14,-1.,1.1518563880486E-13));
#21644=DIRECTION('',(-1.00515054169548E-26,1.1518563880486E-13,1.));
#21645=DIRECTION('center_axis',(-1.00515054169548E-26,1.1518563880486E-13,
1.));
#21646=DIRECTION('ref_axis',(8.72635297355373E-14,-1.,1.1518563880486E-13));
#21647=DIRECTION('center_axis',(1.00515054169548E-26,-1.1518563880486E-13,
-1.));
#21648=DIRECTION('ref_axis',(8.72635297355373E-14,-1.,1.1518563880486E-13));
#21649=DIRECTION('center_axis',(-1.00515054169548E-26,1.1518563880486E-13,
1.));
#21650=DIRECTION('ref_axis',(8.72635297355373E-14,-1.,1.1518563880486E-13));
#21651=DIRECTION('',(-1.00515054169548E-26,1.1518563880486E-13,1.));
#21652=DIRECTION('center_axis',(1.00515054169548E-26,-1.1518563880486E-13,
-1.));
#21653=DIRECTION('ref_axis',(8.72635297355373E-14,-1.,1.1518563880486E-13));
#21654=DIRECTION('center_axis',(9.74874922969709E-27,-1.11716191852906E-13,
-1.));
#21655=DIRECTION('ref_axis',(8.73144149574993E-14,-1.,1.11716191852906E-13));
#21656=DIRECTION('',(-9.74874922969709E-27,1.11716191852906E-13,1.));
#21657=DIRECTION('',(9.74874922969709E-27,-1.11716191852906E-13,-1.));
#21658=DIRECTION('center_axis',(9.74874922969709E-27,-1.11716191852906E-13,
-1.));
#21659=DIRECTION('ref_axis',(8.73144149574993E-14,-1.,1.11716191852906E-13));
#21660=DIRECTION('',(-9.74874922969709E-27,1.11716191852906E-13,1.));
#21661=DIRECTION('',(9.74874922969709E-27,-1.11716191852906E-13,-1.));
#21662=DIRECTION('center_axis',(9.74874922969709E-27,-1.11716191852906E-13,
-1.));
#21663=DIRECTION('ref_axis',(8.73144149574993E-14,-1.,1.11716191852906E-13));
#21664=DIRECTION('center_axis',(-0.86602540378444,-1.44241112198798E-13,
-0.499999999999998));
#21665=DIRECTION('ref_axis',(0.499999999999998,-5.6498411616905E-12,-0.86602540378444));
#21666=DIRECTION('',(-9.74874922969709E-27,1.11716191852906E-13,1.));
#21667=DIRECTION('center_axis',(-0.866025403784441,-1.99589445949051E-13,
0.499999999999995));
#21668=DIRECTION('ref_axis',(0.499999999999995,-1.38913863763611E-11,0.866025403784441));
#21669=DIRECTION('',(9.74874922969709E-27,-1.11716191852906E-13,-1.));
#21670=DIRECTION('center_axis',(9.74874922969709E-27,-1.11716191852906E-13,
-1.));
#21671=DIRECTION('ref_axis',(8.73144149574993E-14,-1.,1.11716191852906E-13));
#21672=DIRECTION('',(-9.74874922969709E-27,1.11716191852906E-13,1.));
#21673=DIRECTION('center_axis',(-9.74874922969709E-27,1.11716191852906E-13,
1.));
#21674=DIRECTION('ref_axis',(8.38449680055457E-14,-1.,1.11716191852906E-13));
#21675=DIRECTION('',(9.74874922969709E-27,-1.11716191852906E-13,-1.));
#21676=DIRECTION('center_axis',(9.74874922969709E-27,-1.11716191852906E-13,
-1.));
#21677=DIRECTION('ref_axis',(8.73144149574993E-14,-1.,1.11716191852906E-13));
#21678=DIRECTION('',(-9.74874922969709E-27,1.11716191852906E-13,1.));
#21679=DIRECTION('',(9.74874922969709E-27,-1.11716191852906E-13,-1.));
#21680=DIRECTION('center_axis',(-1.00515054169548E-26,1.1518563880486E-13,
1.));
#21681=DIRECTION('ref_axis',(0.923879532511253,0.382683432365171,-4.40796356170093E-14));
#21682=DIRECTION('center_axis',(-1.00515054169548E-26,1.1518563880486E-13,
1.));
#21683=DIRECTION('ref_axis',(-8.72635297355373E-14,1.,-1.1518563880486E-13));
#21684=DIRECTION('center_axis',(-1.00515054169548E-26,1.1518563880486E-13,
1.));
#21685=DIRECTION('ref_axis',(-8.72635297355373E-14,1.,-1.1518563880486E-13));
#21686=DIRECTION('',(-1.00515054169548E-26,1.1518563880486E-13,1.));
#21687=DIRECTION('center_axis',(1.00515054169548E-26,-1.1518563880486E-13,
-1.));
#21688=DIRECTION('ref_axis',(-8.90398865749375E-14,1.,-1.1518563880486E-13));
#21689=DIRECTION('',(-1.00515054169548E-26,1.1518563880486E-13,1.));
#21690=DIRECTION('center_axis',(-1.00515054169548E-26,1.1518563880486E-13,
1.));
#21691=DIRECTION('ref_axis',(-8.72635297355372E-14,1.,-1.1518563880486E-13));
#21692=DIRECTION('center_axis',(1.00515054169548E-26,-1.1518563880486E-13,
-1.));
#21693=DIRECTION('ref_axis',(-8.72635297355372E-14,1.,-1.1518563880486E-13));
#21694=DIRECTION('',(-1.00515054169548E-26,1.1518563880486E-13,1.));
#21695=DIRECTION('center_axis',(1.00515054169548E-26,-1.1518563880486E-13,
-1.));
#21696=DIRECTION('ref_axis',(-8.72635297355372E-14,1.,-1.1518563880486E-13));
#21697=DIRECTION('center_axis',(-1.00515054169548E-26,1.1518563880486E-13,
1.));
#21698=DIRECTION('ref_axis',(-8.63506796930677E-14,1.,-1.1518563880486E-13));
#21699=DIRECTION('center_axis',(1.00515054169548E-26,-1.1518563880486E-13,
-1.));
#21700=DIRECTION('ref_axis',(-8.63506796930677E-14,1.,-1.1518563880486E-13));
#21701=DIRECTION('',(-1.00515054169548E-26,1.1518563880486E-13,1.));
#21702=DIRECTION('center_axis',(1.00515054169548E-26,-1.1518563880486E-13,
-1.));
#21703=DIRECTION('ref_axis',(-8.63506796930677E-14,1.,-1.1518563880486E-13));
#21704=DIRECTION('center_axis',(-1.00515054169548E-26,1.1518563880486E-13,
1.));
#21705=DIRECTION('ref_axis',(-8.72635297355373E-14,1.,-1.1518563880486E-13));
#21706=DIRECTION('center_axis',(1.00515054169548E-26,-1.1518563880486E-13,
-1.));
#21707=DIRECTION('ref_axis',(-8.72635297355373E-14,1.,-1.1518563880486E-13));
#21708=DIRECTION('',(-1.00515054169548E-26,1.1518563880486E-13,1.));
#21709=DIRECTION('center_axis',(1.00515054169548E-26,-1.1518563880486E-13,
-1.));
#21710=DIRECTION('ref_axis',(-8.72635297355373E-14,1.,-1.1518563880486E-13));
#21711=DIRECTION('center_axis',(-1.00515054169548E-26,1.1518563880486E-13,
1.));
#21712=DIRECTION('ref_axis',(-8.63506796930677E-14,1.,-1.1518563880486E-13));
#21713=DIRECTION('center_axis',(1.00515054169548E-26,-1.1518563880486E-13,
-1.));
#21714=DIRECTION('ref_axis',(-8.63506796930677E-14,1.,-1.1518563880486E-13));
#21715=DIRECTION('',(-1.00515054169548E-26,1.1518563880486E-13,1.));
#21716=DIRECTION('center_axis',(1.00515054169548E-26,-1.1518563880486E-13,
-1.));
#21717=DIRECTION('ref_axis',(-8.63506796930677E-14,1.,-1.1518563880486E-13));
#21718=DIRECTION('center_axis',(1.00515054169548E-26,-1.1518563880486E-13,
-1.));
#21719=DIRECTION('ref_axis',(8.72635297355373E-14,-1.,1.1518563880486E-13));
#21720=DIRECTION('center_axis',(1.00515054169548E-26,-1.1518563880486E-13,
-1.));
#21721=DIRECTION('ref_axis',(8.72635297355373E-14,-1.,1.1518563880486E-13));
#21722=DIRECTION('',(-1.00515054169548E-26,1.1518563880486E-13,1.));
#21723=DIRECTION('center_axis',(1.00515054169548E-26,-1.1518563880486E-13,
-1.));
#21724=DIRECTION('ref_axis',(8.72635297355373E-14,-1.,1.1518563880486E-13));
#21725=DIRECTION('center_axis',(9.74874922969709E-27,-1.11716191852906E-13,
-1.));
#21726=DIRECTION('ref_axis',(8.73144149574993E-14,-1.,1.11716191852906E-13));
#21727=DIRECTION('center_axis',(9.74874922969709E-27,-1.11716191852906E-13,
-1.));
#21728=DIRECTION('ref_axis',(8.73144149574993E-14,-1.,1.11716191852906E-13));
#21729=DIRECTION('',(-9.74874922969709E-27,1.11716191852906E-13,1.));
#21730=DIRECTION('',(9.74874922969709E-27,-1.11716191852906E-13,-1.));
#21731=DIRECTION('center_axis',(-8.72635297355373E-14,1.,-1.11716191852906E-13));
#21732=DIRECTION('ref_axis',(-6.05512374515382E-29,-1.11716191852906E-13,
-1.));
#21733=DIRECTION('center_axis',(-8.72635297355373E-14,1.,-1.11716191852906E-13));
#21734=DIRECTION('ref_axis',(-6.05512374515382E-29,-1.11716191852906E-13,
-1.));
#21735=DIRECTION('',(8.87753855036761E-14,-1.,1.14312768470149E-13));
#21736=DIRECTION('',(-8.57516739673986E-14,1.,-1.14312768470149E-13));
#21737=DIRECTION('center_axis',(9.74874922969709E-27,-1.11716191852906E-13,
-1.));
#21738=DIRECTION('ref_axis',(8.73144149574993E-14,-1.,1.11716191852906E-13));
#21739=DIRECTION('center_axis',(0.86602540378444,1.19740931593546E-14,-0.499999999999999));
#21740=DIRECTION('ref_axis',(0.499999999999998,4.90026582553221E-12,0.86602540378444));
#21741=DIRECTION('',(-9.74874922969709E-27,1.11716191852906E-13,1.));
#21742=DIRECTION('center_axis',(0.866025403784415,4.89441057888314E-13,
0.500000000000041));
#21743=DIRECTION('ref_axis',(0.500000000000041,-6.4989672014377E-12,-0.866025403784415));
#21744=DIRECTION('',(9.74874922969709E-27,-1.11716191852906E-13,-1.));
#21745=DIRECTION('center_axis',(-1.81408990941771E-16,-1.1518563880486E-13,
-1.));
#21746=DIRECTION('ref_axis',(-1.,-8.72577246478268E-14,1.81408990951822E-16));
#21747=DIRECTION('center_axis',(-1.00515054169548E-26,1.1518563880486E-13,
1.));
#21748=DIRECTION('ref_axis',(8.19344592173366E-14,-1.,1.1518563880486E-13));
#21749=DIRECTION('center_axis',(-1.00515054169548E-26,1.1518563880486E-13,
1.));
#21750=DIRECTION('ref_axis',(8.01581023779363E-14,-1.,1.1518563880486E-13));
#21751=DIRECTION('center_axis',(-1.00515054169548E-26,1.1518563880486E-13,
1.));
#21752=DIRECTION('ref_axis',(8.72635297355373E-14,-1.,1.1518563880486E-13));
#21753=DIRECTION('center_axis',(-1.00515054169548E-26,1.1518563880486E-13,
1.));
#21754=DIRECTION('ref_axis',(8.63753513158372E-14,-1.,1.1518563880486E-13));
#21755=DIRECTION('center_axis',(-1.00515054169548E-26,1.1518563880486E-13,
1.));
#21756=DIRECTION('ref_axis',(8.72635297355373E-14,-1.,1.1518563880486E-13));
#21757=DIRECTION('',(-0.970295726275999,-5.66810422692838E-14,0.241921895599659));
#21758=DIRECTION('center_axis',(-1.00515054169548E-26,1.1518563880486E-13,
1.));
#21759=DIRECTION('ref_axis',(8.72635297355373E-14,-1.,1.1518563880486E-13));
#21760=DIRECTION('center_axis',(-1.00515054169548E-26,1.1518563880486E-13,
1.));
#21761=DIRECTION('ref_axis',(8.01581023779363E-14,-1.,1.1518563880486E-13));
#21762=DIRECTION('center_axis',(-1.00515054169548E-26,1.1518563880486E-13,
1.));
#21763=DIRECTION('ref_axis',(8.45989944764369E-14,-1.,1.1518563880486E-13));
#21764=DIRECTION('center_axis',(-1.00515054169548E-26,1.1518563880486E-13,
1.));
#21765=DIRECTION('ref_axis',(9.79216707719388E-14,-1.,1.1518563880486E-13));
#21766=DIRECTION('center_axis',(0.868162779192246,0.38268343239671,0.315985410097158));
#21767=DIRECTION('ref_axis',(0.403349423721025,-0.915046032931632,1.06907841467309E-13));
#21768=DIRECTION('center_axis',(-0.868162779195909,-0.359604797490725,-0.342020143325639));
#21769=DIRECTION('ref_axis',(0.0151045167327983,0.669702936743006,-0.742475474404415));
#21770=DIRECTION('center_axis',(-0.868162779192246,-0.38268343239671,-0.315985410097158));
#21771=DIRECTION('ref_axis',(0.403349423721026,-0.915046032931631,1.02974997442446E-13));
#21772=DIRECTION('',(-0.868162779192246,-0.38268343239671,-0.315985410097158));
#21773=DIRECTION('center_axis',(0.868162779192246,0.38268343239671,0.315985410097158));
#21774=DIRECTION('ref_axis',(0.403349423721025,-0.915046032931632,1.06907841467309E-13));
#21775=DIRECTION('center_axis',(0.868162779192246,0.38268343239671,0.315985410097158));
#21776=DIRECTION('ref_axis',(0.403349423721025,-0.915046032931632,1.06907841467309E-13));
#21777=DIRECTION('center_axis',(-0.868162779192246,-0.38268343239671,-0.315985410097158));
#21778=DIRECTION('ref_axis',(0.403349423721026,-0.915046032931631,1.02974997442446E-13));
#21779=DIRECTION('center_axis',(9.74874922969709E-27,-1.11716191852906E-13,
-1.));
#21780=DIRECTION('ref_axis',(8.73144149574993E-14,-1.,1.11716191852906E-13));
#21781=DIRECTION('center_axis',(9.74874922969709E-27,-1.11716191852906E-13,
-1.));
#21782=DIRECTION('ref_axis',(8.73144149574993E-14,-1.,1.11716191852906E-13));
#21783=DIRECTION('',(-9.74874922969709E-27,1.11716191852906E-13,1.));
#21784=DIRECTION('center_axis',(-9.74874922969709E-27,1.11716191852906E-13,
1.));
#21785=DIRECTION('ref_axis',(9.07838619094529E-14,-1.,1.11716191852906E-13));
#21786=DIRECTION('',(9.74874922969709E-27,-1.11716191852906E-13,-1.));
#21787=DIRECTION('center_axis',(-1.00515054169548E-26,1.1518563880486E-13,
1.));
#21788=DIRECTION('ref_axis',(-8.72635297355373E-14,1.,-1.1518563880486E-13));
#21789=DIRECTION('center_axis',(-1.00515054169548E-26,1.1518563880486E-13,
1.));
#21790=DIRECTION('ref_axis',(-8.72635297355373E-14,1.,-1.1518563880486E-13));
#21791=DIRECTION('',(-1.00515054169548E-26,1.1518563880486E-13,1.));
#21792=DIRECTION('center_axis',(-1.00515054169548E-26,1.1518563880486E-13,
1.));
#21793=DIRECTION('ref_axis',(-8.72635297355373E-14,1.,-1.1518563880486E-13));
#21794=DIRECTION('',(1.00515054169548E-26,-1.1518563880486E-13,-1.));
#21795=DIRECTION('',(1.00515054169548E-26,-1.1518563880486E-13,-1.));
#21796=DIRECTION('center_axis',(-1.00515054169548E-26,1.1518563880486E-13,
1.));
#21797=DIRECTION('ref_axis',(-8.72635297355373E-14,1.,-1.1518563880486E-13));
#21798=DIRECTION('',(1.00515054169548E-26,-1.1518563880486E-13,-1.));
#21799=DIRECTION('center_axis',(0.868162779192246,0.382683432396709,0.315985410097158));
#21800=DIRECTION('ref_axis',(0.403349423721025,-0.915046032931632,1.06983183810373E-13));
#21801=DIRECTION('',(-0.328672675627568,-0.917633305084373,-0.223435426232604));
#21802=DIRECTION('center_axis',(0.868162779192246,0.382683432396709,0.315985410097158));
#21803=DIRECTION('ref_axis',(0.403349423721025,-0.915046032931632,1.06502267550115E-13));
#21804=DIRECTION('center_axis',(-1.00515054169548E-26,1.1518563880486E-13,
1.));
#21805=DIRECTION('ref_axis',(-8.72635297355372E-14,1.,-1.1518563880486E-13));
#21806=DIRECTION('center_axis',(-1.00515054169548E-26,1.1518563880486E-13,
1.));
#21807=DIRECTION('ref_axis',(-8.72635297355372E-14,1.,-1.1518563880486E-13));
#21808=DIRECTION('',(-1.00515054169548E-26,1.1518563880486E-13,1.));
#21809=DIRECTION('center_axis',(1.00515054169548E-26,-1.1518563880486E-13,
-1.));
#21810=DIRECTION('ref_axis',(-8.72635297355372E-14,1.,-1.1518563880486E-13));
#21811=DIRECTION('center_axis',(-1.00515054169548E-26,1.1518563880486E-13,
1.));
#21812=DIRECTION('ref_axis',(-8.67361737988404E-14,1.,-1.1518563880486E-13));
#21813=DIRECTION('center_axis',(-1.00515054169548E-26,1.1518563880486E-13,
1.));
#21814=DIRECTION('ref_axis',(-8.67361737988404E-14,1.,-1.1518563880486E-13));
#21815=DIRECTION('',(-1.00515054169548E-26,1.1518563880486E-13,1.));
#21816=DIRECTION('center_axis',(1.00515054169548E-26,-1.1518563880486E-13,
-1.));
#21817=DIRECTION('ref_axis',(-8.67361737988404E-14,1.,-1.1518563880486E-13));
#21818=DIRECTION('center_axis',(-1.00515054169548E-26,1.1518563880486E-13,
1.));
#21819=DIRECTION('ref_axis',(-8.72635297355372E-14,1.,-1.1518563880486E-13));
#21820=DIRECTION('center_axis',(-1.00515054169548E-26,1.1518563880486E-13,
1.));
#21821=DIRECTION('ref_axis',(-8.72635297355373E-14,1.,-1.1518563880486E-13));
#21822=DIRECTION('',(-1.00515054169548E-26,1.1518563880486E-13,1.));
#21823=DIRECTION('center_axis',(1.00515054169548E-26,-1.1518563880486E-13,
-1.));
#21824=DIRECTION('ref_axis',(-8.72635297355373E-14,1.,-1.1518563880486E-13));
#21825=DIRECTION('center_axis',(-1.00515054169548E-26,1.1518563880486E-13,
1.));
#21826=DIRECTION('ref_axis',(-8.67361737988404E-14,1.,-1.1518563880486E-13));
#21827=DIRECTION('center_axis',(-1.00515054169548E-26,1.1518563880486E-13,
1.));
#21828=DIRECTION('ref_axis',(-8.67361737988404E-14,1.,-1.1518563880486E-13));
#21829=DIRECTION('',(-1.00515054169548E-26,1.1518563880486E-13,1.));
#21830=DIRECTION('center_axis',(1.00515054169548E-26,-1.1518563880486E-13,
-1.));
#21831=DIRECTION('ref_axis',(-8.67361737988404E-14,1.,-1.1518563880486E-13));
#21832=DIRECTION('center_axis',(1.00515054169548E-26,-1.1518563880486E-13,
-1.));
#21833=DIRECTION('ref_axis',(8.72635297355373E-14,-1.,1.1518563880486E-13));
#21834=DIRECTION('center_axis',(1.00515054169548E-26,-1.1518563880486E-13,
-1.));
#21835=DIRECTION('ref_axis',(8.72635297355373E-14,-1.,1.1518563880486E-13));
#21836=DIRECTION('',(-1.00515054169548E-26,1.1518563880486E-13,1.));
#21837=DIRECTION('center_axis',(1.00515054169548E-26,-1.1518563880486E-13,
-1.));
#21838=DIRECTION('ref_axis',(8.72635297355373E-14,-1.,1.1518563880486E-13));
#21839=DIRECTION('',(-1.00515054169548E-26,1.1518563880486E-13,1.));
#21840=DIRECTION('center_axis',(-1.00515054169548E-26,1.1518563880486E-13,
1.));
#21841=DIRECTION('ref_axis',(8.72635297355373E-14,-1.,1.1518563880486E-13));
#21842=DIRECTION('',(-1.00515054169548E-26,1.1518563880486E-13,1.));
#21843=DIRECTION('center_axis',(1.00515054169548E-26,-1.1518563880486E-13,
-1.));
#21844=DIRECTION('ref_axis',(8.72635297355373E-14,-1.,1.1518563880486E-13));
#21845=DIRECTION('center_axis',(-1.00515054169548E-26,1.1518563880486E-13,
1.));
#21846=DIRECTION('ref_axis',(8.72635297355373E-14,-1.,1.1518563880486E-13));
#21847=DIRECTION('',(1.00515054169548E-26,-1.1518563880486E-13,-1.));
#21848=DIRECTION('center_axis',(1.00515054169548E-26,-1.1518563880486E-13,
-1.));
#21849=DIRECTION('ref_axis',(8.72635297355373E-14,-1.,1.1518563880486E-13));
#21850=DIRECTION('center_axis',(-8.72635297355373E-14,1.,-1.11716191852906E-13));
#21851=DIRECTION('ref_axis',(6.05512374515283E-29,-1.11716191852906E-13,
-1.));
#21852=DIRECTION('center_axis',(-8.72635297355373E-14,1.,-1.11716191852906E-13));
#21853=DIRECTION('ref_axis',(6.05512374515455E-29,-1.11716191852906E-13,
-1.));
#21854=DIRECTION('',(-8.72635297355373E-14,1.,-1.11716191852906E-13));
#21855=DIRECTION('center_axis',(8.72635297355373E-14,-1.,1.11716191852906E-13));
#21856=DIRECTION('ref_axis',(6.05512374515283E-29,-1.11716191852906E-13,
-1.));
#21857=DIRECTION('center_axis',(-8.72635297355373E-14,1.,-1.11716191852906E-13));
#21858=DIRECTION('ref_axis',(6.05512374515455E-29,-1.11716191852906E-13,
-1.));
#21859=DIRECTION('center_axis',(-8.72635297355373E-14,1.,-1.11716191852906E-13));
#21860=DIRECTION('ref_axis',(6.05512374515455E-29,-1.11716191852906E-13,
-1.));
#21861=DIRECTION('',(-8.72635297355373E-14,1.,-1.11716191852906E-13));
#21862=DIRECTION('center_axis',(-8.72635297355373E-14,1.,-1.11716191852906E-13));
#21863=DIRECTION('ref_axis',(6.05512374515455E-29,-1.11716191852906E-13,
-1.));
#21864=DIRECTION('center_axis',(1.00515054169548E-26,-1.1518563880486E-13,
-1.));
#21865=DIRECTION('ref_axis',(8.72635297355373E-14,-1.,1.1518563880486E-13));
#21866=DIRECTION('',(6.16180380206417E-14,-0.707106781186466,0.707106781186629));
#21867=DIRECTION('center_axis',(1.00515054169548E-26,-1.1518563880486E-13,
-1.));
#21868=DIRECTION('ref_axis',(8.72635297355373E-14,-1.,1.1518563880486E-13));
#21869=DIRECTION('center_axis',(8.72635297355373E-14,-1.,1.1518563880486E-13));
#21870=DIRECTION('ref_axis',(-1.73003535575891E-29,1.1518563880486E-13,
1.));
#21871=DIRECTION('center_axis',(8.72635297355373E-14,-1.,1.1518563880486E-13));
#21872=DIRECTION('ref_axis',(-1.73003535575891E-29,1.1518563880486E-13,
1.));
#21873=DIRECTION('',(-8.72635297355373E-14,1.,-1.1518563880486E-13));
#21874=DIRECTION('center_axis',(8.72635297355373E-14,-1.,1.1518563880486E-13));
#21875=DIRECTION('ref_axis',(-1.73003535575891E-29,1.1518563880486E-13,
1.));
#21876=DIRECTION('center_axis',(8.72635297355373E-14,-1.,1.1518563880486E-13));
#21877=DIRECTION('ref_axis',(-1.73003535575891E-29,1.1518563880486E-13,
1.));
#21878=DIRECTION('center_axis',(8.72635297355373E-14,-1.,1.1518563880486E-13));
#21879=DIRECTION('ref_axis',(-1.73003535575891E-29,1.1518563880486E-13,
1.));
#21880=DIRECTION('',(-8.72635297355373E-14,1.,-1.1518563880486E-13));
#21881=DIRECTION('center_axis',(8.72635297355373E-14,-1.,1.1518563880486E-13));
#21882=DIRECTION('ref_axis',(-1.73003535575891E-29,1.1518563880486E-13,
1.));
#21883=DIRECTION('center_axis',(-1.00515054169548E-26,1.1518563880486E-13,
1.));
#21884=DIRECTION('ref_axis',(-8.78926561161581E-14,1.,-1.1518563880486E-13));
#21885=DIRECTION('center_axis',(-1.00515054169548E-26,1.1518563880486E-13,
1.));
#21886=DIRECTION('ref_axis',(-8.78926561161581E-14,1.,-1.1518563880486E-13));
#21887=DIRECTION('',(1.00515054169548E-26,-1.1518563880486E-13,-1.));
#21888=DIRECTION('center_axis',(-1.00515054169548E-26,1.1518563880486E-13,
1.));
#21889=DIRECTION('ref_axis',(-8.78926561161581E-14,1.,-1.1518563880486E-13));
#21890=DIRECTION('center_axis',(-1.00515054169548E-26,1.1518563880486E-13,
1.));
#21891=DIRECTION('ref_axis',(-8.78926561160683E-14,1.,-1.1518563880486E-13));
#21892=DIRECTION('center_axis',(-1.00515054169548E-26,1.1518563880486E-13,
1.));
#21893=DIRECTION('ref_axis',(-8.78926561160683E-14,1.,-1.1518563880486E-13));
#21894=DIRECTION('',(1.00515054169548E-26,-1.1518563880486E-13,-1.));
#21895=DIRECTION('center_axis',(-1.00515054169548E-26,1.1518563880486E-13,
1.));
#21896=DIRECTION('ref_axis',(-8.78926561160683E-14,1.,-1.1518563880486E-13));
#21897=DIRECTION('center_axis',(-1.00515054169548E-26,1.1518563880486E-13,
1.));
#21898=DIRECTION('ref_axis',(-8.78926561160967E-14,1.,-1.1518563880486E-13));
#21899=DIRECTION('center_axis',(-1.00515054169548E-26,1.1518563880486E-13,
1.));
#21900=DIRECTION('ref_axis',(-8.78926561160967E-14,1.,-1.1518563880486E-13));
#21901=DIRECTION('',(1.00515054169548E-26,-1.1518563880486E-13,-1.));
#21902=DIRECTION('center_axis',(-1.00515054169548E-26,1.1518563880486E-13,
1.));
#21903=DIRECTION('ref_axis',(-8.78926561160967E-14,1.,-1.1518563880486E-13));
#21904=DIRECTION('center_axis',(-1.00515054169548E-26,1.1518563880486E-13,
1.));
#21905=DIRECTION('ref_axis',(-8.78926561161797E-14,1.,-1.1518563880486E-13));
#21906=DIRECTION('center_axis',(-1.00515054169548E-26,1.1518563880486E-13,
1.));
#21907=DIRECTION('ref_axis',(-8.78926561161797E-14,1.,-1.1518563880486E-13));
#21908=DIRECTION('',(1.00515054169548E-26,-1.1518563880486E-13,-1.));
#21909=DIRECTION('center_axis',(-1.00515054169548E-26,1.1518563880486E-13,
1.));
#21910=DIRECTION('ref_axis',(-8.78926561161797E-14,1.,-1.1518563880486E-13));
#21911=DIRECTION('center_axis',(1.00515054169548E-26,-1.1518563880486E-13,
-1.));
#21912=DIRECTION('ref_axis',(8.72635297355373E-14,-1.,1.1518563880486E-13));
#21913=DIRECTION('center_axis',(1.00515054169548E-26,-1.1518563880486E-13,
-1.));
#21914=DIRECTION('ref_axis',(8.72635297355373E-14,-1.,1.1518563880486E-13));
#21915=DIRECTION('',(-1.00515054169548E-26,1.1518563880486E-13,1.));
#21916=DIRECTION('center_axis',(-1.00515054169548E-26,1.1518563880486E-13,
1.));
#21917=DIRECTION('ref_axis',(8.72635297355373E-14,-1.,1.1518563880486E-13));
#21918=DIRECTION('',(1.00515054169548E-26,-1.1518563880486E-13,-1.));
#21919=DIRECTION('center_axis',(1.00515054169548E-26,-1.1518563880486E-13,
-1.));
#21920=DIRECTION('ref_axis',(8.72635297355373E-14,-1.,1.1518563880486E-13));
#21921=DIRECTION('',(1.00515054169548E-26,-1.1518563880486E-13,-1.));
#21922=DIRECTION('center_axis',(-1.00515054169548E-26,1.1518563880486E-13,
1.));
#21923=DIRECTION('ref_axis',(8.72635297355373E-14,-1.,1.1518563880486E-13));
#21924=DIRECTION('center_axis',(-1.00515054169548E-26,1.1518563880486E-13,
1.));
#21925=DIRECTION('ref_axis',(8.72635297355373E-14,-1.,1.1518563880486E-13));
#21926=DIRECTION('center_axis',(1.05148106564929E-14,1.13041557302278E-13,
1.));
#21927=DIRECTION('ref_axis',(1.,8.72630157433963E-14,-1.05148106565028E-14));
#21928=DIRECTION('center_axis',(1.05148106564929E-14,1.13041557302278E-13,
1.));
#21929=DIRECTION('ref_axis',(1.,8.72632848014737E-14,-1.05148106565028E-14));
#21930=DIRECTION('',(-0.0174340297464476,-0.000800685489193615,-0.999847695156391));
#21931=DIRECTION('center_axis',(1.05148106564929E-14,1.13041557302278E-13,
1.));
#21932=DIRECTION('ref_axis',(1.,8.72630157433963E-14,-1.05148106565028E-14));
#21933=DIRECTION('',(-0.0174340297464478,0.000800685488960295,-0.999847695156391));
#21934=DIRECTION('center_axis',(5.13992141019283E-16,1.1518563880486E-13,
1.));
#21935=DIRECTION('ref_axis',(1.,8.72635297355373E-14,-5.13992141029335E-16));
#21936=DIRECTION('center_axis',(-1.00515054169548E-26,1.1518563880486E-13,
1.));
#21937=DIRECTION('ref_axis',(8.72635297355373E-14,-1.,1.1518563880486E-13));
#21938=DIRECTION('center_axis',(-1.00515054169548E-26,1.1518563880486E-13,
1.));
#21939=DIRECTION('ref_axis',(8.72635297355373E-14,-1.,1.1518563880486E-13));
#21940=DIRECTION('',(-0.707106781186547,1.96573170623249E-14,0.707106781186548));
#21941=DIRECTION('center_axis',(-1.00515054169548E-26,1.1518563880486E-13,
1.));
#21942=DIRECTION('ref_axis',(-8.72635297355373E-14,1.,-1.1518563880486E-13));
#21943=DIRECTION('center_axis',(-1.00515054169548E-26,1.1518563880486E-13,
1.));
#21944=DIRECTION('ref_axis',(-8.72635297355373E-14,1.,-1.1518563880486E-13));
#21945=DIRECTION('center_axis',(-1.00515054169548E-26,1.1518563880486E-13,
1.));
#21946=DIRECTION('ref_axis',(-8.72635297355373E-14,1.,-1.1518563880486E-13));
#21947=DIRECTION('',(-1.00515054169548E-26,1.1518563880486E-13,1.));
#21948=DIRECTION('center_axis',(1.04893682793573E-14,1.13034729017238E-13,
1.));
#21949=DIRECTION('ref_axis',(1.,8.72628520516316E-14,-1.04893682793672E-14));
#21950=DIRECTION('center_axis',(1.50814224405608E-9,1.30680347155798E-11,
1.));
#21951=DIRECTION('ref_axis',(0.999950224327263,0.0099774178952433,-1.50819757644053E-9));
#21952=DIRECTION('center_axis',(2.2737638208062E-9,5.96781185745539E-11,
1.));
#21953=DIRECTION('ref_axis',(0.999629828344744,0.0272067323186488,-2.27454576389334E-9));
#21954=DIRECTION('',(-0.0174340340546636,-0.000800591677107547,-0.999847695156391));
#21955=DIRECTION('center_axis',(1.04893682793573E-14,1.13034729017238E-13,
1.));
#21956=DIRECTION('ref_axis',(1.,8.72628520516316E-14,-1.04893682793672E-14));
#21957=DIRECTION('',(-0.0174340340546638,0.00080059167687424,-0.999847695156391));
#21958=DIRECTION('center_axis',(2.01391717416503E-9,-5.2395782353962E-11,
1.));
#21959=DIRECTION('ref_axis',(0.999686135569083,-0.0250525517852406,-2.01459769357307E-9));
#21960=DIRECTION('center_axis',(1.34057310888677E-9,-1.13635839552688E-11,
1.));
#21961=DIRECTION('ref_axis',(0.999970713945725,-0.00765318566846746,-1.34062078067377E-9));
#21962=DIRECTION('center_axis',(1.,8.72635297355373E-14,0.));
#21963=DIRECTION('ref_axis',(8.72635297355373E-14,-1.,1.13545536609336E-13));
#21964=DIRECTION('center_axis',(-1.,-8.55363631858458E-14,2.53597807885338E-16));
#21965=DIRECTION('ref_axis',(8.57899609937212E-14,-1.,1.21115239049959E-13));
#21966=DIRECTION('',(-1.,-8.72635297355373E-14,0.));
#21967=DIRECTION('center_axis',(-1.,-8.72635297355373E-14,0.));
#21968=DIRECTION('ref_axis',(8.72635297355373E-14,-1.,1.19853621976522E-13));
#21969=DIRECTION('center_axis',(1.,8.72635297355373E-14,0.));
#21970=DIRECTION('ref_axis',(8.72635297355373E-14,-1.,1.13545536609336E-13));
#21971=DIRECTION('center_axis',(-1.,-8.55363631858455E-14,2.53597807885001E-16));
#21972=DIRECTION('ref_axis',(8.57899609937217E-14,-1.,1.2111523904996E-13));
#21973=DIRECTION('',(-1.,-8.72635297355373E-14,0.));
#21974=DIRECTION('center_axis',(-1.,-8.72635297355373E-14,0.));
#21975=DIRECTION('ref_axis',(8.72635297355373E-14,-1.,1.19853621976522E-13));
#21976=DIRECTION('center_axis',(1.00515054169548E-26,-1.1518563880486E-13,
-1.));
#21977=DIRECTION('ref_axis',(8.72635297355373E-14,-1.,1.1518563880486E-13));
#21978=DIRECTION('',(-6.16180380185814E-14,0.707106781162823,-0.707106781210272));
#21979=DIRECTION('center_axis',(-1.00515054169548E-26,1.1518563880486E-13,
1.));
#21980=DIRECTION('ref_axis',(8.72635297355373E-14,-1.,1.1518563880486E-13));
#21981=DIRECTION('center_axis',(1.00515054169548E-26,-1.1518563880486E-13,
-1.));
#21982=DIRECTION('ref_axis',(8.72635297355373E-14,-1.,1.1518563880486E-13));
#21983=DIRECTION('center_axis',(-8.07434927010188E-16,1.13848324707016E-13,
1.));
#21984=DIRECTION('ref_axis',(-8.57535022254239E-14,1.,-1.14655759634016E-13));
#21985=DIRECTION('',(1.00515054169548E-26,-1.1518563880486E-13,-1.));
#21986=DIRECTION('center_axis',(-1.00515054169548E-26,1.1518563880486E-13,
1.));
#21987=DIRECTION('ref_axis',(8.72635297355373E-14,-1.,1.1518563880486E-13));
#21988=DIRECTION('center_axis',(-1.00515054169548E-26,1.1518563880486E-13,
1.));
#21989=DIRECTION('ref_axis',(8.72635297355373E-14,-1.,1.1518563880486E-13));
#21990=DIRECTION('center_axis',(-1.04744440165193E-14,-1.15185638804861E-13,
-1.));
#21991=DIRECTION('ref_axis',(-1.,-8.72677046689168E-14,1.04744440165294E-14));
#21992=DIRECTION('center_axis',(-1.60317441773188E-14,-1.30010586908455E-13,
-1.));
#21993=DIRECTION('ref_axis',(-0.986663993658372,0.162770278669396,-5.1459919581511E-15));
#21994=DIRECTION('',(-1.04744440165193E-14,-1.15185638804861E-13,-1.));
#21995=DIRECTION('center_axis',(-5.8420956475864E-12,5.24858042098029E-13,
1.));
#21996=DIRECTION('ref_axis',(-1.,-8.33007448225695E-14,-5.84228425464237E-12));
#21997=DIRECTION('',(-1.04744440165193E-14,-1.15185638804861E-13,-1.));
#21998=DIRECTION('center_axis',(-1.00515054169548E-26,1.1518563880486E-13,
1.));
#21999=DIRECTION('ref_axis',(-8.72635297355373E-14,1.,-1.1518563880486E-13));
#22000=DIRECTION('',(7.81604095158039E-14,-0.894427190977678,0.447213595544433));
#22001=DIRECTION('center_axis',(7.90669341981024E-5,-6.79899070760606E-6,
-0.999999996851097));
#22002=DIRECTION('ref_axis',(-0.224409606993171,0.974494909014575,-2.4368961537286E-5));
#22003=DIRECTION('center_axis',(4.84900603469004E-5,2.12716297860176E-5,
-0.999999998598116));
#22004=DIRECTION('ref_axis',(-0.215549302917957,0.97649295845136,1.03195980090732E-5));
#22005=DIRECTION('',(-0.476471251976903,-0.412057254805414,-0.776649190305242));
#22006=DIRECTION('',(0.497089462473265,0.150347978283572,0.854574485767088));
#22007=DIRECTION('',(0.49708946264798,-0.150347978462221,0.85457448563403));
#22008=DIRECTION('',(0.472361792915602,-0.100907068159122,0.875609559215229));
#22009=DIRECTION('center_axis',(4.84900605051656E-5,-2.12716300746791E-5,
-0.999999998598116));
#22010=DIRECTION('ref_axis',(0.215549302836865,0.97649295846926,-1.03195982611481E-5));
#22011=DIRECTION('',(-0.47647125197697,0.412057254805155,-0.776649190305339));
#22012=DIRECTION('',(-0.379976420578336,0.59082305053514,-0.711720480779376));
#22013=DIRECTION('center_axis',(1.42705873244029E-5,-3.83465092369397E-5,
-0.999999999162948));
#22014=DIRECTION('ref_axis',(0.857448829753204,0.514569241500769,-7.49563577732842E-6));
#22015=DIRECTION('',(-0.590708354574789,0.380106497268313,-0.711746226242163));
#22016=DIRECTION('',(-0.411902009107452,0.476603463260479,-0.776650419237228));
#22017=DIRECTION('center_axis',(-1.2742627722323E-5,-2.90510924139551E-5,
-0.99999999949683));
#22018=DIRECTION('ref_axis',(0.976471046734733,-0.215648544744935,-6.17798123095627E-6));
#22019=DIRECTION('center_axis',(-2.2112189231786E-5,-7.9504155517196E-6,
-0.999999999723921));
#22020=DIRECTION('ref_axis',(-0.574484253249288,0.818515633772637,6.19556509616842E-6));
#22021=DIRECTION('center_axis',(-8.72635297355373E-14,1.,-1.1518563880486E-13));
#22022=DIRECTION('ref_axis',(1.00515054169548E-26,-1.1518563880486E-13,
-1.));
#22023=DIRECTION('',(-0.866025403789923,-1.79796141740169E-14,0.4999999999905));
#22024=DIRECTION('',(-1.00515054169548E-26,1.1518563880486E-13,1.));
#22025=DIRECTION('',(0.866025403789923,1.33165252976688E-13,0.4999999999905));
#22026=DIRECTION('',(0.866025403789923,1.79796141740169E-14,-0.4999999999905));
#22027=DIRECTION('',(1.00515054169548E-26,-1.1518563880486E-13,-1.));
#22028=DIRECTION('',(-0.866025403789923,-1.33165252976688E-13,-0.4999999999905));
#22029=DIRECTION('center_axis',(-8.72635297355373E-14,1.,-1.1518563880486E-13));
#22030=DIRECTION('ref_axis',(1.00515054169548E-26,-1.1518563880486E-13,
-1.));
#22031=DIRECTION('',(-0.866025403789923,-1.79796141740169E-14,0.4999999999905));
#22032=DIRECTION('',(-1.00515054169548E-26,1.1518563880486E-13,1.));
#22033=DIRECTION('',(0.866025403789923,1.33165252976688E-13,0.4999999999905));
#22034=DIRECTION('',(0.866025403789923,1.79796141740169E-14,-0.4999999999905));
#22035=DIRECTION('',(1.00515054169548E-26,-1.1518563880486E-13,-1.));
#22036=DIRECTION('',(-0.866025403789923,-1.33165252976688E-13,-0.4999999999905));
#22037=DIRECTION('center_axis',(-8.72635297355373E-14,1.,-1.1518563880486E-13));
#22038=DIRECTION('ref_axis',(1.00515054169548E-26,-1.1518563880486E-13,
-1.));
#22039=DIRECTION('',(-0.866025403789923,-1.79796141740169E-14,0.4999999999905));
#22040=DIRECTION('',(-1.00515054169548E-26,1.1518563880486E-13,1.));
#22041=DIRECTION('',(0.866025403789923,1.33165252976688E-13,0.4999999999905));
#22042=DIRECTION('',(0.866025403789923,1.79796141740169E-14,-0.4999999999905));
#22043=DIRECTION('',(1.00515054169548E-26,-1.1518563880486E-13,-1.));
#22044=DIRECTION('',(-0.866025403789923,-1.33165252976688E-13,-0.4999999999905));
#22045=DIRECTION('center_axis',(-8.72635297355373E-14,1.,-1.1518563880486E-13));
#22046=DIRECTION('ref_axis',(1.00515054169548E-26,-1.1518563880486E-13,
-1.));
#22047=DIRECTION('',(-0.866025403789923,-1.79796141740169E-14,0.4999999999905));
#22048=DIRECTION('',(-1.00515054169548E-26,1.1518563880486E-13,1.));
#22049=DIRECTION('',(0.866025403789923,1.33165252976688E-13,0.4999999999905));
#22050=DIRECTION('',(0.866025403789923,1.79796141740169E-14,-0.4999999999905));
#22051=DIRECTION('',(1.00515054169548E-26,-1.1518563880486E-13,-1.));
#22052=DIRECTION('',(-0.866025403789923,-1.33165252976688E-13,-0.4999999999905));
#22053=DIRECTION('center_axis',(-1.04744440165193E-14,-1.15185638804861E-13,
-1.));
#22054=DIRECTION('ref_axis',(-1.,-8.72635297355361E-14,1.04744440165294E-14));
#22055=DIRECTION('center_axis',(1.27156302261967E-12,-7.67259042032779E-13,
-1.));
#22056=DIRECTION('ref_axis',(0.707106781186604,-0.707106781186491,1.44328993201271E-12));
#22057=DIRECTION('',(-0.707106781186489,-0.707106781186606,8.14485462942204E-14));
#22058=DIRECTION('center_axis',(-5.76880098885803E-15,-2.11163646621927E-13,
-1.));
#22059=DIRECTION('ref_axis',(0.162770278669586,-0.98666399365834,2.08721928629528E-13));
#22060=DIRECTION('center_axis',(2.90371050762764E-14,-3.54407276356552E-13,
-1.));
#22061=DIRECTION('ref_axis',(9.61069664125861E-14,-1.,3.54281754041935E-13));
#22062=DIRECTION('center_axis',(-3.74976319533066E-13,-9.52526981242744E-13,
-1.));
#22063=DIRECTION('ref_axis',(-0.70710678118649,-0.707106781186605,9.37028232783635E-13));
#22064=DIRECTION('',(-0.707106781186605,0.70710678118649,-8.14485462942213E-14));
#22065=DIRECTION('center_axis',(1.28789942775155E-13,-4.80738143802119E-14,
-1.));
#22066=DIRECTION('ref_axis',(-0.986663993658341,-0.162770278669579,-1.19904086659517E-13));
#22067=DIRECTION('center_axis',(-1.28789942775156E-13,-4.80738143802258E-14,
-1.));
#22068=DIRECTION('ref_axis',(-0.707106781186605,0.70710678118649,5.77315972805082E-14));
#22069=DIRECTION('',(0.70710678118649,0.707106781186605,-8.14485462942203E-14));
#22070=DIRECTION('center_axis',(-1.89685730694799E-13,1.62833466326211E-13,
-1.));
#22071=DIRECTION('ref_axis',(-0.162770278669582,0.986663993658341,1.90958360235528E-13));
#22072=DIRECTION('center_axis',(-1.08828435367454E-13,8.83049349377018E-13,
-1.));
#22073=DIRECTION('ref_axis',(-9.16685483161296E-14,1.,8.83131389125757E-13));
#22074=DIRECTION('center_axis',(-4.23050133913277E-14,-8.23737038467554E-14,
-1.));
#22075=DIRECTION('ref_axis',(0.707106781186495,0.7071067811866,-8.88178419700125E-14));
#22076=DIRECTION('',(0.707106781186606,-0.707106781186489,8.14485462942212E-14));
#22077=DIRECTION('center_axis',(1.73292240336301E-13,-3.33769382396367E-14,
-1.));
#22078=DIRECTION('ref_axis',(0.986663993658341,0.162770278669582,1.64313007644524E-13));
#22079=DIRECTION('center_axis',(2.07777251728183E-13,-1.02140959738333E-13,
-1.));
#22080=DIRECTION('ref_axis',(0.986663993658371,-0.1627702786694,2.21673499735742E-13));
#22081=DIRECTION('center_axis',(1.,8.72635297355373E-14,0.));
#22082=DIRECTION('ref_axis',(8.72635297355373E-14,-1.,1.1518563880486E-13));
#22083=DIRECTION('',(4.36317648683653E-14,-0.500000000006838,-0.866025403780491));
#22084=DIRECTION('',(-4.36317648683479E-14,0.500000000006639,-0.866025403780606));
#22085=DIRECTION('',(-8.72635297355373E-14,1.,-1.1518563880486E-13));
#22086=DIRECTION('',(-4.36317648683653E-14,0.500000000006838,0.866025403780491));
#22087=DIRECTION('',(4.36317648683479E-14,-0.500000000006639,0.866025403780606));
#22088=DIRECTION('',(8.72635297355373E-14,-1.,1.1518563880486E-13));
#22089=DIRECTION('center_axis',(1.,8.72635297355373E-14,0.));
#22090=DIRECTION('ref_axis',(8.72635297355373E-14,-1.,1.1518563880486E-13));
#22091=DIRECTION('',(4.36317648683653E-14,-0.500000000006838,-0.866025403780491));
#22092=DIRECTION('',(-4.36317648683479E-14,0.500000000006639,-0.866025403780606));
#22093=DIRECTION('',(-8.72635297355373E-14,1.,-1.1518563880486E-13));
#22094=DIRECTION('',(-4.36317648683653E-14,0.500000000006838,0.866025403780491));
#22095=DIRECTION('',(4.36317648683479E-14,-0.500000000006639,0.866025403780606));
#22096=DIRECTION('',(8.72635297355373E-14,-1.,1.1518563880486E-13));
#22097=DIRECTION('center_axis',(-0.4999999999905,-1.43385454223719E-13,
-0.866025403789923));
#22098=DIRECTION('ref_axis',(-0.866025403789923,-1.79796141740169E-14,0.4999999999905));
#22099=DIRECTION('',(-0.866025403789921,-1.79796141740162E-14,0.499999999990505));
#22100=DIRECTION('',(8.72635297355373E-14,-1.,1.1518563880486E-13));
#22101=DIRECTION('',(-8.72635297355373E-14,1.,-1.1518563880486E-13));
#22102=DIRECTION('center_axis',(-1.,-8.72635297355373E-14,0.));
#22103=DIRECTION('ref_axis',(-8.72635297355373E-14,1.,-1.1518563880486E-13));
#22104=DIRECTION('',(-1.00515054169548E-26,1.1518563880486E-13,1.));
#22105=DIRECTION('',(8.72635297355373E-14,-1.,1.1518563880486E-13));
#22106=DIRECTION('center_axis',(-0.4999999999905,5.61219244898395E-14,0.866025403789923));
#22107=DIRECTION('ref_axis',(0.866025403789923,1.33165252976688E-13,0.4999999999905));
#22108=DIRECTION('',(0.866025403789921,1.33165252976689E-13,0.499999999990505));
#22109=DIRECTION('',(8.72635297355373E-14,-1.,1.1518563880486E-13));
#22110=DIRECTION('center_axis',(0.4999999999905,1.43385454223719E-13,0.866025403789923));
#22111=DIRECTION('ref_axis',(0.866025403789923,1.79796141740169E-14,-0.4999999999905));
#22112=DIRECTION('',(0.866025403789921,1.79796141740163E-14,-0.499999999990504));
#22113=DIRECTION('',(8.72635297355373E-14,-1.,1.1518563880486E-13));
#22114=DIRECTION('center_axis',(1.,8.72635297355373E-14,0.));
#22115=DIRECTION('ref_axis',(8.72635297355373E-14,-1.,1.1518563880486E-13));
#22116=DIRECTION('',(1.00515054169548E-26,-1.1518563880486E-13,-1.));
#22117=DIRECTION('',(8.72635297355373E-14,-1.,1.1518563880486E-13));
#22118=DIRECTION('center_axis',(0.4999999999905,-5.61219244898395E-14,-0.866025403789923));
#22119=DIRECTION('ref_axis',(-0.866025403789923,-1.33165252976688E-13,-0.4999999999905));
#22120=DIRECTION('',(-0.866025403789921,-1.33165252976689E-13,-0.499999999990504));
#22121=DIRECTION('center_axis',(-1.00515054169548E-26,1.1518563880486E-13,
1.));
#22122=DIRECTION('ref_axis',(-8.72635297355373E-14,1.,-1.1518563880486E-13));
#22123=DIRECTION('',(-8.72635297355373E-14,1.,-1.1518563880486E-13));
#22124=DIRECTION('',(-1.,-8.72635297355373E-14,0.));
#22125=DIRECTION('',(-8.72635297355373E-14,1.,-1.1518563880486E-13));
#22126=DIRECTION('',(-1.,-8.72635297355373E-14,0.));
#22127=DIRECTION('center_axis',(4.90114831233627E-14,4.90114831233761E-14,
1.));
#22128=DIRECTION('ref_axis',(-8.50113630284402E-14,1.,-5.07530525542927E-14));
#22129=DIRECTION('center_axis',(8.72635297355373E-14,-1.,1.1518563880486E-13));
#22130=DIRECTION('ref_axis',(-1.73003535575891E-29,1.1518563880486E-13,
1.));
#22131=DIRECTION('',(-8.72635297355373E-14,1.,-1.1518563880486E-13));
#22132=DIRECTION('center_axis',(5.42890133665177E-14,-1.,1.46185544222939E-13));
#22133=DIRECTION('ref_axis',(-1.,-5.32907051820067E-14,1.01506105108584E-14));
#22134=DIRECTION('center_axis',(8.05891463095976E-14,-1.,1.17347758652129E-13));
#22135=DIRECTION('ref_axis',(-1.,-8.12048840868677E-14,-1.21807326130302E-13));
#22136=DIRECTION('center_axis',(-1.,-8.72635297355373E-14,0.));
#22137=DIRECTION('ref_axis',(-8.72635297355373E-14,1.,-1.1518563880486E-13));
#22138=DIRECTION('',(1.00515054169548E-26,-1.1518563880486E-13,-1.));
#22139=DIRECTION('',(1.00515054169548E-26,-1.1518563880486E-13,-1.));
#22140=DIRECTION('',(8.72635297355373E-14,-1.,1.1518563880486E-13));
#22141=DIRECTION('center_axis',(-1.,-8.81911644086169E-14,6.42148752471851E-16));
#22142=DIRECTION('ref_axis',(-6.34413156928658E-16,-1.14194368247158E-13,
-1.));
#22143=DIRECTION('center_axis',(0.4999999999905,-5.61219244898395E-14,-0.866025403789923));
#22144=DIRECTION('ref_axis',(-0.866025403789923,-1.33165252976688E-13,-0.4999999999905));
#22145=DIRECTION('',(0.866025403789921,1.33165252976689E-13,0.499999999990504));
#22146=DIRECTION('',(8.72635297355373E-14,-1.,1.1518563880486E-13));
#22147=DIRECTION('',(-8.72635297355373E-14,1.,-1.1518563880486E-13));
#22148=DIRECTION('center_axis',(1.,8.72635297355373E-14,0.));
#22149=DIRECTION('ref_axis',(8.72635297355373E-14,-1.,1.1518563880486E-13));
#22150=DIRECTION('',(-1.00515054169548E-26,1.1518563880486E-13,1.));
#22151=DIRECTION('',(-8.72635297355373E-14,1.,-1.1518563880486E-13));
#22152=DIRECTION('center_axis',(0.4999999999905,1.43385454223719E-13,0.866025403789923));
#22153=DIRECTION('ref_axis',(0.866025403789923,1.79796141740169E-14,-0.4999999999905));
#22154=DIRECTION('',(-0.866025403789921,-1.79796141740163E-14,0.499999999990504));
#22155=DIRECTION('',(-8.72635297355373E-14,1.,-1.1518563880486E-13));
#22156=DIRECTION('center_axis',(-0.4999999999905,5.61219244898395E-14,0.866025403789923));
#22157=DIRECTION('ref_axis',(0.866025403789923,1.33165252976688E-13,0.4999999999905));
#22158=DIRECTION('',(-0.866025403789921,-1.33165252976689E-13,-0.499999999990505));
#22159=DIRECTION('',(-8.72635297355373E-14,1.,-1.1518563880486E-13));
#22160=DIRECTION('center_axis',(-1.,-8.72635297355373E-14,0.));
#22161=DIRECTION('ref_axis',(-8.72635297355373E-14,1.,-1.1518563880486E-13));
#22162=DIRECTION('',(1.00515054169548E-26,-1.1518563880486E-13,-1.));
#22163=DIRECTION('',(-8.72635297355373E-14,1.,-1.1518563880486E-13));
#22164=DIRECTION('center_axis',(-0.4999999999905,-1.43385454223719E-13,
-0.866025403789923));
#22165=DIRECTION('ref_axis',(-0.866025403789923,-1.79796141740169E-14,0.4999999999905));
#22166=DIRECTION('',(0.866025403789921,1.79796141740162E-14,-0.499999999990505));
#22167=DIRECTION('center_axis',(-1.00515054169548E-26,1.1518563880486E-13,
1.));
#22168=DIRECTION('ref_axis',(-8.72635297355373E-14,1.,-1.1518563880486E-13));
#22169=DIRECTION('',(-1.,-8.72635297355373E-14,0.));
#22170=DIRECTION('',(8.72635297355373E-14,-1.,1.1518563880486E-13));
#22171=DIRECTION('',(1.,8.72635297355373E-14,0.));
#22172=DIRECTION('',(8.72635297355373E-14,-1.,1.1518563880486E-13));
#22173=DIRECTION('center_axis',(-4.90114831233668E-14,4.90114831233573E-14,
1.));
#22174=DIRECTION('ref_axis',(-1.,-1.06581410364015E-13,-5.07530525542928E-14));
#22175=DIRECTION('center_axis',(-8.72635297355373E-14,1.,-1.1518563880486E-13));
#22176=DIRECTION('ref_axis',(1.73003535575891E-29,-1.1518563880486E-13,
-1.));
#22177=DIRECTION('',(8.72635297355373E-14,-1.,1.1518563880486E-13));
#22178=DIRECTION('center_axis',(-5.82913089187531E-14,1.,-8.87431404513285E-14));
#22179=DIRECTION('ref_axis',(1.,5.83660104374363E-14,1.01506105108585E-14));
#22180=DIRECTION('center_axis',(7.05441796996118E-14,-1.,1.009960112322E-13));
#22181=DIRECTION('ref_axis',(1.26882631385732E-15,1.01506105108585E-13,
1.));
#22182=DIRECTION('center_axis',(1.,8.72635297355373E-14,0.));
#22183=DIRECTION('ref_axis',(8.72635297355373E-14,-1.,1.1518563880486E-13));
#22184=DIRECTION('',(-8.72635297355373E-14,1.,-1.1518563880486E-13));
#22185=DIRECTION('',(1.00515054169548E-26,-1.1518563880486E-13,-1.));
#22186=DIRECTION('',(-1.00515054169548E-26,1.1518563880486E-13,1.));
#22187=DIRECTION('center_axis',(1.,8.90883600992922E-14,-2.80817075700569E-15));
#22188=DIRECTION('ref_axis',(-8.88178419700117E-14,1.,-1.01506105108585E-14));
#22189=DIRECTION('center_axis',(0.4999999999905,-5.61219244898395E-14,-0.866025403789923));
#22190=DIRECTION('ref_axis',(-0.866025403789923,-1.33165252976688E-13,-0.4999999999905));
#22191=DIRECTION('',(0.866025403789926,1.33165252976688E-13,0.499999999990495));
#22192=DIRECTION('',(8.72635297355373E-14,-1.,1.1518563880486E-13));
#22193=DIRECTION('',(-8.72635297355373E-14,1.,-1.1518563880486E-13));
#22194=DIRECTION('center_axis',(1.,8.72635297355373E-14,0.));
#22195=DIRECTION('ref_axis',(8.72635297355373E-14,-1.,1.1518563880486E-13));
#22196=DIRECTION('',(-1.00515054169548E-26,1.1518563880486E-13,1.));
#22197=DIRECTION('',(-8.72635297355373E-14,1.,-1.1518563880486E-13));
#22198=DIRECTION('center_axis',(0.4999999999905,1.43385454223719E-13,0.866025403789923));
#22199=DIRECTION('ref_axis',(0.866025403789923,1.79796141740169E-14,-0.4999999999905));
#22200=DIRECTION('',(-0.866025403789926,-1.79796141740178E-14,0.499999999990495));
#22201=DIRECTION('',(-8.72635297355373E-14,1.,-1.1518563880486E-13));
#22202=DIRECTION('center_axis',(-0.4999999999905,5.61219244898395E-14,0.866025403789923));
#22203=DIRECTION('ref_axis',(0.866025403789923,1.33165252976688E-13,0.4999999999905));
#22204=DIRECTION('',(-0.866025403789926,-1.33165252976688E-13,-0.499999999990495));
#22205=DIRECTION('',(-8.72635297355373E-14,1.,-1.1518563880486E-13));
#22206=DIRECTION('center_axis',(-1.,-8.72635297355373E-14,0.));
#22207=DIRECTION('ref_axis',(-8.72635297355373E-14,1.,-1.1518563880486E-13));
#22208=DIRECTION('',(1.00515054169548E-26,-1.1518563880486E-13,-1.));
#22209=DIRECTION('',(-8.72635297355373E-14,1.,-1.1518563880486E-13));
#22210=DIRECTION('center_axis',(-0.4999999999905,-1.43385454223719E-13,
-0.866025403789923));
#22211=DIRECTION('ref_axis',(-0.866025403789923,-1.79796141740169E-14,0.4999999999905));
#22212=DIRECTION('',(0.866025403789926,1.79796141740177E-14,-0.499999999990495));
#22213=DIRECTION('center_axis',(1.00515054169548E-26,-1.1518563880486E-13,
-1.));
#22214=DIRECTION('ref_axis',(8.72635297355373E-14,-1.,1.1518563880486E-13));
#22215=DIRECTION('',(1.,8.72635297355373E-14,0.));
#22216=DIRECTION('',(8.72635297355373E-14,-1.,1.1518563880486E-13));
#22217=DIRECTION('',(-1.,-8.72635297355373E-14,0.));
#22218=DIRECTION('',(8.72635297355373E-14,-1.,1.1518563880486E-13));
#22219=DIRECTION('center_axis',(-6.12643539041984E-14,-6.12643539042085E-14,
-1.));
#22220=DIRECTION('ref_axis',(1.,7.86672314591538E-14,-6.09036630651514E-14));
#22221=DIRECTION('center_axis',(-8.72635297355373E-14,1.,-1.1518563880486E-13));
#22222=DIRECTION('ref_axis',(1.73003535575891E-29,-1.1518563880486E-13,
-1.));
#22223=DIRECTION('',(8.72635297355373E-14,-1.,1.1518563880486E-13));
#22224=DIRECTION('center_axis',(-4.42440467565883E-14,1.,-7.21582256614495E-14));
#22225=DIRECTION('ref_axis',(-1.,-4.31400946711492E-14,5.07530525542931E-15));
#22226=DIRECTION('center_axis',(8.1002659099073E-14,-1.,1.0891683800392E-13));
#22227=DIRECTION('ref_axis',(1.26882631385732E-15,-1.0911906299173E-13,
-1.));
#22228=DIRECTION('center_axis',(-1.,-8.72635297355373E-14,0.));
#22229=DIRECTION('ref_axis',(-8.72635297355373E-14,1.,-1.1518563880486E-13));
#22230=DIRECTION('',(-8.72635297355373E-14,1.,-1.1518563880486E-13));
#22231=DIRECTION('',(-1.00515054169548E-26,1.1518563880486E-13,1.));
#22232=DIRECTION('',(1.00515054169548E-26,-1.1518563880486E-13,-1.));
#22233=DIRECTION('center_axis',(-1.,-8.81911644086279E-14,-6.4214875247015E-16));
#22234=DIRECTION('ref_axis',(-8.81834288130837E-14,1.,0.));
#22235=DIRECTION('center_axis',(-8.72635297355373E-14,1.,-1.1518563880486E-13));
#22236=DIRECTION('ref_axis',(1.00515054169548E-26,-1.1518563880486E-13,
-1.));
#22237=DIRECTION('',(1.,8.72635297355373E-14,0.));
#22238=DIRECTION('',(1.00515054169548E-26,-1.1518563880486E-13,-1.));
#22239=DIRECTION('',(1.,8.72635297355373E-14,0.));
#22240=DIRECTION('center_axis',(-6.73907892946183E-14,-1.,6.73907892946096E-14));
#22241=DIRECTION('ref_axis',(1.,-6.85166209482953E-14,1.26882631385732E-13));
#22242=DIRECTION('',(-1.00515054169548E-26,1.1518563880486E-13,1.));
#22243=DIRECTION('',(-1.,-8.72635297355373E-14,0.));
#22244=DIRECTION('',(-1.00515054169548E-26,1.1518563880486E-13,1.));
#22245=DIRECTION('center_axis',(0.4999999999905,-5.61219244898395E-14,-0.866025403789923));
#22246=DIRECTION('ref_axis',(-0.866025403789923,-1.33165252976688E-13,-0.4999999999905));
#22247=DIRECTION('',(0.866025403789926,1.33165252976688E-13,0.499999999990495));
#22248=DIRECTION('',(8.72635297355373E-14,-1.,1.1518563880486E-13));
#22249=DIRECTION('',(-8.72635297355373E-14,1.,-1.1518563880486E-13));
#22250=DIRECTION('center_axis',(1.,8.72635297355373E-14,0.));
#22251=DIRECTION('ref_axis',(8.72635297355373E-14,-1.,1.1518563880486E-13));
#22252=DIRECTION('',(-1.00515054169548E-26,1.1518563880486E-13,1.));
#22253=DIRECTION('',(-8.72635297355373E-14,1.,-1.1518563880486E-13));
#22254=DIRECTION('center_axis',(0.4999999999905,1.43385454223719E-13,0.866025403789923));
#22255=DIRECTION('ref_axis',(0.866025403789923,1.79796141740169E-14,-0.4999999999905));
#22256=DIRECTION('',(-0.866025403789926,-1.79796141740178E-14,0.499999999990495));
#22257=DIRECTION('',(-8.72635297355373E-14,1.,-1.1518563880486E-13));
#22258=DIRECTION('center_axis',(-0.4999999999905,5.61219244898395E-14,0.866025403789923));
#22259=DIRECTION('ref_axis',(0.866025403789923,1.33165252976688E-13,0.4999999999905));
#22260=DIRECTION('',(-0.866025403789926,-1.33165252976688E-13,-0.499999999990495));
#22261=DIRECTION('',(-8.72635297355373E-14,1.,-1.1518563880486E-13));
#22262=DIRECTION('center_axis',(-1.,-8.72635297355373E-14,0.));
#22263=DIRECTION('ref_axis',(-8.72635297355373E-14,1.,-1.1518563880486E-13));
#22264=DIRECTION('',(1.00515054169548E-26,-1.1518563880486E-13,-1.));
#22265=DIRECTION('',(-8.72635297355373E-14,1.,-1.1518563880486E-13));
#22266=DIRECTION('center_axis',(-0.4999999999905,-1.43385454223719E-13,
-0.866025403789923));
#22267=DIRECTION('ref_axis',(-0.866025403789923,-1.79796141740169E-14,0.4999999999905));
#22268=DIRECTION('',(0.866025403789926,1.79796141740177E-14,-0.499999999990495));
#22269=DIRECTION('center_axis',(1.,8.72635297355373E-14,0.));
#22270=DIRECTION('ref_axis',(8.72635297355373E-14,-1.,1.1518563880486E-13));
#22271=DIRECTION('',(8.72635297355373E-14,-1.,1.1518563880486E-13));
#22272=DIRECTION('',(1.00515054169548E-26,-1.1518563880486E-13,-1.));
#22273=DIRECTION('',(8.72635297355373E-14,-1.,1.1518563880486E-13));
#22274=DIRECTION('center_axis',(1.,8.90883600993061E-14,2.80817075700403E-15));
#22275=DIRECTION('ref_axis',(-2.53765262771465E-15,4.82153999265783E-14,
1.));
#22276=DIRECTION('center_axis',(-8.72635297355373E-14,1.,-1.1518563880486E-13));
#22277=DIRECTION('ref_axis',(1.73003535575891E-29,-1.1518563880486E-13,
-1.));
#22278=DIRECTION('',(8.72635297355373E-14,-1.,1.1518563880486E-13));
#22279=DIRECTION('center_axis',(6.73907892946244E-14,1.,-6.73907892946245E-14));
#22280=DIRECTION('ref_axis',(-2.53765262771465E-15,-6.85166209482954E-14,
-1.));
#22281=DIRECTION('center_axis',(1.00515054169548E-26,-1.1518563880486E-13,
-1.));
#22282=DIRECTION('ref_axis',(8.72635297355373E-14,-1.,1.1518563880486E-13));
#22283=DIRECTION('',(-8.72635297355373E-14,1.,-1.1518563880486E-13));
#22284=DIRECTION('',(-1.,-8.72635297355373E-14,0.));
#22285=DIRECTION('center_axis',(7.35172246850504E-14,-7.35172246850366E-14,
-1.));
#22286=DIRECTION('ref_axis',(-8.62801893422977E-14,1.,-7.10542735760099E-14));
#22287=DIRECTION('center_axis',(-1.04744440165193E-14,-1.15185638804861E-13,
-1.));
#22288=DIRECTION('ref_axis',(-1.,-8.71698546678346E-14,1.04744440165294E-14));
#22289=DIRECTION('',(1.04744440165193E-14,1.15185638804861E-13,1.));
#22290=DIRECTION('',(-5.23722200825506E-15,-1.09948416796596E-13,-1.));
#22291=DIRECTION('center_axis',(2.66521584365477E-12,-5.1895433423456E-12,
1.));
#22292=DIRECTION('ref_axis',(0.707106781186605,-0.70710678118649,-5.55555601522426E-12));
#22293=DIRECTION('center_axis',(0.707106781186606,-0.707106781186489,7.40419959009745E-14));
#22294=DIRECTION('ref_axis',(-0.707106781186489,-0.707106781186606,8.14485462942204E-14));
#22295=DIRECTION('',(-1.04744440165193E-14,-1.15185638804861E-13,-1.));
#22296=DIRECTION('',(0.707106781186493,0.707106781186602,-8.95362847158453E-14));
#22297=DIRECTION('center_axis',(-1.04744440165193E-14,-1.15185638804861E-13,
-1.));
#22298=DIRECTION('ref_axis',(-1.,-8.71698546678346E-14,1.04744440165294E-14));
#22299=DIRECTION('',(-1.04744440165193E-14,-1.15185638804861E-13,-1.));
#22300=DIRECTION('center_axis',(4.57696995050001E-12,-2.23639690875147E-12,
1.));
#22301=DIRECTION('ref_axis',(0.986663993658371,-0.162770278669399,-4.88054041625221E-12));
#22302=DIRECTION('center_axis',(-1.04744440165193E-14,-1.15185638804861E-13,
-1.));
#22303=DIRECTION('ref_axis',(1.,9.24743105072028E-14,-1.047444401653E-14));
#22304=DIRECTION('',(-1.04744440165193E-14,-1.15185638804861E-13,-1.));
#22305=DIRECTION('center_axis',(1.67705924609206E-12,1.20380416834642E-13,
1.));
#22306=DIRECTION('ref_axis',(0.986663993658341,0.162770278669584,-1.67442661407532E-12));
#22307=DIRECTION('center_axis',(-1.04744440165193E-14,-1.15185638804861E-13,
-1.));
#22308=DIRECTION('ref_axis',(-1.,-8.72782748850831E-14,1.04744440165294E-14));
#22309=DIRECTION('',(-5.23722200825424E-15,-1.20422860813125E-13,-1.));
#22310=DIRECTION('center_axis',(4.86004852695852E-12,2.49599579008935E-12,
1.));
#22311=DIRECTION('ref_axis',(0.707106781186489,0.707106781186606,-5.20028464734421E-12));
#22312=DIRECTION('center_axis',(0.707106781186489,0.707106781186606,-8.88550966874672E-14));
#22313=DIRECTION('ref_axis',(0.707106781186606,-0.707106781186489,8.14485462942212E-14));
#22314=DIRECTION('',(-1.04744440165193E-14,-1.15185638804861E-13,-1.));
#22315=DIRECTION('',(-0.707106781186601,0.707106781186494,-7.33608078725965E-14));
#22316=DIRECTION('center_axis',(-1.04744440165193E-14,-1.15185638804861E-13,
-1.));
#22317=DIRECTION('ref_axis',(-1.,-8.71698546678346E-14,1.04744440165294E-14));
#22318=DIRECTION('',(-1.04744440165193E-14,-1.15185638804861E-13,-1.));
#22319=DIRECTION('center_axis',(3.04596096417561E-12,5.93090667696643E-12,
1.));
#22320=DIRECTION('ref_axis',(0.162770278669402,0.986663993658371,-6.34603480875743E-12));
#22321=DIRECTION('center_axis',(-1.04744440165193E-14,-1.15185638804861E-13,
-1.));
#22322=DIRECTION('ref_axis',(-1.,-8.72097194830903E-14,1.04744440165294E-14));
#22323=DIRECTION('',(-1.04744440165193E-14,-1.15185638804861E-13,-1.));
#22324=DIRECTION('center_axis',(-5.78383051437747E-13,7.50458952439442E-12,
1.));
#22325=DIRECTION('ref_axis',(-0.162770278669582,0.986663993658341,-7.49850197409643E-12));
#22326=DIRECTION('center_axis',(-1.04744440165193E-14,-1.15185638804861E-13,
-1.));
#22327=DIRECTION('ref_axis',(-1.,-8.71698546678346E-14,1.04744440165294E-14));
#22328=DIRECTION('',(-5.23722200825505E-15,-1.09948416796596E-13,-1.));
#22329=DIRECTION('center_axis',(-2.58060581687203E-12,5.02479593465201E-12,
1.));
#22330=DIRECTION('ref_axis',(-0.707106781186607,0.707106781186488,-5.37792033128426E-12));
#22331=DIRECTION('center_axis',(-0.707106781186605,0.70710678118649,-7.40419959009746E-14));
#22332=DIRECTION('ref_axis',(0.70710678118649,0.707106781186605,-8.14485462942203E-14));
#22333=DIRECTION('',(-1.04744440165193E-14,-1.15185638804861E-13,-1.));
#22334=DIRECTION('',(-0.707106781186489,-0.707106781186606,8.54924155050331E-14));
#22335=DIRECTION('center_axis',(-1.04744440165193E-14,-1.15185638804861E-13,
-1.));
#22336=DIRECTION('ref_axis',(-1.,-8.72782748850831E-14,1.04744440165294E-14));
#22337=DIRECTION('center_axis',(-5.63736932649778E-12,3.00942475177315E-12,
1.));
#22338=DIRECTION('ref_axis',(-0.986663993658371,0.162770278669398,-6.05293593025637E-12));
#22339=DIRECTION('center_axis',(-1.04744440165193E-14,-1.15185638804861E-13,
-1.));
#22340=DIRECTION('ref_axis',(-1.,-8.71698546678346E-14,1.04744440165294E-14));
#22341=DIRECTION('',(-5.23722200825426E-15,-1.20422860813125E-13,-1.));
#22342=DIRECTION('center_axis',(-5.68569950679339E-12,-2.8139702200907E-12,
1.));
#22343=DIRECTION('ref_axis',(-0.70710678118649,-0.707106781186605,-6.00852700927135E-12));
#22344=DIRECTION('center_axis',(-0.70710678118649,-0.707106781186605,8.88550966874671E-14));
#22345=DIRECTION('ref_axis',(-0.707106781186605,0.70710678118649,-8.14485462942213E-14));
#22346=DIRECTION('',(-1.04744440165193E-14,-1.15185638804861E-13,-1.));
#22347=DIRECTION('',(0.707106781186601,-0.707106781186494,7.74046770834091E-14));
#22348=DIRECTION('center_axis',(-1.04744440165193E-14,-1.15185638804861E-13,
-1.));
#22349=DIRECTION('ref_axis',(-1.,-8.71698546678346E-14,1.04744440165294E-14));
#22350=DIRECTION('',(-1.04744440165193E-14,-1.15185638804861E-13,-1.));
#22351=DIRECTION('center_axis',(-2.65628776850208E-12,-4.93387739816273E-12,
1.));
#22352=DIRECTION('ref_axis',(-0.162770278669406,-0.98666399365837,-5.30242516560978E-12));
#22353=DIRECTION('center_axis',(-1.04744440165193E-14,-1.15185638804861E-13,
-1.));
#22354=DIRECTION('ref_axis',(-1.,-8.72870330641923E-14,1.04744440165294E-14));
#22355=DIRECTION('center_axis',(6.31496326740432E-13,-7.26238032379499E-12,
1.));
#22356=DIRECTION('ref_axis',(0.162770278669577,-0.986663993658342,-7.26851571812066E-12));
#22357=DIRECTION('center_axis',(7.55724335745396E-14,-0.866025403780606,
-0.500000000006639));
#22358=DIRECTION('ref_axis',(4.36317648683479E-14,-0.500000000006639,0.866025403780606));
#22359=DIRECTION('',(-1.,-8.72635297355373E-14,0.));
#22360=DIRECTION('',(1.,8.72635297355373E-14,0.));
#22361=DIRECTION('center_axis',(7.55724335745396E-14,-0.866025403780606,
-0.500000000006639));
#22362=DIRECTION('ref_axis',(0.,-0.500000000006639,0.866025403780606));
#22363=DIRECTION('center_axis',(7.55724335745296E-14,-0.866025403780491,
0.500000000006838));
#22364=DIRECTION('ref_axis',(-4.36317648683653E-14,0.500000000006838,0.866025403780491));
#22365=DIRECTION('',(1.,8.72635297355373E-14,0.));
#22366=DIRECTION('center_axis',(7.55724335745296E-14,-0.866025403780491,
0.500000000006838));
#22367=DIRECTION('ref_axis',(0.,0.500000000006838,0.866025403780491));
#22368=DIRECTION('center_axis',(-1.00515054169548E-26,1.1518563880486E-13,
1.));
#22369=DIRECTION('ref_axis',(-8.72635297355373E-14,1.,-1.1518563880486E-13));
#22370=DIRECTION('',(1.,8.72635297355373E-14,0.));
#22371=DIRECTION('center_axis',(-2.00908022958255E-11,-2.95761452118009E-13,
1.));
#22372=DIRECTION('ref_axis',(0.989245507946394,0.146264571950559,1.99196012991554E-11));
#22373=DIRECTION('center_axis',(-7.55724335745396E-14,0.866025403780606,
0.500000000006639));
#22374=DIRECTION('ref_axis',(-4.36317648683479E-14,0.500000000006639,-0.866025403780606));
#22375=DIRECTION('',(1.,8.72635297355373E-14,0.));
#22376=DIRECTION('center_axis',(-7.55724335745396E-14,0.866025403780606,
0.500000000006639));
#22377=DIRECTION('ref_axis',(0.,0.500000000006639,-0.866025403780606));
#22378=DIRECTION('center_axis',(-7.55724335745296E-14,0.866025403780491,
-0.500000000006838));
#22379=DIRECTION('ref_axis',(4.36317648683653E-14,-0.500000000006838,-0.866025403780491));
#22380=DIRECTION('',(1.,8.72635297355373E-14,0.));
#22381=DIRECTION('center_axis',(-7.55724335745296E-14,0.866025403780491,
-0.500000000006838));
#22382=DIRECTION('ref_axis',(0.,-0.500000000006838,-0.866025403780491));
#22383=DIRECTION('center_axis',(1.00515054169548E-26,-1.1518563880486E-13,
-1.));
#22384=DIRECTION('ref_axis',(8.72635297355373E-14,-1.,1.1518563880486E-13));
#22385=DIRECTION('center_axis',(4.00087977969525E-12,-2.94175337366331E-13,
-1.));
#22386=DIRECTION('ref_axis',(0.989245507946313,-0.14626457195111,3.99976089707118E-12));
#22387=DIRECTION('center_axis',(7.55724335745396E-14,-0.866025403780606,
-0.500000000006639));
#22388=DIRECTION('ref_axis',(4.36317648683479E-14,-0.500000000006639,0.866025403780606));
#22389=DIRECTION('',(-1.,-8.72635297355373E-14,0.));
#22390=DIRECTION('',(1.,8.72635297355373E-14,0.));
#22391=DIRECTION('center_axis',(7.55724335745396E-14,-0.866025403780606,
-0.500000000006639));
#22392=DIRECTION('ref_axis',(0.,-0.500000000006639,0.866025403780606));
#22393=DIRECTION('center_axis',(7.55724335745296E-14,-0.866025403780491,
0.500000000006838));
#22394=DIRECTION('ref_axis',(-4.36317648683653E-14,0.500000000006838,0.866025403780491));
#22395=DIRECTION('',(1.,8.72635297355373E-14,0.));
#22396=DIRECTION('center_axis',(7.55724335745296E-14,-0.866025403780491,
0.500000000006838));
#22397=DIRECTION('ref_axis',(0.,0.500000000006838,0.866025403780491));
#22398=DIRECTION('center_axis',(-1.00515054169548E-26,1.1518563880486E-13,
1.));
#22399=DIRECTION('ref_axis',(-8.72635297355373E-14,1.,-1.1518563880486E-13));
#22400=DIRECTION('',(1.,8.72635297355373E-14,0.));
#22401=DIRECTION('center_axis',(3.33226641230312E-12,2.69627681862394E-13,
1.));
#22402=DIRECTION('ref_axis',(0.98924550794629,0.146264571951266,-3.33733424985186E-12));
#22403=DIRECTION('center_axis',(-7.55724335745396E-14,0.866025403780606,
0.500000000006639));
#22404=DIRECTION('ref_axis',(-4.36317648683479E-14,0.500000000006639,-0.866025403780606));
#22405=DIRECTION('',(1.,8.72635297355373E-14,0.));
#22406=DIRECTION('center_axis',(-7.55724335745396E-14,0.866025403780606,
0.500000000006639));
#22407=DIRECTION('ref_axis',(0.,0.500000000006639,-0.866025403780606));
#22408=DIRECTION('center_axis',(-7.55724335745296E-14,0.866025403780491,
-0.500000000006838));
#22409=DIRECTION('ref_axis',(4.36317648683653E-14,-0.500000000006838,-0.866025403780491));
#22410=DIRECTION('',(1.,8.72635297355373E-14,0.));
#22411=DIRECTION('center_axis',(-7.55724335745296E-14,0.866025403780491,
-0.500000000006838));
#22412=DIRECTION('ref_axis',(0.,-0.500000000006838,-0.866025403780491));
#22413=DIRECTION('center_axis',(1.00515054169548E-26,-1.1518563880486E-13,
-1.));
#22414=DIRECTION('ref_axis',(8.72635297355373E-14,-1.,1.1518563880486E-13));
#22415=DIRECTION('center_axis',(2.66725318646372E-12,-1.96116891577676E-13,
-1.));
#22416=DIRECTION('ref_axis',(0.989245507946304,-0.146264571951168,2.66770731298914E-12));
#22417=DIRECTION('center_axis',(1.00515054169548E-26,-1.1518563880486E-13,
-1.));
#22418=DIRECTION('ref_axis',(8.72318090776908E-14,-1.,1.1518563880486E-13));
#22419=DIRECTION('',(-1.00515054169548E-26,1.1518563880486E-13,1.));
#22420=DIRECTION('center_axis',(1.,8.72635297355373E-14,0.));
#22421=DIRECTION('ref_axis',(8.72635297355373E-14,-1.,1.18952466924124E-13));
#22422=DIRECTION('',(1.,8.72635297355373E-14,0.));
#22423=DIRECTION('center_axis',(8.72635297355373E-14,-1.,1.1518563880486E-13));
#22424=DIRECTION('ref_axis',(-1.00515054169548E-26,1.1518563880486E-13,
1.));
#22425=DIRECTION('center_axis',(8.49211903186698E-14,-1.,1.15553367270777E-13));
#22426=DIRECTION('ref_axis',(1.,8.37425367145833E-14,9.13554945977273E-14));
#22427=DIRECTION('',(1.,8.72635297355373E-14,0.));
#22428=DIRECTION('',(-1.00515054169548E-26,1.1518563880486E-13,1.));
#22429=DIRECTION('center_axis',(-1.00515054169548E-26,1.1518563880486E-13,
1.));
#22430=DIRECTION('ref_axis',(-8.72318090776908E-14,1.,-1.1518563880486E-13));
#22431=DIRECTION('',(1.00515054169548E-26,-1.1518563880486E-13,-1.));
#22432=DIRECTION('center_axis',(-8.72635297355373E-14,1.,-1.1518563880486E-13));
#22433=DIRECTION('ref_axis',(1.00515054169548E-26,-1.1518563880486E-13,
-1.));
#22434=DIRECTION('',(1.,8.72635297355373E-14,0.));
#22435=DIRECTION('center_axis',(8.71290944895014E-14,-1.,1.15043273394353E-13));
#22436=DIRECTION('ref_axis',(-1.26882631385732E-15,-1.14194368247158E-13,
-1.));
#22437=DIRECTION('',(1.00515054169548E-26,-1.1518563880486E-13,-1.));
#22438=DIRECTION('center_axis',(-8.72635297355373E-14,1.,-1.1518563880486E-13));
#22439=DIRECTION('ref_axis',(1.00515054169548E-26,-1.1518563880486E-13,
-1.));
#22440=DIRECTION('',(-1.,-8.72635297355373E-14,0.));
#22441=DIRECTION('center_axis',(8.2797050480443E-14,-1.,1.13248882013028E-13));
#22442=DIRECTION('ref_axis',(-1.26882631385733E-15,1.1419436824716E-13,
1.));
#22443=DIRECTION('',(-1.00515054169548E-26,1.1518563880486E-13,1.));
#22444=DIRECTION('center_axis',(1.,8.72635297355373E-14,0.));
#22445=DIRECTION('ref_axis',(8.72635297355373E-14,-1.,1.18952466924124E-13));
#22446=DIRECTION('',(-1.,-8.72635297355373E-14,0.));
#22447=DIRECTION('center_axis',(-8.72635297355373E-14,1.,-1.1518563880486E-13));
#22448=DIRECTION('ref_axis',(1.00515054169548E-26,-1.1518563880486E-13,
-1.));
#22449=DIRECTION('',(1.00515054169548E-26,-1.1518563880486E-13,-1.));
#22450=DIRECTION('center_axis',(-1.8379306171262E-14,-1.,1.83793061712636E-14));
#22451=DIRECTION('ref_axis',(-1.,1.77635683940026E-14,7.61295788314397E-14));
#22452=DIRECTION('',(-1.,-8.72635297355373E-14,0.));
#22453=DIRECTION('center_axis',(-0.86602540378448,0.499999999999929,-4.85216847935981E-14));
#22454=DIRECTION('ref_axis',(0.499999999999929,0.86602540378448,-9.9753689356147E-14));
#22455=DIRECTION('',(0.499999999999923,0.866025403784483,-1.06713055052629E-13));
#22456=DIRECTION('',(-1.04744440165193E-14,-1.15185638804861E-13,-1.));
#22457=DIRECTION('center_axis',(-1.04744440165193E-14,-1.15185638804861E-13,
-1.));
#22458=DIRECTION('ref_axis',(-1.,-8.72533584376409E-14,1.04744440165294E-14));
#22459=DIRECTION('center_axis',(-4.93888884645662E-14,-1.74996285159289E-13,
-1.));
#22460=DIRECTION('ref_axis',(-0.757843547050805,-0.652436325010689,1.51817826771104E-13));
#22461=DIRECTION('',(-2.61861100412291E-15,-1.10650071500444E-13,-1.));
#22462=DIRECTION('center_axis',(0.500000000000096,-0.866025403784383,9.4516467347881E-14));
#22463=DIRECTION('ref_axis',(-0.866025403784383,-0.500000000000096,5.75928194024323E-14));
#22464=DIRECTION('',(-0.866025403784382,-0.500000000000098,6.45521992358119E-14));
#22465=DIRECTION('center_axis',(-0.499999999999945,-0.866025403784471,1.04990911364411E-13));
#22466=DIRECTION('ref_axis',(-0.866025403784471,0.499999999999945,-5.75928194024323E-14));
#22467=DIRECTION('',(-0.866025403784468,0.499999999999948,-4.71542784478838E-14));
#22468=DIRECTION('',(-1.04744440165193E-14,-1.15185638804861E-13,-1.));
#22469=DIRECTION('center_axis',(-1.04744440165193E-14,-1.15185638804861E-13,
-1.));
#22470=DIRECTION('ref_axis',(-1.,-8.72533584376409E-14,1.04744440165294E-14));
#22471=DIRECTION('center_axis',(4.93888884646039E-14,-1.74996285159287E-13,
-1.));
#22472=DIRECTION('ref_axis',(0.652436325010704,-0.757843547050793,1.65057753524397E-13));
#22473=DIRECTION('',(-7.85583301238657E-15,-1.19721206109277E-13,-1.));
#22474=DIRECTION('center_axis',(0.866025403784393,0.50000000000008,-6.66639540112628E-14));
#22475=DIRECTION('ref_axis',(0.50000000000008,-0.866025403784393,9.9753689356147E-14));
#22476=DIRECTION('',(0.500000000000079,-0.866025403784393,9.62741799074761E-14));
#22477=DIRECTION('center_axis',(0.86602540378448,-0.499999999999929,4.85216847935981E-14));
#22478=DIRECTION('ref_axis',(-0.499999999999929,-0.86602540378448,9.9753689356147E-14));
#22479=DIRECTION('',(-0.49999999999993,-0.866025403784479,1.03233198804818E-13));
#22480=DIRECTION('',(-1.04744440165193E-14,-1.15185638804861E-13,-1.));
#22481=DIRECTION('center_axis',(-1.04744440165193E-14,-1.15185638804861E-13,
-1.));
#22482=DIRECTION('ref_axis',(-1.,-8.72533584376409E-14,1.04744440165294E-14));
#22483=DIRECTION('center_axis',(-5.77627149108745E-14,-1.66622458712969E-13,
-1.));
#22484=DIRECTION('ref_axis',(0.757843547050804,0.65243632501069,-1.52700488554662E-13));
#22485=DIRECTION('',(-2.61861100412291E-15,-1.10650071500444E-13,-1.));
#22486=DIRECTION('center_axis',(-0.500000000000096,0.866025403784383,-9.4516467347881E-14));
#22487=DIRECTION('ref_axis',(0.866025403784383,0.500000000000096,-5.75928194024323E-14));
#22488=DIRECTION('',(0.866025403784385,0.500000000000094,-6.80317109102609E-14));
#22489=DIRECTION('center_axis',(0.499999999999945,0.866025403784471,-1.04990911364411E-13));
#22490=DIRECTION('ref_axis',(0.866025403784471,-0.499999999999945,5.75928194024323E-14));
#22491=DIRECTION('',(0.86602540378447,-0.499999999999945,5.0632879163502E-14));
#22492=DIRECTION('',(-1.04744440165193E-14,-1.15185638804861E-13,-1.));
#22493=DIRECTION('center_axis',(-1.04744440165193E-14,-1.15185638804861E-13,
-1.));
#22494=DIRECTION('ref_axis',(-1.,-8.72533584376409E-14,1.04744440165294E-14));
#22495=DIRECTION('center_axis',(4.93888884645922E-14,-1.74996285159275E-13,
-1.));
#22496=DIRECTION('ref_axis',(-0.652436325010692,0.757843547050803,-1.65057753524405E-13));
#22497=DIRECTION('',(-7.85583301238656E-15,-1.19721206109277E-13,-1.));
#22498=DIRECTION('center_axis',(-0.866025403784393,-0.500000000000079,6.66639540112628E-14));
#22499=DIRECTION('ref_axis',(-0.500000000000079,0.866025403784393,-9.97536893561471E-14));
#22500=DIRECTION('',(-0.500000000000078,0.866025403784394,-9.27937835876813E-14));
#22501=DIRECTION('center_axis',(-1.04744440165193E-14,-1.15185638804861E-13,
-1.));
#22502=DIRECTION('ref_axis',(-1.,-8.72635297355361E-14,1.04744440165294E-14));
#22503=DIRECTION('center_axis',(1.14717457973843E-12,4.09170500797773E-13,
1.));
#22504=DIRECTION('ref_axis',(0.977277070396433,0.211965864415397,-1.20792265079108E-12));
#22505=DIRECTION('center_axis',(0.,0.,1.));
#22506=DIRECTION('ref_axis',(0.984863869999403,-0.173329621155183,0.));
#22507=DIRECTION('center_axis',(-4.47790050492473E-13,2.40527186556087E-12,
1.));
#22508=DIRECTION('ref_axis',(0.211965864415374,-0.977277070396437,2.44568809648228E-12));
#22509=DIRECTION('center_axis',(1.41284845480624E-12,7.19501758928192E-12,
1.));
#22510=DIRECTION('ref_axis',(-0.173329621155189,-0.984863869999402,7.33090625241919E-12));
#22511=DIRECTION('center_axis',(-2.39833919642918E-12,-4.70949484936173E-13,
1.));
#22512=DIRECTION('ref_axis',(-0.977277070396424,-0.211965864415433,-2.44379331585598E-12));
#22513=DIRECTION('center_axis',(-1.19362346291077E-11,2.54002290023133E-12,
1.));
#22514=DIRECTION('ref_axis',(-0.98486386999939,0.173329621155259,-1.21957555165768E-11));
#22515=DIRECTION('center_axis',(-1.05315117764831E-14,-2.7438796246474E-15,
1.));
#22516=DIRECTION('ref_axis',(-0.211965864415394,0.977277070396433,4.7369515717317E-16));
#22517=DIRECTION('center_axis',(1.00515054169548E-26,-1.1518563880486E-13,
-1.));
#22518=DIRECTION('ref_axis',(8.72635297355373E-14,-1.,1.1518563880486E-13));
#22519=DIRECTION('center_axis',(1.91944255730871E-14,-1.10978678768031E-13,
-1.));
#22520=DIRECTION('ref_axis',(1.,0.,1.95434151289614E-14));
#22521=DIRECTION('center_axis',(1.9194425573087E-14,-1.1097867876803E-13,
-1.));
#22522=DIRECTION('ref_axis',(1.,0.,1.95434151289613E-14));
#22523=DIRECTION('center_axis',(-8.72635297355373E-14,1.,-1.1518563880486E-13));
#22524=DIRECTION('ref_axis',(1.73003535575891E-29,-1.1518563880486E-13,
-1.));
#22525=DIRECTION('center_axis',(-8.71290944895063E-14,1.,-1.15043273394367E-13));
#22526=DIRECTION('ref_axis',(1.,8.6280189342298E-14,0.));
#22527=DIRECTION('',(8.72635297355373E-14,-1.,1.1518563880486E-13));
#22528=DIRECTION('',(-8.72635297355373E-14,1.,-1.1518563880486E-13));
#22529=DIRECTION('center_axis',(1.,8.72635297355373E-14,0.));
#22530=DIRECTION('ref_axis',(8.72635297355373E-14,-1.,1.1518563880486E-13));
#22531=DIRECTION('',(1.00515054169548E-26,-1.1518563880486E-13,-1.));
#22532=DIRECTION('',(8.72635297355373E-14,-1.,1.1518563880486E-13));
#22533=DIRECTION('center_axis',(-8.72635297355373E-14,1.,-1.1518563880486E-13));
#22534=DIRECTION('ref_axis',(1.73003535575891E-29,-1.1518563880486E-13,
-1.));
#22535=DIRECTION('center_axis',(-8.67155817000303E-14,1.,-1.11221323261711E-13));
#22536=DIRECTION('ref_axis',(-1.26882631385732E-15,-1.11656715619444E-13,
-1.));
#22537=DIRECTION('',(8.72635297355373E-14,-1.,1.1518563880486E-13));
#22538=DIRECTION('center_axis',(1.00515054169548E-26,-1.1518563880486E-13,
-1.));
#22539=DIRECTION('ref_axis',(8.72635297355373E-14,-1.,1.1518563880486E-13));
#22540=DIRECTION('',(-1.,-8.72635297355373E-14,0.));
#22541=DIRECTION('',(8.72635297355373E-14,-1.,1.1518563880486E-13));
#22542=DIRECTION('center_axis',(-8.72635297355373E-14,1.,-1.1518563880486E-13));
#22543=DIRECTION('ref_axis',(1.73003535575891E-29,-1.1518563880486E-13,
-1.));
#22544=DIRECTION('center_axis',(-8.27970504804384E-14,1.,-1.13248882013014E-13));
#22545=DIRECTION('ref_axis',(-1.,-8.37425367145831E-14,0.));
#22546=DIRECTION('',(8.72635297355373E-14,-1.,1.1518563880486E-13));
#22547=DIRECTION('center_axis',(-1.,-8.72635297355373E-14,0.));
#22548=DIRECTION('ref_axis',(-8.72635297355373E-14,1.,-1.1518563880486E-13));
#22549=DIRECTION('',(-1.00515054169548E-26,1.1518563880486E-13,1.));
#22550=DIRECTION('',(8.72635297355373E-14,-1.,1.1518563880486E-13));
#22551=DIRECTION('center_axis',(-8.72635297355373E-14,1.,-1.1518563880486E-13));
#22552=DIRECTION('ref_axis',(1.73003535575891E-29,-1.1518563880486E-13,
-1.));
#22553=DIRECTION('center_axis',(1.22528707808408E-14,1.,-1.22528707808409E-14));
#22554=DIRECTION('ref_axis',(0.,1.26882631385732E-14,1.));
#22555=DIRECTION('',(8.72635297355373E-14,-1.,1.1518563880486E-13));
#22556=DIRECTION('center_axis',(-1.00515054169548E-26,1.1518563880486E-13,
1.));
#22557=DIRECTION('ref_axis',(-8.72635297355373E-14,1.,-1.1518563880486E-13));
#22558=DIRECTION('',(1.,8.72635297355373E-14,0.));
#22559=DIRECTION('',(0.379745299517171,0.590960642274619,-0.711729602290775));
#22560=DIRECTION('',(-0.476347793731818,-0.412136157605333,0.776683054405812));
#22561=DIRECTION('',(0.590600287990408,0.380161574531733,-0.711806488503161));
#22562=DIRECTION('',(0.411815896436094,0.476626859392517,-0.776681726544511));
#22563=DIRECTION('center_axis',(-1.04744440165193E-14,-1.15185638804861E-13,
-1.));
#22564=DIRECTION('ref_axis',(-1.,-8.72635297355361E-14,1.04744440165294E-14));
#22565=DIRECTION('center_axis',(-8.48926851182745E-12,-3.34708584909148E-10,
1.));
#22566=DIRECTION('ref_axis',(-0.0249675486418349,-0.999688262167171,-3.34816203926024E-10));
#22567=DIRECTION('',(-0.100909211142278,-0.472292312794079,0.875646790882181));
#22568=DIRECTION('',(-0.0724190381853189,-0.456279544171757,0.886884694015365));
#22569=DIRECTION('center_axis',(-1.04744440165193E-14,-1.15185638804861E-13,
-1.));
#22570=DIRECTION('ref_axis',(-1.,-8.72635297355361E-14,1.04744440165294E-14));
#22571=DIRECTION('center_axis',(-2.29622482795222E-12,-2.87759861733811E-10,
1.));
#22572=DIRECTION('ref_axis',(-0.00756134748309062,-0.9999714126035,-2.8776898705888E-10));
#22573=DIRECTION('',(-0.0127111307240333,-0.450090627151626,0.892892409255433));
#22574=DIRECTION('',(0.0127111306191146,-0.450090672347739,0.892892386474397));
#22575=DIRECTION('center_axis',(-1.04744440165193E-14,-1.15185638804861E-13,
-1.));
#22576=DIRECTION('ref_axis',(-1.,-8.72635297355361E-14,1.04744440165294E-14));
#22577=DIRECTION('center_axis',(-1.69115474723865E-12,1.9183849313996E-10,
1.));
#22578=DIRECTION('ref_axis',(0.0100693168850478,-0.999949303143649,1.91845790211371E-10));
#22579=DIRECTION('',(0.0724190350594109,-0.456279674184686,0.886884627382266));
#22580=DIRECTION('',(0.100909204542893,-0.472292525389385,0.875646676976415));
#22581=DIRECTION('center_axis',(-1.04744440165193E-14,-1.15185638804861E-13,
-1.));
#22582=DIRECTION('ref_axis',(-1.,-8.72635297355361E-14,1.04744440165294E-14));
#22583=DIRECTION('center_axis',(4.60132114045041E-12,-1.67344966178724E-10,
1.));
#22584=DIRECTION('ref_axis',(0.0272919172742142,-0.999627506249952,-1.67408177429198E-10));
#22585=DIRECTION('center_axis',(-1.04744440165193E-14,-1.15185638804861E-13,
-1.));
#22586=DIRECTION('ref_axis',(-1.,-8.72635297355361E-14,1.04744440165294E-14));
#22587=DIRECTION('center_axis',(-0.845914384560533,-0.303272038408841,0.438696848305206));
#22588=DIRECTION('ref_axis',(0.194713288745752,-0.941418664629657,-0.275350019198703));
#22589=DIRECTION('center_axis',(-1.04744440165193E-14,-1.15185638804861E-13,
-1.));
#22590=DIRECTION('ref_axis',(-1.,-8.72635297355361E-14,1.04744440165294E-14));
#22591=DIRECTION('',(0.456351649509837,-0.0724173292173613,0.886847733502586));
#22592=DIRECTION('center_axis',(-1.04744440165193E-14,-1.15185638804861E-13,
-1.));
#22593=DIRECTION('ref_axis',(-1.,-8.72635297355361E-14,1.04744440165294E-14));
#22594=DIRECTION('',(0.450163801758523,-0.0127110352586768,0.892855520881719));
#22595=DIRECTION('',(0.450163801758538,0.0127110352589581,0.892855520881708));
#22596=DIRECTION('center_axis',(-1.04744440165193E-14,-1.15185638804861E-13,
-1.));
#22597=DIRECTION('ref_axis',(-1.,-8.72635297355361E-14,1.04744440165294E-14));
#22598=DIRECTION('',(0.45635164950983,0.0724173292176335,0.886847733502568));
#22599=DIRECTION('',(0.472361792915589,0.100907068159402,0.875609559215204));
#22600=DIRECTION('center_axis',(0.00208426357814304,-0.478871212227244,
0.877882690309671));
#22601=DIRECTION('ref_axis',(0.261186023449167,0.84767244816946,0.461771893654439));
#22602=DIRECTION('center_axis',(1.04744440165193E-14,1.15185638804861E-13,
1.));
#22603=DIRECTION('ref_axis',(1.,8.72635297355361E-14,-1.04744440165294E-14));
#22604=DIRECTION('center_axis',(1.02694929293583E-14,1.15185638804861E-13,
1.));
#22605=DIRECTION('ref_axis',(1.,8.72362563773224E-14,-1.02694929293684E-14));
#22606=DIRECTION('',(0.368107017006031,0.529525460520388,0.764264359166115));
#22607=DIRECTION('',(0.215658660878526,0.571281776348565,0.79191443603467));
#22608=DIRECTION('center_axis',(1.04744440165193E-14,1.15185638804861E-13,
1.));
#22609=DIRECTION('ref_axis',(1.,8.72635297355361E-14,-1.04744440165294E-14));
#22610=DIRECTION('center_axis',(1.02694929293583E-14,1.15185638804861E-13,
1.));
#22611=DIRECTION('ref_axis',(1.,8.72362563773224E-14,-1.02694929293684E-14));
#22612=DIRECTION('',(0.111788425215345,0.585178590638193,0.803162103841168));
#22613=DIRECTION('',(-0.111788300989806,0.585180930864035,0.803160416053302));
#22614=DIRECTION('center_axis',(1.04744440165193E-14,1.15185638804861E-13,
1.));
#22615=DIRECTION('ref_axis',(1.,8.72635297355361E-14,-1.04744440165294E-14));
#22616=DIRECTION('center_axis',(1.02695629360633E-14,1.15185638804861E-13,
1.));
#22617=DIRECTION('ref_axis',(1.,8.72362563773224E-14,-1.02695629360733E-14));
#22618=DIRECTION('',(-0.215658204214253,0.571287278227592,0.791910591348792));
#22619=DIRECTION('',(-0.368105810341799,0.529534956436002,0.764258360965014));
#22620=DIRECTION('center_axis',(1.04744440165193E-14,1.15185638804861E-13,
1.));
#22621=DIRECTION('ref_axis',(1.,8.72635297355361E-14,-1.04744440165294E-14));
#22622=DIRECTION('center_axis',(1.02695629360633E-14,1.15185638804861E-13,
1.));
#22623=DIRECTION('ref_axis',(1.,8.72362563773224E-14,-1.02695629360733E-14));
#22624=DIRECTION('',(0.379787668322238,-0.590832026048182,-0.711813770579185));
#22625=DIRECTION('',(0.476375308922749,-0.412016801957993,-0.77672950243509));
#22626=DIRECTION('center_axis',(-0.000653357528254759,0.000583642099734136,
0.999999616242846));
#22627=DIRECTION('ref_axis',(-0.831134725976919,0.556070422329433,-0.000867574572038));
#22628=DIRECTION('center_axis',(-1.04744440165193E-14,-1.15185638804861E-13,
-1.));
#22629=DIRECTION('ref_axis',(-1.,-8.72635297355361E-14,1.04744440165294E-14));
#22630=DIRECTION('center_axis',(1.04599037721437E-14,1.17366013112296E-13,
1.));
#22631=DIRECTION('ref_axis',(1.,8.72640651830633E-14,-1.0459903772154E-14));
#22632=DIRECTION('center_axis',(-1.04744440165193E-14,-1.15185638804861E-13,
-1.));
#22633=DIRECTION('ref_axis',(-1.,-8.72635297355361E-14,1.04744440165294E-14));
#22634=DIRECTION('center_axis',(1.04599037721437E-14,1.17366013112296E-13,
1.));
#22635=DIRECTION('ref_axis',(1.,8.72640651830633E-14,-1.0459903772154E-14));
#22636=DIRECTION('center_axis',(1.04675235693219E-6,-2.73632311340696E-8,
-0.999999999999452));
#22637=DIRECTION('ref_axis',(0.995602221707021,-0.0936814609778925,1.04471240189441E-6));
#22638=DIRECTION('',(-0.472240244388769,0.100910816440637,0.87567468771509));
#22639=DIRECTION('',(-0.456226081184184,0.0724203048515813,0.886912093892358));
#22640=DIRECTION('center_axis',(-1.04744440165193E-14,-1.15185638804861E-13,
-1.));
#22641=DIRECTION('ref_axis',(-1.,-8.72635297355361E-14,1.04744440165294E-14));
#22642=DIRECTION('center_axis',(1.04599037721437E-14,1.17366013112296E-13,
1.));
#22643=DIRECTION('ref_axis',(1.,8.72640651830633E-14,-1.0459903772154E-14));
#22644=DIRECTION('',(-0.450036916879799,0.0127112008260562,0.892919480590991));
#22645=DIRECTION('',(-0.450037561084516,-0.0127111996490203,0.892919155924311));
#22646=DIRECTION('center_axis',(-1.04744440165193E-14,-1.15185638804861E-13,
-1.));
#22647=DIRECTION('ref_axis',(-1.,-8.72635297355361E-14,1.04744440165294E-14));
#22648=DIRECTION('center_axis',(1.04599037721437E-14,1.17366013112296E-13,
1.));
#22649=DIRECTION('ref_axis',(1.,8.72640651830633E-14,-1.0459903772154E-14));
#22650=DIRECTION('',(-0.456227934233452,-0.0724202606201595,0.886911144296195));
#22651=DIRECTION('',(-0.472243274438807,-0.100910722705367,0.875673064442657));
#22652=DIRECTION('center_axis',(-8.72635297355373E-14,1.,-1.1518563880486E-13));
#22653=DIRECTION('ref_axis',(1.00515054169548E-26,-1.1518563880486E-13,
-1.));
#22654=DIRECTION('',(1.,8.72635297355373E-14,0.));
#22655=DIRECTION('center_axis',(8.72635297355373E-14,-1.,1.1518563880486E-13));
#22656=DIRECTION('ref_axis',(6.05512374515433E-29,-1.1518563880486E-13,
-1.));
#22657=DIRECTION('',(1.00515054169548E-26,-1.1518563880486E-13,-1.));
#22658=DIRECTION('center_axis',(8.72635297355373E-14,-1.,1.1518563880486E-13));
#22659=DIRECTION('ref_axis',(6.05512374515433E-29,-1.1518563880486E-13,
-1.));
#22660=DIRECTION('',(-1.,-8.72635297355373E-14,0.));
#22661=DIRECTION('center_axis',(8.72635297355373E-14,-1.,1.1518563880486E-13));
#22662=DIRECTION('ref_axis',(6.05512374515433E-29,-1.1518563880486E-13,
-1.));
#22663=DIRECTION('',(-1.00515054169548E-26,1.1518563880486E-13,1.));
#22664=DIRECTION('center_axis',(8.72635297355373E-14,-1.,1.1518563880486E-13));
#22665=DIRECTION('ref_axis',(6.05512374515433E-29,-1.1518563880486E-13,
-1.));
#22666=DIRECTION('center_axis',(9.95715680553083E-15,1.12696349603476E-13,
1.));
#22667=DIRECTION('ref_axis',(1.,8.71251220484807E-14,-9.95715680554065E-15));
#22668=DIRECTION('center_axis',(9.95715680553083E-15,1.12696349603476E-13,
1.));
#22669=DIRECTION('ref_axis',(1.,8.71251220484807E-14,-9.95715680554065E-15));
#22670=DIRECTION('',(-0.0174340345131866,-0.000800581691362652,0.999847695156391));
#22671=DIRECTION('',(0.0130759035045374,0.0115588597183791,-0.999847695156393));
#22672=DIRECTION('center_axis',(1.06503951930529E-14,1.15185638804861E-13,
1.));
#22673=DIRECTION('ref_axis',(1.,8.72606242522541E-14,-1.06503951930629E-14));
#22674=DIRECTION('center_axis',(1.06503951930529E-14,1.15185638804861E-13,
1.));
#22675=DIRECTION('ref_axis',(1.,8.72606242522541E-14,-1.06503951930629E-14));
#22676=DIRECTION('',(0.0115565367885269,0.0130779565645496,-0.999847695156393));
#22677=DIRECTION('center_axis',(1.12018012904865E-14,1.15185638804861E-13,
1.));
#22678=DIRECTION('ref_axis',(1.,8.71251211483066E-14,-1.12018012904966E-14));
#22679=DIRECTION('center_axis',(1.12018012904865E-14,1.15185638804861E-13,
1.));
#22680=DIRECTION('ref_axis',(1.,8.71251211483066E-14,-1.12018012904966E-14));
#22681=DIRECTION('',(0.000800462344174388,0.0174340399931744,-0.999847695156393));
#22682=DIRECTION('center_axis',(1.04599037500094E-14,1.15185638804861E-13,
1.));
#22683=DIRECTION('ref_axis',(1.,8.72149721128382E-14,-1.04599037500194E-14));
#22684=DIRECTION('',(-0.000800509149934771,0.0174340378440839,-0.999847695156393));
#22685=DIRECTION('center_axis',(1.04599037500094E-14,1.15185638804861E-13,
1.));
#22686=DIRECTION('ref_axis',(1.,8.72149721128382E-14,-1.04599037500194E-14));
#22687=DIRECTION('center_axis',(1.12018011379709E-14,1.15185638804861E-13,
1.));
#22688=DIRECTION('ref_axis',(1.,8.71251199620744E-14,-1.1201801137981E-14));
#22689=DIRECTION('center_axis',(1.12018011379709E-14,1.15185638804861E-13,
1.));
#22690=DIRECTION('ref_axis',(1.,8.71251199620744E-14,-1.1201801137981E-14));
#22691=DIRECTION('',(-0.0115568680204753,0.0130776638589093,-0.999847695156393));
#22692=DIRECTION('center_axis',(1.06503951254365E-14,1.15185638804861E-13,
1.));
#22693=DIRECTION('ref_axis',(1.,8.72606236982606E-14,-1.06503951254465E-14));
#22694=DIRECTION('center_axis',(1.06503951254365E-14,1.15185638804861E-13,
1.));
#22695=DIRECTION('ref_axis',(1.,8.72606236982606E-14,-1.06503951254465E-14));
#22696=DIRECTION('',(-0.0130765548702522,0.0115581228222826,-0.999847695156392));
#22697=DIRECTION('center_axis',(9.957156389593E-15,1.18919572450962E-13,
1.));
#22698=DIRECTION('ref_axis',(1.,8.71251184090297E-14,-9.95715638960336E-15));
#22699=DIRECTION('center_axis',(9.957156389593E-15,1.18919572450962E-13,
1.));
#22700=DIRECTION('ref_axis',(1.,8.71251184090297E-14,-9.95715638960336E-15));
#22701=DIRECTION('center_axis',(9.95715638959301E-15,1.18919572450962E-13,
1.));
#22702=DIRECTION('ref_axis',(1.,8.72806989776172E-14,-9.95715638960339E-15));
#22703=DIRECTION('center_axis',(9.95715638959301E-15,1.18919572450962E-13,
1.));
#22704=DIRECTION('ref_axis',(1.,8.72806989776172E-14,-9.95715638960339E-15));
#22705=DIRECTION('',(-0.0130765548702503,-0.0115581228225151,-0.99984769515639));
#22706=DIRECTION('center_axis',(1.03276558792108E-14,1.15185638804861E-13,
1.));
#22707=DIRECTION('ref_axis',(1.,8.72606236982606E-14,-1.03276558792209E-14));
#22708=DIRECTION('center_axis',(1.03276558792108E-14,1.15185638804861E-13,
1.));
#22709=DIRECTION('ref_axis',(1.,8.72606236982606E-14,-1.03276558792209E-14));
#22710=DIRECTION('',(-0.0115163028275352,-0.0131134000030443,-0.99984769515639));
#22711=DIRECTION('center_axis',(1.01544784648356E-14,1.16878051882335E-13,
1.));
#22712=DIRECTION('ref_axis',(1.,8.72650493072682E-14,-1.01544784648458E-14));
#22713=DIRECTION('center_axis',(1.01544784648356E-14,1.16878051882335E-13,
1.));
#22714=DIRECTION('ref_axis',(1.,8.72650493072682E-14,-1.01544784648458E-14));
#22715=DIRECTION('center_axis',(1.02695629360633E-14,1.15185638804861E-13,
1.));
#22716=DIRECTION('ref_axis',(1.,8.72912849566231E-14,-1.02695629360733E-14));
#22717=DIRECTION('',(0.00366432240577321,-0.0170633886365656,-0.999847695156389));
#22718=DIRECTION('center_axis',(1.02695629360633E-14,1.15185638804861E-13,
1.));
#22719=DIRECTION('ref_axis',(1.,8.72912849566231E-14,-1.02695629360733E-14));
#22720=DIRECTION('center_axis',(9.30827207959047E-15,1.12647019146788E-13,
1.));
#22721=DIRECTION('ref_axis',(1.,8.72650507462529E-14,-9.3082720796003E-15));
#22722=DIRECTION('center_axis',(9.30827207959047E-15,1.12647019146788E-13,
1.));
#22723=DIRECTION('ref_axis',(1.,8.72650507462529E-14,-9.3082720796003E-15));
#22724=DIRECTION('',(0.0115164418467348,-0.013113277913841,-0.99984769515639));
#22725=DIRECTION('center_axis',(1.03276559454674E-14,1.15185638804861E-13,
1.));
#22726=DIRECTION('ref_axis',(1.,8.7260624258077E-14,-1.03276559454775E-14));
#22727=DIRECTION('center_axis',(1.03276559454674E-14,1.15185638804861E-13,
1.));
#22728=DIRECTION('ref_axis',(1.,8.7260624258077E-14,-1.03276559454775E-14));
#22729=DIRECTION('',(0.0130759007521692,-0.0115588628322128,-0.99984769515639));
#22730=DIRECTION('center_axis',(1.12018014099246E-14,1.11451705001549E-13,
1.));
#22731=DIRECTION('ref_axis',(1.,8.72807026524047E-14,-1.12018014099343E-14));
#22732=DIRECTION('center_axis',(1.12018014099246E-14,1.11451705001549E-13,
1.));
#22733=DIRECTION('ref_axis',(1.,8.72807026524047E-14,-1.12018014099343E-14));
#22734=DIRECTION('',(0.0174340340546429,-0.000800591677104543,-0.999847695156391));
#22735=DIRECTION('center_axis',(1.04599037721437E-14,1.17366013112296E-13,
1.));
#22736=DIRECTION('ref_axis',(-0.999999999999959,2.86379829728456E-7,1.04598701608845E-14));
#22737=DIRECTION('center_axis',(1.04599037721437E-14,1.17366013112296E-13,
1.));
#22738=DIRECTION('ref_axis',(1.,8.72628521386072E-14,-1.0459903772154E-14));
#22739=DIRECTION('center_axis',(-1.00515054169548E-26,1.1518563880486E-13,
1.));
#22740=DIRECTION('ref_axis',(-8.72635297355373E-14,1.,-1.1518563880486E-13));
#22741=DIRECTION('',(8.72635297355373E-14,-1.,1.1518563880486E-13));
#22742=DIRECTION('',(-8.72635297355373E-14,1.,-1.1518563880486E-13));
#22743=DIRECTION('',(-1.,-8.72635297355373E-14,0.));
#22744=DIRECTION('center_axis',(1.,8.72635297355373E-14,0.));
#22745=DIRECTION('ref_axis',(8.72635297355373E-14,-1.,1.1518563880486E-13));
#22746=DIRECTION('',(8.72635297355373E-14,-1.,1.1518563880486E-13));
#22747=DIRECTION('',(-8.72635297355373E-14,1.,-1.1518563880486E-13));
#22748=DIRECTION('',(-1.00515054169548E-26,1.1518563880486E-13,1.));
#22749=DIRECTION('center_axis',(-8.72635297355373E-14,1.,-1.1518563880486E-13));
#22750=DIRECTION('ref_axis',(6.05512374515433E-29,-1.1518563880486E-13,
-1.));
#22751=DIRECTION('center_axis',(-8.72635297355373E-14,1.,-1.1518563880486E-13));
#22752=DIRECTION('ref_axis',(6.05512374515433E-29,-1.1518563880486E-13,
-1.));
#22753=DIRECTION('center_axis',(1.00515054169548E-26,-1.1518563880486E-13,
-1.));
#22754=DIRECTION('ref_axis',(8.72635297355373E-14,-1.,1.1518563880486E-13));
#22755=DIRECTION('',(8.72635297355373E-14,-1.,1.1518563880486E-13));
#22756=DIRECTION('',(-8.72635297355373E-14,1.,-1.1518563880486E-13));
#22757=DIRECTION('',(1.,8.72635297355373E-14,0.));
#22758=DIRECTION('center_axis',(-8.72635297355373E-14,1.,-1.1518563880486E-13));
#22759=DIRECTION('ref_axis',(6.05512374515433E-29,-1.1518563880486E-13,
-1.));
#22760=DIRECTION('center_axis',(-8.72635297355373E-14,1.,-1.1518563880486E-13));
#22761=DIRECTION('ref_axis',(6.05512374515433E-29,-1.1518563880486E-13,
-1.));
#22762=DIRECTION('center_axis',(-8.72635297355373E-14,1.,-1.1518563880486E-13));
#22763=DIRECTION('ref_axis',(6.05512374515433E-29,-1.1518563880486E-13,
-1.));
#22764=DIRECTION('center_axis',(-8.72635297355373E-14,1.,-1.1518563880486E-13));
#22765=DIRECTION('ref_axis',(6.05512374515433E-29,-1.1518563880486E-13,
-1.));
#22766=DIRECTION('',(8.72635297355373E-14,-1.,1.1518563880486E-13));
#22767=DIRECTION('center_axis',(-8.72635297355373E-14,1.,-1.1518563880486E-13));
#22768=DIRECTION('ref_axis',(6.05512374515433E-29,-1.1518563880486E-13,
-1.));
#22769=DIRECTION('',(-8.72635297355373E-14,1.,-1.1518563880486E-13));
#22770=DIRECTION('center_axis',(-8.72635297355373E-14,1.,-1.1518563880486E-13));
#22771=DIRECTION('ref_axis',(6.05512374515433E-29,-1.1518563880486E-13,
-1.));
#22772=DIRECTION('center_axis',(-1.,-8.72635297355373E-14,0.));
#22773=DIRECTION('ref_axis',(-8.72635297355373E-14,1.,-1.1518563880486E-13));
#22774=DIRECTION('',(1.00515054169548E-26,-1.1518563880486E-13,-1.));
#22775=DIRECTION('',(-0.581868005306999,0.0361272616194947,0.812480427682988));
#22776=DIRECTION('center_axis',(-0.706995946343866,-0.707002335908082,-0.0174478902408474));
#22777=DIRECTION('ref_axis',(-0.485490346420283,0.503130085971089,-0.714954012593424));
#22778=DIRECTION('center_axis',(1.01785891439412E-10,1.01653359675599E-10,
-1.));
#22779=DIRECTION('ref_axis',(-0.707106780085371,0.707106782287724,-9.37138848923848E-14));
#22780=DIRECTION('',(0.0361272616297709,-0.581868005321186,0.81248042767237));
#22781=DIRECTION('center_axis',(-0.707002336415719,-0.70699594584904,-0.0174478897215777));
#22782=DIRECTION('ref_axis',(0.514376723468753,-0.497136627511086,-0.698764452401848));
#22783=DIRECTION('',(0.0361272616182702,0.581868005288873,-0.812480427696024));
#22784=DIRECTION('center_axis',(-0.707002329658505,0.706995952382432,0.0174478987934091));
#22785=DIRECTION('ref_axis',(-0.514376732675718,-0.497136618246221,-0.698764452215883));
#22786=DIRECTION('',(-0.581868005317437,-0.0361272616345021,-0.812480427674845));
#22787=DIRECTION('center_axis',(-4.27803755150032E-11,4.26274542481757E-11,
-1.));
#22788=DIRECTION('ref_axis',(0.707106783659767,0.707106778713328,-1.08131875993609E-13));
#22789=DIRECTION('center_axis',(0.706995945311992,-0.707002336973518,-0.0174478888805456));
#22790=DIRECTION('ref_axis',(0.497136628295254,0.514376722639527,-0.698764452454363));
#22791=DIRECTION('',(-0.58186800529869,0.0361272616310885,-0.812480427688423));
#22792=DIRECTION('center_axis',(-0.706984234058496,-0.707014463525137,0.0174310401004826));
#22793=DIRECTION('ref_axis',(0.497157132168199,-0.514363398390198,-0.698759672799438));
#22794=DIRECTION('',(0.0361272616460507,-0.581868005335907,-0.812480427661104));
#22795=DIRECTION('center_axis',(8.98778795138279E-11,8.97351529997424E-11,
-1.));
#22796=DIRECTION('ref_axis',(-0.707106777512622,0.707106784860473,-1.00922226080033E-13));
#22797=DIRECTION('center_axis',(-4.3591368164562E-11,-5.61674536871897E-11,
-1.));
#22798=DIRECTION('ref_axis',(0.78941644366153,-0.613858027948469,6.70995244962243E-14));
#22799=DIRECTION('center_axis',(0.707006995355329,0.706991448016083,-0.0174413574801738));
#22800=DIRECTION('ref_axis',(-0.513636500710189,0.496382763560557,-0.699844052041721));
#22801=DIRECTION('center_axis',(1.99622914093862E-10,-2.721998042675E-10,
-1.));
#22802=DIRECTION('ref_axis',(0.789416439455461,0.613858033357439,-9.50642645022728E-12));
#22803=DIRECTION('',(0.0361272616208185,0.581868005208879,0.812480427753199));
#22804=DIRECTION('center_axis',(-0.707006955053561,0.706991486952665,-0.0174414128542213));
#22805=DIRECTION('ref_axis',(0.501153812357023,0.483458857880451,-0.717713305642965));
#22806=DIRECTION('center_axis',(2.27115393216186E-10,-2.14586044118155E-10,
-1.));
#22807=DIRECTION('ref_axis',(0.707106783402892,0.707106778970203,8.85958869003344E-12));
#22808=DIRECTION('',(-0.581868005296781,-0.0361272616296084,0.812480427689856));
#22809=DIRECTION('center_axis',(-0.706995952053428,0.70700232999654,-0.0174478984273346));
#22810=DIRECTION('ref_axis',(-0.497136618691357,-0.514376732281121,-0.698764452189664));
#22811=DIRECTION('center_axis',(-1.04744440165193E-14,-1.15185638804861E-13,
-1.));
#22812=DIRECTION('ref_axis',(-1.,-8.72635297355361E-14,1.04744440165294E-14));
#22813=DIRECTION('center_axis',(1.20840226997713E-14,1.16284186323023E-13,
1.));
#22814=DIRECTION('ref_axis',(1.,8.73461657600799E-14,-1.20840226997814E-14));
#22815=DIRECTION('center_axis',(1.09854751816067E-14,1.15185638804861E-13,
1.));
#22816=DIRECTION('ref_axis',(1.,8.73461657600583E-14,-1.09854751816168E-14));
#22817=DIRECTION('center_axis',(1.04854396770053E-14,1.15185638804861E-13,
1.));
#22818=DIRECTION('ref_axis',(1.,8.72173693231828E-14,-1.04854396770154E-14));
#22819=DIRECTION('center_axis',(1.09854751816067E-14,1.15185638804861E-13,
1.));
#22820=DIRECTION('ref_axis',(1.,8.73461657600581E-14,-1.09854751816168E-14));
#22821=DIRECTION('center_axis',(9.88692766344469E-15,1.18481281359346E-13,
1.));
#22822=DIRECTION('ref_axis',(1.,8.73461657600578E-14,-9.88692766345504E-15));
#22823=DIRECTION('center_axis',(1.04854396770055E-14,1.1301218632279E-13,
1.));
#22824=DIRECTION('ref_axis',(1.,8.72632848014737E-14,-1.04854396770154E-14));
#22825=DIRECTION('center_axis',(1.09854751816069E-14,1.14087091286699E-13,
1.));
#22826=DIRECTION('ref_axis',(1.,8.72061879303152E-14,-1.09854751816168E-14));
#22827=DIRECTION('center_axis',(1.03092138003362E-14,1.18357704589583E-13,
1.));
#22828=DIRECTION('ref_axis',(1.,8.72387369821193E-14,-1.03092138003465E-14));
#22829=DIRECTION('center_axis',(1.06396373193144E-14,1.15185638804861E-13,
1.));
#22830=DIRECTION('ref_axis',(1.,8.72773155181867E-14,-1.06396373193244E-14));
#22831=DIRECTION('center_axis',(1.03092138003367E-14,1.135996059125E-13,
1.));
#22832=DIRECTION('ref_axis',(1.,8.72387369821196E-14,-1.03092138003466E-14));
#22833=DIRECTION('center_axis',(9.88692766344536E-15,1.12988543768537E-13,
1.));
#22834=DIRECTION('ref_axis',(1.,8.72061879303152E-14,-9.88692766345521E-15));
#22835=DIRECTION('center_axis',(8.72635297355373E-14,-1.,1.1518563880486E-13));
#22836=DIRECTION('ref_axis',(-1.00515054169548E-26,1.1518563880486E-13,
1.));
#22837=DIRECTION('',(0.499999999980758,-5.61219244913375E-14,-0.866025403795548));
#22838=DIRECTION('',(-0.499999999980758,-1.43385454223517E-13,-0.866025403795548));
#22839=DIRECTION('',(-1.,-8.72635297355373E-14,0.));
#22840=DIRECTION('',(-0.499999999980758,5.61219244913375E-14,0.866025403795548));
#22841=DIRECTION('',(0.499999999980758,1.43385454223517E-13,0.866025403795548));
#22842=DIRECTION('',(1.,8.72635297355373E-14,0.));
#22843=DIRECTION('center_axis',(8.72635297355373E-14,-1.,1.1518563880486E-13));
#22844=DIRECTION('ref_axis',(-1.00515054169548E-26,1.1518563880486E-13,
1.));
#22845=DIRECTION('',(0.499999999980758,-5.61219244913375E-14,-0.866025403795548));
#22846=DIRECTION('',(-0.499999999980758,-1.43385454223517E-13,-0.866025403795548));
#22847=DIRECTION('',(-1.,-8.72635297355373E-14,0.));
#22848=DIRECTION('',(-0.499999999980758,5.61219244913375E-14,0.866025403795548));
#22849=DIRECTION('',(0.499999999980758,1.43385454223517E-13,0.866025403795548));
#22850=DIRECTION('',(1.,8.72635297355373E-14,0.));
#22851=DIRECTION('center_axis',(1.,8.72635297355373E-14,0.));
#22852=DIRECTION('ref_axis',(8.72635297355373E-14,-1.,1.11022302462516E-13));
#22853=DIRECTION('',(1.,8.72635297355373E-14,0.));
#22854=DIRECTION('center_axis',(-1.00515054169548E-26,1.1518563880486E-13,
1.));
#22855=DIRECTION('ref_axis',(-9.02056207507939E-14,1.,-1.1518563880486E-13));
#22856=DIRECTION('',(1.00515054169548E-26,-1.1518563880486E-13,-1.));
#22857=DIRECTION('center_axis',(1.,8.72635297355373E-14,0.));
#22858=DIRECTION('ref_axis',(8.72635297355373E-14,-1.,1.11022302462516E-13));
#22859=DIRECTION('',(-1.,-8.72635297355373E-14,0.));
#22860=DIRECTION('center_axis',(-1.00515054169548E-26,1.1518563880486E-13,
1.));
#22861=DIRECTION('ref_axis',(-9.02056207507939E-14,1.,-1.1518563880486E-13));
#22862=DIRECTION('',(-1.00515054169548E-26,1.1518563880486E-13,1.));
#22863=DIRECTION('center_axis',(9.88692766344469E-15,1.18481281359346E-13,
1.));
#22864=DIRECTION('ref_axis',(1.,8.73345276938528E-14,-9.88692766345504E-15));
#22865=DIRECTION('center_axis',(9.88692766344469E-15,1.18481281359346E-13,
1.));
#22866=DIRECTION('ref_axis',(1.,8.73345276938528E-14,-9.88692766345504E-15));
#22867=DIRECTION('',(-0.0174340297464267,-0.000800685488963285,0.999847695156391));
#22868=DIRECTION('center_axis',(-0.998896061698716,0.0436127439212717,-0.0174524064372782));
#22869=DIRECTION('ref_axis',(0.0436193873652447,0.999048221581862,-1.1507597159015E-13));
#22870=DIRECTION('',(0.0177702355175903,0.00691046665269606,-0.999818215567356));
#22871=DIRECTION('',(-0.0436193873652537,-0.999048221581861,1.15076007599765E-13));
#22872=DIRECTION('center_axis',(-0.706999085398757,-0.706999085398894,-0.0174524064371947));
#22873=DIRECTION('ref_axis',(-0.707106781186615,0.70710678118648,-8.14490323933116E-14));
#22874=DIRECTION('',(0.00691046665279671,0.0177702355174836,-0.999818215567357));
#22875=DIRECTION('',(0.707106781186617,-0.707106781186478,7.26836276787581E-14));
#22876=DIRECTION('center_axis',(0.043612743921459,-0.99889606169871,-0.017452406437169));
#22877=DIRECTION('ref_axis',(-0.999048221581854,-0.04361938736543,5.02432903970128E-15));
#22878=DIRECTION('',(0.999048221581854,0.0436193873654325,-1.79912716949635E-14));
#22879=DIRECTION('center_axis',(1.09854751816067E-14,1.15185638804861E-13,
1.));
#22880=DIRECTION('ref_axis',(1.,8.73345276938534E-14,-1.09854751816168E-14));
#22881=DIRECTION('center_axis',(1.09854751816067E-14,1.15185638804861E-13,
1.));
#22882=DIRECTION('ref_axis',(1.,8.73345276938534E-14,-1.09854751816168E-14));
#22883=DIRECTION('',(0.000800685489064943,0.0174340297463221,-0.999847695156393));
#22884=DIRECTION('center_axis',(1.04854396770053E-14,1.15185638804861E-13,
1.));
#22885=DIRECTION('ref_axis',(1.,8.72905510366657E-14,-1.04854396770154E-14));
#22886=DIRECTION('',(-0.000800685489088981,0.017434029746322,-0.999847695156393));
#22887=DIRECTION('center_axis',(1.04854396770053E-14,1.15185638804861E-13,
1.));
#22888=DIRECTION('ref_axis',(1.,8.72905510366657E-14,-1.04854396770154E-14));
#22889=DIRECTION('center_axis',(1.09854751816067E-14,1.15185638804861E-13,
1.));
#22890=DIRECTION('ref_axis',(1.,8.73345276938534E-14,-1.09854751816168E-14));
#22891=DIRECTION('center_axis',(1.09854751816067E-14,1.15185638804861E-13,
1.));
#22892=DIRECTION('ref_axis',(1.,8.73345276938534E-14,-1.09854751816168E-14));
#22893=DIRECTION('center_axis',(-0.0436127439212822,-0.998896061698718,
-0.017452406437168));
#22894=DIRECTION('ref_axis',(-0.999048221581861,0.0436193873652532,-5.02437150627773E-15));
#22895=DIRECTION('',(-0.00691046665282191,0.0177702355174846,-0.999818215567357));
#22896=DIRECTION('',(0.999048221581861,-0.0436193873652517,-7.94261769905107E-15));
#22897=DIRECTION('center_axis',(0.706999085398879,-0.706999085398772,-0.0174524064372095));
#22898=DIRECTION('ref_axis',(-0.707106781186493,-0.707106781186602,8.14494986888246E-14));
#22899=DIRECTION('',(-0.0177702355176088,0.00691046665269189,-0.999818215567355));
#22900=DIRECTION('',(0.707106781186494,0.707106781186601,-9.02134649096816E-14));
#22901=DIRECTION('center_axis',(0.998896061698708,0.0436127439214494,-0.017452406437299));
#22902=DIRECTION('ref_axis',(0.0436193873654224,-0.999048221581854,1.15076006713017E-13));
#22903=DIRECTION('',(-0.0436193873654263,0.999048221581854,-1.15076007599766E-13));
#22904=DIRECTION('center_axis',(1.20840226997713E-14,1.16284186323023E-13,
1.));
#22905=DIRECTION('ref_axis',(1.,8.73345276938747E-14,-1.20840226997814E-14));
#22906=DIRECTION('center_axis',(1.20840226997713E-14,1.16284186323023E-13,
1.));
#22907=DIRECTION('ref_axis',(1.,8.73345276938747E-14,-1.20840226997814E-14));
#22908=DIRECTION('center_axis',(9.88692766344536E-15,1.12988543768537E-13,
1.));
#22909=DIRECTION('ref_axis',(1.,8.71972092540841E-14,-9.88692766345521E-15));
#22910=DIRECTION('center_axis',(9.88692766344536E-15,1.12988543768537E-13,
1.));
#22911=DIRECTION('ref_axis',(1.,8.71972092540841E-14,-9.88692766345521E-15));
#22912=DIRECTION('center_axis',(0.99888282418075,-0.0439169962041995,-0.0174470914793711));
#22913=DIRECTION('ref_axis',(-0.0439236819193947,-0.999034889364052,1.15074518868834E-13));
#22914=DIRECTION('',(-0.0177673819895374,-0.00691332094576837,-0.999818246548211));
#22915=DIRECTION('',(0.043923681919403,0.999034889364052,-1.1507447191974E-13));
#22916=DIRECTION('center_axis',(0.706999085398756,0.706999085398891,-0.0174524064373725));
#22917=DIRECTION('ref_axis',(0.707106781186616,-0.707106781186479,8.14482412682667E-14));
#22918=DIRECTION('',(-0.00691046665282119,-0.0177702355177138,-0.999818215567353));
#22919=DIRECTION('',(-0.707106781186614,0.707106781186481,-7.26836276787585E-14));
#22920=DIRECTION('center_axis',(-0.043612743921454,0.998896061698706,-0.0174524064373982));
#22921=DIRECTION('ref_axis',(0.999048221581854,0.043619387365425,-5.02429633897994E-15));
#22922=DIRECTION('',(-0.999048221581854,-0.0436193873654181,1.37629650946532E-14));
#22923=DIRECTION('center_axis',(1.03092138003367E-14,1.135996059125E-13,
1.));
#22924=DIRECTION('ref_axis',(1.,8.7231809079856E-14,-1.03092138003466E-14));
#22925=DIRECTION('center_axis',(1.03092138003367E-14,1.135996059125E-13,
1.));
#22926=DIRECTION('ref_axis',(1.,8.7231809079856E-14,-1.03092138003466E-14));
#22927=DIRECTION('',(-0.00411922378064456,-0.0169593185565058,-0.999847695156389));
#22928=DIRECTION('center_axis',(1.06396373193144E-14,1.15185638804861E-13,
1.));
#22929=DIRECTION('ref_axis',(1.,8.7275865546922E-14,-1.06396373193244E-14));
#22930=DIRECTION('',(0.00411922378062659,-0.0169593185565051,-0.999847695156389));
#22931=DIRECTION('center_axis',(1.06396373193144E-14,1.15185638804861E-13,
1.));
#22932=DIRECTION('ref_axis',(1.,8.7275865546922E-14,-1.06396373193244E-14));
#22933=DIRECTION('center_axis',(1.03092138003362E-14,1.18357704589583E-13,
1.));
#22934=DIRECTION('ref_axis',(1.,8.72318090798554E-14,-1.03092138003465E-14));
#22935=DIRECTION('center_axis',(1.03092138003362E-14,1.18357704589583E-13,
1.));
#22936=DIRECTION('ref_axis',(1.,8.72318090798554E-14,-1.03092138003465E-14));
#22937=DIRECTION('center_axis',(0.0436127439212838,0.998896061698714,-0.0174524064373991));
#22938=DIRECTION('ref_axis',(0.999048221581861,-0.0436193873652548,5.0243115308101E-15));
#22939=DIRECTION('',(0.00691046665280434,-0.0177702355177117,-0.999818215567353));
#22940=DIRECTION('',(-0.999048221581863,0.0436193873652139,3.71431109875224E-15));
#22941=DIRECTION('center_axis',(-0.706999085398881,0.706999085398766,-0.0174524064373575));
#22942=DIRECTION('ref_axis',(0.707106781186491,0.707106781186604,-8.14480637193561E-14));
#22943=DIRECTION('',(0.0177702355175879,-0.00691046665292151,-0.999818215567354));
#22944=DIRECTION('',(-0.707106781186494,-0.707106781186601,9.02134649096816E-14));
#22945=DIRECTION('center_axis',(-0.998896061698709,-0.0436127439214501,
-0.0174524064372681));
#22946=DIRECTION('ref_axis',(-0.0436193873654191,0.999048221581854,-1.15076106866482E-13));
#22947=DIRECTION('',(0.0436193873654296,-0.999048221581854,1.15076007599765E-13));
#22948=DIRECTION('center_axis',(1.09854751816069E-14,1.14087091286699E-13,
1.));
#22949=DIRECTION('ref_axis',(1.,8.71972092540835E-14,-1.09854751816168E-14));
#22950=DIRECTION('center_axis',(1.09854751816069E-14,1.14087091286699E-13,
1.));
#22951=DIRECTION('ref_axis',(1.,8.71972092540835E-14,-1.09854751816168E-14));
#22952=DIRECTION('',(0.0174340297464268,-0.000800685489190584,-0.999847695156391));
#22953=DIRECTION('center_axis',(1.04854396770055E-14,1.1301218632279E-13,
1.));
#22954=DIRECTION('ref_axis',(-1.,-8.71405510634815E-14,1.04854396770154E-14));
#22955=DIRECTION('center_axis',(1.04854396770055E-14,1.1301218632279E-13,
1.));
#22956=DIRECTION('ref_axis',(1.,8.72630157433963E-14,-1.04854396770154E-14));
#22957=DIRECTION('center_axis',(-1.00515054169548E-26,1.1518563880486E-13,
1.));
#22958=DIRECTION('ref_axis',(-8.72635297355373E-14,1.,-1.1518563880486E-13));
#22959=DIRECTION('',(8.72635297355373E-14,-1.,1.1518563880486E-13));
#22960=DIRECTION('',(-8.72635297355373E-14,1.,-1.1518563880486E-13));
#22961=DIRECTION('',(-1.,-8.72635297355373E-14,0.));
#22962=DIRECTION('center_axis',(-0.866025403795548,-1.79796141756299E-14,
0.499999999980758));
#22963=DIRECTION('ref_axis',(0.499999999980758,1.43385454223517E-13,0.866025403795548));
#22964=DIRECTION('',(-8.72635297355373E-14,1.,-1.1518563880486E-13));
#22965=DIRECTION('',(-0.499999999980757,-1.43385454223517E-13,-0.866025403795548));
#22966=DIRECTION('center_axis',(-0.866025403795548,-1.33165252976057E-13,
-0.499999999980758));
#22967=DIRECTION('ref_axis',(-0.499999999980758,5.61219244913375E-14,0.866025403795548));
#22968=DIRECTION('',(-8.72635297355373E-14,1.,-1.1518563880486E-13));
#22969=DIRECTION('',(0.499999999980757,-5.61219244913376E-14,-0.866025403795548));
#22970=DIRECTION('center_axis',(1.00515054169548E-26,-1.1518563880486E-13,
-1.));
#22971=DIRECTION('ref_axis',(8.72635297355373E-14,-1.,1.1518563880486E-13));
#22972=DIRECTION('',(-8.72635297355373E-14,1.,-1.1518563880486E-13));
#22973=DIRECTION('',(1.,8.72635297355373E-14,0.));
#22974=DIRECTION('center_axis',(0.866025403795548,1.79796141756299E-14,
-0.499999999980758));
#22975=DIRECTION('ref_axis',(-0.499999999980758,-1.43385454223517E-13,-0.866025403795548));
#22976=DIRECTION('',(-8.72635297355373E-14,1.,-1.1518563880486E-13));
#22977=DIRECTION('',(0.499999999980757,1.43385454223517E-13,0.866025403795548));
#22978=DIRECTION('center_axis',(0.866025403795548,1.33165252976057E-13,
0.499999999980758));
#22979=DIRECTION('ref_axis',(0.499999999980758,-5.61219244913375E-14,-0.866025403795548));
#22980=DIRECTION('',(-0.499999999980757,5.61219244913376E-14,0.866025403795548));
#22981=DIRECTION('center_axis',(-1.00515054169548E-26,1.1518563880486E-13,
1.));
#22982=DIRECTION('ref_axis',(-8.72635297355373E-14,1.,-1.1518563880486E-13));
#22983=DIRECTION('',(8.72635297355373E-14,-1.,1.1518563880486E-13));
#22984=DIRECTION('',(-8.72635297355373E-14,1.,-1.1518563880486E-13));
#22985=DIRECTION('',(-1.,-8.72635297355373E-14,0.));
#22986=DIRECTION('center_axis',(-0.866025403795548,-1.79796141756299E-14,
0.499999999980758));
#22987=DIRECTION('ref_axis',(0.499999999980758,1.43385454223517E-13,0.866025403795548));
#22988=DIRECTION('',(-8.72635297355373E-14,1.,-1.1518563880486E-13));
#22989=DIRECTION('',(-0.499999999980758,-1.43385454223516E-13,-0.866025403795548));
#22990=DIRECTION('center_axis',(-0.866025403795548,-1.33165252976057E-13,
-0.499999999980758));
#22991=DIRECTION('ref_axis',(-0.499999999980758,5.61219244913375E-14,0.866025403795548));
#22992=DIRECTION('',(-8.72635297355373E-14,1.,-1.1518563880486E-13));
#22993=DIRECTION('',(0.499999999980758,-5.61219244913375E-14,-0.866025403795548));
#22994=DIRECTION('center_axis',(1.00515054169548E-26,-1.1518563880486E-13,
-1.));
#22995=DIRECTION('ref_axis',(8.72635297355373E-14,-1.,1.1518563880486E-13));
#22996=DIRECTION('',(-8.72635297355373E-14,1.,-1.1518563880486E-13));
#22997=DIRECTION('',(1.,8.72635297355373E-14,0.));
#22998=DIRECTION('center_axis',(0.866025403795548,1.79796141756299E-14,
-0.499999999980758));
#22999=DIRECTION('ref_axis',(-0.499999999980758,-1.43385454223517E-13,-0.866025403795548));
#23000=DIRECTION('',(-8.72635297355373E-14,1.,-1.1518563880486E-13));
#23001=DIRECTION('',(0.499999999980757,1.43385454223517E-13,0.866025403795548));
#23002=DIRECTION('center_axis',(0.866025403795548,1.33165252976057E-13,
0.499999999980758));
#23003=DIRECTION('ref_axis',(0.499999999980758,-5.61219244913375E-14,-0.866025403795548));
#23004=DIRECTION('',(-0.499999999980757,5.61219244913376E-14,0.866025403795548));
#23005=DIRECTION('center_axis',(1.00515054169548E-26,-1.1518563880486E-13,
-1.));
#23006=DIRECTION('ref_axis',(8.72635297355373E-14,-1.,1.1518563880486E-13));
#23007=DIRECTION('center_axis',(1.00515054169548E-26,-1.1518563880486E-13,
-1.));
#23008=DIRECTION('ref_axis',(8.72635297355373E-14,-1.,1.1518563880486E-13));
#23009=DIRECTION('',(1.00515054169548E-26,-1.1518563880486E-13,-1.));
#23010=DIRECTION('center_axis',(1.00515054169548E-26,-1.1518563880486E-13,
-1.));
#23011=DIRECTION('ref_axis',(8.72635297355373E-14,-1.,1.1518563880486E-13));
#23012=DIRECTION('',(-1.00515054169548E-26,1.1518563880486E-13,1.));
#23013=DIRECTION('center_axis',(1.00515054169548E-26,-1.1518563880486E-13,
-1.));
#23014=DIRECTION('ref_axis',(8.72635297355373E-14,-1.,1.1518563880486E-13));
#23015=DIRECTION('center_axis',(1.00515054169548E-26,-1.1518563880486E-13,
-1.));
#23016=DIRECTION('ref_axis',(8.72635297355373E-14,-1.,1.1518563880486E-13));
#23017=DIRECTION('',(-1.00515054169548E-26,1.1518563880486E-13,1.));
#23018=DIRECTION('center_axis',(1.00515054169548E-26,-1.1518563880486E-13,
-1.));
#23019=DIRECTION('ref_axis',(8.72635297355373E-14,-1.,1.1518563880486E-13));
#23020=DIRECTION('',(1.00515054169548E-26,-1.1518563880486E-13,-1.));
#23021=DIRECTION('center_axis',(-8.72635297355373E-14,1.,-1.1518563880486E-13));
#23022=DIRECTION('ref_axis',(1.00515054169548E-26,-1.1518563880486E-13,
-1.));
#23023=DIRECTION('',(1.00515054169548E-26,-1.1518563880486E-13,-1.));
#23024=DIRECTION('',(-1.,-8.72635297355373E-14,0.));
#23025=DIRECTION('',(-8.97974505221575E-16,1.1518563880486E-13,1.));
#23026=DIRECTION('',(1.,8.72635297355374E-14,6.53072367426562E-16));
#23027=DIRECTION('center_axis',(-1.00515054169548E-26,1.1518563880486E-13,
1.));
#23028=DIRECTION('ref_axis',(-8.72635297355373E-14,1.,-1.1518563880486E-13));
#23029=DIRECTION('',(0.997564050259831,-0.0697564737440288,8.03494398899043E-15));
#23030=DIRECTION('center_axis',(1.00515054169548E-26,-1.1518563880486E-13,
-1.));
#23031=DIRECTION('ref_axis',(8.72635297355373E-14,-1.,1.1518563880486E-13));
#23032=DIRECTION('',(0.997564050259819,0.069756473744203,-8.03494398899043E-15));
#23033=DIRECTION('',(-8.72635297355373E-14,1.,-1.1518563880486E-13));
#23034=DIRECTION('',(8.72635297355373E-14,-1.,1.1518563880486E-13));
#23035=DIRECTION('center_axis',(1.00515054169548E-26,-1.1518563880486E-13,
-1.));
#23036=DIRECTION('ref_axis',(-8.7385994415452E-14,1.,-1.1518563880486E-13));
#23037=DIRECTION('',(1.00515054169548E-26,-1.1518563880486E-13,-1.));
#23038=DIRECTION('',(-1.00515054169548E-26,1.1518563880486E-13,1.));
#23039=DIRECTION('center_axis',(1.00515054169548E-26,-1.1518563880486E-13,
-1.));
#23040=DIRECTION('ref_axis',(8.72635297355373E-14,-1.,1.1518563880486E-13));
#23041=DIRECTION('center_axis',(1.00515054169548E-26,-1.1518563880486E-13,
-1.));
#23042=DIRECTION('ref_axis',(8.72635297355373E-14,-1.,1.1518563880486E-13));
#23043=DIRECTION('center_axis',(1.00515054169548E-26,-1.1518563880486E-13,
-1.));
#23044=DIRECTION('ref_axis',(8.72635297355373E-14,-1.,1.1518563880486E-13));
#23045=DIRECTION('',(-1.00515054169548E-26,1.1518563880486E-13,1.));
#23046=DIRECTION('center_axis',(1.00515054169548E-26,-1.1518563880486E-13,
-1.));
#23047=DIRECTION('ref_axis',(8.72635297355373E-14,-1.,1.1518563880486E-13));
#23048=DIRECTION('',(1.00515054169548E-26,-1.1518563880486E-13,-1.));
#23049=DIRECTION('center_axis',(1.00515054169548E-26,-1.1518563880486E-13,
-1.));
#23050=DIRECTION('ref_axis',(8.72635297355373E-14,-1.,1.1518563880486E-13));
#23051=DIRECTION('center_axis',(1.00515054169548E-26,-1.1518563880486E-13,
-1.));
#23052=DIRECTION('ref_axis',(8.72635297355373E-14,-1.,1.1518563880486E-13));
#23053=DIRECTION('',(1.00515054169548E-26,-1.1518563880486E-13,-1.));
#23054=DIRECTION('center_axis',(1.00515054169548E-26,-1.1518563880486E-13,
-1.));
#23055=DIRECTION('ref_axis',(8.72635297355373E-14,-1.,1.1518563880486E-13));
#23056=DIRECTION('',(-1.00515054169548E-26,1.1518563880486E-13,1.));
#23057=DIRECTION('center_axis',(1.00515054169548E-26,-1.1518563880486E-13,
-1.));
#23058=DIRECTION('ref_axis',(8.72635297355373E-14,-1.,1.1518563880486E-13));
#23059=DIRECTION('center_axis',(1.00515054169548E-26,-1.1518563880486E-13,
-1.));
#23060=DIRECTION('ref_axis',(8.72635297355373E-14,-1.,1.1518563880486E-13));
#23061=DIRECTION('',(-1.00515054169548E-26,1.1518563880486E-13,1.));
#23062=DIRECTION('center_axis',(1.00515054169548E-26,-1.1518563880486E-13,
-1.));
#23063=DIRECTION('ref_axis',(8.72635297355373E-14,-1.,1.1518563880486E-13));
#23064=DIRECTION('',(1.00515054169548E-26,-1.1518563880486E-13,-1.));
#23065=DIRECTION('center_axis',(1.04744440165193E-14,1.15185638804861E-13,
1.));
#23066=DIRECTION('ref_axis',(1.,8.72635297355361E-14,-1.04744440165294E-14));
#23067=DIRECTION('',(0.0697564737442121,-0.997564050259818,1.14905052377941E-13));
#23068=DIRECTION('',(-0.0697564737440384,-0.99756405025983,1.14905052377941E-13));
#23069=DIRECTION('',(-0.997564050259819,-0.069756473744203,8.03494398899043E-15));
#23070=DIRECTION('',(-0.997564050259831,0.0697564737440288,-8.03494398899043E-15));
#23071=DIRECTION('',(-0.069756473744214,0.997564050259818,-1.14905052377941E-13));
#23072=DIRECTION('',(0.0697564737440366,0.997564050259831,-1.14905052377941E-13));
#23073=DIRECTION('center_axis',(-1.00515054169548E-26,1.1518563880486E-13,
1.));
#23074=DIRECTION('ref_axis',(8.72635297355373E-14,-1.,1.1518563880486E-13));
#23075=DIRECTION('',(0.997564050259819,0.0697564737442016,-8.03494398899027E-15));
#23076=DIRECTION('',(0.997564050259831,-0.0697564737440285,8.03494398899039E-15));
#23077=DIRECTION('center_axis',(1.00515054169548E-26,-1.1518563880486E-13,
-1.));
#23078=DIRECTION('ref_axis',(8.72635297355373E-14,-1.,1.1518563880486E-13));
#23079=DIRECTION('center_axis',(1.00515054169548E-26,-1.1518563880486E-13,
-1.));
#23080=DIRECTION('ref_axis',(8.72635297355373E-14,-1.,1.1518563880486E-13));
#23081=DIRECTION('',(-1.00515054169548E-26,1.1518563880486E-13,1.));
#23082=DIRECTION('',(1.00515054169548E-26,-1.1518563880486E-13,-1.));
#23083=DIRECTION('center_axis',(-8.72635297355373E-14,1.,-1.1518563880486E-13));
#23084=DIRECTION('ref_axis',(1.00515054169548E-26,-1.1518563880486E-13,
-1.));
#23085=DIRECTION('center_axis',(-8.72635297355373E-14,1.,-1.1518563880486E-13));
#23086=DIRECTION('ref_axis',(1.00515054169548E-26,-1.1518563880486E-13,
-1.));
#23087=DIRECTION('center_axis',(0.997564050259831,-0.0697564737440366,8.03494398899132E-15));
#23088=DIRECTION('ref_axis',(-0.0697564737440366,-0.997564050259831,1.14905052377941E-13));
#23089=DIRECTION('',(-0.0697564737440395,-0.99756405025983,1.14905052377941E-13));
#23090=DIRECTION('',(-1.00515054169548E-26,1.1518563880486E-13,1.));
#23091=DIRECTION('',(-0.069756473744048,-0.99756405025983,1.14905052377941E-13));
#23092=DIRECTION('center_axis',(0.997564050259818,0.069756473744214,-8.0349439889917E-15));
#23093=DIRECTION('ref_axis',(0.069756473744214,-0.997564050259818,1.14905052377941E-13));
#23094=DIRECTION('',(0.0697564737442205,-0.997564050259818,1.14905052377941E-13));
#23095=DIRECTION('',(1.00515054169548E-26,-1.1518563880486E-13,-1.));
#23096=DIRECTION('',(0.069756473744213,-0.997564050259818,1.14905052377941E-13));
#23097=DIRECTION('center_axis',(-1.00515054169548E-26,1.1518563880486E-13,
1.));
#23098=DIRECTION('ref_axis',(-8.72635297355373E-14,1.,-1.1518563880486E-13));
#23099=DIRECTION('',(1.,8.67672446588636E-14,5.71649135859831E-29));
#23100=DIRECTION('center_axis',(-1.00515054169548E-26,1.1518563880486E-13,
1.));
#23101=DIRECTION('ref_axis',(-8.67361737988403E-14,1.,-1.1518563880486E-13));
#23102=DIRECTION('',(0.374606593415996,-0.927183854566754,1.06798264577828E-13));
#23103=DIRECTION('',(8.72635297355373E-14,-1.,1.1518563880486E-13));
#23104=DIRECTION('',(-0.374606593415834,-0.927183854566819,1.06798264577828E-13));
#23105=DIRECTION('center_axis',(-1.00515054169548E-26,1.1518563880486E-13,
1.));
#23106=DIRECTION('ref_axis',(-8.67361737988403E-14,1.,-1.1518563880486E-13));
#23107=DIRECTION('',(-1.,-8.7759814812211E-14,5.71649135859831E-29));
#23108=DIRECTION('center_axis',(-1.00515054169548E-26,1.1518563880486E-13,
1.));
#23109=DIRECTION('ref_axis',(-8.74300631892311E-14,1.,-1.1518563880486E-13));
#23110=DIRECTION('',(-1.00515054169548E-26,1.1518563880486E-13,1.));
#23111=DIRECTION('center_axis',(1.00515054169548E-26,-1.1518563880486E-13,
-1.));
#23112=DIRECTION('ref_axis',(-8.60422844084497E-14,1.,-1.1518563880486E-13));
#23113=DIRECTION('',(1.00515054169548E-26,-1.1518563880486E-13,-1.));
#23114=DIRECTION('center_axis',(1.00515054169548E-26,-1.1518563880486E-13,
-1.));
#23115=DIRECTION('ref_axis',(-8.88178419700126E-14,1.,-1.1518563880486E-13));
#23116=DIRECTION('center_axis',(0.0697564737440288,0.997564050259831,-1.14905052377941E-13));
#23117=DIRECTION('ref_axis',(0.997564050259831,-0.0697564737440288,8.03494398899043E-15));
#23118=DIRECTION('',(-1.00515054169548E-26,1.1518563880486E-13,1.));
#23119=DIRECTION('',(0.997564050259829,-0.0697564737440514,8.03494398899303E-15));
#23120=DIRECTION('',(-1.00515054169548E-26,1.1518563880486E-13,1.));
#23121=DIRECTION('',(0.997564050259831,-0.0697564737440331,8.03494398899092E-15));
#23122=DIRECTION('center_axis',(1.00515054169548E-26,-1.1518563880486E-13,
-1.));
#23123=DIRECTION('ref_axis',(8.72635297355373E-14,-1.,1.1518563880486E-13));
#23124=DIRECTION('',(8.67672446588636E-14,-1.,1.1518563880486E-13));
#23125=DIRECTION('',(1.,8.67672446588636E-14,5.71649135859831E-29));
#23126=DIRECTION('center_axis',(-1.00515054169548E-26,1.1518563880486E-13,
1.));
#23127=DIRECTION('ref_axis',(-8.72635297355373E-14,1.,-1.1518563880486E-13));
#23128=DIRECTION('',(-0.927183854566823,0.374606593415825,-4.31492997631236E-14));
#23129=DIRECTION('center_axis',(-1.00515054169548E-26,1.1518563880486E-13,
1.));
#23130=DIRECTION('ref_axis',(-8.67361737988404E-14,1.,-1.1518563880486E-13));
#23131=DIRECTION('',(8.67672446588636E-14,-1.,1.1518563880486E-13));
#23132=DIRECTION('',(-8.72635297355373E-14,1.,-1.1518563880486E-13));
#23133=DIRECTION('center_axis',(-1.,-8.72635297355373E-14,0.));
#23134=DIRECTION('ref_axis',(-8.72635297355373E-14,1.,-1.1518563880486E-13));
#23135=DIRECTION('',(1.00515054169548E-26,-1.1518563880486E-13,-1.));
#23136=DIRECTION('',(8.72635297355373E-14,-1.,1.1518563880486E-13));
#23137=DIRECTION('center_axis',(1.,8.72635297355374E-14,8.97974505211524E-16));
#23138=DIRECTION('ref_axis',(8.97974505221575E-16,-1.1518563880486E-13,
-1.));
#23139=DIRECTION('',(-1.00515054169548E-26,1.1518563880486E-13,1.));
#23140=DIRECTION('',(-8.72635297355373E-14,1.,-1.1518563880486E-13));
#23141=DIRECTION('',(1.00515054169548E-26,-1.1518563880486E-13,-1.));
#23142=DIRECTION('',(-8.72635297355373E-14,1.,-1.1518563880486E-13));
#23143=DIRECTION('center_axis',(6.53072367436613E-16,-1.1518563880486E-13,
-1.));
#23144=DIRECTION('ref_axis',(-1.,-8.72635297355374E-14,-6.53072367426562E-16));
#23145=DIRECTION('',(0.927183854566753,0.374606593415997,-4.31492997631248E-14));
#23146=DIRECTION('',(1.,8.72635297355373E-14,0.));
#23147=DIRECTION('',(0.927183854566819,-0.374606593415835,4.31492997631247E-14));
#23148=DIRECTION('center_axis',(-0.069756473744203,0.997564050259819,-1.14905052377941E-13));
#23149=DIRECTION('ref_axis',(0.997564050259819,0.069756473744203,-8.03494398899043E-15));
#23150=DIRECTION('',(1.00515054169548E-26,-1.1518563880486E-13,-1.));
#23151=DIRECTION('',(0.997564050259817,0.0697564737442254,-8.03494398899302E-15));
#23152=DIRECTION('',(0.997564050259819,0.0697564737442072,-8.03494398899092E-15));
#23153=DIRECTION('center_axis',(-1.00515054169548E-26,1.1518563880486E-13,
1.));
#23154=DIRECTION('ref_axis',(-8.72635297355373E-14,1.,-1.1518563880486E-13));
#23155=DIRECTION('',(-8.7759814812211E-14,1.,-1.1518563880486E-13));
#23156=DIRECTION('center_axis',(-1.00515054169548E-26,1.1518563880486E-13,
1.));
#23157=DIRECTION('ref_axis',(-8.67361737988404E-14,1.,-1.1518563880486E-13));
#23158=DIRECTION('',(0.927183854566753,0.374606593415997,-4.31492997631248E-14));
#23159=DIRECTION('center_axis',(-1.00515054169548E-26,1.1518563880486E-13,
1.));
#23160=DIRECTION('ref_axis',(-8.74300631892311E-14,1.,-1.1518563880486E-13));
#23161=DIRECTION('',(-1.00515054169548E-26,1.1518563880486E-13,1.));
#23162=DIRECTION('center_axis',(1.00515054169548E-26,-1.1518563880486E-13,
-1.));
#23163=DIRECTION('ref_axis',(-8.74300631892311E-14,1.,-1.1518563880486E-13));
#23164=DIRECTION('',(1.00515054169548E-26,-1.1518563880486E-13,-1.));
#23165=DIRECTION('center_axis',(1.00515054169548E-26,-1.1518563880486E-13,
-1.));
#23166=DIRECTION('ref_axis',(-8.74300631892311E-14,1.,-1.1518563880486E-13));
#23167=DIRECTION('center_axis',(-0.99756405025983,0.0697564737440384,-8.03494398899153E-15));
#23168=DIRECTION('ref_axis',(0.0697564737440384,0.99756405025983,-1.14905052377941E-13));
#23169=DIRECTION('',(0.0697564737440399,0.99756405025983,-1.14905052377941E-13));
#23170=DIRECTION('',(-1.00515054169548E-26,1.1518563880486E-13,1.));
#23171=DIRECTION('',(0.069756473744023,0.997564050259831,-1.14905052377941E-13));
#23172=DIRECTION('center_axis',(1.00515054169548E-26,-1.1518563880486E-13,
-1.));
#23173=DIRECTION('ref_axis',(8.72635297355373E-14,-1.,1.1518563880486E-13));
#23174=DIRECTION('',(1.,8.7759814812211E-14,-5.71649135859831E-29));
#23175=DIRECTION('',(-8.7759814812211E-14,1.,-1.1518563880486E-13));
#23176=DIRECTION('center_axis',(-0.997564050259818,-0.0697564737442121,
8.03494398899149E-15));
#23177=DIRECTION('ref_axis',(-0.0697564737442121,0.997564050259818,-1.14905052377941E-13));
#23178=DIRECTION('',(-0.069756473744197,0.997564050259819,-1.14905052377941E-13));
#23179=DIRECTION('',(1.00515054169548E-26,-1.1518563880486E-13,-1.));
#23180=DIRECTION('',(-0.0697564737442141,0.997564050259818,-1.14905052377941E-13));
#23181=DIRECTION('center_axis',(-1.00515054169548E-26,1.1518563880486E-13,
1.));
#23182=DIRECTION('ref_axis',(-8.72635297355373E-14,1.,-1.1518563880486E-13));
#23183=DIRECTION('',(-1.,-8.67672446588636E-14,-5.71649135859831E-29));
#23184=DIRECTION('center_axis',(-1.00515054169548E-26,1.1518563880486E-13,
1.));
#23185=DIRECTION('ref_axis',(-8.67361737988403E-14,1.,-1.1518563880486E-13));
#23186=DIRECTION('',(-0.374606593415996,0.927183854566754,-1.06798264577828E-13));
#23187=DIRECTION('',(-8.72635297355373E-14,1.,-1.1518563880486E-13));
#23188=DIRECTION('',(0.374606593415834,0.927183854566819,-1.06798264577828E-13));
#23189=DIRECTION('center_axis',(-1.00515054169548E-26,1.1518563880486E-13,
1.));
#23190=DIRECTION('ref_axis',(-8.67361737988404E-14,1.,-1.1518563880486E-13));
#23191=DIRECTION('',(1.,8.7759814812211E-14,-5.71649135859831E-29));
#23192=DIRECTION('center_axis',(-1.00515054169548E-26,1.1518563880486E-13,
1.));
#23193=DIRECTION('ref_axis',(-8.74300631892311E-14,1.,-1.1518563880486E-13));
#23194=DIRECTION('',(-1.00515054169548E-26,1.1518563880486E-13,1.));
#23195=DIRECTION('center_axis',(1.00515054169548E-26,-1.1518563880486E-13,
-1.));
#23196=DIRECTION('ref_axis',(-8.04911692853239E-14,1.,-1.1518563880486E-13));
#23197=DIRECTION('',(1.00515054169548E-26,-1.1518563880486E-13,-1.));
#23198=DIRECTION('center_axis',(1.00515054169548E-26,-1.1518563880486E-13,
-1.));
#23199=DIRECTION('ref_axis',(-8.04911692853239E-14,1.,-1.1518563880486E-13));
#23200=DIRECTION('center_axis',(-0.0697564737440285,-0.997564050259831,
1.14905052377941E-13));
#23201=DIRECTION('ref_axis',(-0.997564050259831,0.0697564737440285,-8.03494398899039E-15));
#23202=DIRECTION('',(-0.997564050259831,0.0697564737440297,-8.03494398899053E-15));
#23203=DIRECTION('',(-1.00515054169548E-26,1.1518563880486E-13,1.));
#23204=DIRECTION('',(-0.997564050259831,0.0697564737440314,-8.03494398899072E-15));
#23205=DIRECTION('center_axis',(1.00515054169548E-26,-1.1518563880486E-13,
-1.));
#23206=DIRECTION('ref_axis',(8.72635297355373E-14,-1.,1.1518563880486E-13));
#23207=DIRECTION('',(-8.67672446588636E-14,1.,-1.1518563880486E-13));
#23208=DIRECTION('',(-1.,-8.67672446588636E-14,-5.71649135859831E-29));
#23209=DIRECTION('center_axis',(-1.00515054169548E-26,1.1518563880486E-13,
1.));
#23210=DIRECTION('ref_axis',(-8.74300631892311E-14,1.,-1.1518563880486E-13));
#23211=DIRECTION('',(-1.00515054169548E-26,1.1518563880486E-13,1.));
#23212=DIRECTION('center_axis',(1.00515054169548E-26,-1.1518563880486E-13,
-1.));
#23213=DIRECTION('ref_axis',(-1.13797860024079E-13,1.,-1.1518563880486E-13));
#23214=DIRECTION('',(1.00515054169548E-26,-1.1518563880486E-13,-1.));
#23215=DIRECTION('center_axis',(1.00515054169548E-26,-1.1518563880486E-13,
-1.));
#23216=DIRECTION('ref_axis',(-1.13797860024079E-13,1.,-1.1518563880486E-13));
#23217=DIRECTION('center_axis',(1.00515054169548E-26,-1.1518563880486E-13,
-1.));
#23218=DIRECTION('ref_axis',(8.72635297355373E-14,-1.,1.1518563880486E-13));
#23219=DIRECTION('',(-1.,-8.7759814812211E-14,5.71649135859831E-29));
#23220=DIRECTION('',(8.7759814812211E-14,-1.,1.1518563880486E-13));
#23221=DIRECTION('',(-0.997564050259819,-0.0697564737442016,8.03494398899027E-15));
#23222=DIRECTION('center_axis',(0.0697564737442016,-0.997564050259819,1.14905052377941E-13));
#23223=DIRECTION('ref_axis',(-0.997564050259819,-0.0697564737442016,8.03494398899027E-15));
#23224=DIRECTION('',(1.00515054169548E-26,-1.1518563880486E-13,-1.));
#23225=DIRECTION('',(-0.997564050259819,-0.0697564737441972,8.03494398898977E-15));
#23226=DIRECTION('center_axis',(-1.00515054169548E-26,1.1518563880486E-13,
1.));
#23227=DIRECTION('ref_axis',(-8.72635297355373E-14,1.,-1.1518563880486E-13));
#23228=DIRECTION('',(8.7759814812211E-14,-1.,1.1518563880486E-13));
#23229=DIRECTION('center_axis',(-1.00515054169548E-26,1.1518563880486E-13,
1.));
#23230=DIRECTION('ref_axis',(-8.67361737988403E-14,1.,-1.1518563880486E-13));
#23231=DIRECTION('',(-0.927183854566753,-0.374606593415997,4.31492997631248E-14));
#23232=DIRECTION('',(-1.,-8.72635297355373E-14,0.));
#23233=DIRECTION('',(-0.927183854566819,0.374606593415835,-4.31492997631247E-14));
#23234=DIRECTION('center_axis',(-1.00515054169548E-26,1.1518563880486E-13,
1.));
#23235=DIRECTION('ref_axis',(-8.67361737988403E-14,1.,-1.1518563880486E-13));
#23236=DIRECTION('',(-8.67672446588636E-14,1.,-1.1518563880486E-13));
#23237=DIRECTION('center_axis',(0.868162779195958,0.359604797490614,0.34202014332563));
#23238=DIRECTION('ref_axis',(0.382683432365172,-0.923879532511253,1.06407127951475E-13));
#23239=DIRECTION('',(0.145459785961516,0.474519896165923,-0.868143029005423));
#23240=DIRECTION('',(0.483645502898238,-0.458543714227443,-0.745536511291574));
#23241=DIRECTION('',(0.338019145174967,-0.933063205484026,0.123028907444791));
#23242=DIRECTION('',(-0.145459785961518,-0.474519896165925,0.868143029005422));
#23243=DIRECTION('',(-0.483645502898236,0.458543714227446,0.745536511291574));
#23244=DIRECTION('',(-0.338019145174969,0.933063205484025,-0.123028907444792));
#23245=DIRECTION('center_axis',(8.72635297355373E-14,-1.,1.1518563880486E-13));
#23246=DIRECTION('ref_axis',(-1.00515054169548E-26,1.1518563880486E-13,
1.));
#23247=DIRECTION('',(-1.,-8.72635297355373E-14,0.));
#23248=DIRECTION('',(-1.00515054169548E-26,1.1518563880486E-13,1.));
#23249=DIRECTION('',(-1.,-8.72635297355373E-14,0.));
#23250=DIRECTION('',(1.00515054169548E-26,-1.1518563880486E-13,-1.));
#23251=DIRECTION('center_axis',(-1.00515054169548E-26,1.1518563880486E-13,
1.));
#23252=DIRECTION('ref_axis',(-8.72635297355373E-14,1.,-1.1518563880486E-13));
#23253=DIRECTION('center_axis',(1.00515054169548E-26,-1.1518563880486E-13,
-1.));
#23254=DIRECTION('ref_axis',(8.72635297355373E-14,-1.,1.1518563880486E-13));
#23255=DIRECTION('',(-0.997564050259819,-0.0697564737442026,8.03494398899039E-15));
#23256=DIRECTION('',(-8.7759814812211E-14,1.,-1.1518563880486E-13));
#23257=DIRECTION('',(1.,8.7759814812211E-14,-5.71649135859831E-29));
#23258=DIRECTION('',(-0.0697564737440384,-0.99756405025983,1.14905052377941E-13));
#23259=DIRECTION('center_axis',(-1.00515054169548E-26,1.1518563880486E-13,
1.));
#23260=DIRECTION('ref_axis',(-8.72635297355373E-14,1.,-1.1518563880486E-13));
#23261=DIRECTION('center_axis',(-1.00515054169548E-26,1.1518563880486E-13,
1.));
#23262=DIRECTION('ref_axis',(-8.72635297355373E-14,1.,-1.1518563880486E-13));
#23263=DIRECTION('',(-1.00515054169548E-26,1.1518563880486E-13,1.));
#23264=DIRECTION('center_axis',(1.00515054169548E-26,-1.1518563880486E-13,
-1.));
#23265=DIRECTION('ref_axis',(-8.01581023779363E-14,1.,-1.1518563880486E-13));
#23266=DIRECTION('',(1.00515054169548E-26,-1.1518563880486E-13,-1.));
#23267=DIRECTION('center_axis',(-8.7759814812211E-14,1.,-1.1518563880486E-13));
#23268=DIRECTION('ref_axis',(1.,8.7759814812211E-14,-5.71649135859828E-29));
#23269=DIRECTION('',(1.00515054169548E-26,-1.1518563880486E-13,-1.));
#23270=DIRECTION('',(1.,8.72635297355373E-14,0.));
#23271=DIRECTION('',(1.00515054169548E-26,-1.1518563880486E-13,-1.));
#23272=DIRECTION('center_axis',(-1.00515054169548E-26,1.1518563880486E-13,
1.));
#23273=DIRECTION('ref_axis',(-8.67361737988403E-14,1.,-1.1518563880486E-13));
#23274=DIRECTION('',(-1.00515054169548E-26,1.1518563880486E-13,1.));
#23275=DIRECTION('center_axis',(-1.00515054169548E-26,1.1518563880486E-13,
1.));
#23276=DIRECTION('ref_axis',(-8.67361737988403E-14,1.,-1.1518563880486E-13));
#23277=DIRECTION('center_axis',(-0.927183854566819,0.374606593415834,-4.31492997631247E-14));
#23278=DIRECTION('ref_axis',(0.374606593415834,0.927183854566819,-1.06798264577828E-13));
#23279=DIRECTION('',(-1.00515054169548E-26,1.1518563880486E-13,1.));
#23280=DIRECTION('',(0.374606593415835,0.927183854566819,-1.06798264577828E-13));
#23281=DIRECTION('center_axis',(-1.,-8.72635297355373E-14,0.));
#23282=DIRECTION('ref_axis',(-8.72635297355373E-14,1.,-1.1518563880486E-13));
#23283=DIRECTION('',(-1.00515054169548E-26,1.1518563880486E-13,1.));
#23284=DIRECTION('',(-8.72635297355373E-14,1.,-1.1518563880486E-13));
#23285=DIRECTION('center_axis',(-0.927183854566754,-0.374606593415996,4.31492997631246E-14));
#23286=DIRECTION('ref_axis',(-0.374606593415996,0.927183854566754,-1.06798264577828E-13));
#23287=DIRECTION('',(1.00515054169548E-26,-1.1518563880486E-13,-1.));
#23288=DIRECTION('',(-0.374606593415997,0.927183854566753,-1.06798264577828E-13));
#23289=DIRECTION('center_axis',(-1.00515054169548E-26,1.1518563880486E-13,
1.));
#23290=DIRECTION('ref_axis',(-8.67361737988403E-14,1.,-1.1518563880486E-13));
#23291=DIRECTION('',(-1.00515054169548E-26,1.1518563880486E-13,1.));
#23292=DIRECTION('center_axis',(-1.00515054169548E-26,1.1518563880486E-13,
1.));
#23293=DIRECTION('ref_axis',(-8.67361737988404E-14,1.,-1.1518563880486E-13));
#23294=DIRECTION('center_axis',(8.67672446588636E-14,-1.,1.1518563880486E-13));
#23295=DIRECTION('ref_axis',(-1.,-8.67672446588636E-14,-5.71649135859828E-29));
#23296=DIRECTION('',(-1.,-8.72635297355373E-14,0.));
#23297=DIRECTION('',(-1.00515054169548E-26,1.1518563880486E-13,1.));
#23298=DIRECTION('',(-1.,-8.72635297355373E-14,0.));
#23299=DIRECTION('center_axis',(1.00515054169548E-26,-1.1518563880486E-13,
-1.));
#23300=DIRECTION('ref_axis',(8.72635297355373E-14,-1.,1.1518563880486E-13));
#23301=DIRECTION('',(0.0697564737442125,-0.997564050259818,1.14905052377941E-13));
#23302=DIRECTION('',(-8.67672446588636E-14,1.,-1.1518563880486E-13));
#23303=DIRECTION('',(0.997564050259831,-0.0697564737440285,8.03494398899039E-15));
#23304=DIRECTION('center_axis',(-1.00515054169548E-26,1.1518563880486E-13,
1.));
#23305=DIRECTION('ref_axis',(-8.72635297355373E-14,1.,-1.1518563880486E-13));
#23306=DIRECTION('center_axis',(-1.00515054169548E-26,1.1518563880486E-13,
1.));
#23307=DIRECTION('ref_axis',(-8.72635297355373E-14,1.,-1.1518563880486E-13));
#23308=DIRECTION('',(-1.00515054169548E-26,1.1518563880486E-13,1.));
#23309=DIRECTION('center_axis',(1.00515054169548E-26,-1.1518563880486E-13,
-1.));
#23310=DIRECTION('ref_axis',(-8.72635297355373E-14,1.,-1.1518563880486E-13));
#23311=DIRECTION('',(1.00515054169548E-26,-1.1518563880486E-13,-1.));
#23312=DIRECTION('center_axis',(-1.,-8.67672446588636E-14,-5.71649135859828E-29));
#23313=DIRECTION('ref_axis',(-8.67672446588636E-14,1.,-1.1518563880486E-13));
#23314=DIRECTION('',(1.00515054169548E-26,-1.1518563880486E-13,-1.));
#23315=DIRECTION('',(-8.72635297355373E-14,1.,-1.1518563880486E-13));
#23316=DIRECTION('',(1.00515054169548E-26,-1.1518563880486E-13,-1.));
#23317=DIRECTION('center_axis',(-1.00515054169548E-26,1.1518563880486E-13,
1.));
#23318=DIRECTION('ref_axis',(-8.67361737988404E-14,1.,-1.1518563880486E-13));
#23319=DIRECTION('',(-1.00515054169548E-26,1.1518563880486E-13,1.));
#23320=DIRECTION('center_axis',(-1.00515054169548E-26,1.1518563880486E-13,
1.));
#23321=DIRECTION('ref_axis',(-8.67361737988404E-14,1.,-1.1518563880486E-13));
#23322=DIRECTION('center_axis',(-0.374606593415835,-0.927183854566819,1.06798264577828E-13));
#23323=DIRECTION('ref_axis',(-0.927183854566819,0.374606593415835,-4.31492997631247E-14));
#23324=DIRECTION('',(-1.00515054169548E-26,1.1518563880486E-13,1.));
#23325=DIRECTION('',(-0.92718385456682,0.374606593415832,-4.31492997631244E-14));
#23326=DIRECTION('center_axis',(8.72635297355373E-14,-1.,1.1518563880486E-13));
#23327=DIRECTION('ref_axis',(-1.00515054169548E-26,1.1518563880486E-13,
1.));
#23328=DIRECTION('',(-1.00515054169548E-26,1.1518563880486E-13,1.));
#23329=DIRECTION('',(-1.,-8.72635297355373E-14,0.));
#23330=DIRECTION('center_axis',(0.374606593415997,-0.927183854566753,1.06798264577828E-13));
#23331=DIRECTION('ref_axis',(-0.927183854566753,-0.374606593415997,4.31492997631247E-14));
#23332=DIRECTION('',(1.00515054169548E-26,-1.1518563880486E-13,-1.));
#23333=DIRECTION('',(-0.927183854566754,-0.374606593415995,4.31492997631245E-14));
#23334=DIRECTION('center_axis',(-1.00515054169548E-26,1.1518563880486E-13,
1.));
#23335=DIRECTION('ref_axis',(-8.67361737988404E-14,1.,-1.1518563880486E-13));
#23336=DIRECTION('',(-1.00515054169548E-26,1.1518563880486E-13,1.));
#23337=DIRECTION('center_axis',(-1.00515054169548E-26,1.1518563880486E-13,
1.));
#23338=DIRECTION('ref_axis',(-8.67361737988404E-14,1.,-1.1518563880486E-13));
#23339=DIRECTION('center_axis',(1.,8.7759814812211E-14,-5.71649135859828E-29));
#23340=DIRECTION('ref_axis',(8.7759814812211E-14,-1.,1.1518563880486E-13));
#23341=DIRECTION('',(8.72635297355373E-14,-1.,1.1518563880486E-13));
#23342=DIRECTION('',(-1.00515054169548E-26,1.1518563880486E-13,1.));
#23343=DIRECTION('',(8.72635297355373E-14,-1.,1.1518563880486E-13));
#23344=DIRECTION('center_axis',(1.00515054169548E-26,-1.1518563880486E-13,
-1.));
#23345=DIRECTION('ref_axis',(8.72635297355373E-14,-1.,1.1518563880486E-13));
#23346=DIRECTION('',(0.997564050259819,0.0697564737442022,-8.03494398899034E-15));
#23347=DIRECTION('',(-1.,-8.7759814812211E-14,5.71649135859831E-29));
#23348=DIRECTION('',(0.0697564737440384,0.99756405025983,-1.14905052377941E-13));
#23349=DIRECTION('center_axis',(-1.00515054169548E-26,1.1518563880486E-13,
1.));
#23350=DIRECTION('ref_axis',(-8.72635297355373E-14,1.,-1.1518563880486E-13));
#23351=DIRECTION('center_axis',(-1.00515054169548E-26,1.1518563880486E-13,
1.));
#23352=DIRECTION('ref_axis',(-8.72635297355373E-14,1.,-1.1518563880486E-13));
#23353=DIRECTION('',(-1.00515054169548E-26,1.1518563880486E-13,1.));
#23354=DIRECTION('center_axis',(1.00515054169548E-26,-1.1518563880486E-13,
-1.));
#23355=DIRECTION('ref_axis',(-9.17044218340379E-14,1.,-1.1518563880486E-13));
#23356=DIRECTION('',(1.00515054169548E-26,-1.1518563880486E-13,-1.));
#23357=DIRECTION('center_axis',(8.7759814812211E-14,-1.,1.1518563880486E-13));
#23358=DIRECTION('ref_axis',(-1.,-8.7759814812211E-14,5.71649135859828E-29));
#23359=DIRECTION('',(1.00515054169548E-26,-1.1518563880486E-13,-1.));
#23360=DIRECTION('',(-1.,-8.72635297355373E-14,0.));
#23361=DIRECTION('',(1.00515054169548E-26,-1.1518563880486E-13,-1.));
#23362=DIRECTION('center_axis',(-1.00515054169548E-26,1.1518563880486E-13,
1.));
#23363=DIRECTION('ref_axis',(-8.67361737988404E-14,1.,-1.1518563880486E-13));
#23364=DIRECTION('',(-1.00515054169548E-26,1.1518563880486E-13,1.));
#23365=DIRECTION('center_axis',(-1.00515054169548E-26,1.1518563880486E-13,
1.));
#23366=DIRECTION('ref_axis',(-8.67361737988404E-14,1.,-1.1518563880486E-13));
#23367=DIRECTION('center_axis',(0.927183854566819,-0.374606593415834,4.31492997631247E-14));
#23368=DIRECTION('ref_axis',(-0.374606593415834,-0.927183854566819,1.06798264577828E-13));
#23369=DIRECTION('',(-1.00515054169548E-26,1.1518563880486E-13,1.));
#23370=DIRECTION('',(-0.374606593415836,-0.927183854566818,1.06798264577828E-13));
#23371=DIRECTION('center_axis',(1.,8.72635297355373E-14,0.));
#23372=DIRECTION('ref_axis',(8.72635297355373E-14,-1.,1.1518563880486E-13));
#23373=DIRECTION('',(-1.00515054169548E-26,1.1518563880486E-13,1.));
#23374=DIRECTION('',(8.72635297355373E-14,-1.,1.1518563880486E-13));
#23375=DIRECTION('center_axis',(0.927183854566754,0.374606593415996,-4.31492997631246E-14));
#23376=DIRECTION('ref_axis',(0.374606593415996,-0.927183854566754,1.06798264577828E-13));
#23377=DIRECTION('',(1.00515054169548E-26,-1.1518563880486E-13,-1.));
#23378=DIRECTION('',(0.374606593415997,-0.927183854566753,1.06798264577828E-13));
#23379=DIRECTION('center_axis',(-1.00515054169548E-26,1.1518563880486E-13,
1.));
#23380=DIRECTION('ref_axis',(-8.67361737988403E-14,1.,-1.1518563880486E-13));
#23381=DIRECTION('',(-1.00515054169548E-26,1.1518563880486E-13,1.));
#23382=DIRECTION('center_axis',(-1.00515054169548E-26,1.1518563880486E-13,
1.));
#23383=DIRECTION('ref_axis',(-8.67361737988404E-14,1.,-1.1518563880486E-13));
#23384=DIRECTION('center_axis',(-8.67672446588636E-14,1.,-1.1518563880486E-13));
#23385=DIRECTION('ref_axis',(1.,8.67672446588636E-14,5.71649135859828E-29));
#23386=DIRECTION('',(1.,8.72635297355373E-14,0.));
#23387=DIRECTION('',(-1.00515054169548E-26,1.1518563880486E-13,1.));
#23388=DIRECTION('',(1.,8.72635297355373E-14,0.));
#23389=DIRECTION('center_axis',(1.00515054169548E-26,-1.1518563880486E-13,
-1.));
#23390=DIRECTION('ref_axis',(8.72635297355373E-14,-1.,1.1518563880486E-13));
#23391=DIRECTION('',(-0.0697564737442125,0.997564050259818,-1.14905052377941E-13));
#23392=DIRECTION('',(8.67672446588636E-14,-1.,1.1518563880486E-13));
#23393=DIRECTION('',(-0.997564050259831,0.0697564737440281,-8.03494398899034E-15));
#23394=DIRECTION('center_axis',(-1.00515054169548E-26,1.1518563880486E-13,
1.));
#23395=DIRECTION('ref_axis',(-8.72635297355373E-14,1.,-1.1518563880486E-13));
#23396=DIRECTION('center_axis',(-1.00515054169548E-26,1.1518563880486E-13,
1.));
#23397=DIRECTION('ref_axis',(-8.72635297355373E-14,1.,-1.1518563880486E-13));
#23398=DIRECTION('',(-1.00515054169548E-26,1.1518563880486E-13,1.));
#23399=DIRECTION('center_axis',(1.00515054169548E-26,-1.1518563880486E-13,
-1.));
#23400=DIRECTION('ref_axis',(-8.72635297355373E-14,1.,-1.1518563880486E-13));
#23401=DIRECTION('',(1.00515054169548E-26,-1.1518563880486E-13,-1.));
#23402=DIRECTION('center_axis',(1.,8.67672446588636E-14,5.71649135859828E-29));
#23403=DIRECTION('ref_axis',(8.67672446588636E-14,-1.,1.1518563880486E-13));
#23404=DIRECTION('',(1.00515054169548E-26,-1.1518563880486E-13,-1.));
#23405=DIRECTION('',(8.72635297355373E-14,-1.,1.1518563880486E-13));
#23406=DIRECTION('',(1.00515054169548E-26,-1.1518563880486E-13,-1.));
#23407=DIRECTION('center_axis',(-1.00515054169548E-26,1.1518563880486E-13,
1.));
#23408=DIRECTION('ref_axis',(-8.67361737988403E-14,1.,-1.1518563880486E-13));
#23409=DIRECTION('',(-1.00515054169548E-26,1.1518563880486E-13,1.));
#23410=DIRECTION('center_axis',(-1.00515054169548E-26,1.1518563880486E-13,
1.));
#23411=DIRECTION('ref_axis',(-8.67361737988403E-14,1.,-1.1518563880486E-13));
#23412=DIRECTION('center_axis',(0.374606593415835,0.927183854566819,-1.06798264577828E-13));
#23413=DIRECTION('ref_axis',(0.927183854566819,-0.374606593415835,4.31492997631247E-14));
#23414=DIRECTION('',(-1.00515054169548E-26,1.1518563880486E-13,1.));
#23415=DIRECTION('',(0.927183854566819,-0.374606593415834,4.31492997631246E-14));
#23416=DIRECTION('center_axis',(-8.72635297355373E-14,1.,-1.1518563880486E-13));
#23417=DIRECTION('ref_axis',(1.00515054169548E-26,-1.1518563880486E-13,
-1.));
#23418=DIRECTION('',(-1.00515054169548E-26,1.1518563880486E-13,1.));
#23419=DIRECTION('',(1.,8.72635297355373E-14,0.));
#23420=DIRECTION('center_axis',(-0.374606593415997,0.927183854566753,-1.06798264577828E-13));
#23421=DIRECTION('ref_axis',(0.927183854566753,0.374606593415997,-4.31492997631247E-14));
#23422=DIRECTION('',(1.00515054169548E-26,-1.1518563880486E-13,-1.));
#23423=DIRECTION('',(0.927183854566754,0.374606593415995,-4.31492997631245E-14));
#23424=DIRECTION('center_axis',(-1.00515054169548E-26,1.1518563880486E-13,
1.));
#23425=DIRECTION('ref_axis',(-8.67361737988403E-14,1.,-1.1518563880486E-13));
#23426=DIRECTION('',(-1.00515054169548E-26,1.1518563880486E-13,1.));
#23427=DIRECTION('center_axis',(-1.00515054169548E-26,1.1518563880486E-13,
1.));
#23428=DIRECTION('ref_axis',(-8.67361737988403E-14,1.,-1.1518563880486E-13));
#23429=DIRECTION('center_axis',(-1.,-8.7759814812211E-14,5.71649135859828E-29));
#23430=DIRECTION('ref_axis',(-8.7759814812211E-14,1.,-1.1518563880486E-13));
#23431=DIRECTION('',(-1.00515054169548E-26,1.1518563880486E-13,1.));
#23432=DIRECTION('',(-8.72635297355373E-14,1.,-1.1518563880486E-13));
#23433=DIRECTION('center_axis',(-0.342020143298471,7.83793320738915E-14,
0.939692620795808));
#23434=DIRECTION('ref_axis',(0.939692620795808,1.21396703647044E-13,0.342020143298471));
#23435=DIRECTION('',(-0.868162779198992,-0.382683432380925,-0.315985410097739));
#23436=DIRECTION('',(0.359604797523941,-0.923879532498189,0.130885442386437));
#23437=DIRECTION('',(0.868162779198971,0.382683432380902,0.315985410097825));
#23438=DIRECTION('center_axis',(0.140416818327027,-0.800103145195805,0.58319642846874));
#23439=DIRECTION('ref_axis',(-5.1390560202283E-14,0.589032278086391,0.808109507042429));
#23440=DIRECTION('',(-0.868162779198997,-0.382683432381008,-0.315985410097624));
#23441=DIRECTION('',(0.476000531462651,-0.461939766230853,-0.748354960177227));
#23442=DIRECTION('center_axis',(0.482436961612334,-0.800103145195884,-0.356496192290904));
#23443=DIRECTION('ref_axis',(-0.856369374376448,-0.516363723193343,5.94698587038405E-14));
#23444=DIRECTION('',(-0.868162779198969,-0.38268343238096,-0.315985410097759));
#23445=DIRECTION('',(0.116395733952524,0.461939766231793,-0.879240402558577));
#23446=DIRECTION('center_axis',(0.342020143298471,-7.83793320738915E-14,
-0.939692620795808));
#23447=DIRECTION('ref_axis',(-0.939692620795808,-1.21396703647044E-13,-0.342020143298471));
#23448=DIRECTION('',(-0.868162779198955,-0.382683432380959,-0.3159854100978));
#23449=DIRECTION('',(-0.359604797523941,0.923879532498189,-0.130885442386437));
#23450=DIRECTION('center_axis',(-0.140416818327027,0.800103145195805,-0.58319642846874));
#23451=DIRECTION('ref_axis',(5.1390560202283E-14,-0.589032278086391,-0.808109507042429));
#23452=DIRECTION('',(-0.86816277919896,-0.382683432380859,-0.315985410097906));
#23453=DIRECTION('',(-0.476000531462647,0.461939766230845,0.748354960177234));
#23454=DIRECTION('center_axis',(-0.482436961612334,0.800103145195884,0.356496192290904));
#23455=DIRECTION('ref_axis',(0.856369374376448,0.516363723193343,-5.94698587038405E-14));
#23456=DIRECTION('',(-0.116395733952528,-0.461939766231792,0.879240402558578));
#23457=DIRECTION('center_axis',(-8.72635297355373E-14,1.,-1.11694157466017E-13));
#23458=DIRECTION('ref_axis',(9.74682643132155E-27,-1.11694157466017E-13,
-1.));
#23459=DIRECTION('center_axis',(-8.72635297355373E-14,1.,-1.11694157466017E-13));
#23460=DIRECTION('ref_axis',(9.74682643132155E-27,-1.11694157466017E-13,
-1.));
#23461=DIRECTION('center_axis',(1.,8.72635297355373E-14,0.));
#23462=DIRECTION('ref_axis',(8.72635297355373E-14,-1.,1.1518563880486E-13));
#23463=DIRECTION('',(8.72635297355373E-14,-1.,1.1518563880486E-13));
#23464=DIRECTION('',(8.72635297355373E-14,-1.,1.1518563880486E-13));
#23465=DIRECTION('center_axis',(-1.00515054169548E-26,1.1518563880486E-13,
1.));
#23466=DIRECTION('ref_axis',(-8.72635297355373E-14,1.,-1.1518563880486E-13));
#23467=DIRECTION('',(8.72635297355373E-14,-1.,1.1518563880486E-13));
#23468=DIRECTION('center_axis',(-1.,-8.72635297355373E-14,0.));
#23469=DIRECTION('ref_axis',(-8.72635297355373E-14,1.,-1.1518563880486E-13));
#23470=DIRECTION('',(-8.72635297355373E-14,1.,-1.1518563880486E-13));
#23471=DIRECTION('center_axis',(-1.00515054169548E-26,1.1518563880486E-13,
1.));
#23472=DIRECTION('ref_axis',(-8.72635297355373E-14,1.,-1.1518563880486E-13));
#23473=DIRECTION('center_axis',(-1.00515054169548E-26,1.1518563880486E-13,
1.));
#23474=DIRECTION('ref_axis',(-8.72635297355373E-14,1.,-1.1518563880486E-13));
#23475=DIRECTION('center_axis',(-1.00515054169548E-26,1.1518563880486E-13,
1.));
#23476=DIRECTION('ref_axis',(-8.72635297355373E-14,1.,-1.1518563880486E-13));
#23477=DIRECTION('center_axis',(-1.00515054169548E-26,1.1518563880486E-13,
1.));
#23478=DIRECTION('ref_axis',(-8.72635297355373E-14,1.,-1.1518563880486E-13));
#23479=DIRECTION('center_axis',(-1.00515054169548E-26,1.1518563880486E-13,
1.));
#23480=DIRECTION('ref_axis',(-8.72635297355373E-14,1.,-1.1518563880486E-13));
#23481=DIRECTION('center_axis',(-0.0697564737442026,0.997564050259819,-1.14905052377941E-13));
#23482=DIRECTION('ref_axis',(0.997564050259819,0.0697564737442026,-8.03494398899039E-15));
#23483=DIRECTION('',(-0.997564050259819,-0.0697564737441991,8.03494398898999E-15));
#23484=DIRECTION('',(-1.00515054169548E-26,1.1518563880486E-13,1.));
#23485=DIRECTION('',(-0.997564050259819,-0.0697564737441972,8.03494398898977E-15));
#23486=DIRECTION('center_axis',(1.00515054169548E-26,-1.1518563880486E-13,
-1.));
#23487=DIRECTION('ref_axis',(8.72635297355373E-14,-1.,1.1518563880486E-13));
#23488=DIRECTION('',(0.0697564737440412,0.99756405025983,-1.14905052377941E-13));
#23489=DIRECTION('center_axis',(-1.00515054169548E-26,1.1518563880486E-13,
1.));
#23490=DIRECTION('ref_axis',(-8.72635297355373E-14,1.,-1.1518563880486E-13));
#23491=DIRECTION('',(0.997564050259818,0.0697564737442111,-8.03494398899137E-15));
#23492=DIRECTION('center_axis',(-1.00515054169548E-26,1.1518563880486E-13,
1.));
#23493=DIRECTION('ref_axis',(-8.72635297355373E-14,1.,-1.1518563880486E-13));
#23494=DIRECTION('',(0.0697564737440384,0.99756405025983,-1.14905052377941E-13));
#23495=DIRECTION('center_axis',(-1.00515054169548E-26,1.1518563880486E-13,
1.));
#23496=DIRECTION('ref_axis',(-8.72635297355373E-14,1.,-1.1518563880486E-13));
#23497=DIRECTION('center_axis',(-0.99756405025983,0.0697564737440384,-8.03494398899153E-15));
#23498=DIRECTION('ref_axis',(0.0697564737440384,0.99756405025983,-1.14905052377941E-13));
#23499=DIRECTION('',(-0.0697564737440323,-0.997564050259831,1.14905052377941E-13));
#23500=DIRECTION('',(1.00515054169548E-26,-1.1518563880486E-13,-1.));
#23501=DIRECTION('center_axis',(-1.00515054169548E-26,1.1518563880486E-13,
1.));
#23502=DIRECTION('ref_axis',(-8.72635297355373E-14,1.,-1.1518563880486E-13));
#23503=DIRECTION('',(0.0697564737442125,-0.997564050259818,1.14905052377941E-13));
#23504=DIRECTION('center_axis',(-1.00515054169548E-26,1.1518563880486E-13,
1.));
#23505=DIRECTION('ref_axis',(-8.72635297355373E-14,1.,-1.1518563880486E-13));
#23506=DIRECTION('center_axis',(-0.997564050259818,-0.0697564737442125,
8.03494398899153E-15));
#23507=DIRECTION('ref_axis',(-0.0697564737442125,0.997564050259818,-1.14905052377941E-13));
#23508=DIRECTION('',(0.0697564737442101,-0.997564050259818,1.14905052377941E-13));
#23509=DIRECTION('',(-1.00515054169548E-26,1.1518563880486E-13,1.));
#23510=DIRECTION('center_axis',(1.00515054169548E-26,-1.1518563880486E-13,
-1.));
#23511=DIRECTION('ref_axis',(8.72635297355373E-14,-1.,1.1518563880486E-13));
#23512=DIRECTION('',(-0.99756405025983,0.069756473744037,-8.03494398899137E-15));
#23513=DIRECTION('center_axis',(-1.00515054169548E-26,1.1518563880486E-13,
1.));
#23514=DIRECTION('ref_axis',(-8.72635297355373E-14,1.,-1.1518563880486E-13));
#23515=DIRECTION('',(-0.0697564737442153,0.997564050259818,-1.14905052377941E-13));
#23516=DIRECTION('center_axis',(-1.00515054169548E-26,1.1518563880486E-13,
1.));
#23517=DIRECTION('ref_axis',(-8.72635297355373E-14,1.,-1.1518563880486E-13));
#23518=DIRECTION('',(-0.997564050259831,0.0697564737440285,-8.03494398899039E-15));
#23519=DIRECTION('center_axis',(-0.0697564737440285,-0.997564050259831,
1.14905052377941E-13));
#23520=DIRECTION('ref_axis',(-0.997564050259831,0.0697564737440285,-8.03494398899039E-15));
#23521=DIRECTION('',(0.997564050259831,-0.0697564737440292,8.03494398899047E-15));
#23522=DIRECTION('center_axis',(-1.00515054169548E-26,1.1518563880486E-13,
1.));
#23523=DIRECTION('ref_axis',(-8.72635297355373E-14,1.,-1.1518563880486E-13));
#23524=DIRECTION('',(0.997564050259819,0.0697564737442022,-8.03494398899034E-15));
#23525=DIRECTION('center_axis',(0.0697564737442022,-0.997564050259819,1.14905052377941E-13));
#23526=DIRECTION('ref_axis',(-0.997564050259819,-0.0697564737442022,8.03494398899034E-15));
#23527=DIRECTION('',(0.997564050259819,0.0697564737442046,-8.03494398899062E-15));
#23528=DIRECTION('center_axis',(1.00515054169548E-26,-1.1518563880486E-13,
-1.));
#23529=DIRECTION('ref_axis',(8.72635297355373E-14,-1.,1.1518563880486E-13));
#23530=DIRECTION('',(-0.0697564737440384,-0.99756405025983,1.14905052377941E-13));
#23531=DIRECTION('center_axis',(-1.00515054169548E-26,1.1518563880486E-13,
1.));
#23532=DIRECTION('ref_axis',(-8.72635297355373E-14,1.,-1.1518563880486E-13));
#23533=DIRECTION('',(-0.0697564737440412,-0.99756405025983,1.14905052377941E-13));
#23534=DIRECTION('center_axis',(-1.00515054169548E-26,1.1518563880486E-13,
1.));
#23535=DIRECTION('ref_axis',(-8.72635297355373E-14,1.,-1.1518563880486E-13));
#23536=DIRECTION('',(-0.997564050259818,-0.0697564737442111,8.03494398899137E-15));
#23537=DIRECTION('center_axis',(0.99756405025983,-0.0697564737440384,8.03494398899153E-15));
#23538=DIRECTION('ref_axis',(-0.0697564737440384,-0.99756405025983,1.14905052377941E-13));
#23539=DIRECTION('',(0.0697564737440399,0.99756405025983,-1.14905052377941E-13));
#23540=DIRECTION('',(1.00515054169548E-26,-1.1518563880486E-13,-1.));
#23541=DIRECTION('center_axis',(-1.00515054169548E-26,1.1518563880486E-13,
1.));
#23542=DIRECTION('ref_axis',(-8.72635297355373E-14,1.,-1.1518563880486E-13));
#23543=DIRECTION('',(-0.0697564737442125,0.997564050259818,-1.14905052377941E-13));
#23544=DIRECTION('center_axis',(-1.00515054169548E-26,1.1518563880486E-13,
1.));
#23545=DIRECTION('ref_axis',(-8.72635297355373E-14,1.,-1.1518563880486E-13));
#23546=DIRECTION('center_axis',(0.997564050259818,0.0697564737442125,-8.03494398899153E-15));
#23547=DIRECTION('ref_axis',(0.0697564737442125,-0.997564050259818,1.14905052377941E-13));
#23548=DIRECTION('',(-0.0697564737442101,0.997564050259818,-1.14905052377941E-13));
#23549=DIRECTION('',(-1.00515054169548E-26,1.1518563880486E-13,1.));
#23550=DIRECTION('center_axis',(1.00515054169548E-26,-1.1518563880486E-13,
-1.));
#23551=DIRECTION('ref_axis',(8.72635297355373E-14,-1.,1.1518563880486E-13));
#23552=DIRECTION('',(0.997564050259831,-0.0697564737440281,8.03494398899034E-15));
#23553=DIRECTION('center_axis',(-1.00515054169548E-26,1.1518563880486E-13,
1.));
#23554=DIRECTION('ref_axis',(-8.72635297355373E-14,1.,-1.1518563880486E-13));
#23555=DIRECTION('',(0.99756405025983,-0.069756473744037,8.03494398899137E-15));
#23556=DIRECTION('center_axis',(-1.00515054169548E-26,1.1518563880486E-13,
1.));
#23557=DIRECTION('ref_axis',(-8.72635297355373E-14,1.,-1.1518563880486E-13));
#23558=DIRECTION('',(0.0697564737442153,-0.997564050259818,1.14905052377941E-13));
#23559=DIRECTION('center_axis',(-1.00515054169548E-26,1.1518563880486E-13,
1.));
#23560=DIRECTION('ref_axis',(-8.72635297355373E-14,1.,-1.1518563880486E-13));
#23561=DIRECTION('center_axis',(0.0697564737440281,0.997564050259831,-1.14905052377941E-13));
#23562=DIRECTION('ref_axis',(0.997564050259831,-0.0697564737440281,8.03494398899034E-15));
#23563=DIRECTION('',(-0.997564050259831,0.0697564737440302,-8.03494398899059E-15));
#23564=DIRECTION('',(1.00515054169548E-26,-1.1518563880486E-13,-1.));
#23565=DIRECTION('center_axis',(-1.00515054169548E-26,1.1518563880486E-13,
1.));
#23566=DIRECTION('ref_axis',(-8.72635297355373E-14,1.,-1.1518563880486E-13));
#23567=DIRECTION('center_axis',(-1.00515054169548E-26,1.1518563880486E-13,
1.));
#23568=DIRECTION('ref_axis',(-8.72635297355373E-14,1.,-1.1518563880486E-13));
#23569=DIRECTION('center_axis',(-0.868162779192245,-0.38268343239671,-0.315985410097158));
#23570=DIRECTION('ref_axis',(-0.403349423721026,0.915046032931631,-1.05414319346039E-13));
#23571=DIRECTION('center_axis',(-8.72635297355373E-14,1.,-1.11694157466017E-13));
#23572=DIRECTION('ref_axis',(9.74682643132155E-27,-1.11694157466017E-13,
-1.));
#23573=DIRECTION('',(0.5,-5.61219244883788E-14,-0.866025403784439));
#23574=DIRECTION('',(-0.5,-1.43385454223916E-13,-0.866025403784438));
#23575=DIRECTION('',(-1.,-8.72635297355373E-14,0.));
#23576=DIRECTION('',(-0.5,5.61219244883788E-14,0.866025403784439));
#23577=DIRECTION('',(0.5,1.43385454223916E-13,0.866025403784439));
#23578=DIRECTION('',(1.,8.72635297355373E-14,-1.21904419394898E-29));
#23579=DIRECTION('center_axis',(0.0697564737442111,-0.997564050259818,1.14905052377941E-13));
#23580=DIRECTION('ref_axis',(-0.997564050259818,-0.0697564737442111,8.03494398899137E-15));
#23581=DIRECTION('',(1.00515054169548E-26,-1.1518563880486E-13,-1.));
#23582=DIRECTION('',(1.00515054169548E-26,-1.1518563880486E-13,-1.));
#23583=DIRECTION('center_axis',(-1.00515054169548E-26,1.1518563880486E-13,
1.));
#23584=DIRECTION('ref_axis',(-8.72635297355373E-14,1.,-1.1518563880486E-13));
#23585=DIRECTION('',(1.00515054169548E-26,-1.1518563880486E-13,-1.));
#23586=DIRECTION('center_axis',(0.99756405025983,-0.0697564737440412,8.03494398899185E-15));
#23587=DIRECTION('ref_axis',(-0.0697564737440412,-0.99756405025983,1.14905052377941E-13));
#23588=DIRECTION('',(1.00515054169548E-26,-1.1518563880486E-13,-1.));
#23589=DIRECTION('center_axis',(-1.00515054169548E-26,1.1518563880486E-13,
1.));
#23590=DIRECTION('ref_axis',(-8.72635297355373E-14,1.,-1.1518563880486E-13));
#23591=DIRECTION('',(1.00515054169548E-26,-1.1518563880486E-13,-1.));
#23592=DIRECTION('center_axis',(0.997564050259818,0.0697564737442153,-8.03494398899185E-15));
#23593=DIRECTION('ref_axis',(0.0697564737442153,-0.997564050259818,1.14905052377941E-13));
#23594=DIRECTION('',(1.00515054169548E-26,-1.1518563880486E-13,-1.));
#23595=DIRECTION('center_axis',(-1.00515054169548E-26,1.1518563880486E-13,
1.));
#23596=DIRECTION('ref_axis',(-8.72635297355373E-14,1.,-1.1518563880486E-13));
#23597=DIRECTION('',(1.00515054169548E-26,-1.1518563880486E-13,-1.));
#23598=DIRECTION('center_axis',(0.069756473744037,0.99756405025983,-1.14905052377941E-13));
#23599=DIRECTION('ref_axis',(0.99756405025983,-0.069756473744037,8.03494398899137E-15));
#23600=DIRECTION('center_axis',(-0.0697564737442111,0.997564050259818,-1.14905052377941E-13));
#23601=DIRECTION('ref_axis',(0.997564050259818,0.0697564737442111,-8.03494398899137E-15));
#23602=DIRECTION('',(1.00515054169548E-26,-1.1518563880486E-13,-1.));
#23603=DIRECTION('center_axis',(-1.00515054169548E-26,1.1518563880486E-13,
1.));
#23604=DIRECTION('ref_axis',(-8.72635297355373E-14,1.,-1.1518563880486E-13));
#23605=DIRECTION('',(1.00515054169548E-26,-1.1518563880486E-13,-1.));
#23606=DIRECTION('center_axis',(-0.99756405025983,0.0697564737440412,-8.03494398899185E-15));
#23607=DIRECTION('ref_axis',(0.0697564737440412,0.99756405025983,-1.14905052377941E-13));
#23608=DIRECTION('',(1.00515054169548E-26,-1.1518563880486E-13,-1.));
#23609=DIRECTION('center_axis',(-1.00515054169548E-26,1.1518563880486E-13,
1.));
#23610=DIRECTION('ref_axis',(-8.72635297355373E-14,1.,-1.1518563880486E-13));
#23611=DIRECTION('',(1.00515054169548E-26,-1.1518563880486E-13,-1.));
#23612=DIRECTION('center_axis',(-0.997564050259818,-0.0697564737442153,
8.03494398899185E-15));
#23613=DIRECTION('ref_axis',(-0.0697564737442153,0.997564050259818,-1.14905052377941E-13));
#23614=DIRECTION('',(1.00515054169548E-26,-1.1518563880486E-13,-1.));
#23615=DIRECTION('center_axis',(-1.00515054169548E-26,1.1518563880486E-13,
1.));
#23616=DIRECTION('ref_axis',(-8.72635297355373E-14,1.,-1.1518563880486E-13));
#23617=DIRECTION('',(1.00515054169548E-26,-1.1518563880486E-13,-1.));
#23618=DIRECTION('center_axis',(-0.069756473744037,-0.99756405025983,1.14905052377941E-13));
#23619=DIRECTION('ref_axis',(-0.99756405025983,0.069756473744037,-8.03494398899137E-15));
#23620=DIRECTION('',(1.00515054169548E-26,-1.1518563880486E-13,-1.));
#23621=DIRECTION('center_axis',(-1.00515054169548E-26,1.1518563880486E-13,
1.));
#23622=DIRECTION('ref_axis',(8.71410650556226E-14,-1.,1.1518563880486E-13));
#23623=DIRECTION('center_axis',(8.72635297355373E-14,-1.,1.1518563880486E-13));
#23624=DIRECTION('ref_axis',(-1.,-8.72635297355373E-14,-1.43492962746861E-42));
#23625=DIRECTION('',(-1.,-8.72635297355373E-14,0.));
#23626=DIRECTION('',(-1.,-8.72635297355373E-14,0.));
#23627=DIRECTION('',(-1.00515054169548E-26,1.1518563880486E-13,1.));
#23628=DIRECTION('',(1.,8.72635297355373E-14,2.47817639425246E-16));
#23629=DIRECTION('',(1.,8.72635297355373E-14,2.47817639425246E-16));
#23630=DIRECTION('',(1.,8.72635297355373E-14,1.40416384211369E-42));
#23631=DIRECTION('',(1.65211759626891E-16,-1.1518563880486E-13,-1.));
#23632=DIRECTION('',(-1.,-8.72635297355373E-14,0.));
#23633=DIRECTION('center_axis',(2.47817639435298E-16,-1.1518563880486E-13,
-1.));
#23634=DIRECTION('ref_axis',(-1.,-8.72635297355373E-14,-2.47817639425246E-16));
#23635=DIRECTION('center_axis',(9.74874922969709E-27,-1.11716191852906E-13,
-1.));
#23636=DIRECTION('ref_axis',(8.73144149574993E-14,-1.,1.11716191852906E-13));
#23637=DIRECTION('center_axis',(9.74874922969709E-27,-1.11716191852906E-13,
-1.));
#23638=DIRECTION('ref_axis',(8.73144149574993E-14,-1.,1.11716191852906E-13));
#23639=DIRECTION('center_axis',(-9.74682643132153E-27,1.11694157466017E-13,
1.));
#23640=DIRECTION('ref_axis',(-8.72635297355373E-14,1.,-1.11694157466017E-13));
#23641=DIRECTION('center_axis',(-9.74874922969709E-27,1.11716191852906E-13,
1.));
#23642=DIRECTION('ref_axis',(9.07838619094529E-14,-1.,1.11716191852906E-13));
#23643=DIRECTION('',(1.,8.72635297355373E-14,0.));
#23644=DIRECTION('center_axis',(-9.74874922969709E-27,1.11716191852906E-13,
1.));
#23645=DIRECTION('ref_axis',(8.38449680055457E-14,-1.,1.11716191852906E-13));
#23646=DIRECTION('center_axis',(-8.72635297355373E-14,1.,-1.11694157466017E-13));
#23647=DIRECTION('ref_axis',(9.74682643132155E-27,-1.11694157466017E-13,
-1.));
#23648=DIRECTION('',(6.60847038457304E-16,1.1518563880486E-13,1.));
#23649=DIRECTION('',(1.,8.72635297355373E-14,-1.21904419394898E-29));
#23650=DIRECTION('',(1.,8.72635297355373E-14,-1.21904419394898E-29));
#23651=DIRECTION('',(-1.,-8.72635297355373E-14,0.));
#23652=DIRECTION('',(6.60847038477406E-16,-1.1518563880486E-13,-1.));
#23653=DIRECTION('',(-1.,-8.72635297355373E-14,0.));
#23654=DIRECTION('',(-1.,-8.72635297355373E-14,0.));
#23655=DIRECTION('center_axis',(-8.72635297355373E-14,1.,-1.11694157466017E-13));
#23656=DIRECTION('ref_axis',(9.74682643132155E-27,-1.11694157466017E-13,
-1.));
#23657=DIRECTION('',(0.5,-5.61219244883788E-14,-0.866025403784439));
#23658=DIRECTION('',(-0.5,-1.43385454223916E-13,-0.866025403784439));
#23659=DIRECTION('',(-1.,-8.72635297355373E-14,0.));
#23660=DIRECTION('',(-0.5,5.61219244883788E-14,0.866025403784439));
#23661=DIRECTION('',(0.5,1.43385454223916E-13,0.866025403784439));
#23662=DIRECTION('',(1.,8.72635297355373E-14,-1.21904419394898E-29));
#23663=DIRECTION('center_axis',(9.74874922969709E-27,-1.11716191852906E-13,
-1.));
#23664=DIRECTION('ref_axis',(1.28885450781528E-13,1.,-1.11716191852906E-13));
#23665=DIRECTION('center_axis',(0.866025403784439,1.97253548418657E-14,
-0.5));
#23666=DIRECTION('ref_axis',(-0.5,-1.43385454223916E-13,-0.866025403784439));
#23667=DIRECTION('',(8.57516739673986E-14,-1.,1.14312768470149E-13));
#23668=DIRECTION('',(0.500000000000001,1.43385454223916E-13,0.866025403784438));
#23669=DIRECTION('',(-8.72635297355373E-14,1.,-1.1518563880486E-13));
#23670=DIRECTION('center_axis',(1.00393149750153E-26,-1.1518563880486E-13,
-1.));
#23671=DIRECTION('ref_axis',(-1.,-8.72635297355373E-14,1.219044193949E-29));
#23672=DIRECTION('',(1.,8.72635297355373E-14,1.40416384211369E-42));
#23673=DIRECTION('',(-8.57516739673986E-14,1.,-1.14312768470149E-13));
#23674=DIRECTION('center_axis',(-0.866025403784439,-1.31419512307882E-13,
-0.5));
#23675=DIRECTION('ref_axis',(-0.5,5.61219244883788E-14,0.866025403784439));
#23676=DIRECTION('',(0.500000000000001,-5.61219244883783E-14,-0.866025403784438));
#23677=DIRECTION('',(-8.8775385503676E-14,1.,-1.14312768470149E-13));
#23678=DIRECTION('center_axis',(-0.866025403784438,-1.97253548418655E-14,
0.5));
#23679=DIRECTION('ref_axis',(0.5,1.43385454223916E-13,0.866025403784438));
#23680=DIRECTION('',(-0.5,-1.43385454223916E-13,-0.866025403784438));
#23681=DIRECTION('',(-8.72635297355373E-14,1.,-1.11694157466017E-13));
#23682=DIRECTION('center_axis',(-9.74682643132153E-27,1.11694157466017E-13,
1.));
#23683=DIRECTION('ref_axis',(-8.72635297355373E-14,1.,-1.11694157466017E-13));
#23684=DIRECTION('',(-1.,-8.72635297355373E-14,-1.40416384211369E-42));
#23685=DIRECTION('',(-8.57516739673986E-14,1.,-1.14312768470149E-13));
#23686=DIRECTION('center_axis',(0.866025403784439,1.31419512307882E-13,
0.5));
#23687=DIRECTION('ref_axis',(0.5,-5.61219244883788E-14,-0.866025403784439));
#23688=DIRECTION('',(-0.5,5.61219244883785E-14,0.866025403784438));
#23689=DIRECTION('center_axis',(-8.72635297355373E-14,1.,-1.11716191852906E-13));
#23690=DIRECTION('ref_axis',(-1.89882151931492E-15,1.11716191852906E-13,
1.));
#23691=DIRECTION('',(-8.57516739673986E-14,1.,-1.14312768470149E-13));
#23692=DIRECTION('center_axis',(8.72635297355373E-14,-1.,1.11716191852906E-13));
#23693=DIRECTION('ref_axis',(-1.77809156287629E-15,-1.11716191852907E-13,
-1.));
#23694=DIRECTION('',(8.87753855036761E-14,-1.,1.14312768470149E-13));
#23695=DIRECTION('center_axis',(1.00393149750153E-26,-1.1518563880486E-13,
-1.));
#23696=DIRECTION('ref_axis',(-1.,-8.72635297355373E-14,1.219044193949E-29));
#23697=DIRECTION('center_axis',(9.74874922969709E-27,-1.11716191852906E-13,
-1.));
#23698=DIRECTION('ref_axis',(8.73144149574993E-14,-1.,1.11716191852906E-13));
#23699=DIRECTION('center_axis',(9.74874922969709E-27,-1.11716191852906E-13,
-1.));
#23700=DIRECTION('ref_axis',(8.73144149574993E-14,-1.,1.11716191852906E-13));
#23701=DIRECTION('center_axis',(-1.00515054169548E-26,1.1518563880486E-13,
1.));
#23702=DIRECTION('ref_axis',(-8.72635297355373E-14,1.,-1.1518563880486E-13));
#23703=DIRECTION('center_axis',(1.00515054169548E-26,-1.1518563880486E-13,
-1.));
#23704=DIRECTION('ref_axis',(8.72635297355373E-14,-1.,1.1518563880486E-13));
#23705=DIRECTION('center_axis',(1.00515054169548E-26,-1.1518563880486E-13,
-1.));
#23706=DIRECTION('ref_axis',(8.72635297355373E-14,-1.,1.1518563880486E-13));
#23707=DIRECTION('center_axis',(1.00515054169548E-26,-1.1518563880486E-13,
-1.));
#23708=DIRECTION('ref_axis',(8.72635297355373E-14,-1.,1.1518563880486E-13));
#23709=DIRECTION('center_axis',(1.00515054169548E-26,-1.1518563880486E-13,
-1.));
#23710=DIRECTION('ref_axis',(8.72635297355373E-14,-1.,1.1518563880486E-13));
#23711=DIRECTION('center_axis',(0.868162779192246,0.38268343239671,0.315985410097158));
#23712=DIRECTION('ref_axis',(-0.0151045175936891,0.656788415924971,-0.753923623621802));
#23713=DIRECTION('center_axis',(-0.868162779195953,-0.359604797490619,-0.342020143325637));
#23714=DIRECTION('ref_axis',(0.0151045173766889,0.669702935899703,-0.742475475151965));
#23715=DIRECTION('center_axis',(-0.868162779192246,-0.38268343239671,-0.315985410097158));
#23716=DIRECTION('ref_axis',(0.403349423721026,-0.915046032931631,1.05237388736238E-13));
#23717=DIRECTION('center_axis',(0.868162779192245,0.38268343239671,0.315985410097158));
#23718=DIRECTION('ref_axis',(0.403349423721026,-0.915046032931631,1.05414319346039E-13));
#23719=DIRECTION('',(0.496049637005668,-0.649755621195856,-0.575979505148345));
#23720=DIRECTION('',(0.496049637005668,-0.649755621195843,-0.57597950514836));
#23721=DIRECTION('center_axis',(1.,8.72635297355373E-14,0.));
#23722=DIRECTION('ref_axis',(8.72635297355373E-14,-1.,1.1518563880486E-13));
#23723=DIRECTION('',(4.36317648660808E-14,-0.499999999980658,0.866025403795606));
#23724=DIRECTION('',(-4.36317648660983E-14,0.499999999980858,0.86602540379549));
#23725=DIRECTION('',(-8.72635297355373E-14,1.,-1.1518563880486E-13));
#23726=DIRECTION('',(-4.36317648660808E-14,0.499999999980658,-0.866025403795606));
#23727=DIRECTION('',(4.36317648660983E-14,-0.499999999980858,-0.86602540379549));
#23728=DIRECTION('',(8.72635297355373E-14,-1.,1.1518563880486E-13));
#23729=DIRECTION('center_axis',(-8.72635297355373E-14,1.,-1.11694157466017E-13));
#23730=DIRECTION('ref_axis',(9.74682643132155E-27,-1.11694157466017E-13,
-1.));
#23731=DIRECTION('',(0.5,-5.61219244883788E-14,-0.866025403784439));
#23732=DIRECTION('',(-0.5,-1.43385454223916E-13,-0.866025403784438));
#23733=DIRECTION('',(-1.,-8.72635297355372E-14,1.20185167898972E-15));
#23734=DIRECTION('',(-0.5,5.61219244883789E-14,0.866025403784439));
#23735=DIRECTION('',(0.5,1.43385454223916E-13,0.866025403784439));
#23736=DIRECTION('',(1.,8.72635297355373E-14,-1.21904419394898E-29));
#23737=DIRECTION('center_axis',(-8.72635297355373E-14,1.,-1.11694157466017E-13));
#23738=DIRECTION('ref_axis',(9.74682643132155E-27,-1.11694157466017E-13,
-1.));
#23739=DIRECTION('',(0.5,-5.61219244883789E-14,-0.866025403784439));
#23740=DIRECTION('',(-0.5,-1.43385454223916E-13,-0.866025403784438));
#23741=DIRECTION('',(-1.,-8.72635297355373E-14,0.));
#23742=DIRECTION('',(-0.499999999999999,5.6121924488379E-14,0.866025403784439));
#23743=DIRECTION('',(0.5,1.43385454223916E-13,0.866025403784438));
#23744=DIRECTION('',(1.,8.72635297355373E-14,-1.21904419394898E-29));
#23745=DIRECTION('center_axis',(1.00393149750153E-26,-1.1518563880486E-13,
-1.));
#23746=DIRECTION('ref_axis',(-1.,-8.72635297355373E-14,1.219044193949E-29));
#23747=DIRECTION('center_axis',(9.74874922969709E-27,-1.11716191852906E-13,
-1.));
#23748=DIRECTION('ref_axis',(8.73144149574993E-14,-1.,1.11716191852906E-13));
#23749=DIRECTION('',(-8.72635297355373E-14,1.,-1.1518563880486E-13));
#23750=DIRECTION('center_axis',(1.,8.72635297355372E-14,-6.60847038467355E-16));
#23751=DIRECTION('ref_axis',(-6.60847038457304E-16,-1.1518563880486E-13,
-1.));
#23752=DIRECTION('',(-8.72635297355373E-14,1.,-1.11694157466017E-13));
#23753=DIRECTION('',(-9.74874922969709E-27,1.11716191852906E-13,1.));
#23754=DIRECTION('center_axis',(-9.74682643132153E-27,1.11694157466017E-13,
1.));
#23755=DIRECTION('ref_axis',(-8.72635297355373E-14,1.,-1.11694157466017E-13));
#23756=DIRECTION('center_axis',(-9.74874922969709E-27,1.11716191852906E-13,
1.));
#23757=DIRECTION('ref_axis',(8.73144149574993E-14,-1.,1.11716191852906E-13));
#23758=DIRECTION('center_axis',(2.47817639435298E-16,-1.1518563880486E-13,
-1.));
#23759=DIRECTION('ref_axis',(-1.,-8.72635297355373E-14,-2.47817639425246E-16));
#23760=DIRECTION('center_axis',(9.74874922969709E-27,-1.11716191852906E-13,
-1.));
#23761=DIRECTION('ref_axis',(8.73144149574993E-14,-1.,1.11716191852906E-13));
#23762=DIRECTION('',(-8.72635297355373E-14,1.,-1.1518563880486E-13));
#23763=DIRECTION('center_axis',(1.,8.72635297355373E-14,0.));
#23764=DIRECTION('ref_axis',(8.72635297355373E-14,-1.,1.1518563880486E-13));
#23765=DIRECTION('',(-8.72635297355373E-14,1.,-1.11694157466017E-13));
#23766=DIRECTION('',(-9.74874922969709E-27,1.11716191852906E-13,1.));
#23767=DIRECTION('center_axis',(-9.74682643132153E-27,1.11694157466017E-13,
1.));
#23768=DIRECTION('ref_axis',(-8.72635297355373E-14,1.,-1.11694157466017E-13));
#23769=DIRECTION('center_axis',(-9.74874922969709E-27,1.11716191852906E-13,
1.));
#23770=DIRECTION('ref_axis',(7.63278329429795E-14,-1.,1.11716191852906E-13));
#23771=DIRECTION('center_axis',(-9.74682643132153E-27,1.11694157466017E-13,
1.));
#23772=DIRECTION('ref_axis',(-8.72635297355373E-14,1.,-1.11694157466017E-13));
#23773=DIRECTION('center_axis',(-9.74874922969709E-27,1.11716191852906E-13,
1.));
#23774=DIRECTION('ref_axis',(8.73144149574993E-14,-1.,1.11716191852906E-13));
#23775=DIRECTION('center_axis',(-9.74874922969709E-27,1.11716191852906E-13,
1.));
#23776=DIRECTION('ref_axis',(8.73144149574993E-14,-1.,1.11716191852906E-13));
#23777=DIRECTION('center_axis',(-9.74682643132153E-27,1.11694157466017E-13,
1.));
#23778=DIRECTION('ref_axis',(-8.72635297355373E-14,1.,-1.11694157466017E-13));
#23779=DIRECTION('center_axis',(-9.74874922969709E-27,1.11716191852906E-13,
1.));
#23780=DIRECTION('ref_axis',(8.73144149574993E-14,-1.,1.11716191852906E-13));
#23781=DIRECTION('',(-8.72635297355373E-14,1.,-1.1518563880486E-13));
#23782=DIRECTION('center_axis',(-1.,-8.72635297355373E-14,-1.65211759616839E-16));
#23783=DIRECTION('ref_axis',(-1.65211759626891E-16,1.1518563880486E-13,
1.));
#23784=DIRECTION('',(-8.72635297355373E-14,1.,-1.1518563880486E-13));
#23785=DIRECTION('',(9.74874922969709E-27,-1.11716191852906E-13,-1.));
#23786=DIRECTION('center_axis',(2.47817639435298E-16,-1.1518563880486E-13,
-1.));
#23787=DIRECTION('ref_axis',(-1.,-8.72635297355373E-14,-2.47817639425246E-16));
#23788=DIRECTION('center_axis',(9.74874922969709E-27,-1.11716191852906E-13,
-1.));
#23789=DIRECTION('ref_axis',(8.73144149574993E-14,-1.,1.11716191852906E-13));
#23790=DIRECTION('center_axis',(-9.74682643132153E-27,1.11694157466017E-13,
1.));
#23791=DIRECTION('ref_axis',(-8.72635297355373E-14,1.,-1.11694157466017E-13));
#23792=DIRECTION('center_axis',(-9.74874922969709E-27,1.11716191852906E-13,
1.));
#23793=DIRECTION('ref_axis',(8.73144149574993E-14,-1.,1.11716191852906E-13));
#23794=DIRECTION('',(-8.72635297355373E-14,1.,-1.1518563880486E-13));
#23795=DIRECTION('center_axis',(-1.,-8.72635297355374E-14,-6.60847038467355E-16));
#23796=DIRECTION('ref_axis',(-6.60847038477406E-16,1.1518563880486E-13,
1.));
#23797=DIRECTION('',(-8.72635297355373E-14,1.,-1.1518563880486E-13));
#23798=DIRECTION('',(9.74874922969709E-27,-1.11716191852906E-13,-1.));
#23799=DIRECTION('center_axis',(1.00393149750153E-26,-1.1518563880486E-13,
-1.));
#23800=DIRECTION('ref_axis',(-1.,-8.72635297355373E-14,1.219044193949E-29));
#23801=DIRECTION('center_axis',(9.74874922969709E-27,-1.11716191852906E-13,
-1.));
#23802=DIRECTION('ref_axis',(8.73144149574993E-14,-1.,1.11716191852906E-13));
#23803=DIRECTION('center_axis',(0.866025403784439,1.97253548418657E-14,
-0.5));
#23804=DIRECTION('ref_axis',(-0.5,-1.43385454223916E-13,-0.866025403784439));
#23805=DIRECTION('',(8.57516739673986E-14,-1.,1.14312768470149E-13));
#23806=DIRECTION('',(-0.5,-1.40981750865937E-13,-0.866025403784439));
#23807=DIRECTION('',(-8.72635297355373E-14,1.,-1.1518563880486E-13));
#23808=DIRECTION('center_axis',(0.866025403784439,1.31419512307882E-13,
0.5));
#23809=DIRECTION('ref_axis',(0.5,-5.61219244883788E-14,-0.866025403784439));
#23810=DIRECTION('',(8.72635297355373E-14,-1.,1.11694157466017E-13));
#23811=DIRECTION('',(0.5,-5.37182211303994E-14,-0.866025403784439));
#23812=DIRECTION('center_axis',(-9.74682643132153E-27,1.11694157466017E-13,
1.));
#23813=DIRECTION('ref_axis',(-8.72635297355373E-14,1.,-1.11694157466017E-13));
#23814=DIRECTION('',(8.87753855036761E-14,-1.,1.14312768470149E-13));
#23815=DIRECTION('',(1.,8.72635297355373E-14,0.));
#23816=DIRECTION('center_axis',(-0.866025403784439,-1.97253548418657E-14,
0.5));
#23817=DIRECTION('ref_axis',(0.5,1.43385454223916E-13,0.866025403784439));
#23818=DIRECTION('',(8.57516739673986E-14,-1.,1.14312768470149E-13));
#23819=DIRECTION('',(0.5,1.40981750865937E-13,0.866025403784438));
#23820=DIRECTION('center_axis',(-0.866025403784439,-1.31419512307882E-13,
-0.5));
#23821=DIRECTION('ref_axis',(-0.5,5.61219244883788E-14,0.866025403784439));
#23822=DIRECTION('',(8.72635297355373E-14,-1.,1.1518563880486E-13));
#23823=DIRECTION('',(-0.5,5.37182211303995E-14,0.866025403784439));
#23824=DIRECTION('center_axis',(1.00393149750153E-26,-1.1518563880486E-13,
-1.));
#23825=DIRECTION('ref_axis',(-1.,-8.72635297355373E-14,1.219044193949E-29));
#23826=DIRECTION('',(-1.,-8.72635297355373E-14,0.));
#23827=DIRECTION('center_axis',(0.866025403784439,1.97253548418657E-14,
-0.5));
#23828=DIRECTION('ref_axis',(-0.5,-1.43385454223916E-13,-0.866025403784439));
#23829=DIRECTION('center_axis',(-0.866025403784486,6.32642106711312E-14,
0.499999999999918));
#23830=DIRECTION('ref_axis',(0.499999999999918,-1.40512606311845E-10,0.866025403784486));
#23831=DIRECTION('',(-0.500000000000001,-1.43385454223916E-13,-0.866025403784438));
#23832=DIRECTION('',(8.72635297355373E-14,-1.,1.11716191852906E-13));
#23833=DIRECTION('center_axis',(-8.72635297355373E-14,1.,-1.11716191852906E-13));
#23834=DIRECTION('ref_axis',(6.05512374515455E-29,-1.11716191852906E-13,
-1.));
#23835=DIRECTION('center_axis',(-8.72635297355373E-14,1.,-1.11716191852906E-13));
#23836=DIRECTION('ref_axis',(6.05512374515455E-29,-1.11716191852906E-13,
-1.));
#23837=DIRECTION('center_axis',(8.72635297355373E-14,-1.,1.1518563880486E-13));
#23838=DIRECTION('ref_axis',(-1.,-8.72635297355373E-14,-1.43492962746861E-42));
#23839=DIRECTION('',(-0.5,5.61219244883788E-14,0.866025403784439));
#23840=DIRECTION('center_axis',(-8.72635297355373E-14,1.,-1.11716191852906E-13));
#23841=DIRECTION('ref_axis',(6.05512374515455E-29,-1.11716191852906E-13,
-1.));
#23842=DIRECTION('',(1.,8.69744091562078E-14,3.23084885458356E-29));
#23843=DIRECTION('center_axis',(-8.72635297355373E-14,1.,-1.11716191852906E-13));
#23844=DIRECTION('ref_axis',(6.05512374515455E-29,-1.11716191852906E-13,
-1.));
#23845=DIRECTION('',(8.57516739673986E-14,-1.,1.14312768470149E-13));
#23846=DIRECTION('center_axis',(-0.866025403784439,-1.31419512307882E-13,
-0.5));
#23847=DIRECTION('ref_axis',(-0.5,5.61219244883788E-14,0.866025403784439));
#23848=DIRECTION('center_axis',(0.866025403784523,-8.63609033881368E-13,
0.499999999999854));
#23849=DIRECTION('ref_axis',(0.499999999999854,4.79670877767529E-10,-0.866025403784523));
#23850=DIRECTION('center_axis',(0.866025403784434,1.17391797327623E-13,
0.500000000000008));
#23851=DIRECTION('ref_axis',(0.500000000000008,-2.53120997629797E-11,-0.866025403784434));
#23852=DIRECTION('center_axis',(-8.72635297355373E-14,1.,-1.11694157466017E-13));
#23853=DIRECTION('ref_axis',(9.74682643132155E-27,-1.11694157466017E-13,
-1.));
#23854=DIRECTION('',(0.5,-5.61219244883789E-14,-0.866025403784439));
#23855=DIRECTION('',(-0.5,-1.43385454223916E-13,-0.866025403784439));
#23856=DIRECTION('',(-1.,-8.72635297355373E-14,0.));
#23857=DIRECTION('',(-0.5,5.61219244883788E-14,0.866025403784439));
#23858=DIRECTION('',(0.5,1.43385454223916E-13,0.866025403784439));
#23859=DIRECTION('',(1.,8.72635297355373E-14,-1.21904419394898E-29));
#23860=DIRECTION('center_axis',(-8.72635297355373E-14,1.,-1.11694157466017E-13));
#23861=DIRECTION('ref_axis',(9.74682643132155E-27,-1.11694157466017E-13,
-1.));
#23862=DIRECTION('',(0.5,-5.61219244883788E-14,-0.866025403784439));
#23863=DIRECTION('',(-0.5,-1.43385454223916E-13,-0.866025403784438));
#23864=DIRECTION('',(-1.,-8.72635297355373E-14,0.));
#23865=DIRECTION('',(-0.499999999999999,5.6121924488379E-14,0.866025403784439));
#23866=DIRECTION('',(0.5,1.43385454223916E-13,0.866025403784439));
#23867=DIRECTION('',(1.,8.72635297355373E-14,-1.21904419394898E-29));
#23868=DIRECTION('center_axis',(1.,8.72635297355373E-14,0.));
#23869=DIRECTION('ref_axis',(8.72635297355373E-14,-1.,1.1518563880486E-13));
#23870=DIRECTION('',(4.36317648660983E-14,-0.499999999980858,-0.86602540379549));
#23871=DIRECTION('',(-4.36317648660808E-14,0.499999999980658,-0.866025403795606));
#23872=DIRECTION('',(-8.72635297355373E-14,1.,-1.1518563880486E-13));
#23873=DIRECTION('',(-4.36317648660983E-14,0.499999999980858,0.86602540379549));
#23874=DIRECTION('',(4.36317648660808E-14,-0.499999999980658,0.866025403795606));
#23875=DIRECTION('',(8.72635297355373E-14,-1.,1.1518563880486E-13));
#23876=DIRECTION('center_axis',(0.382683432365171,-0.923879532511253,1.06417654131048E-13));
#23877=DIRECTION('ref_axis',(-0.923879532511253,-0.382683432365171,4.40796356170094E-14));
#23878=DIRECTION('',(-0.923879532511252,-0.382683432365173,4.40796356170097E-14));
#23879=DIRECTION('',(0.315985410125154,0.130885442385788,-0.939692620785922));
#23880=DIRECTION('center_axis',(0.868162779195958,0.359604797490614,0.34202014332563));
#23881=DIRECTION('ref_axis',(0.382683432365172,-0.923879532511253,1.06407127951475E-13));
#23882=DIRECTION('',(-0.382683432365169,0.923879532511254,-1.06417654131048E-13));
#23883=DIRECTION('',(0.315985410125162,0.130885442385792,-0.939692620785919));
#23884=DIRECTION('center_axis',(0.382683432365171,-0.923879532511253,1.06417654131048E-13));
#23885=DIRECTION('ref_axis',(-0.923879532511253,-0.382683432365171,4.40796356170094E-14));
#23886=DIRECTION('',(0.923879532511254,0.382683432365169,-4.40796356170092E-14));
#23887=DIRECTION('center_axis',(1.00515054169548E-26,-1.1518563880486E-13,
-1.));
#23888=DIRECTION('ref_axis',(8.72635297355373E-14,-1.,1.1518563880486E-13));
#23889=DIRECTION('',(0.866025403795592,-0.499999999980683,5.75928194002136E-14));
#23890=DIRECTION('',(0.866025403795504,0.499999999980834,-5.75928194002136E-14));
#23891=DIRECTION('',(-8.72635297355373E-14,1.,-1.1518563880486E-13));
#23892=DIRECTION('',(-0.866025403795591,0.499999999980683,-5.75928194002135E-14));
#23893=DIRECTION('',(-0.866025403795504,-0.499999999980834,5.75928194002136E-14));
#23894=DIRECTION('',(8.72635297355373E-14,-1.,1.1518563880486E-13));
#23895=DIRECTION('center_axis',(1.,8.72635297355373E-14,0.));
#23896=DIRECTION('ref_axis',(8.72635297355373E-14,-1.,1.1518563880486E-13));
#23897=DIRECTION('',(4.36317648660808E-14,-0.499999999980658,0.866025403795606));
#23898=DIRECTION('',(-4.36317648660983E-14,0.499999999980858,0.86602540379549));
#23899=DIRECTION('',(-8.72635297355373E-14,1.,-1.1518563880486E-13));
#23900=DIRECTION('',(-4.36317648660808E-14,0.499999999980658,-0.866025403795606));
#23901=DIRECTION('',(4.36317648660983E-14,-0.499999999980858,-0.86602540379549));
#23902=DIRECTION('',(8.72635297355373E-14,-1.,1.1518563880486E-13));
#23903=DIRECTION('center_axis',(1.00515054169548E-26,-1.1518563880486E-13,
-1.));
#23904=DIRECTION('ref_axis',(8.72635297355373E-14,-1.,1.1518563880486E-13));
#23905=DIRECTION('',(1.,8.72635297355373E-14,0.));
#23906=DIRECTION('',(-1.,-8.72635297355373E-14,0.));
#23907=DIRECTION('',(-8.72635297355373E-14,1.,-1.1518563880486E-13));
#23908=DIRECTION('center_axis',(-7.55724335758385E-14,0.86602540379549,
-0.499999999980858));
#23909=DIRECTION('ref_axis',(4.36317648660983E-14,-0.499999999980858,-0.86602540379549));
#23910=DIRECTION('',(-1.,-8.72635297355373E-14,0.));
#23911=DIRECTION('',(-4.36317648660983E-14,0.499999999980859,0.86602540379549));
#23912=DIRECTION('center_axis',(-7.55724335758485E-14,0.866025403795606,
0.499999999980658));
#23913=DIRECTION('ref_axis',(-4.36317648660808E-14,0.499999999980658,-0.866025403795606));
#23914=DIRECTION('',(-1.,-8.72635297355373E-14,0.));
#23915=DIRECTION('',(4.36317648660808E-14,-0.499999999980657,0.866025403795606));
#23916=DIRECTION('center_axis',(-1.00515054169548E-26,1.1518563880486E-13,
1.));
#23917=DIRECTION('ref_axis',(-8.72635297355373E-14,1.,-1.1518563880486E-13));
#23918=DIRECTION('',(-1.,-8.72635297355373E-14,0.));
#23919=DIRECTION('',(8.72635297355373E-14,-1.,1.1518563880486E-13));
#23920=DIRECTION('center_axis',(7.55724335758385E-14,-0.86602540379549,
0.499999999980858));
#23921=DIRECTION('ref_axis',(-4.36317648660983E-14,0.499999999980858,0.86602540379549));
#23922=DIRECTION('',(-1.,-8.72635297355373E-14,0.));
#23923=DIRECTION('',(4.36317648660981E-14,-0.499999999980857,-0.866025403795491));
#23924=DIRECTION('center_axis',(7.55724335758485E-14,-0.866025403795606,
-0.499999999980658));
#23925=DIRECTION('ref_axis',(4.36317648660808E-14,-0.499999999980658,0.866025403795606));
#23926=DIRECTION('',(-4.36317648660809E-14,0.49999999998066,-0.866025403795605));
#23927=DIRECTION('center_axis',(-1.,-8.72635297355374E-14,-1.15648231731787E-15));
#23928=DIRECTION('ref_axis',(-1.15648231732792E-15,1.1518563880486E-13,
1.));
#23929=DIRECTION('',(-8.72635297355373E-14,1.,-1.11716191852906E-13));
#23930=DIRECTION('center_axis',(1.,8.69744091562078E-14,3.23084885458356E-29));
#23931=DIRECTION('ref_axis',(8.69744091562078E-14,-1.,1.15648231731787E-13));
#23932=DIRECTION('',(-1.00515054169548E-26,1.1518563880486E-13,1.));
#23933=DIRECTION('center_axis',(-8.72635297355373E-14,1.,-1.11716191852906E-13));
#23934=DIRECTION('ref_axis',(-6.05512374515239E-29,-1.11716191852906E-13,
-1.));
#23935=DIRECTION('',(8.72635297355373E-14,-1.,1.1518563880486E-13));
#23936=DIRECTION('center_axis',(-8.72635297355373E-14,1.,-1.11716191852906E-13));
#23937=DIRECTION('ref_axis',(-6.05512374515239E-29,-1.11716191852906E-13,
-1.));
#23938=DIRECTION('center_axis',(8.72635297355373E-14,-1.,1.11716191852906E-13));
#23939=DIRECTION('ref_axis',(-6.05512374515239E-29,-1.11716191852906E-13,
-1.));
#23940=DIRECTION('center_axis',(1.00393149750153E-26,-1.1518563880486E-13,
-1.));
#23941=DIRECTION('ref_axis',(-1.,-8.72635297355373E-14,1.219044193949E-29));
#23942=DIRECTION('',(-1.,-8.72635297355373E-14,-1.40416384211369E-42));
#23943=DIRECTION('',(-8.72635297355373E-14,1.,-1.1518563880486E-13));
#23944=DIRECTION('center_axis',(-9.56709551734248E-27,1.09634523681734E-13,
1.));
#23945=DIRECTION('ref_axis',(8.88178419700124E-14,-1.,1.09634523681734E-13));
#23946=DIRECTION('',(1.,8.69608263101991E-14,3.48670874160052E-29));
#23947=DIRECTION('center_axis',(0.866025403784439,1.97253548418658E-14,
-0.5));
#23948=DIRECTION('ref_axis',(-0.5,-1.43385454223916E-13,-0.866025403784439));
#23949=DIRECTION('',(8.57516739673986E-14,-1.,1.14312768470149E-13));
#23950=DIRECTION('',(0.499999999999999,1.43385454223916E-13,0.866025403784439));
#23951=DIRECTION('',(-8.72635297355373E-14,1.,-1.1518563880486E-13));
#23952=DIRECTION('center_axis',(1.00393149750153E-26,-1.1518563880486E-13,
-1.));
#23953=DIRECTION('ref_axis',(-1.,-8.72635297355373E-14,1.219044193949E-29));
#23954=DIRECTION('',(1.,8.72635297355373E-14,1.40416384211369E-42));
#23955=DIRECTION('',(-8.57516739673986E-14,1.,-1.14312768470149E-13));
#23956=DIRECTION('center_axis',(-0.866025403784439,-1.31419512307882E-13,
-0.5));
#23957=DIRECTION('ref_axis',(-0.5,5.61219244883788E-14,0.866025403784439));
#23958=DIRECTION('',(0.5,-5.61219244883788E-14,-0.866025403784439));
#23959=DIRECTION('',(-8.8775385503676E-14,1.,-1.14312768470149E-13));
#23960=DIRECTION('center_axis',(-0.866025403784438,-1.97253548418655E-14,
0.5));
#23961=DIRECTION('ref_axis',(0.5,1.43385454223916E-13,0.866025403784438));
#23962=DIRECTION('',(-0.499999999999999,-1.43385454223916E-13,-0.866025403784439));
#23963=DIRECTION('',(-8.72635297355373E-14,1.,-1.11694157466017E-13));
#23964=DIRECTION('center_axis',(1.20185167897997E-15,1.11694157466017E-13,
1.));
#23965=DIRECTION('ref_axis',(-8.72635297355373E-14,1.,-1.11694157466017E-13));
#23966=DIRECTION('',(-1.,-8.72635297355373E-14,-1.40416384211369E-42));
#23967=DIRECTION('',(-8.57516739673986E-14,1.,-1.14312768470149E-13));
#23968=DIRECTION('center_axis',(0.866025403784439,1.31419512307882E-13,
0.5));
#23969=DIRECTION('ref_axis',(0.5,-5.61219244883789E-14,-0.866025403784439));
#23970=DIRECTION('',(-0.499999999999983,5.61219244883814E-14,0.866025403784448));
#23971=DIRECTION('center_axis',(-8.72635297355373E-14,1.,-1.11716191852906E-13));
#23972=DIRECTION('ref_axis',(-6.05512374515382E-29,-1.11716191852906E-13,
-1.));
#23973=DIRECTION('',(8.72635297355373E-14,-1.,1.1518563880486E-13));
#23974=DIRECTION('center_axis',(-8.72635297355373E-14,1.,-1.11716191852906E-13));
#23975=DIRECTION('ref_axis',(-6.05512374515382E-29,-1.11716191852906E-13,
-1.));
#23976=DIRECTION('',(-8.72635297355373E-14,1.,-1.11694157466017E-13));
#23977=DIRECTION('center_axis',(-8.72635297355373E-14,1.,-1.11716191852906E-13));
#23978=DIRECTION('ref_axis',(-6.05512374515382E-29,-1.11716191852906E-13,
-1.));
#23979=DIRECTION('center_axis',(-9.74682643132153E-27,1.11694157466017E-13,
1.));
#23980=DIRECTION('ref_axis',(-8.72635297355373E-14,1.,-1.11694157466017E-13));
#23981=DIRECTION('',(-1.,-8.69608263101991E-14,-3.48670874160052E-29));
#23982=DIRECTION('center_axis',(9.56709551734248E-27,-1.09634523681734E-13,
-1.));
#23983=DIRECTION('ref_axis',(8.88178419700124E-14,-1.,1.09634523681734E-13));
#23984=DIRECTION('',(8.72635297355373E-14,-1.,1.11694157466017E-13));
#23985=DIRECTION('',(-1.,-8.72635297355373E-14,0.));
#23986=DIRECTION('center_axis',(0.866025403784438,1.97253548418655E-14,
-0.5));
#23987=DIRECTION('ref_axis',(-0.5,-1.43385454223916E-13,-0.866025403784438));
#23988=DIRECTION('',(8.57516739673986E-14,-1.,1.14312768470149E-13));
#23989=DIRECTION('',(-0.499999999999999,-1.40981750865936E-13,-0.866025403784439));
#23990=DIRECTION('',(-8.72635297355373E-14,1.,-1.1518563880486E-13));
#23991=DIRECTION('center_axis',(0.866025403784439,1.31419512307882E-13,
0.5));
#23992=DIRECTION('ref_axis',(0.5,-5.6121924488379E-14,-0.866025403784439));
#23993=DIRECTION('',(8.72635297355373E-14,-1.,1.11694157466017E-13));
#23994=DIRECTION('',(0.499999999999999,-5.37182211303998E-14,-0.866025403784439));
#23995=DIRECTION('center_axis',(-9.74682643132153E-27,1.11694157466017E-13,
1.));
#23996=DIRECTION('ref_axis',(-8.72635297355373E-14,1.,-1.11694157466017E-13));
#23997=DIRECTION('',(8.8775385503676E-14,-1.,1.14312768470149E-13));
#23998=DIRECTION('',(1.,8.72635297355373E-14,0.));
#23999=DIRECTION('center_axis',(-0.866025403784438,-1.97253548418655E-14,
0.5));
#24000=DIRECTION('ref_axis',(0.5,1.43385454223916E-13,0.866025403784438));
#24001=DIRECTION('',(8.57516739673986E-14,-1.,1.14312768470149E-13));
#24002=DIRECTION('',(0.499999999999999,1.40981750865936E-13,0.866025403784439));
#24003=DIRECTION('center_axis',(-0.866025403784439,-1.31419512307882E-13,
-0.5));
#24004=DIRECTION('ref_axis',(-0.5,5.61219244883789E-14,0.866025403784439));
#24005=DIRECTION('',(8.72635297355373E-14,-1.,1.1518563880486E-13));
#24006=DIRECTION('',(-0.499999999999999,5.37182211303996E-14,0.866025403784439));
#24007=DIRECTION('center_axis',(1.00393149750153E-26,-1.1518563880486E-13,
-1.));
#24008=DIRECTION('ref_axis',(-1.,-8.72635297355373E-14,1.219044193949E-29));
#24009=DIRECTION('',(-1.,-8.72635297355373E-14,0.));
#24010=DIRECTION('center_axis',(9.74874922969709E-27,-1.11716191852906E-13,
-1.));
#24011=DIRECTION('ref_axis',(-0.178927238307379,0.983862309163073,-1.09913350487307E-13));
#24012=DIRECTION('',(1.00515054169548E-26,-1.1518563880486E-13,-1.));
#24013=DIRECTION('center_axis',(9.74874922969709E-27,-1.11716191852906E-13,
-1.));
#24014=DIRECTION('ref_axis',(-8.65487012177139E-14,1.,-1.11716191852906E-13));
#24015=DIRECTION('center_axis',(9.74874922969709E-27,-1.11716191852906E-13,
-1.));
#24016=DIRECTION('ref_axis',(-8.61046120078639E-14,1.,-1.11716191852906E-13));
#24017=DIRECTION('center_axis',(-0.866025403784341,-1.24346714277096E-12,
0.50000000000017));
#24018=DIRECTION('ref_axis',(0.50000000000017,5.32565284059118E-10,0.866025403784341));
#24019=DIRECTION('center_axis',(-0.866025403784439,-1.97253548418657E-14,
0.5));
#24020=DIRECTION('ref_axis',(0.5,1.43385454223916E-13,0.866025403784439));
#24021=DIRECTION('',(8.72635297355373E-14,-1.,1.11716191852906E-13));
#24022=DIRECTION('center_axis',(0.866025403784439,2.16945826683511E-14,
-0.5));
#24023=DIRECTION('ref_axis',(0.5,-5.04270596729575E-12,0.866025403784439));
#24024=DIRECTION('',(-0.499999999999999,-1.40981750865936E-13,-0.866025403784439));
#24025=DIRECTION('center_axis',(-8.72635297355373E-14,1.,-1.11716191852906E-13));
#24026=DIRECTION('ref_axis',(6.05512374515455E-29,-1.11716191852906E-13,
-1.));
#24027=DIRECTION('center_axis',(8.72635297355373E-14,-1.,1.11716191852906E-13));
#24028=DIRECTION('ref_axis',(8.67361737988409E-15,-1.11716191852906E-13,
-1.));
#24029=DIRECTION('center_axis',(-8.72635297355373E-14,1.,-1.11694157466017E-13));
#24030=DIRECTION('ref_axis',(9.74682643132155E-27,-1.11694157466017E-13,
-1.));
#24031=DIRECTION('center_axis',(-8.72635297355373E-14,1.,-1.11716191852906E-13));
#24032=DIRECTION('ref_axis',(6.05512374515455E-29,-1.11716191852906E-13,
-1.));
#24033=DIRECTION('',(-1.,-8.69744091562078E-14,-3.22930795142916E-29));
#24034=DIRECTION('',(0.5,-5.61219244883788E-14,-0.866025403784439));
#24035=DIRECTION('center_axis',(-8.72635297355373E-14,1.,-1.11716191852906E-13));
#24036=DIRECTION('ref_axis',(6.05512374515455E-29,-1.11716191852906E-13,
-1.));
#24037=DIRECTION('',(8.57516739673986E-14,-1.,1.14312768470149E-13));
#24038=DIRECTION('center_axis',(0.866025403784439,1.31419512307882E-13,
0.5));
#24039=DIRECTION('ref_axis',(0.5,-5.61219244883788E-14,-0.866025403784439));
#24040=DIRECTION('center_axis',(-0.866025403784486,-5.29905354331503E-14,
-0.499999999999918));
#24041=DIRECTION('ref_axis',(0.499999999999918,-1.6531018130455E-11,-0.866025403784486));
#24042=DIRECTION('center_axis',(9.74874922969709E-27,-1.11716191852906E-13,
-1.));
#24043=DIRECTION('ref_axis',(-8.56605227980138E-14,1.,-1.11716191852906E-13));
#24044=DIRECTION('center_axis',(9.74874922969709E-27,-1.11716191852906E-13,
-1.));
#24045=DIRECTION('ref_axis',(-8.56605227980138E-14,1.,-1.11716191852906E-13));
#24046=DIRECTION('center_axis',(9.74874922969709E-27,-1.11716191852906E-13,
-1.));
#24047=DIRECTION('ref_axis',(0.170744263336185,0.985315379225243,-1.10075681941145E-13));
#24048=DIRECTION('',(-1.00515054169548E-26,1.1518563880486E-13,1.));
#24049=DIRECTION('center_axis',(8.69608263101991E-14,-1.,1.1518563880486E-13));
#24050=DIRECTION('ref_axis',(-1.,-8.69608263101991E-14,-3.48670874160055E-29));
#24051=DIRECTION('',(9.56709551734248E-27,-1.09634523681734E-13,-1.));
#24052=DIRECTION('',(-1.,-8.69744091562078E-14,-3.22930795142916E-29));
#24053=DIRECTION('',(1.,8.69744091562078E-14,3.23084885458356E-29));
#24054=DIRECTION('center_axis',(-1.,-8.72635297355372E-14,1.15648231731787E-15));
#24055=DIRECTION('ref_axis',(1.15648231730782E-15,1.1518563880486E-13,1.));
#24056=DIRECTION('',(9.74682643132155E-27,-1.11694157466017E-13,-1.));
#24057=DIRECTION('center_axis',(1.,8.69744091562078E-14,3.22930795142916E-29));
#24058=DIRECTION('ref_axis',(-8.69744091562078E-14,1.,-1.14491749414469E-13));
#24059=DIRECTION('center_axis',(8.69608263101991E-14,-1.,1.1518563880486E-13));
#24060=DIRECTION('ref_axis',(-1.,-8.69608263101991E-14,-3.48670874160055E-29));
#24061=DIRECTION('',(-1.,-8.72635297355373E-14,0.));
#24062=DIRECTION('',(-9.56709551734248E-27,1.09634523681734E-13,1.));
#24063=DIRECTION('',(1.,8.72635297355373E-14,-1.21904419394898E-29));
#24064=DIRECTION('center_axis',(8.72635297355373E-14,-1.,1.11716191852906E-13));
#24065=DIRECTION('ref_axis',(-6.05512374515239E-29,-1.11716191852906E-13,
-1.));
#24066=DIRECTION('',(1.,8.69744091562078E-14,3.23084885458356E-29));
#24067=DIRECTION('',(-1.,-8.69744091562078E-14,-3.22930795142916E-29));
#24068=DIRECTION('center_axis',(8.72635297355373E-14,-1.,1.11716191852906E-13));
#24069=DIRECTION('ref_axis',(-6.05512374515382E-29,-1.11716191852906E-13,
-1.));
#24070=DIRECTION('center_axis',(1.,8.72635297355372E-14,-1.15648231731787E-15));
#24071=DIRECTION('ref_axis',(-1.15648231730782E-15,-1.1518563880486E-13,
-1.));
#24072=DIRECTION('',(-9.74682643132155E-27,1.11694157466017E-13,1.));
#24073=DIRECTION('center_axis',(-1.,-8.69744091562078E-14,-3.23084885458356E-29));
#24074=DIRECTION('ref_axis',(8.69744091562078E-14,-1.,1.15648231731787E-13));
#24075=DIRECTION('',(8.72635297355373E-14,-1.,1.11716191852906E-13));
#24076=DIRECTION('center_axis',(-8.72635297355373E-14,1.,-1.11716191852906E-13));
#24077=DIRECTION('ref_axis',(-6.05512374515239E-29,-1.11716191852906E-13,
-1.));
#24078=DIRECTION('',(-8.72635297355373E-14,1.,-1.1518563880486E-13));
#24079=DIRECTION('center_axis',(-8.72635297355373E-14,1.,-1.11716191852906E-13));
#24080=DIRECTION('ref_axis',(-6.05512374515239E-29,-1.11716191852906E-13,
-1.));
#24081=DIRECTION('center_axis',(1.00393149750153E-26,-1.1518563880486E-13,
-1.));
#24082=DIRECTION('ref_axis',(-1.,-8.72635297355373E-14,1.219044193949E-29));
#24083=DIRECTION('center_axis',(-9.56709551734248E-27,1.09634523681734E-13,
1.));
#24084=DIRECTION('ref_axis',(8.88178419700124E-14,-1.,1.09634523681734E-13));
#24085=DIRECTION('',(8.72635297355373E-14,-1.,1.1518563880486E-13));
#24086=DIRECTION('',(1.,8.72635297355373E-14,0.));
#24087=DIRECTION('center_axis',(1.,8.69744091562078E-14,3.23084885458356E-29));
#24088=DIRECTION('ref_axis',(8.69744091562078E-14,-1.,1.15648231731787E-13));
#24089=DIRECTION('',(-1.,-8.72635297355373E-14,0.));
#24090=DIRECTION('center_axis',(0.863779089886205,-0.503870701519188,-5.09114224033432E-6));
#24091=DIRECTION('ref_axis',(0.502518782934927,0.861460773419583,0.0732134458752874));
#24092=DIRECTION('',(1.,8.72635297355373E-14,-1.21904419394898E-29));
#24093=DIRECTION('',(1.,8.72635297355373E-14,1.40416384211369E-42));
#24094=DIRECTION('center_axis',(0.866025403784439,1.97253548418657E-14,
-0.5));
#24095=DIRECTION('ref_axis',(-0.5,-1.43385454223916E-13,-0.866025403784439));
#24096=DIRECTION('',(8.57516739673986E-14,-1.,1.14312768470149E-13));
#24097=DIRECTION('',(-0.5,-1.40981750865937E-13,-0.866025403784439));
#24098=DIRECTION('',(-8.72635297355373E-14,1.,-1.1518563880486E-13));
#24099=DIRECTION('center_axis',(0.866025403784439,1.31419512307882E-13,
0.5));
#24100=DIRECTION('ref_axis',(0.5,-5.61219244883788E-14,-0.866025403784439));
#24101=DIRECTION('',(8.72635297355373E-14,-1.,1.11694157466017E-13));
#24102=DIRECTION('',(0.499999999999999,-5.37182211303996E-14,-0.866025403784439));
#24103=DIRECTION('center_axis',(-9.74682643132153E-27,1.11694157466017E-13,
1.));
#24104=DIRECTION('ref_axis',(-8.72635297355373E-14,1.,-1.11694157466017E-13));
#24105=DIRECTION('',(8.87753855036761E-14,-1.,1.14312768470149E-13));
#24106=DIRECTION('',(1.,8.72635297355373E-14,0.));
#24107=DIRECTION('center_axis',(-0.866025403784439,-1.97253548418658E-14,
0.5));
#24108=DIRECTION('ref_axis',(0.5,1.43385454223916E-13,0.866025403784439));
#24109=DIRECTION('',(8.57516739673986E-14,-1.,1.14312768470149E-13));
#24110=DIRECTION('',(0.500000000000008,1.40981750865937E-13,0.866025403784434));
#24111=DIRECTION('center_axis',(-0.866025403784439,-1.31419512307882E-13,
-0.5));
#24112=DIRECTION('ref_axis',(-0.5,5.61219244883789E-14,0.866025403784439));
#24113=DIRECTION('',(8.72635297355373E-14,-1.,1.1518563880486E-13));
#24114=DIRECTION('',(-0.50000000000001,5.37182211303977E-14,0.866025403784433));
#24115=DIRECTION('center_axis',(1.00393149750153E-26,-1.1518563880486E-13,
-1.));
#24116=DIRECTION('ref_axis',(-1.,-8.72635297355373E-14,1.219044193949E-29));
#24117=DIRECTION('',(-1.,-8.72635297355373E-14,0.));
#24118=DIRECTION('center_axis',(1.,8.72635297355374E-14,1.15648231731787E-15));
#24119=DIRECTION('ref_axis',(1.15648231732792E-15,-1.1518563880486E-13,
-1.));
#24120=DIRECTION('',(-8.72635297355373E-14,1.,-1.11716191852906E-13));
#24121=DIRECTION('center_axis',(-1.,-8.69744091562078E-14,-3.22930795142916E-29));
#24122=DIRECTION('ref_axis',(-8.69744091562078E-14,1.,-1.15648231731787E-13));
#24123=DIRECTION('',(1.00515054169548E-26,-1.1518563880486E-13,-1.));
#24124=DIRECTION('center_axis',(-8.72635297355373E-14,1.,-1.11716191852906E-13));
#24125=DIRECTION('ref_axis',(-6.05512374515382E-29,-1.11716191852906E-13,
-1.));
#24126=DIRECTION('',(8.72635297355373E-14,-1.,1.11694157466017E-13));
#24127=DIRECTION('center_axis',(8.72635297355373E-14,-1.,1.11716191852906E-13));
#24128=DIRECTION('ref_axis',(-6.05512374515382E-29,-1.11716191852906E-13,
-1.));
#24129=DIRECTION('center_axis',(-9.74682643132153E-27,1.11694157466017E-13,
1.));
#24130=DIRECTION('ref_axis',(-8.72635297355373E-14,1.,-1.11694157466017E-13));
#24131=DIRECTION('',(1.,8.72635297355373E-14,1.40416384211369E-42));
#24132=DIRECTION('',(-8.72635297355373E-14,1.,-1.11694157466017E-13));
#24133=DIRECTION('center_axis',(9.56709551734248E-27,-1.09634523681734E-13,
-1.));
#24134=DIRECTION('ref_axis',(8.88178419700124E-14,-1.,1.09634523681734E-13));
#24135=DIRECTION('center_axis',(0.866025403784439,1.97253548418658E-14,
-0.5));
#24136=DIRECTION('ref_axis',(-0.5,-1.43385454223916E-13,-0.866025403784439));
#24137=DIRECTION('',(8.57516739673986E-14,-1.,1.14312768470149E-13));
#24138=DIRECTION('',(0.499999999999999,1.43385454223916E-13,0.866025403784439));
#24139=DIRECTION('',(-8.72635297355373E-14,1.,-1.1518563880486E-13));
#24140=DIRECTION('center_axis',(1.00393149750153E-26,-1.1518563880486E-13,
-1.));
#24141=DIRECTION('ref_axis',(-1.,-8.72635297355373E-14,1.219044193949E-29));
#24142=DIRECTION('',(1.,8.72635297355373E-14,1.40416384211369E-42));
#24143=DIRECTION('',(-8.57516739673986E-14,1.,-1.14312768470149E-13));
#24144=DIRECTION('center_axis',(-0.866025403784439,-1.31419512307882E-13,
-0.5));
#24145=DIRECTION('ref_axis',(-0.5,5.61219244883788E-14,0.866025403784439));
#24146=DIRECTION('',(0.500000000000008,-5.61219244883775E-14,-0.866025403784434));
#24147=DIRECTION('',(-8.8775385503676E-14,1.,-1.14312768470149E-13));
#24148=DIRECTION('center_axis',(-0.866025403784438,-1.97253548418655E-14,
0.5));
#24149=DIRECTION('ref_axis',(0.5,1.43385454223916E-13,0.866025403784438));
#24150=DIRECTION('',(-0.500000000000009,-1.43385454223916E-13,-0.866025403784433));
#24151=DIRECTION('',(-8.72635297355373E-14,1.,-1.11694157466017E-13));
#24152=DIRECTION('center_axis',(-9.74682643132153E-27,1.11694157466017E-13,
1.));
#24153=DIRECTION('ref_axis',(-8.72635297355373E-14,1.,-1.11694157466017E-13));
#24154=DIRECTION('',(-1.,-8.72635297355373E-14,-1.40416384211369E-42));
#24155=DIRECTION('',(-8.57516739673986E-14,1.,-1.14312768470149E-13));
#24156=DIRECTION('center_axis',(0.866025403784439,1.31419512307882E-13,
0.5));
#24157=DIRECTION('ref_axis',(0.5,-5.6121924488379E-14,-0.866025403784439));
#24158=DIRECTION('',(-0.499999999999999,5.6121924488379E-14,0.866025403784439));
#24159=DIRECTION('center_axis',(1.00515054169548E-26,-1.1518563880486E-13,
-1.));
#24160=DIRECTION('ref_axis',(8.72635297355373E-14,-1.,1.1518563880486E-13));
#24161=DIRECTION('',(-1.,-8.72635297355373E-14,0.));
#24162=DIRECTION('',(1.,8.72635297355373E-14,0.));
#24163=DIRECTION('',(8.72635297355373E-14,-1.,1.1518563880486E-13));
#24164=DIRECTION('center_axis',(7.55724335758485E-14,-0.866025403795606,
-0.499999999980658));
#24165=DIRECTION('ref_axis',(4.36317648660808E-14,-0.499999999980658,0.866025403795606));
#24166=DIRECTION('',(1.,8.72635297355373E-14,0.));
#24167=DIRECTION('',(4.36317648660808E-14,-0.499999999980658,0.866025403795606));
#24168=DIRECTION('center_axis',(7.55724335758385E-14,-0.86602540379549,
0.499999999980858));
#24169=DIRECTION('ref_axis',(-4.36317648660983E-14,0.499999999980858,0.86602540379549));
#24170=DIRECTION('',(1.,8.72635297355373E-14,0.));
#24171=DIRECTION('',(-4.36317648660983E-14,0.499999999980859,0.86602540379549));
#24172=DIRECTION('center_axis',(-1.00515054169548E-26,1.1518563880486E-13,
1.));
#24173=DIRECTION('ref_axis',(-8.72635297355373E-14,1.,-1.1518563880486E-13));
#24174=DIRECTION('',(1.,8.72635297355373E-14,0.));
#24175=DIRECTION('',(-8.72635297355373E-14,1.,-1.1518563880486E-13));
#24176=DIRECTION('center_axis',(-7.55724335758485E-14,0.866025403795606,
0.499999999980658));
#24177=DIRECTION('ref_axis',(-4.36317648660808E-14,0.499999999980658,-0.866025403795606));
#24178=DIRECTION('',(1.,8.72635297355373E-14,0.));
#24179=DIRECTION('',(-4.36317648660809E-14,0.499999999980659,-0.866025403795605));
#24180=DIRECTION('center_axis',(-7.55724335758385E-14,0.86602540379549,
-0.499999999980858));
#24181=DIRECTION('ref_axis',(4.36317648660983E-14,-0.499999999980858,-0.86602540379549));
#24182=DIRECTION('',(4.36317648660983E-14,-0.499999999980858,-0.86602540379549));
#24183=DIRECTION('center_axis',(-1.00515054169548E-26,1.1518563880486E-13,
1.));
#24184=DIRECTION('ref_axis',(-8.72635297355373E-14,1.,-1.1518563880486E-13));
#24185=DIRECTION('center_axis',(1.,8.72635297355373E-14,0.));
#24186=DIRECTION('ref_axis',(8.72635297355373E-14,-1.,1.1518563880486E-13));
#24187=DIRECTION('',(4.36317648660808E-14,-0.499999999980658,0.866025403795606));
#24188=DIRECTION('',(-4.36317648660983E-14,0.499999999980858,0.86602540379549));
#24189=DIRECTION('',(-8.72635297355373E-14,1.,-1.1518563880486E-13));
#24190=DIRECTION('',(-4.36317648660808E-14,0.499999999980658,-0.866025403795606));
#24191=DIRECTION('',(4.36317648660983E-14,-0.499999999980858,-0.86602540379549));
#24192=DIRECTION('',(8.72635297355373E-14,-1.,1.1518563880486E-13));
#24193=DIRECTION('center_axis',(-1.00515054169548E-26,1.1518563880486E-13,
1.));
#24194=DIRECTION('ref_axis',(-8.72635297355373E-14,1.,-1.1518563880486E-13));
#24195=DIRECTION('center_axis',(1.00515054169548E-26,-1.1518563880486E-13,
-1.));
#24196=DIRECTION('ref_axis',(8.72635297355373E-14,-1.,1.1518563880486E-13));
#24197=DIRECTION('',(-1.,-8.72635297355373E-14,0.));
#24198=DIRECTION('',(-0.206879256138141,0.978366482142418,-1.1269376823084E-13));
#24199=DIRECTION('',(0.238241565688704,-0.971205928924548,1.11868975334244E-13));
#24200=DIRECTION('',(1.,8.72635297355373E-14,0.));
#24201=DIRECTION('',(0.238241565688535,0.97120592892459,-1.11868975334244E-13));
#24202=DIRECTION('',(-0.20687925613797,-0.978366482142454,1.1269376823084E-13));
#24203=DIRECTION('center_axis',(-8.72635297355373E-14,1.,-1.1518563880486E-13));
#24204=DIRECTION('ref_axis',(1.00515054169548E-26,-1.1518563880486E-13,
-1.));
#24205=DIRECTION('',(1.,8.72635297355373E-14,0.));
#24206=DIRECTION('',(-1.00515054169548E-26,1.1518563880486E-13,1.));
#24207=DIRECTION('',(1.00515054169548E-26,-1.1518563880486E-13,-1.));
#24208=DIRECTION('center_axis',(1.00515054169548E-26,-1.1518563880486E-13,
-1.));
#24209=DIRECTION('ref_axis',(8.72635297355373E-14,-1.,1.1518563880486E-13));
#24210=DIRECTION('',(0.206879256138141,-0.978366482142418,1.1269376823084E-13));
#24211=DIRECTION('',(0.20687925613797,0.978366482142454,-1.1269376823084E-13));
#24212=DIRECTION('',(-0.238241565688535,-0.97120592892459,1.11868975334244E-13));
#24213=DIRECTION('',(-1.,-8.72635297355373E-14,0.));
#24214=DIRECTION('',(-0.238241565688704,0.971205928924548,-1.11868975334244E-13));
#24215=DIRECTION('center_axis',(-8.72635297355373E-14,1.,-1.1518563880486E-13));
#24216=DIRECTION('ref_axis',(1.00515054169548E-26,-1.1518563880486E-13,
-1.));
#24217=DIRECTION('',(1.,8.72635297355373E-14,0.));
#24218=DIRECTION('',(-1.00515054169548E-26,1.1518563880486E-13,1.));
#24219=DIRECTION('',(1.00515054169548E-26,-1.1518563880486E-13,-1.));
#24220=DIRECTION('center_axis',(-1.,-8.72635297355373E-14,0.));
#24221=DIRECTION('ref_axis',(-8.72635297355373E-14,1.,-1.1518563880486E-13));
#24222=DIRECTION('',(1.00515054169548E-26,-1.1518563880486E-13,-1.));
#24223=DIRECTION('',(-1.00515054169548E-26,1.1518563880486E-13,1.));
#24224=DIRECTION('',(-8.72635297355373E-14,1.,-1.1518563880486E-13));
#24225=DIRECTION('center_axis',(-0.499999999980834,0.866025403795504,-9.9753689357427E-14));
#24226=DIRECTION('ref_axis',(0.866025403795504,0.499999999980834,-5.75928194002136E-14));
#24227=DIRECTION('',(-1.00515054169548E-26,1.1518563880486E-13,1.));
#24228=DIRECTION('',(0.866025403795504,0.499999999980834,-5.75928194002136E-14));
#24229=DIRECTION('center_axis',(0.499999999980683,0.866025403795592,-9.9753689357427E-14));
#24230=DIRECTION('ref_axis',(0.866025403795591,-0.499999999980683,5.75928194002136E-14));
#24231=DIRECTION('',(-1.00515054169548E-26,1.1518563880486E-13,1.));
#24232=DIRECTION('',(0.866025403795592,-0.499999999980682,5.75928194002136E-14));
#24233=DIRECTION('center_axis',(1.,8.72635297355373E-14,0.));
#24234=DIRECTION('ref_axis',(8.72635297355373E-14,-1.,1.1518563880486E-13));
#24235=DIRECTION('',(-1.00515054169548E-26,1.1518563880486E-13,1.));
#24236=DIRECTION('',(8.72635297355373E-14,-1.,1.1518563880486E-13));
#24237=DIRECTION('center_axis',(0.499999999980834,-0.866025403795504,9.9753689357427E-14));
#24238=DIRECTION('ref_axis',(-0.866025403795504,-0.499999999980834,5.75928194002136E-14));
#24239=DIRECTION('',(-1.00515054169548E-26,1.1518563880486E-13,1.));
#24240=DIRECTION('',(-0.866025403795505,-0.499999999980833,5.75928194002135E-14));
#24241=DIRECTION('center_axis',(-0.499999999980683,-0.866025403795592,9.9753689357427E-14));
#24242=DIRECTION('ref_axis',(-0.866025403795591,0.499999999980683,-5.75928194002136E-14));
#24243=DIRECTION('',(-0.866025403795592,0.499999999980682,-5.75928194002135E-14));
#24244=DIRECTION('center_axis',(1.00515054169548E-26,-1.1518563880486E-13,
-1.));
#24245=DIRECTION('ref_axis',(8.72635297355373E-14,-1.,1.1518563880486E-13));
#24246=DIRECTION('center_axis',(1.00515054169548E-26,-1.1518563880486E-13,
-1.));
#24247=DIRECTION('ref_axis',(8.67361737988404E-14,-1.,1.1518563880486E-13));
#24248=DIRECTION('',(-8.72635297355373E-14,1.,-1.1518563880486E-13));
#24249=DIRECTION('',(1.,8.72635297355373E-14,0.));
#24250=DIRECTION('',(-1.,-8.72635297355373E-14,0.));
#24251=DIRECTION('',(-8.72635297355373E-14,1.,-1.1518563880486E-13));
#24252=DIRECTION('center_axis',(-7.55724335758385E-14,0.86602540379549,
-0.499999999980858));
#24253=DIRECTION('ref_axis',(4.36317648660983E-14,-0.499999999980858,-0.86602540379549));
#24254=DIRECTION('',(-1.,-8.72635297355373E-14,0.));
#24255=DIRECTION('',(-4.36317648660983E-14,0.499999999980858,0.86602540379549));
#24256=DIRECTION('center_axis',(-7.55724335758485E-14,0.866025403795606,
0.499999999980658));
#24257=DIRECTION('ref_axis',(-4.36317648660808E-14,0.499999999980658,-0.866025403795606));
#24258=DIRECTION('',(-1.,-8.72635297355373E-14,0.));
#24259=DIRECTION('',(4.36317648660809E-14,-0.499999999980659,0.866025403795605));
#24260=DIRECTION('center_axis',(-1.00515054169548E-26,1.1518563880486E-13,
1.));
#24261=DIRECTION('ref_axis',(-8.72635297355373E-14,1.,-1.1518563880486E-13));
#24262=DIRECTION('',(-1.,-8.72635297355373E-14,0.));
#24263=DIRECTION('',(8.72635297355373E-14,-1.,1.1518563880486E-13));
#24264=DIRECTION('center_axis',(-1.00515054169548E-26,1.1518563880486E-13,
1.));
#24265=DIRECTION('ref_axis',(1.11022302462516E-13,-1.,1.1518563880486E-13));
#24266=DIRECTION('',(8.72635297355373E-14,-1.,1.1518563880486E-13));
#24267=DIRECTION('center_axis',(7.55724335758385E-14,-0.86602540379549,
0.499999999980858));
#24268=DIRECTION('ref_axis',(-4.36317648660983E-14,0.499999999980858,0.86602540379549));
#24269=DIRECTION('',(-1.,-8.72635297355373E-14,0.));
#24270=DIRECTION('',(4.36317648660983E-14,-0.499999999980859,-0.86602540379549));
#24271=DIRECTION('center_axis',(7.55724335758485E-14,-0.866025403795606,
-0.499999999980658));
#24272=DIRECTION('ref_axis',(4.36317648660808E-14,-0.499999999980658,0.866025403795606));
#24273=DIRECTION('',(-4.36317648660808E-14,0.499999999980658,-0.866025403795606));
#24274=DIRECTION('center_axis',(-1.,-8.72635297355373E-14,0.));
#24275=DIRECTION('ref_axis',(-8.72635297355373E-14,1.,-1.1518563880486E-13));
#24276=DIRECTION('center_axis',(9.56709551734248E-27,-1.09634523681734E-13,
-1.));
#24277=DIRECTION('ref_axis',(8.88178419700124E-14,-1.,1.09634523681734E-13));
#24278=DIRECTION('',(-1.00572058919142E-26,1.1518563880486E-13,1.));
#24279=DIRECTION('center_axis',(8.72635297355373E-14,-1.,1.1518563880486E-13));
#24280=DIRECTION('ref_axis',(-1.,-8.72635297355373E-14,-1.43492962746861E-42));
#24281=DIRECTION('center_axis',(8.89982532115141E-14,-1.,1.11694157466017E-13));
#24282=DIRECTION('ref_axis',(9.25185853854302E-15,-1.11694157466016E-13,
-1.));
#24283=DIRECTION('',(-1.00572058919142E-26,1.1518563880486E-13,1.));
#24284=DIRECTION('center_axis',(0.863769935395407,0.503886382132179,0.000112288726983334));
#24285=DIRECTION('ref_axis',(0.502538534396613,-0.861475679507312,0.0729018179740325));
#24286=DIRECTION('center_axis',(-8.72635297355373E-14,1.,-1.11694157466017E-13));
#24287=DIRECTION('ref_axis',(9.74682643132155E-27,-1.11694157466017E-13,
-1.));
#24288=DIRECTION('',(-1.,-8.69744091562078E-14,-3.22930795142916E-29));
#24289=DIRECTION('',(-1.00572058919142E-26,1.1518563880486E-13,1.));
#24290=DIRECTION('center_axis',(8.89982532115141E-14,-1.,1.11694157466017E-13));
#24291=DIRECTION('ref_axis',(-5.97939217230155E-29,1.11694157466017E-13,
1.));
#24292=DIRECTION('center_axis',(-1.,-8.69744091562078E-14,-3.22930795142916E-29));
#24293=DIRECTION('ref_axis',(-8.69744091562078E-14,1.,-1.15648231731787E-13));
#24294=DIRECTION('',(1.,8.72635297355373E-14,-1.21904419394898E-29));
#24295=DIRECTION('center_axis',(0.863777735208662,-0.503873023735671,-1.04530852487832E-5));
#24296=DIRECTION('ref_axis',(0.502519089939509,0.861458237603484,-0.0732411708772271));
#24297=DIRECTION('',(-1.,-8.72635297355373E-14,-1.40416384211369E-42));
#24298=DIRECTION('center_axis',(1.00515054169548E-26,-1.1518563880486E-13,
-1.));
#24299=DIRECTION('ref_axis',(8.72635297355373E-14,-1.,1.1518563880486E-13));
#24300=DIRECTION('',(0.238241565688704,-0.971205928924548,1.11868975334244E-13));
#24301=DIRECTION('',(0.238241565688534,0.97120592892459,-1.11868975334244E-13));
#24302=DIRECTION('',(-1.,-8.72635297355373E-14,0.));
#24303=DIRECTION('center_axis',(-8.89982532115141E-14,1.,-1.11694157466017E-13));
#24304=DIRECTION('ref_axis',(5.9793921723027E-29,-1.11694157466017E-13,
-1.));
#24305=DIRECTION('center_axis',(8.89982532115141E-14,-1.,1.11694157466017E-13));
#24306=DIRECTION('ref_axis',(-4.31309843882671E-29,-1.11694157466017E-13,
-1.));
#24307=DIRECTION('',(-8.88962106541037E-14,1.,-1.1518563880486E-13));
#24308=DIRECTION('',(-8.72635297355373E-14,1.,-1.1518563880486E-13));
#24309=DIRECTION('center_axis',(1.00393149750153E-26,-1.1518563880486E-13,
-1.));
#24310=DIRECTION('ref_axis',(-1.,-8.72635297355373E-14,1.219044193949E-29));
#24311=DIRECTION('',(1.,8.72635297355373E-14,0.));
#24312=DIRECTION('',(-8.55288062595605E-14,1.,-1.11694157466017E-13));
#24313=DIRECTION('center_axis',(9.56709551734248E-27,-1.09634523681734E-13,
-1.));
#24314=DIRECTION('ref_axis',(8.88178419700124E-14,-1.,1.09634523681734E-13));
#24315=DIRECTION('',(1.00484705889771E-26,-1.1518563880486E-13,-1.));
#24316=DIRECTION('center_axis',(-8.72635297355373E-14,1.,-1.11694157466017E-13));
#24317=DIRECTION('ref_axis',(9.74682643132155E-27,-1.11694157466017E-13,
-1.));
#24318=DIRECTION('',(1.00484705889771E-26,-1.1518563880486E-13,-1.));
#24319=DIRECTION('center_axis',(8.55288062595605E-14,-1.,1.11694157466017E-13));
#24320=DIRECTION('ref_axis',(-5.74629564289751E-29,1.11694157466017E-13,
1.));
#24321=DIRECTION('center_axis',(8.55288062595605E-14,-1.,1.11694157466017E-13));
#24322=DIRECTION('ref_axis',(-5.74629564289751E-29,1.11694157466017E-13,
1.));
#24323=DIRECTION('center_axis',(8.55288062595605E-14,-1.,1.11694157466017E-13));
#24324=DIRECTION('ref_axis',(4.14495956315118E-29,1.11694157466017E-13,
1.));
#24325=DIRECTION('',(8.72635297355373E-14,-1.,1.1518563880486E-13));
#24326=DIRECTION('center_axis',(8.72635297355373E-14,-1.,1.1518563880486E-13));
#24327=DIRECTION('ref_axis',(-1.,-8.72635297355373E-14,-1.43492962746861E-42));
#24328=DIRECTION('center_axis',(8.56308488169709E-14,-1.,1.11694157466017E-13));
#24329=DIRECTION('ref_axis',(5.75315142317297E-29,-1.11694157466017E-13,
-1.));
#24330=DIRECTION('',(1.00484705889771E-26,-1.1518563880486E-13,-1.));
#24331=DIRECTION('center_axis',(1.,8.72635297355373E-14,0.));
#24332=DIRECTION('ref_axis',(8.72635297355373E-14,-1.,1.1518563880486E-13));
#24333=DIRECTION('center_axis',(1.00515054169548E-26,-1.1518563880486E-13,
-1.));
#24334=DIRECTION('ref_axis',(8.72635297355373E-14,-1.,1.1518563880486E-13));
#24335=DIRECTION('',(1.,8.72635297355373E-14,0.));
#24336=DIRECTION('',(-1.,-8.72635297355373E-14,0.));
#24337=DIRECTION('',(-8.72635297355373E-14,1.,-1.1518563880486E-13));
#24338=DIRECTION('center_axis',(-7.55724335758385E-14,0.86602540379549,
-0.499999999980858));
#24339=DIRECTION('ref_axis',(4.36317648660983E-14,-0.499999999980858,-0.86602540379549));
#24340=DIRECTION('',(-1.,-8.72635297355373E-14,0.));
#24341=DIRECTION('',(-4.36317648660978E-14,0.499999999980852,0.866025403795494));
#24342=DIRECTION('center_axis',(-7.55724335758485E-14,0.866025403795606,
0.499999999980658));
#24343=DIRECTION('ref_axis',(-4.36317648660808E-14,0.499999999980658,-0.866025403795606));
#24344=DIRECTION('',(-1.,-8.72635297355373E-14,0.));
#24345=DIRECTION('',(4.36317648660803E-14,-0.499999999980653,0.866025403795609));
#24346=DIRECTION('center_axis',(-1.00515054169548E-26,1.1518563880486E-13,
1.));
#24347=DIRECTION('ref_axis',(-8.72635297355373E-14,1.,-1.1518563880486E-13));
#24348=DIRECTION('',(-1.,-8.72635297355373E-14,0.));
#24349=DIRECTION('',(8.72635297355373E-14,-1.,1.1518563880486E-13));
#24350=DIRECTION('center_axis',(7.55724335758385E-14,-0.86602540379549,
0.499999999980858));
#24351=DIRECTION('ref_axis',(-4.36317648660983E-14,0.499999999980858,0.86602540379549));
#24352=DIRECTION('',(-1.,-8.72635297355373E-14,0.));
#24353=DIRECTION('',(4.36317648660981E-14,-0.499999999980856,-0.866025403795491));
#24354=DIRECTION('center_axis',(7.55724335758485E-14,-0.866025403795606,
-0.499999999980658));
#24355=DIRECTION('ref_axis',(4.36317648660808E-14,-0.499999999980658,0.866025403795606));
#24356=DIRECTION('',(-4.36317648660806E-14,0.499999999980657,-0.866025403795607));
#24357=DIRECTION('center_axis',(-0.97120592892459,0.238241565688534,-2.74420069337136E-14));
#24358=DIRECTION('ref_axis',(0.238241565688534,0.97120592892459,-1.11868975334244E-13));
#24359=DIRECTION('',(1.00515054169548E-26,-1.1518563880486E-13,-1.));
#24360=DIRECTION('center_axis',(-0.978366482142454,0.20687925613797,-2.38295192737362E-14));
#24361=DIRECTION('ref_axis',(0.20687925613797,0.978366482142454,-1.1269376823084E-13));
#24362=DIRECTION('',(1.00515054169548E-26,-1.1518563880486E-13,-1.));
#24363=DIRECTION('center_axis',(-0.97120592892459,0.238241565688534,-2.74420069337136E-14));
#24364=DIRECTION('ref_axis',(0.238241565688534,0.97120592892459,-1.11868975334244E-13));
#24365=DIRECTION('',(0.238241565688534,0.97120592892459,-1.11868975334244E-13));
#24366=DIRECTION('',(1.00515054169548E-26,-1.1518563880486E-13,-1.));
#24367=DIRECTION('',(-1.00515054169548E-26,1.1518563880486E-13,1.));
#24368=DIRECTION('center_axis',(-8.72635297355373E-14,1.,-1.1518563880486E-13));
#24369=DIRECTION('ref_axis',(1.00515054169548E-26,-1.1518563880486E-13,
-1.));
#24370=DIRECTION('',(1.,8.72635297355373E-14,0.));
#24371=DIRECTION('',(-1.00515054169548E-26,1.1518563880486E-13,1.));
#24372=DIRECTION('center_axis',(0.971205928924548,0.238241565688704,-2.74420069337136E-14));
#24373=DIRECTION('ref_axis',(0.238241565688704,-0.971205928924548,1.11868975334244E-13));
#24374=DIRECTION('',(0.238241565688704,-0.971205928924548,1.11868975334244E-13));
#24375=DIRECTION('',(-1.00515054169548E-26,1.1518563880486E-13,1.));
#24376=DIRECTION('center_axis',(0.978366482142418,0.206879256138141,-2.38295192737362E-14));
#24377=DIRECTION('ref_axis',(0.206879256138141,-0.978366482142418,1.1269376823084E-13));
#24378=DIRECTION('',(-1.00515054169548E-26,1.1518563880486E-13,1.));
#24379=DIRECTION('center_axis',(0.971205928924548,0.238241565688704,-2.74420069337136E-14));
#24380=DIRECTION('ref_axis',(0.238241565688704,-0.971205928924548,1.11868975334244E-13));
#24381=DIRECTION('',(-1.00515054169548E-26,1.1518563880486E-13,1.));
#24382=DIRECTION('center_axis',(-1.00515054169548E-26,1.1518563880486E-13,
1.));
#24383=DIRECTION('ref_axis',(-8.72635297355373E-14,1.,-1.1518563880486E-13));
#24384=DIRECTION('center_axis',(1.,8.72635297355373E-14,0.));
#24385=DIRECTION('ref_axis',(8.72635297355373E-14,-1.,1.1518563880486E-13));
#24386=DIRECTION('',(1.00515054169548E-26,-1.1518563880486E-13,-1.));
#24387=DIRECTION('center_axis',(-1.,-8.72635297355373E-14,0.));
#24388=DIRECTION('ref_axis',(-8.72635297355373E-14,1.,-1.1518563880486E-13));
#24389=DIRECTION('',(1.00515054169548E-26,-1.1518563880486E-13,-1.));
#24390=DIRECTION('',(1.00515054169548E-26,-1.1518563880486E-13,-1.));
#24391=DIRECTION('center_axis',(1.00515054169548E-26,-1.1518563880486E-13,
-1.));
#24392=DIRECTION('ref_axis',(8.72635297355373E-14,-1.,1.1518563880486E-13));
#24393=DIRECTION('',(-8.72635297355373E-14,1.,-1.1518563880486E-13));
#24394=DIRECTION('center_axis',(-1.00515054169548E-26,1.1518563880486E-13,
1.));
#24395=DIRECTION('ref_axis',(8.67361737988404E-14,-1.,1.1518563880486E-13));
#24396=DIRECTION('center_axis',(1.00515054169548E-26,-1.1518563880486E-13,
-1.));
#24397=DIRECTION('ref_axis',(8.72635297355373E-14,-1.,1.1518563880486E-13));
#24398=DIRECTION('',(-8.72635297355373E-14,1.,-1.1518563880486E-13));
#24399=DIRECTION('center_axis',(-1.00515054169548E-26,1.1518563880486E-13,
1.));
#24400=DIRECTION('ref_axis',(8.67361737988403E-14,-1.,1.1518563880486E-13));
#24401=DIRECTION('center_axis',(1.,8.72635297355373E-14,0.));
#24402=DIRECTION('ref_axis',(8.72635297355373E-14,-1.,1.1518563880486E-13));
#24403=DIRECTION('',(-1.00515054169548E-26,1.1518563880486E-13,1.));
#24404=DIRECTION('center_axis',(1.,8.88962106541037E-14,-1.82360919610117E-28));
#24405=DIRECTION('ref_axis',(8.88962106541037E-14,-1.,1.1518563880486E-13));
#24406=DIRECTION('',(1.00515054169548E-26,-1.1518563880486E-13,-1.));
#24407=DIRECTION('',(8.89982532115141E-14,-1.,1.11694157466017E-13));
#24408=DIRECTION('center_axis',(8.89982532115141E-14,-1.,1.11694157466017E-13));
#24409=DIRECTION('ref_axis',(-5.97939217230155E-29,1.11694157466017E-13,
1.));
#24410=DIRECTION('center_axis',(-8.89982532115141E-14,1.,-1.11694157466017E-13));
#24411=DIRECTION('ref_axis',(-2.77555756156289E-14,1.11694157466014E-13,
1.));
#24412=DIRECTION('',(-8.72635297355373E-14,1.,-1.1518563880486E-13));
#24413=DIRECTION('center_axis',(8.89982532115141E-14,-1.,1.11694157466017E-13));
#24414=DIRECTION('ref_axis',(4.31309843882786E-29,1.11694157466017E-13,
1.));
#24415=DIRECTION('center_axis',(1.00393149750153E-26,-1.1518563880486E-13,
-1.));
#24416=DIRECTION('ref_axis',(-1.,-8.72635297355373E-14,1.219044193949E-29));
#24417=DIRECTION('',(8.56308488169709E-14,-1.,1.11694157466017E-13));
#24418=DIRECTION('',(1.,8.69573680357505E-14,3.41964731060544E-29));
#24419=DIRECTION('center_axis',(-8.56308488169709E-14,1.,-1.11694157466017E-13));
#24420=DIRECTION('ref_axis',(-4.14990482420177E-29,-1.11694157466017E-13,
-1.));
#24421=DIRECTION('center_axis',(8.56308488169709E-14,-1.,1.11694157466017E-13));
#24422=DIRECTION('ref_axis',(-4.14990482420177E-29,-1.11694157466017E-13,
-1.));
#24423=DIRECTION('',(-8.72635297355373E-14,1.,-1.1518563880486E-13));
#24424=DIRECTION('center_axis',(-8.56308488169709E-14,1.,-1.11694157466017E-13));
#24425=DIRECTION('ref_axis',(-4.14990482420177E-29,-1.11694157466017E-13,
-1.));
#24426=DIRECTION('center_axis',(-8.72635297355373E-14,1.,-1.1518563880486E-13));
#24427=DIRECTION('ref_axis',(1.00515054169548E-26,-1.1518563880486E-13,
-1.));
#24428=DIRECTION('',(-1.00515054169548E-26,1.1518563880486E-13,1.));
#24429=DIRECTION('',(1.00515054169548E-26,-1.1518563880486E-13,-1.));
#24430=DIRECTION('center_axis',(-1.,-8.72635297355373E-14,3.03482797761984E-30));
#24431=DIRECTION('ref_axis',(-1.00484705889771E-26,1.1518563880486E-13,
1.));
#24432=DIRECTION('',(-1.00515054169548E-26,1.1518563880486E-13,1.));
#24433=DIRECTION('center_axis',(1.00515054169548E-26,-1.1518563880486E-13,
-1.));
#24434=DIRECTION('ref_axis',(8.72635297355373E-14,-1.,1.1518563880486E-13));
#24435=DIRECTION('',(8.72635297355373E-14,-1.,1.1518563880486E-13));
#24436=DIRECTION('center_axis',(-1.00515054169548E-26,1.1518563880486E-13,
1.));
#24437=DIRECTION('ref_axis',(8.90491384334761E-14,-1.,1.1518563880486E-13));
#24438=DIRECTION('center_axis',(1.00515054169548E-26,-1.1518563880486E-13,
-1.));
#24439=DIRECTION('ref_axis',(8.72635297355373E-14,-1.,1.1518563880486E-13));
#24440=DIRECTION('',(8.72635297355373E-14,-1.,1.1518563880486E-13));
#24441=DIRECTION('center_axis',(-1.00515054169548E-26,1.1518563880486E-13,
1.));
#24442=DIRECTION('ref_axis',(8.67361737988404E-14,-1.,1.1518563880486E-13));
#24443=DIRECTION('center_axis',(-1.00515054169548E-26,1.1518563880486E-13,
1.));
#24444=DIRECTION('ref_axis',(-8.72635297355373E-14,1.,-1.1518563880486E-13));
#24445=DIRECTION('center_axis',(-1.00515054169548E-26,1.1518563880486E-13,
1.));
#24446=DIRECTION('ref_axis',(-1.25899290992493E-13,-1.,1.1518563880486E-13));
#24447=DIRECTION('center_axis',(-1.00515054169548E-26,1.1518563880486E-13,
1.));
#24448=DIRECTION('ref_axis',(8.63130705120167E-14,-1.,1.1518563880486E-13));
#24449=DIRECTION('center_axis',(1.00515054169548E-26,-1.1518563880486E-13,
-1.));
#24450=DIRECTION('ref_axis',(-0.46275581060595,0.886485792187574,-1.02110432264563E-13));
#24451=DIRECTION('center_axis',(-1.00515054169548E-26,1.1518563880486E-13,
1.));
#24452=DIRECTION('ref_axis',(8.56289034950253E-14,-1.,1.1518563880486E-13));
#24453=DIRECTION('center_axis',(-1.00515054169548E-26,1.1518563880486E-13,
1.));
#24454=DIRECTION('ref_axis',(8.65147197380774E-14,-1.,1.1518563880486E-13));
#24455=DIRECTION('center_axis',(1.00515054169548E-26,-1.1518563880486E-13,
-1.));
#24456=DIRECTION('ref_axis',(8.72635297355373E-14,-1.,1.1518563880486E-13));
#24457=DIRECTION('center_axis',(1.00515054169548E-26,-1.1518563880486E-13,
-1.));
#24458=DIRECTION('ref_axis',(8.72912853111529E-14,-1.,1.1518563880486E-13));
#24459=DIRECTION('center_axis',(1.00515054169548E-26,-1.1518563880486E-13,
-1.));
#24460=DIRECTION('ref_axis',(8.72635297355373E-14,-1.,1.1518563880486E-13));
#24461=DIRECTION('center_axis',(1.00515054169548E-26,-1.1518563880486E-13,
-1.));
#24462=DIRECTION('ref_axis',(8.72912853111529E-14,-1.,1.1518563880486E-13));
#24463=DIRECTION('center_axis',(1.00515054169548E-26,-1.1518563880486E-13,
-1.));
#24464=DIRECTION('ref_axis',(8.72635297355373E-14,-1.,1.1518563880486E-13));
#24465=DIRECTION('center_axis',(1.00515054169548E-26,-1.1518563880486E-13,
-1.));
#24466=DIRECTION('ref_axis',(8.73285184003934E-14,-1.,1.1518563880486E-13));
#24467=DIRECTION('center_axis',(1.00515054169548E-26,-1.1518563880486E-13,
-1.));
#24468=DIRECTION('ref_axis',(0.232483687494752,0.972600295624488,-1.120295863533E-13));
#24469=DIRECTION('center_axis',(-1.00515054169548E-26,1.1518563880486E-13,
1.));
#24470=DIRECTION('ref_axis',(-8.72635297355373E-14,1.,-1.1518563880486E-13));
#24471=DIRECTION('center_axis',(-1.00515054169548E-26,1.1518563880486E-13,
1.));
#24472=DIRECTION('ref_axis',(8.72425792474809E-14,-1.,1.1518563880486E-13));
#24473=DIRECTION('center_axis',(-1.,-8.72635297355373E-14,0.));
#24474=DIRECTION('ref_axis',(-8.72635297355373E-14,1.,-1.1518563880486E-13));
#24475=DIRECTION('center_axis',(1.00515054169548E-26,-1.1518563880486E-13,
-1.));
#24476=DIRECTION('ref_axis',(8.72635297355373E-14,-1.,1.1518563880486E-13));
#24477=DIRECTION('',(8.72635297355373E-14,-1.,1.1518563880486E-13));
#24478=DIRECTION('',(-0.133254699246628,-0.991081825647454,1.14158393195087E-13));
#24479=DIRECTION('',(0.181426836203858,0.983404445335213,-1.13274069239474E-13));
#24480=DIRECTION('',(-0.148350608954417,0.988934829411349,-1.13911090062123E-13));
#24481=DIRECTION('',(-0.499999999998003,-0.866025403785592,9.97536893562752E-14));
#24482=DIRECTION('',(-1.,-8.72635297355373E-14,0.));
#24483=DIRECTION('center_axis',(-0.983404445335213,0.181426836203859,-2.0897766024496E-14));
#24484=DIRECTION('ref_axis',(0.181426836203859,0.983404445335213,-1.13274069239474E-13));
#24485=DIRECTION('',(-0.181426836203858,-0.983404445335213,1.13274069239474E-13));
#24486=DIRECTION('',(1.00515054169548E-26,-1.1518563880486E-13,-1.));
#24487=DIRECTION('center_axis',(1.00515054169548E-26,-1.1518563880486E-13,
-1.));
#24488=DIRECTION('ref_axis',(8.72635297355373E-14,-1.,1.1518563880486E-13));
#24489=DIRECTION('',(0.189038743476621,0.981969629604083,-1.13108799072916E-13));
#24490=DIRECTION('',(-0.177165010652742,0.984181161677267,-1.13363535807507E-13));
#24491=DIRECTION('',(0.148350608954417,-0.988934829411349,1.13911090062123E-13));
#24492=DIRECTION('center_axis',(-0.981969629604083,0.189038743476621,-2.17745484262326E-14));
#24493=DIRECTION('ref_axis',(0.189038743476621,0.981969629604083,-1.13108799072916E-13));
#24494=DIRECTION('',(0.189038743476622,0.981969629604083,-1.13108799072916E-13));
#24495=DIRECTION('',(1.00515054169548E-26,-1.1518563880486E-13,-1.));
#24496=DIRECTION('center_axis',(1.00515054169548E-26,-1.1518563880486E-13,
-1.));
#24497=DIRECTION('ref_axis',(8.72635297355373E-14,-1.,1.1518563880486E-13));
#24498=DIRECTION('',(0.177165010652742,-0.984181161677267,1.13363535807507E-13));
#24499=DIRECTION('',(0.181426836203858,0.983404445335213,-1.13274069239474E-13));
#24500=DIRECTION('',(-0.148350608954417,0.988934829411349,-1.13911090062123E-13));
#24501=DIRECTION('center_axis',(-0.983404445335213,0.181426836203859,-2.0897766024496E-14));
#24502=DIRECTION('ref_axis',(0.181426836203859,0.983404445335213,-1.13274069239474E-13));
#24503=DIRECTION('',(0.181426836203858,0.983404445335213,-1.13274069239474E-13));
#24504=DIRECTION('',(1.00515054169548E-26,-1.1518563880486E-13,-1.));
#24505=DIRECTION('center_axis',(1.00515054169548E-26,-1.1518563880486E-13,
-1.));
#24506=DIRECTION('ref_axis',(8.72635297355373E-14,-1.,1.1518563880486E-13));
#24507=DIRECTION('',(0.499999999998003,0.866025403785592,-9.97536893562752E-14));
#24508=DIRECTION('',(1.,8.72635297355373E-14,0.));
#24509=DIRECTION('',(0.499999999998154,-0.866025403785505,9.97536893562751E-14));
#24510=DIRECTION('',(1.,8.72635297355373E-14,0.));
#24511=DIRECTION('',(0.499999999998003,0.866025403785592,-9.97536893562752E-14));
#24512=DIRECTION('',(0.148350608954417,-0.988934829411349,1.13911090062123E-13));
#24513=DIRECTION('',(-0.18142683620403,0.983404445335182,-1.13274069239474E-13));
#24514=DIRECTION('',(0.148350608954245,0.988934829411375,-1.13911090062123E-13));
#24515=DIRECTION('',(0.499999999998154,-0.866025403785505,9.97536893562751E-14));
#24516=DIRECTION('',(1.,8.72635297355373E-14,0.));
#24517=DIRECTION('center_axis',(0.983404445335182,0.18142683620403,-2.0897766024496E-14));
#24518=DIRECTION('ref_axis',(0.18142683620403,-0.983404445335182,1.13274069239474E-13));
#24519=DIRECTION('',(-0.18142683620403,0.983404445335181,-1.13274069239474E-13));
#24520=DIRECTION('',(-1.00515054169548E-26,1.1518563880486E-13,1.));
#24521=DIRECTION('center_axis',(1.00515054169548E-26,-1.1518563880486E-13,
-1.));
#24522=DIRECTION('ref_axis',(8.72635297355373E-14,-1.,1.1518563880486E-13));
#24523=DIRECTION('',(0.17716501065257,0.984181161677298,-1.13363535807507E-13));
#24524=DIRECTION('',(-0.148350608954245,-0.988934829411375,1.13911090062123E-13));
#24525=DIRECTION('',(-0.189038743476793,0.98196962960405,-1.13108799072916E-13));
#24526=DIRECTION('center_axis',(0.98196962960405,0.189038743476793,-2.17745484262326E-14));
#24527=DIRECTION('ref_axis',(0.189038743476793,-0.98196962960405,1.13108799072916E-13));
#24528=DIRECTION('',(0.189038743476793,-0.98196962960405,1.13108799072916E-13));
#24529=DIRECTION('',(-1.00515054169548E-26,1.1518563880486E-13,1.));
#24530=DIRECTION('center_axis',(1.00515054169548E-26,-1.1518563880486E-13,
-1.));
#24531=DIRECTION('ref_axis',(8.72635297355373E-14,-1.,1.1518563880486E-13));
#24532=DIRECTION('',(0.148350608954245,0.988934829411375,-1.13911090062123E-13));
#24533=DIRECTION('',(-0.17716501065257,-0.984181161677298,1.13363535807507E-13));
#24534=DIRECTION('',(-0.18142683620403,0.983404445335182,-1.13274069239474E-13));
#24535=DIRECTION('center_axis',(0.983404445335182,0.18142683620403,-2.0897766024496E-14));
#24536=DIRECTION('ref_axis',(0.18142683620403,-0.983404445335182,1.13274069239474E-13));
#24537=DIRECTION('',(0.18142683620403,-0.983404445335181,1.13274069239474E-13));
#24538=DIRECTION('',(-1.00515054169548E-26,1.1518563880486E-13,1.));
#24539=DIRECTION('center_axis',(1.00515054169548E-26,-1.1518563880486E-13,
-1.));
#24540=DIRECTION('ref_axis',(8.72635297355373E-14,-1.,1.1518563880486E-13));
#24541=DIRECTION('',(-0.499999999998154,0.866025403785505,-9.97536893562751E-14));
#24542=DIRECTION('',(-0.148350608954245,-0.988934829411375,1.13911090062123E-13));
#24543=DIRECTION('',(-0.133254699246801,0.991081825647431,-1.14158393195087E-13));
#24544=DIRECTION('',(-8.72635297355373E-14,1.,-1.1518563880486E-13));
#24545=DIRECTION('',(-1.,-8.72635297355373E-14,0.));
#24546=DIRECTION('center_axis',(1.,8.72635297355373E-14,0.));
#24547=DIRECTION('ref_axis',(8.72635297355373E-14,-1.,1.1518563880486E-13));
#24548=DIRECTION('',(8.72635297355373E-14,-1.,1.1518563880486E-13));
#24549=DIRECTION('',(1.00515054169548E-26,-1.1518563880486E-13,-1.));
#24550=DIRECTION('',(-1.00515054169548E-26,1.1518563880486E-13,1.));
#24551=DIRECTION('center_axis',(1.00515054169548E-26,-1.1518563880486E-13,
-1.));
#24552=DIRECTION('ref_axis',(8.67361737988403E-14,-1.,1.1518563880486E-13));
#24553=DIRECTION('center_axis',(-1.00515054169548E-26,1.1518563880486E-13,
1.));
#24554=DIRECTION('ref_axis',(8.90491384334761E-14,-1.,1.1518563880486E-13));
#24555=DIRECTION('',(-1.00515054169548E-26,1.1518563880486E-13,1.));
#24556=DIRECTION('',(1.00515054169548E-26,-1.1518563880486E-13,-1.));
#24557=DIRECTION('center_axis',(1.00515054169548E-26,-1.1518563880486E-13,
-1.));
#24558=DIRECTION('ref_axis',(8.67361737988404E-14,-1.,1.1518563880486E-13));
#24559=DIRECTION('center_axis',(-1.00515054169548E-26,1.1518563880486E-13,
1.));
#24560=DIRECTION('ref_axis',(8.67361737988404E-14,-1.,1.1518563880486E-13));
#24561=DIRECTION('',(-1.00515054169548E-26,1.1518563880486E-13,1.));
#24562=DIRECTION('',(1.00515054169548E-26,-1.1518563880486E-13,-1.));
#24563=DIRECTION('center_axis',(1.00515054169548E-26,-1.1518563880486E-13,
-1.));
#24564=DIRECTION('ref_axis',(8.67361737988403E-14,-1.,1.1518563880486E-13));
#24565=DIRECTION('center_axis',(-1.00515054169548E-26,1.1518563880486E-13,
1.));
#24566=DIRECTION('ref_axis',(8.67361737988404E-14,-1.,1.1518563880486E-13));
#24567=DIRECTION('',(-1.00515054169548E-26,1.1518563880486E-13,1.));
#24568=DIRECTION('',(1.00515054169548E-26,-1.1518563880486E-13,-1.));
#24569=DIRECTION('center_axis',(-1.,-8.72635297355373E-14,0.));
#24570=DIRECTION('ref_axis',(-8.72635297355373E-14,1.,-1.1518563880486E-13));
#24571=DIRECTION('',(-8.72635297355373E-14,1.,-1.1518563880486E-13));
#24572=DIRECTION('',(-1.00515054169548E-26,1.1518563880486E-13,1.));
#24573=DIRECTION('',(-1.00515054169548E-26,1.1518563880486E-13,1.));
#24574=DIRECTION('',(1.00515054169548E-26,-1.1518563880486E-13,-1.));
#24575=DIRECTION('',(-8.72635297355373E-14,1.,-1.1518563880486E-13));
#24576=DIRECTION('',(-8.72635297355373E-14,1.,-1.1518563880486E-13));
#24577=DIRECTION('center_axis',(-0.991081825647454,0.133254699246628,-1.53490276564824E-14));
#24578=DIRECTION('ref_axis',(0.133254699246628,0.991081825647454,-1.14158393195087E-13));
#24579=DIRECTION('',(0.133254699246629,0.991081825647454,-1.14158393195087E-13));
#24580=DIRECTION('',(-1.00515054169548E-26,1.1518563880486E-13,1.));
#24581=DIRECTION('center_axis',(-8.72635297355373E-14,1.,-1.1518563880486E-13));
#24582=DIRECTION('ref_axis',(1.00515054169548E-26,-1.1518563880486E-13,
-1.));
#24583=DIRECTION('',(1.,8.72635297355373E-14,0.));
#24584=DIRECTION('center_axis',(-8.69573680357505E-14,1.,-1.11694157466017E-13));
#24585=DIRECTION('ref_axis',(9.74682643132155E-27,-1.11694157466017E-13,
-1.));
#24586=DIRECTION('',(1.,8.72635297355373E-14,0.));
#24587=DIRECTION('center_axis',(-8.72635297355373E-14,1.,-1.1518563880486E-13));
#24588=DIRECTION('ref_axis',(1.00515054169548E-26,-1.1518563880486E-13,
-1.));
#24589=DIRECTION('',(1.,8.72635297355373E-14,0.));
#24590=DIRECTION('',(-1.00515054169548E-26,1.1518563880486E-13,1.));
#24591=DIRECTION('center_axis',(0.991081825647431,0.133254699246801,-1.53490276564823E-14));
#24592=DIRECTION('ref_axis',(0.133254699246801,-0.991081825647431,1.14158393195087E-13));
#24593=DIRECTION('',(0.133254699246801,-0.991081825647431,1.14158393195087E-13));
#24594=DIRECTION('',(-1.00515054169548E-26,1.1518563880486E-13,1.));
#24595=DIRECTION('center_axis',(1.,8.72635297355373E-14,0.));
#24596=DIRECTION('ref_axis',(8.72635297355373E-14,-1.,1.1518563880486E-13));
#24597=DIRECTION('',(-1.00515054169548E-26,1.1518563880486E-13,1.));
#24598=DIRECTION('',(8.72635297355373E-14,-1.,1.1518563880486E-13));
#24599=DIRECTION('',(-1.00515054169548E-26,1.1518563880486E-13,1.));
#24600=DIRECTION('',(8.72635297355373E-14,-1.,1.1518563880486E-13));
#24601=DIRECTION('',(1.00515054169548E-26,-1.1518563880486E-13,-1.));
#24602=DIRECTION('center_axis',(1.00515054169548E-26,-1.1518563880486E-13,
-1.));
#24603=DIRECTION('ref_axis',(8.67361737988404E-14,-1.,1.1518563880486E-13));
#24604=DIRECTION('center_axis',(-1.00515054169548E-26,1.1518563880486E-13,
1.));
#24605=DIRECTION('ref_axis',(8.78926561161582E-14,-1.,1.1518563880486E-13));
#24606=DIRECTION('center_axis',(1.00515054169548E-26,-1.1518563880486E-13,
-1.));
#24607=DIRECTION('ref_axis',(8.72370886447792E-14,-1.,1.1518563880486E-13));
#24608=DIRECTION('center_axis',(-1.00515054169548E-26,1.1518563880486E-13,
1.));
#24609=DIRECTION('ref_axis',(8.72370886447792E-14,-1.,1.1518563880486E-13));
#24610=DIRECTION('center_axis',(1.00515054169548E-26,-1.1518563880486E-13,
-1.));
#24611=DIRECTION('ref_axis',(-8.80292434753227E-14,1.,-1.1518563880486E-13));
#24612=DIRECTION('center_axis',(-1.00515054169548E-26,1.1518563880486E-13,
1.));
#24613=DIRECTION('ref_axis',(8.54871728961371E-14,-1.,1.1518563880486E-13));
#24614=DIRECTION('center_axis',(1.00515054169548E-26,-1.1518563880486E-13,
-1.));
#24615=DIRECTION('ref_axis',(8.72370886447792E-14,-1.,1.1518563880486E-13));
#24616=DIRECTION('center_axis',(-1.00515054169548E-26,1.1518563880486E-13,
1.));
#24617=DIRECTION('ref_axis',(8.90504802424435E-14,-1.,1.1518563880486E-13));
#24618=DIRECTION('center_axis',(1.00515054169548E-26,-1.1518563880486E-13,
-1.));
#24619=DIRECTION('ref_axis',(8.72635297355373E-14,-1.,1.1518563880486E-13));
#24620=DIRECTION('center_axis',(-1.00515054169548E-26,1.1518563880486E-13,
1.));
#24621=DIRECTION('ref_axis',(5.08482145278322E-14,-1.,1.1518563880486E-13));
#24622=DIRECTION('center_axis',(-8.72635297355373E-14,1.,-1.1518563880486E-13));
#24623=DIRECTION('ref_axis',(1.00515054169548E-26,-1.1518563880486E-13,
-1.));
#24624=DIRECTION('',(1.,8.72635297355373E-14,0.));
#24625=DIRECTION('',(-1.00515054169548E-26,1.1518563880486E-13,1.));
#24626=DIRECTION('',(-1.,-8.72635297355373E-14,0.));
#24627=DIRECTION('',(1.00515054169548E-26,-1.1518563880486E-13,-1.));
#24628=DIRECTION('center_axis',(0.866025403785505,0.499999999998154,-5.75928194022086E-14));
#24629=DIRECTION('ref_axis',(0.499999999998154,-0.866025403785505,9.97536893562752E-14));
#24630=DIRECTION('',(0.499999999998154,-0.866025403785505,9.97536893562751E-14));
#24631=DIRECTION('',(-1.00515054169548E-26,1.1518563880486E-13,1.));
#24632=DIRECTION('',(-0.499999999998154,0.866025403785505,-9.97536893562751E-14));
#24633=DIRECTION('center_axis',(-0.866025403785592,0.499999999998003,-5.75928194022086E-14));
#24634=DIRECTION('ref_axis',(0.499999999998003,0.866025403785592,-9.97536893562752E-14));
#24635=DIRECTION('',(0.499999999998002,0.866025403785592,-9.97536893562751E-14));
#24636=DIRECTION('',(1.00515054169548E-26,-1.1518563880486E-13,-1.));
#24637=DIRECTION('center_axis',(-0.988934829411349,-0.148350608954417,1.70878596594946E-14));
#24638=DIRECTION('ref_axis',(-0.148350608954417,0.988934829411349,-1.13911090062123E-13));
#24639=DIRECTION('',(1.00515054169548E-26,-1.1518563880486E-13,-1.));
#24640=DIRECTION('center_axis',(-0.984181161677267,-0.177165010652742,2.0406864925896E-14));
#24641=DIRECTION('ref_axis',(-0.177165010652742,0.984181161677267,-1.13363535807507E-13));
#24642=DIRECTION('',(1.00515054169548E-26,-1.1518563880486E-13,-1.));
#24643=DIRECTION('center_axis',(-0.988934829411349,-0.148350608954417,1.70878596594946E-14));
#24644=DIRECTION('ref_axis',(-0.148350608954417,0.988934829411349,-1.13911090062123E-13));
#24645=DIRECTION('',(1.00515054169548E-26,-1.1518563880486E-13,-1.));
#24646=DIRECTION('',(1.00515054169548E-26,-1.1518563880486E-13,-1.));
#24647=DIRECTION('center_axis',(-0.866025403785592,0.499999999998003,-5.75928194022086E-14));
#24648=DIRECTION('ref_axis',(0.499999999998003,0.866025403785592,-9.97536893562752E-14));
#24649=DIRECTION('',(0.499999999998002,0.866025403785592,-9.97536893562751E-14));
#24650=DIRECTION('',(1.00515054169548E-26,-1.1518563880486E-13,-1.));
#24651=DIRECTION('',(-1.00515054169548E-26,1.1518563880486E-13,1.));
#24652=DIRECTION('center_axis',(-8.72635297355373E-14,1.,-1.1518563880486E-13));
#24653=DIRECTION('ref_axis',(1.00515054169548E-26,-1.1518563880486E-13,
-1.));
#24654=DIRECTION('',(1.,8.72635297355373E-14,0.));
#24655=DIRECTION('',(-1.00515054169548E-26,1.1518563880486E-13,1.));
#24656=DIRECTION('center_axis',(0.866025403785505,0.499999999998154,-5.75928194022086E-14));
#24657=DIRECTION('ref_axis',(0.499999999998154,-0.866025403785505,9.97536893562752E-14));
#24658=DIRECTION('',(0.499999999998154,-0.866025403785505,9.97536893562751E-14));
#24659=DIRECTION('',(-1.00515054169548E-26,1.1518563880486E-13,1.));
#24660=DIRECTION('center_axis',(8.72635297355373E-14,-1.,1.1518563880486E-13));
#24661=DIRECTION('ref_axis',(-1.00515054169548E-26,1.1518563880486E-13,
1.));
#24662=DIRECTION('',(1.00515054169548E-26,-1.1518563880486E-13,-1.));
#24663=DIRECTION('',(1.,8.72635297355373E-14,0.));
#24664=DIRECTION('',(-1.00515054169548E-26,1.1518563880486E-13,1.));
#24665=DIRECTION('center_axis',(-0.866025403785592,0.499999999998003,-5.75928194022086E-14));
#24666=DIRECTION('ref_axis',(0.499999999998003,0.866025403785592,-9.97536893562752E-14));
#24667=DIRECTION('',(0.499999999998002,0.866025403785592,-9.97536893562752E-14));
#24668=DIRECTION('',(1.00515054169548E-26,-1.1518563880486E-13,-1.));
#24669=DIRECTION('',(-1.00515054169548E-26,1.1518563880486E-13,1.));
#24670=DIRECTION('center_axis',(-8.72635297355373E-14,1.,-1.1518563880486E-13));
#24671=DIRECTION('ref_axis',(1.00515054169548E-26,-1.1518563880486E-13,
-1.));
#24672=DIRECTION('',(1.,8.72635297355373E-14,0.));
#24673=DIRECTION('',(-1.00515054169548E-26,1.1518563880486E-13,1.));
#24674=DIRECTION('center_axis',(0.866025403785505,0.499999999998154,-5.75928194022086E-14));
#24675=DIRECTION('ref_axis',(0.499999999998154,-0.866025403785505,9.97536893562752E-14));
#24676=DIRECTION('',(0.499999999998153,-0.866025403785505,9.97536893562752E-14));
#24677=DIRECTION('',(-1.00515054169548E-26,1.1518563880486E-13,1.));
#24678=DIRECTION('center_axis',(0.988934829411375,-0.148350608954245,1.70878596594946E-14));
#24679=DIRECTION('ref_axis',(-0.148350608954245,-0.988934829411375,1.13911090062123E-13));
#24680=DIRECTION('',(-1.00515054169548E-26,1.1518563880486E-13,1.));
#24681=DIRECTION('center_axis',(0.984181161677298,-0.17716501065257,2.0406864925896E-14));
#24682=DIRECTION('ref_axis',(-0.17716501065257,-0.984181161677298,1.13363535807507E-13));
#24683=DIRECTION('',(-1.00515054169548E-26,1.1518563880486E-13,1.));
#24684=DIRECTION('center_axis',(0.988934829411375,-0.148350608954245,1.70878596594946E-14));
#24685=DIRECTION('ref_axis',(-0.148350608954245,-0.988934829411375,1.13911090062123E-13));
#24686=DIRECTION('',(-1.00515054169548E-26,1.1518563880486E-13,1.));
#24687=DIRECTION('center_axis',(-8.72635297355373E-14,1.,-1.1518563880486E-13));
#24688=DIRECTION('ref_axis',(1.00515054169548E-26,-1.1518563880486E-13,
-1.));
#24689=DIRECTION('',(1.,8.72635297355373E-14,0.));
#24690=DIRECTION('',(-1.00515054169548E-26,1.1518563880486E-13,1.));
#24691=DIRECTION('',(-1.,-8.72635297355373E-14,0.));
#24692=DIRECTION('',(1.00515054169548E-26,-1.1518563880486E-13,-1.));
#24693=DIRECTION('center_axis',(0.866025403785505,0.499999999998154,-5.75928194022086E-14));
#24694=DIRECTION('ref_axis',(0.499999999998154,-0.866025403785505,9.97536893562752E-14));
#24695=DIRECTION('',(0.499999999998153,-0.866025403785505,9.97536893562752E-14));
#24696=DIRECTION('',(-1.00515054169548E-26,1.1518563880486E-13,1.));
#24697=DIRECTION('center_axis',(-0.866025403785592,0.499999999998003,-5.75928194022086E-14));
#24698=DIRECTION('ref_axis',(0.499999999998003,0.866025403785592,-9.97536893562752E-14));
#24699=DIRECTION('',(0.499999999998002,0.866025403785592,-9.97536893562752E-14));
#24700=DIRECTION('',(-0.499999999998002,-0.866025403785592,9.97536893562752E-14));
#24701=DIRECTION('',(1.00515054169548E-26,-1.1518563880486E-13,-1.));
#24702=DIRECTION('center_axis',(1.00515054169548E-26,-1.1518563880486E-13,
-1.));
#24703=DIRECTION('ref_axis',(8.72635297355373E-14,-1.,1.1518563880486E-13));
#24704=DIRECTION('',(-8.72635297355373E-14,1.,-1.1518563880486E-13));
#24705=DIRECTION('',(-1.,-8.72635297355373E-14,0.));
#24706=DIRECTION('',(8.72635297355373E-14,-1.,1.1518563880486E-13));
#24707=DIRECTION('center_axis',(1.,8.72635297355373E-14,0.));
#24708=DIRECTION('ref_axis',(8.72635297355373E-14,-1.,1.1518563880486E-13));
#24709=DIRECTION('',(8.72635297355373E-14,-1.,1.1518563880486E-13));
#24710=DIRECTION('',(-1.00515054169548E-26,1.1518563880486E-13,1.));
#24711=DIRECTION('center_axis',(1.00515054169548E-26,-1.1518563880486E-13,
-1.));
#24712=DIRECTION('ref_axis',(8.72635297355373E-14,-1.,1.1518563880486E-13));
#24713=DIRECTION('',(-8.72635297355373E-14,1.,-1.1518563880486E-13));
#24714=DIRECTION('',(-1.,-8.72635297355373E-14,0.));
#24715=DIRECTION('center_axis',(-1.,-8.72635297355373E-14,0.));
#24716=DIRECTION('ref_axis',(-8.72635297355373E-14,1.,-1.1518563880486E-13));
#24717=DIRECTION('',(-8.72635297355373E-14,1.,-1.1518563880486E-13));
#24718=DIRECTION('',(1.00515054169548E-26,-1.1518563880486E-13,-1.));
#24719=DIRECTION('center_axis',(1.00515054169548E-26,-1.1518563880486E-13,
-1.));
#24720=DIRECTION('ref_axis',(8.72635297355373E-14,-1.,1.1518563880486E-13));
#24721=DIRECTION('',(-8.72635297355373E-14,1.,-1.1518563880486E-13));
#24722=DIRECTION('',(1.,8.72635297355373E-14,0.));
#24723=DIRECTION('center_axis',(1.,8.72635297355373E-14,0.));
#24724=DIRECTION('ref_axis',(8.72635297355373E-14,-1.,1.1518563880486E-13));
#24725=DIRECTION('',(-8.72635297355373E-14,1.,-1.1518563880486E-13));
#24726=DIRECTION('',(-1.00515054169548E-26,1.1518563880486E-13,1.));
#24727=DIRECTION('center_axis',(1.00515054169548E-26,-1.1518563880486E-13,
-1.));
#24728=DIRECTION('ref_axis',(8.72635297355373E-14,-1.,1.1518563880486E-13));
#24729=DIRECTION('',(-8.72635297355373E-14,1.,-1.1518563880486E-13));
#24730=DIRECTION('',(1.,8.72635297355373E-14,0.));
#24731=DIRECTION('center_axis',(-1.,-8.72635297355373E-14,0.));
#24732=DIRECTION('ref_axis',(-8.72635297355373E-14,1.,-1.1518563880486E-13));
#24733=DIRECTION('',(-8.72635297355373E-14,1.,-1.1518563880486E-13));
#24734=DIRECTION('',(1.00515054169548E-26,-1.1518563880486E-13,-1.));
#24735=DIRECTION('center_axis',(1.00515054169548E-26,-1.1518563880486E-13,
-1.));
#24736=DIRECTION('ref_axis',(8.72635297355373E-14,-1.,1.1518563880486E-13));
#24737=DIRECTION('',(-8.72635297355373E-14,1.,-1.1518563880486E-13));
#24738=DIRECTION('',(1.,8.72635297355373E-14,0.));
#24739=DIRECTION('center_axis',(1.,8.72635297355373E-14,0.));
#24740=DIRECTION('ref_axis',(8.72635297355373E-14,-1.,1.1518563880486E-13));
#24741=DIRECTION('',(8.72635297355373E-14,-1.,1.1518563880486E-13));
#24742=DIRECTION('',(-1.00515054169548E-26,1.1518563880486E-13,1.));
#24743=DIRECTION('center_axis',(1.00515054169548E-26,-1.1518563880486E-13,
-1.));
#24744=DIRECTION('ref_axis',(8.72635297355373E-14,-1.,1.1518563880486E-13));
#24745=DIRECTION('',(-8.72635297355373E-14,1.,-1.1518563880486E-13));
#24746=DIRECTION('',(-1.,-8.72635297355373E-14,0.));
#24747=DIRECTION('center_axis',(-1.,-8.72635297355373E-14,0.));
#24748=DIRECTION('ref_axis',(-8.72635297355373E-14,1.,-1.1518563880486E-13));
#24749=DIRECTION('',(1.00515054169548E-26,-1.1518563880486E-13,-1.));
#24750=DIRECTION('center_axis',(8.72635297355373E-14,-1.,1.1518563880486E-13));
#24751=DIRECTION('ref_axis',(-1.00515054169548E-26,1.1518563880486E-13,
1.));
#30602=CARTESIAN_POINT('',(0.,0.,0.));
#30603=CARTESIAN_POINT('Origin',(1.3944401189292E-12,-11.1689999999806,
-178.099999999984));
#30604=CARTESIAN_POINT('',(-25.3339394440343,-11.168999999981,-181.499999999985));
#30605=CARTESIAN_POINT('Origin',(1.04025109975431E-12,-11.168999999981,
-181.499999999985));
#30606=CARTESIAN_POINT('',(-27.3317482398788,-11.1689999999812,-182.813484492891));
#30607=CARTESIAN_POINT('Origin',(-28.9999999999993,-11.1689999999806,-178.099999999984));
#30608=CARTESIAN_POINT('',(-1.27149462683012E-12,16.1627482398987,-182.813484492894));
#30609=CARTESIAN_POINT('Origin',(1.11022302462516E-12,-11.1689999999811,
-182.813484492891));
#30610=CARTESIAN_POINT('Origin',(1.11022302462516E-12,-11.1689999999811,
-182.813484492891));
#30611=CARTESIAN_POINT('Origin',(3.84137166520304E-13,-11.1689999999818,
-187.999999999984));
#30612=CARTESIAN_POINT('',(-28.668251760119,-11.1689999999812,-183.286515507081));
#30613=CARTESIAN_POINT('',(-1.38795896703444E-12,17.4992517601389,-183.286515507084));
#30614=CARTESIAN_POINT('Origin',(1.11022302462516E-12,-11.1689999999812,
-183.286515507081));
#30615=CARTESIAN_POINT('',(-29.757543650104,-11.1689999999813,-183.829154400138));
#30616=CARTESIAN_POINT('Origin',(-27.0000000000005,-11.1689999999818,-187.999999999984));
#30617=CARTESIAN_POINT('',(-1.48288102248418E-12,18.5885436501236,-183.829154400142));
#30618=CARTESIAN_POINT('Origin',(1.11022302462516E-12,-11.1689999999813,
-183.829154400138));
#30619=CARTESIAN_POINT('Origin',(1.11022302462516E-12,-11.1689999999813,
-183.829154400138));
#30620=CARTESIAN_POINT('Origin',(1.11022302462516E-12,-11.1689999999812,
-183.286515507081));
#30621=CARTESIAN_POINT('Origin',(1.21236354289067E-12,-11.1689999999812,
-182.999999999985));
#30622=CARTESIAN_POINT('',(-45.3097394023371,-11.1689999999816,-186.995472550883));
#30623=CARTESIAN_POINT('',(-2.8381159242873E-12,34.1407394023565,-186.995472550889));
#30624=CARTESIAN_POINT('Origin',(1.11022302462516E-12,-11.1689999999816,
-186.995472550883));
#30625=CARTESIAN_POINT('',(-49.0555555555546,-11.1689999999814,-184.832491389149));
#30626=CARTESIAN_POINT('Origin',(-45.4999999999988,-11.1689999999812,-182.999999999985));
#30627=CARTESIAN_POINT('',(5.42612633001892E-12,-60.2245555555371,-184.832491389143));
#30628=CARTESIAN_POINT('Origin',(1.11022302462516E-12,-11.1689999999814,
-184.832491389149));
#30629=CARTESIAN_POINT('Origin',(1.11022302462516E-12,-11.1689999999814,
-184.832491389149));
#30630=CARTESIAN_POINT('Origin',(1.11022302462516E-12,-11.1689999999816,
-186.995472550883));
#30631=CARTESIAN_POINT('Origin',(2.33812968986058E-12,-11.1689999999812,
-182.499999999986));
#30632=CARTESIAN_POINT('',(-32.7939650799149,-11.1689999999816,-185.836676479864));
#30633=CARTESIAN_POINT('',(-1.74747801983562E-12,21.6249650799345,-185.836676479867));
#30634=CARTESIAN_POINT('Origin',(1.11022302462516E-12,-11.1689999999815,
-185.836676479864));
#30635=CARTESIAN_POINT('',(-34.8097394023371,-11.1689999999817,-186.495472550884));
#30636=CARTESIAN_POINT('Origin',(-34.9999999999981,-11.1689999999812,-182.499999999986));
#30637=CARTESIAN_POINT('',(-1.92313474120327E-12,23.6407394023566,-186.495472550887));
#30638=CARTESIAN_POINT('Origin',(1.11022302462516E-12,-11.1689999999816,
-186.495472550884));
#30639=CARTESIAN_POINT('Origin',(1.11022302462516E-12,-11.1689999999816,
-186.495472550884));
#30640=CARTESIAN_POINT('Origin',(1.11022302462516E-12,-11.1689999999815,
-185.836676479864));
#30641=CARTESIAN_POINT('Origin',(1.11022302462516E-12,-11.1689999999813,
-183.999999999986));
#30642=CARTESIAN_POINT('',(5.91645271747501E-12,-66.1689999999812,-182.999999999979));
#30643=CARTESIAN_POINT('Origin',(1.12277548732324E-12,-11.1689999999812,
-182.999999999985));
#30644=CARTESIAN_POINT('',(5.91645271747499E-12,-66.168999999981,-181.499999999979));
#30645=CARTESIAN_POINT('',(5.91645271747502E-12,-66.1689999999813,-183.999999999979));
#30646=CARTESIAN_POINT('Origin',(1.11910480882216E-12,-11.168999999981,
-181.499999999985));
#30647=CARTESIAN_POINT('Origin',(1.11022302462516E-12,-11.1689999999812,
-183.286515507081));
#30648=CARTESIAN_POINT('',(-1.38795896703444E-12,17.4992517601389,-183.286515507084));
#30649=CARTESIAN_POINT('Origin',(1.11022302462516E-12,-11.1689999999812,
-182.999999999985));
#30650=CARTESIAN_POINT('',(5.4678483962789E-12,-61.1689999999812,-182.999999999979));
#30651=CARTESIAN_POINT('',(5.47952274539776E-12,-61.1689999999812,-182.99999999998));
#30652=CARTESIAN_POINT('Origin',(1.10617921426542E-12,-11.1689999999812,
-182.999999999985));
#30653=CARTESIAN_POINT('Origin',(1.11022302462516E-12,-11.1689999999815,
-185.836676479864));
#30654=CARTESIAN_POINT('',(-1.74747801983562E-12,21.6249650799345,-185.836676479867));
#30655=CARTESIAN_POINT('Origin',(1.11022302462516E-12,-11.1689999999816,
-186.995472550884));
#30656=CARTESIAN_POINT('',(-2.8381159242873E-12,34.1407394023566,-186.995472550889));
#30657=CARTESIAN_POINT('Origin',(1.11022302462516E-12,-11.168999999981,
-181.499999999986));
#30658=CARTESIAN_POINT('Origin',(-54.9999999999989,-11.168999999986,-182.999999999985));
#30659=CARTESIAN_POINT('Origin',(-6.0507154842071E-12,70.6167142857329,
-355.499999999994));
#30660=CARTESIAN_POINT('',(-6.03542612711786E-12,70.616714285733,-354.642857142845));
#30661=CARTESIAN_POINT('',(-6.04778737592304E-12,70.6167142857215,-356.357142857121));
#30662=CARTESIAN_POINT('Origin',(-6.0507154842071E-12,70.6167142857329,
-355.499999999994));
#30663=CARTESIAN_POINT('Origin',(-6.0507154842071E-12,70.6167142857329,
-355.499999999994));
#30664=CARTESIAN_POINT('',(-6.02295990859147E-12,70.3310000000051,-354.699999999991));
#30665=CARTESIAN_POINT('',(-6.05061051448147E-12,70.616714285733,-354.642857142845));
#30666=CARTESIAN_POINT('Origin',(-6.0278687718437E-12,70.3310000000051,
-355.499999999995));
#30667=CARTESIAN_POINT('Origin',(-6.02295990859147E-12,70.3310000001228,
-355.499999999994));
#30668=CARTESIAN_POINT('',(-6.02295990859147E-12,70.3310000000504,-356.499999999962));
#30669=CARTESIAN_POINT('',(-6.02283744391155E-12,70.3310000001227,-356.49999999992));
#30670=CARTESIAN_POINT('Origin',(-6.03053145953967E-12,70.3310000000491,
-355.499999999995));
#30671=CARTESIAN_POINT('Origin',(-42.5000000000061,70.331,-312.999999999994));
#30672=CARTESIAN_POINT('Origin',(-6.10622663543836E-12,71.3310000000423,
-355.499999999994));
#30673=CARTESIAN_POINT('',(-6.1934901652352E-12,72.3310000007449,-355.499999999995));
#30674=CARTESIAN_POINT('',(-6.10622663543836E-12,71.3309999999794,-356.));
#30675=CARTESIAN_POINT('',(-6.1061654030984E-12,71.3310000000423,-355.999999999961));
#30676=CARTESIAN_POINT('Origin',(-6.10622663543457E-12,71.3309999999989,
-355.499999999994));
#30677=CARTESIAN_POINT('Origin',(-6.10622663543836E-12,71.3309999999989,
-355.499999999994));
#30678=CARTESIAN_POINT('Origin',(-88.2,2.21370231173746E-11,-87.4999999999866));
#30679=CARTESIAN_POINT('',(-88.2,-1.44337567297757,-84.9999999999864));
#30680=CARTESIAN_POINT('',(-88.2,-2.88675134587786,-87.4999999999863));
#30681=CARTESIAN_POINT('',(-88.2,-1.44337567297757,-84.9999999999864));
#30682=CARTESIAN_POINT('',(-88.2,-1.44337567297815,-89.9999999999864));
#30683=CARTESIAN_POINT('',(-88.2,-2.88675134587786,-87.4999999999863));
#30684=CARTESIAN_POINT('',(-88.2,1.44337567302184,-89.9999999999867));
#30685=CARTESIAN_POINT('',(-88.2,2.18594673612182E-11,-89.9999999999866));
#30686=CARTESIAN_POINT('',(-88.2,2.88675134592214,-87.4999999999869));
#30687=CARTESIAN_POINT('',(-88.2,1.44337567302184,-89.9999999999867));
#30688=CARTESIAN_POINT('',(-88.2,1.44337567302243,-84.9999999999868));
#30689=CARTESIAN_POINT('',(-88.2,2.88675134592214,-87.4999999999869));
#30690=CARTESIAN_POINT('',(-88.2,2.24145788735308E-11,-84.9999999999866));
#30691=CARTESIAN_POINT('Origin',(-88.2,-2.165063509428,-88.7499999999863));
#30692=CARTESIAN_POINT('',(-85.,-1.44337567297788,-89.9999999999864));
#30693=CARTESIAN_POINT('',(-88.2,-1.44337567297815,-89.9999999999864));
#30694=CARTESIAN_POINT('',(-85.,-2.88675134587758,-87.4999999999863));
#30695=CARTESIAN_POINT('',(-88.2,-2.88675134587786,-87.4999999999863));
#30696=CARTESIAN_POINT('',(-85.,-2.16506350942773,-88.7499999999863));
#30697=CARTESIAN_POINT('Origin',(-88.2,-2.16506350942773,-86.2499999999863));
#30698=CARTESIAN_POINT('',(-85.,-1.44337567297729,-84.9999999999864));
#30699=CARTESIAN_POINT('',(-88.2,-1.44337567297757,-84.9999999999864));
#30700=CARTESIAN_POINT('',(-85.,-2.16506350942745,-86.2499999999863));
#30701=CARTESIAN_POINT('Origin',(-88.2,2.24145788735308E-11,-84.9999999999866));
#30702=CARTESIAN_POINT('',(-84.8059326826218,1.44337567302271,-84.9999999999868));
#30703=CARTESIAN_POINT('',(-88.2,1.44337567302243,-84.9999999999868));
#30704=CARTESIAN_POINT('',(-85.,2.26921346296871E-11,-84.9999999999866));
#30705=CARTESIAN_POINT('',(-81.0000000000025,29.7500000000231,-84.99999999999));
#30706=CARTESIAN_POINT('',(-85.,2.26921346296871E-11,-84.9999999999866));
#30707=CARTESIAN_POINT('Origin',(-88.2,2.16506350947228,-86.2499999999868));
#30708=CARTESIAN_POINT('',(-84.6118653652572,2.88675134592244,-87.4999999999869));
#30709=CARTESIAN_POINT('',(-88.2,2.88675134592214,-87.4999999999869));
#30710=CARTESIAN_POINT('',(-84.8059326826218,1.44337567302271,-84.9999999999868));
#30711=CARTESIAN_POINT('Origin',(-88.2,2.165063509472,-88.7499999999868));
#30712=CARTESIAN_POINT('',(-84.8059326826218,1.44337567302212,-89.9999999999867));
#30713=CARTESIAN_POINT('',(-88.2,1.44337567302184,-89.9999999999867));
#30714=CARTESIAN_POINT('',(-84.6118653652572,2.88675134592244,-87.4999999999869));
#30715=CARTESIAN_POINT('Origin',(-88.2,-0.721687836478147,-89.9999999999865));
#30716=CARTESIAN_POINT('',(-85.,2.21092675417589E-11,-89.9999999999866));
#30717=CARTESIAN_POINT('',(-84.8059326826218,1.44337567302212,-89.9999999999867));
#30718=CARTESIAN_POINT('',(-85.,-0.72168783647787,-89.9999999999865));
#30719=CARTESIAN_POINT('Origin',(-84.9999999999949,-57.499999999973,-47.49999999998));
#30720=CARTESIAN_POINT('',(-85.,2.70220044257252E-11,-47.4999999999866));
#30721=CARTESIAN_POINT('Origin',(-81.0000000000025,29.7500000000274,-47.49999999999));
#30722=CARTESIAN_POINT('Ctrl Pts',(41.9445347128706,60.6495679335285,-440.998916834174));
#30723=CARTESIAN_POINT('Ctrl Pts',(31.7948796622976,45.4225605594559,-462.499999999992));
#30724=CARTESIAN_POINT('Ctrl Pts',(47.4083864201783,59.4777499755747,-440.999999999994));
#30725=CARTESIAN_POINT('Ctrl Pts',(34.5033857139737,44.8351009291132,-462.499999999992));
#30726=CARTESIAN_POINT('Ctrl Pts',(52.4006927127278,56.9663054203067,-440.999999999994));
#30727=CARTESIAN_POINT('Ctrl Pts',(36.9523181444856,43.5374708585478,-462.499999999992));
#30728=CARTESIAN_POINT('Ctrl Pts',(56.6023578327675,53.2821982242028,-441.000077522351));
#30729=CARTESIAN_POINT('Ctrl Pts',(38.959068146329,41.6254058239817,-462.499232522636));
#30730=CARTESIAN_POINT('',(56.6023578328014,53.2821982241725,-441.000077522353));
#30731=CARTESIAN_POINT('',(41.945683924215,60.6520270238569,-440.996501147464));
#30732=CARTESIAN_POINT('Ctrl Pts',(56.6023578327675,53.2821982242028,-441.000077522351));
#30733=CARTESIAN_POINT('Ctrl Pts',(52.4008552484363,56.9661629056235,-441.000000002993));
#30734=CARTESIAN_POINT('Ctrl Pts',(47.4087643628648,59.4775598442953,-440.999999999995));
#30735=CARTESIAN_POINT('Ctrl Pts',(41.945141845367,60.649437717353,-440.998916954529));
#30736=CARTESIAN_POINT('',(43.5418850322931,44.6532394080568,-456.914860655543));
#30737=CARTESIAN_POINT('',(56.6023578328014,53.2821982241725,-441.000077522353));
#30738=CARTESIAN_POINT('',(38.7052731678116,41.8608202463478,-462.499996475683));
#30739=CARTESIAN_POINT('Ctrl Pts',(43.5418850322409,44.6532394081205,-456.914860655531));
#30740=CARTESIAN_POINT('Ctrl Pts',(42.6909235753114,44.161936581892,-457.897152546731));
#30741=CARTESIAN_POINT('Ctrl Pts',(41.834968106616,43.6677504616438,-458.885370858913));
#30742=CARTESIAN_POINT('Ctrl Pts',(40.2284919679139,42.740251030517,-460.740479172022));
#30743=CARTESIAN_POINT('Ctrl Pts',(39.4654128251454,42.2996870820088,-461.621826686247));
#30744=CARTESIAN_POINT('Ctrl Pts',(38.7058548823679,41.8611560992808,-462.499324435463));
#30745=CARTESIAN_POINT('',(31.7950297288388,45.4227856965977,-462.499682098234));
#30746=CARTESIAN_POINT('Ctrl Pts',(38.7052701171837,41.8608184850676,-462.499999999996));
#30747=CARTESIAN_POINT('Ctrl Pts',(37.73378223273,42.7450246881099,-462.499999999996));
#30748=CARTESIAN_POINT('Ctrl Pts',(36.6501650229394,43.4975098798192,-462.500000000097));
#30749=CARTESIAN_POINT('Ctrl Pts',(34.3164321736615,44.6996244168636,-462.500000000097));
#30750=CARTESIAN_POINT('Ctrl Pts',(33.0766926857734,45.1445339195995,-462.499999999997));
#30751=CARTESIAN_POINT('Ctrl Pts',(31.794974156998,45.4225400637676,-462.499999999997));
#30752=CARTESIAN_POINT('',(41.9454901388008,60.6510013100927,-440.996892854809));
#30753=CARTESIAN_POINT('Ctrl Pts',(56.6023578327675,53.2821982242028,-441.000077522351));
#30754=CARTESIAN_POINT('Ctrl Pts',(43.5418850322312,44.653239408115,-456.914860655543));
#30755=CARTESIAN_POINT('Ctrl Pts',(59.3135877730366,50.8952105744222,-440.999999999993));
#30756=CARTESIAN_POINT('Ctrl Pts',(47.7405554577269,40.7010682615999,-456.919527671004));
#30757=CARTESIAN_POINT('Ctrl Pts',(61.8717342174682,48.3453380510862,-440.999999999993));
#30758=CARTESIAN_POINT('Ctrl Pts',(51.8201097042108,36.6236615680342,-456.919527671003));
#30759=CARTESIAN_POINT('Ctrl Pts',(64.2705054959308,45.6385004273605,-441.000078147052));
#30760=CARTESIAN_POINT('Ctrl Pts',(55.7738565200363,32.4271120479789,-456.914852766313));
#30761=CARTESIAN_POINT('',(64.2705054959311,45.6385004273602,-441.000078147052));
#30762=CARTESIAN_POINT('Ctrl Pts',(64.2705054959308,45.6385004273605,-441.000078147052));
#30763=CARTESIAN_POINT('Ctrl Pts',(61.8717342174683,48.3453380510863,-440.999999999993));
#30764=CARTESIAN_POINT('Ctrl Pts',(59.3135877730366,50.8952105744222,-440.999999999993));
#30765=CARTESIAN_POINT('Ctrl Pts',(56.6023578327675,53.2821982242028,-441.000077522351));
#30766=CARTESIAN_POINT('',(56.5529890060887,33.6385804635181,-455.455487085885));
#30767=CARTESIAN_POINT('',(64.2705054959311,45.6385004273602,-441.000078147052));
#30768=CARTESIAN_POINT('',(61.00640553759,41.3521241633495,-446.556113667091));
#30769=CARTESIAN_POINT('Ctrl Pts',(56.5529890060882,33.6385804635188,-455.455487085885));
#30770=CARTESIAN_POINT('Ctrl Pts',(57.3013610416582,34.9347988520902,-453.959017905079));
#30771=CARTESIAN_POINT('Ctrl Pts',(58.1247838904071,36.361009062298,-452.312909266844));
#30772=CARTESIAN_POINT('Ctrl Pts',(59.6105260061009,38.9343898936254,-449.34393478218));
#30773=CARTESIAN_POINT('Ctrl Pts',(60.3109178717418,40.1475041900623,-447.944807398955));
#30774=CARTESIAN_POINT('Ctrl Pts',(61.0064055375901,41.3521241633496,-446.556113667091));
#30775=CARTESIAN_POINT('',(52.5211241633506,49.8374055375872,-446.553200603166));
#30776=CARTESIAN_POINT('Ctrl Pts',(61.00640553759,41.3521241633495,-446.556113667092));
#30777=CARTESIAN_POINT('Ctrl Pts',(59.7247235140878,42.8408739671962,-446.491862452654));
#30778=CARTESIAN_POINT('Ctrl Pts',(58.3867645976448,44.2845807962581,-446.459956651753));
#30779=CARTESIAN_POINT('Ctrl Pts',(55.5596333134075,47.1193359090829,-446.456714304226));
#30780=CARTESIAN_POINT('Ctrl Pts',(54.0645693704593,48.508635605192,-446.487617979628));
#30781=CARTESIAN_POINT('Ctrl Pts',(52.5211241633507,49.8374055375873,-446.553200603166));
#30782=CARTESIAN_POINT('Ctrl Pts',(52.5211241633505,49.8374055375871,-446.553200603166));
#30783=CARTESIAN_POINT('Ctrl Pts',(51.1319868849515,49.0353867559617,-448.154229195363));
#30784=CARTESIAN_POINT('Ctrl Pts',(49.7318236496382,48.2270021349601,-449.769111065283));
#30785=CARTESIAN_POINT('Ctrl Pts',(46.7368592415848,46.4978586277563,-453.225121323072));
#30786=CARTESIAN_POINT('Ctrl Pts',(45.0537435888084,45.5261113527318,-455.168522441224));
#30787=CARTESIAN_POINT('Ctrl Pts',(43.5418850322419,44.6532394081211,-456.914860655531));
#30788=CARTESIAN_POINT('Origin',(7.99360577730113E-14,4.65447819175679E-11,
57.5187545213137));
#30789=CARTESIAN_POINT('',(9.75000000013433,4.79819245881191E-11,70.0000000000134));
#30790=CARTESIAN_POINT('Origin',(1.11022302462516E-13,4.79774640155251E-11,
70.0000000000134));
#30791=CARTESIAN_POINT('',(6.7500000000709,4.73830448269764E-11,64.7999999999394));
#30792=CARTESIAN_POINT('Origin',(25.3774921629996,4.65416740711132E-11,
57.5187545213137));
#30793=CARTESIAN_POINT('',(-4.78833159847994E-13,6.75000000011816,64.7999999999386));
#30794=CARTESIAN_POINT('Origin',(1.11022302462516E-13,4.73668413519812E-11,
64.7999999999394));
#30795=CARTESIAN_POINT('Origin',(1.11022302462516E-13,4.73668413519812E-11,
64.7999999999394));
#30796=CARTESIAN_POINT('Origin',(-67.4999999999909,-102.999999999988,-194.999999999975));
#30797=CARTESIAN_POINT('',(-67.4999999999899,-114.999999999988,-188.249999999973));
#30798=CARTESIAN_POINT('Origin',(-67.4999999999899,-114.999999999988,-194.999999999974));
#30799=CARTESIAN_POINT('',(-67.499999999992,-90.9999999999876,-188.249999999976));
#30800=CARTESIAN_POINT('',(-67.4999999999909,-102.999999999988,-188.249999999975));
#30801=CARTESIAN_POINT('Origin',(-67.4999999999919,-90.9999999999884,-194.999999999976));
#30802=CARTESIAN_POINT('Origin',(-67.4999999999909,-102.999999999969,-29.9999999999748));
#30803=CARTESIAN_POINT('',(-67.4999999999899,-114.999999999969,-23.2499999999734));
#30804=CARTESIAN_POINT('Origin',(-67.4999999999899,-114.999999999969,-29.9999999999734));
#30805=CARTESIAN_POINT('',(-67.499999999992,-90.9999999999686,-23.2499999999761));
#30806=CARTESIAN_POINT('',(-67.4999999999909,-102.999999999969,-23.2499999999748));
#30807=CARTESIAN_POINT('Origin',(-67.4999999999919,-90.9999999999694,-29.9999999999761));
#30808=CARTESIAN_POINT('Origin',(67.5000000000091,-102.999999999977,-194.999999999975));
#30809=CARTESIAN_POINT('',(67.5000000000102,-114.999999999976,-188.249999999973));
#30810=CARTESIAN_POINT('Origin',(67.5000000000102,-114.999999999977,-194.999999999974));
#30811=CARTESIAN_POINT('',(67.5000000000081,-90.9999999999759,-188.249999999976));
#30812=CARTESIAN_POINT('',(67.5000000000091,-102.999999999976,-188.249999999975));
#30813=CARTESIAN_POINT('Origin',(67.5000000000081,-90.9999999999767,-194.999999999976));
#30814=CARTESIAN_POINT('Origin',(67.5000000000091,-102.999999999958,-29.9999999999748));
#30815=CARTESIAN_POINT('',(67.5000000000102,-114.999999999957,-23.2499999999734));
#30816=CARTESIAN_POINT('Origin',(67.5000000000102,-114.999999999958,-29.9999999999734));
#30817=CARTESIAN_POINT('',(67.5000000000081,-90.9999999999569,-23.2499999999761));
#30818=CARTESIAN_POINT('',(67.5000000000091,-102.999999999957,-23.2499999999748));
#30819=CARTESIAN_POINT('Origin',(67.5000000000081,-90.9999999999577,-29.9999999999761));
#30820=CARTESIAN_POINT('Origin',(-94.9999999999911,-100.749999999987,-164.999999999975));
#30821=CARTESIAN_POINT('',(-94.9999999999913,-98.4999999999867,-158.371463208194));
#30822=CARTESIAN_POINT('',(-94.9999999999913,-98.4999999999882,-171.628536791757));
#30823=CARTESIAN_POINT('Origin',(-94.9999999999911,-100.749999999987,-164.999999999975));
#30824=CARTESIAN_POINT('',(-95.7125498784832,-93.7499999999875,-164.999999999976));
#30825=CARTESIAN_POINT('Origin',(-94.6624763733376,-100.749999999986,-164.999999999976));
#30826=CARTESIAN_POINT('',(-98.9999999999917,-93.7499999999878,-164.999999999976));
#30827=CARTESIAN_POINT('',(-94.9999999999917,-93.7499999999874,-164.999999999976));
#30828=CARTESIAN_POINT('Origin',(-98.9999999999911,-100.749999999988,-164.999999999975));
#30829=CARTESIAN_POINT('Origin',(-94.6624763733376,-100.749999999986,-164.999999999976));
#30830=CARTESIAN_POINT('Origin',(38.0550000000051,-57.556999999962,-44.99999999998));
#30831=CARTESIAN_POINT('',(51.7674904174255,-33.7196845774533,-42.4999999999827));
#30832=CARTESIAN_POINT('',(10.5673523229225,-56.7328488120256,-42.4999999999801));
#30833=CARTESIAN_POINT('Origin',(38.0550000000051,-57.5569999999617,-42.49999999998));
#30834=CARTESIAN_POINT('',(10.5550722920713,-57.620055994213,-47.49999999998));
#30835=CARTESIAN_POINT('Ctrl Pts',(10.5673523229226,-56.7328488120256,-42.4999999999801));
#30836=CARTESIAN_POINT('Ctrl Pts',(10.5584011171405,-57.0313954797058,-44.1797004210614));
#30837=CARTESIAN_POINT('Ctrl Pts',(10.5544011407209,-57.3273540261342,-45.8477046901759));
#30838=CARTESIAN_POINT('Ctrl Pts',(10.5550722920713,-57.620055994213,-47.49999999998));
#30839=CARTESIAN_POINT('',(52.5421582028762,-34.1823931111825,-47.4999999999826));
#30840=CARTESIAN_POINT('Origin',(38.0550000000051,-57.5569999999623,-47.49999999998));
#30841=CARTESIAN_POINT('Ctrl Pts',(52.542158202876,-34.1823931111825,-47.4999999999826));
#30842=CARTESIAN_POINT('Ctrl Pts',(52.2878704277616,-34.0247901514976,-45.8480650809791));
#30843=CARTESIAN_POINT('Ctrl Pts',(52.0293151832961,-33.8703000947384,-44.1791951589754));
#30844=CARTESIAN_POINT('Ctrl Pts',(51.7674904174254,-33.7196845774533,-42.4999999999827));
#30845=CARTESIAN_POINT('Origin',(-4.16333634234434E-12,49.0000000000344,
-47.4999999999922));
#30846=CARTESIAN_POINT('',(15.897355545321,-49.7282841269805,-6.99999999998086));
#30847=CARTESIAN_POINT('',(-10.2448885166815,-50.4738270062687,-6.99999999998077));
#30848=CARTESIAN_POINT('Origin',(-4.16333634234434E-12,49.0000000000391,
-6.99999999999224));
#30849=CARTESIAN_POINT('',(-7.28266813181056,-56.1260192332767,-37.4999999999801));
#30850=CARTESIAN_POINT('Ctrl Pts',(-10.2448885166816,-50.4738270062687,
-6.99999999998077));
#30851=CARTESIAN_POINT('Ctrl Pts',(-10.0507613055644,-50.7351013152882,
-8.36117250371065));
#30852=CARTESIAN_POINT('Ctrl Pts',(-9.86589792999223,-50.9968893519918,
-9.7347210061088));
#30853=CARTESIAN_POINT('Ctrl Pts',(-9.02371416128865,-52.2490441303325,
-16.3436456471985));
#30854=CARTESIAN_POINT('Ctrl Pts',(-8.47879759119335,-53.2442638527576,
-21.7106826495237));
#30855=CARTESIAN_POINT('Ctrl Pts',(-7.74223532726688,-54.8678382816299,
-30.5666815694324));
#30856=CARTESIAN_POINT('Ctrl Pts',(-7.49420517598333,-55.5012098316531,
-34.0479123391732));
#30857=CARTESIAN_POINT('Ctrl Pts',(-7.28266813181053,-56.1260192332767,
-37.4999999999801));
#30858=CARTESIAN_POINT('',(-5.67440940859151,-56.2250837624614,-37.4999999999801));
#30859=CARTESIAN_POINT('Origin',(-4.16333634234434E-12,49.0000000000356,
-37.4999999999922));
#30860=CARTESIAN_POINT('',(-5.20468772204855,-58.0147518663479,-47.4999999999799));
#30861=CARTESIAN_POINT('Ctrl Pts',(-5.67440940859151,-56.2250837624614,
-37.4999999999801));
#30862=CARTESIAN_POINT('Ctrl Pts',(-5.48790484690666,-56.8307083626227,
-40.8727282805478));
#30863=CARTESIAN_POINT('Ctrl Pts',(-5.33237987148615,-57.4289168050392,
-44.216665726727));
#30864=CARTESIAN_POINT('Ctrl Pts',(-5.20468772204851,-58.014751866348,-47.4999999999799));
#30865=CARTESIAN_POINT('Origin',(-4.16333634234434E-12,49.0000000000344,
-47.4999999999922));
#30866=CARTESIAN_POINT('',(14.5912051142114,-56.253033145551,-42.4999999999801));
#30867=CARTESIAN_POINT('Origin',(-4.16333634234434E-12,49.000000000035,
-42.4999999999922));
#30868=CARTESIAN_POINT('Ctrl Pts',(14.5912051142115,-56.253033145551,-42.4999999999801));
#30869=CARTESIAN_POINT('Ctrl Pts',(14.6413830074691,-55.3501238490315,-37.4669303649321));
#30870=CARTESIAN_POINT('Ctrl Pts',(14.7457120954502,-54.4208510744167,-32.3299558893149));
#30871=CARTESIAN_POINT('Ctrl Pts',(15.1306789058763,-52.2343060024871,-20.3730017764038));
#30872=CARTESIAN_POINT('Ctrl Pts',(15.4586955420126,-50.9698252107939,-13.5560974490108));
#30873=CARTESIAN_POINT('Ctrl Pts',(15.8973555453209,-49.7282841269806,-6.99999999998084));
#30874=CARTESIAN_POINT('Origin',(-26.6999999999944,-62.6999999999673,-42.4999999999794));
#30875=CARTESIAN_POINT('',(-42.5246458122939,-47.416656618518,-37.4999999999811));
#30876=CARTESIAN_POINT('Origin',(-26.6999999999944,-62.6999999999668,-37.4999999999794));
#30877=CARTESIAN_POINT('',(-43.7529288036085,-48.8004453589419,-47.499999999981));
#30878=CARTESIAN_POINT('Ctrl Pts',(-42.5246458122939,-47.416656618518,-37.4999999999811));
#30879=CARTESIAN_POINT('Ctrl Pts',(-42.9648697341177,-47.8724723040717,
-40.8727279978944));
#30880=CARTESIAN_POINT('Ctrl Pts',(-43.3741092094881,-48.3356834485934,
-44.216666118921));
#30881=CARTESIAN_POINT('Ctrl Pts',(-43.7529288036086,-48.8004453589419,
-47.499999999981));
#30882=CARTESIAN_POINT('Origin',(-26.6999999999944,-62.6999999999679,-47.4999999999794));
#30883=CARTESIAN_POINT('Origin',(-66.0000000000025,29.5000000000286,-47.49999999999));
#30884=CARTESIAN_POINT('',(-66.0000000000031,36.5000000000286,-47.4999999999908));
#30885=CARTESIAN_POINT('Origin',(-66.0000000000025,29.5000000000286,-47.49999999999));
#30886=CARTESIAN_POINT('',(-66.0000000000031,36.5000000000291,-43.4999999999908));
#30887=CARTESIAN_POINT('',(-66.0000000000031,36.5000000000286,-47.4999999999908));
#30888=CARTESIAN_POINT('Origin',(-66.0000000000025,29.5000000000292,-43.49999999999));
#30889=CARTESIAN_POINT('Origin',(88.4000000000047,-51.9999999999593,-60.4999999999806));
#30890=CARTESIAN_POINT('',(92.4000000000041,-44.999999999959,-60.4999999999814));
#30891=CARTESIAN_POINT('Origin',(92.4000000000047,-51.999999999959,-60.4999999999806));
#30892=CARTESIAN_POINT('',(84.4557280900048,-44.9999999999596,-60.4999999999814));
#30893=CARTESIAN_POINT('',(88.4000000000041,-44.9999999999593,-60.4999999999814));
#30894=CARTESIAN_POINT('',(85.0000000000041,-45.5697141142108,-57.7338793541052));
#30895=CARTESIAN_POINT('Ctrl Pts',(84.4557280900048,-44.9999999999596,-60.4999999999814));
#30896=CARTESIAN_POINT('Ctrl Pts',(84.4557280900048,-44.9999999999596,-59.8974676734178));
#30897=CARTESIAN_POINT('Ctrl Pts',(84.5285835749808,-45.0839151982962,-59.2517827630011));
#30898=CARTESIAN_POINT('Ctrl Pts',(84.7679545571492,-45.3368090946526,-58.3292893663764));
#30899=CARTESIAN_POINT('Ctrl Pts',(84.8741075050836,-45.4463147868548,-58.0207406499748));
#30900=CARTESIAN_POINT('Ctrl Pts',(85.000000000004,-45.5697141142107,-57.7338793541051));
#30901=CARTESIAN_POINT('',(85.0000000000047,-52.4302858857074,-53.5132372262401));
#30902=CARTESIAN_POINT('Origin',(85.0000000000047,-51.9999999999597,-60.4999999999806));
#30903=CARTESIAN_POINT('',(84.4000000000048,-53.0627460667651,-53.5811438230183));
#30904=CARTESIAN_POINT('Ctrl Pts',(85.0000000000047,-52.4302858857074,-53.5132372262401));
#30905=CARTESIAN_POINT('Ctrl Pts',(84.9277840037038,-52.5010717206654,-53.517596633691));
#30906=CARTESIAN_POINT('Ctrl Pts',(84.8566687357403,-52.5725688539638,-53.523079799516));
#30907=CARTESIAN_POINT('Ctrl Pts',(84.6572933790792,-52.7781017148926,-53.5420908204731));
#30908=CARTESIAN_POINT('Ctrl Pts',(84.5277608269389,-52.917878905895,-53.5588920227949));
#30909=CARTESIAN_POINT('Ctrl Pts',(84.4000000000048,-53.0627460667651,-53.5811438230183));
#30910=CARTESIAN_POINT('',(84.4000000000048,-53.0627460667667,-67.4188561769427));
#30911=CARTESIAN_POINT('Origin',(84.4000000000047,-51.9999999999597,-60.4999999999806));
#30912=CARTESIAN_POINT('',(85.0000000000047,-52.4302858857091,-67.486762773721));
#30913=CARTESIAN_POINT('Ctrl Pts',(84.4000000000048,-53.0627460667667,-67.4188561769427));
#30914=CARTESIAN_POINT('Ctrl Pts',(84.5277608269389,-52.9178789058966,-67.4411079771661));
#30915=CARTESIAN_POINT('Ctrl Pts',(84.6572933790792,-52.7781017148941,-67.4579091794879));
#30916=CARTESIAN_POINT('Ctrl Pts',(84.8566687357402,-52.5725688539654,-67.4769202004451));
#30917=CARTESIAN_POINT('Ctrl Pts',(84.9277840037038,-52.501071720667,-67.4824033662701));
#30918=CARTESIAN_POINT('Ctrl Pts',(85.0000000000047,-52.4302858857091,-67.486762773721));
#30919=CARTESIAN_POINT('',(85.0000000000041,-45.5697141142114,-63.2661206458575));
#30920=CARTESIAN_POINT('Origin',(85.0000000000047,-51.9999999999597,-60.4999999999806));
#30921=CARTESIAN_POINT('Ctrl Pts',(85.000000000004,-45.5697141142114,-63.2661206458576));
#30922=CARTESIAN_POINT('Ctrl Pts',(84.8741075050836,-45.4463147868554,-62.9792593499879));
#30923=CARTESIAN_POINT('Ctrl Pts',(84.7679545571492,-45.3368090946531,-62.6707106335864));
#30924=CARTESIAN_POINT('Ctrl Pts',(84.5285835749809,-45.0839151982965,-61.7482172369618));
#30925=CARTESIAN_POINT('Ctrl Pts',(84.4557280900048,-44.9999999999597,-61.102532326545));
#30926=CARTESIAN_POINT('Ctrl Pts',(84.4557280900048,-44.9999999999597,-60.4999999999814));
#30927=CARTESIAN_POINT('Origin',(-88.4,2.21092675417589E-11,-87.4999999999866));
#30928=CARTESIAN_POINT('',(-85.,2.32194905663841E-11,-80.4999999999866));
#30929=CARTESIAN_POINT('',(-85.,2.16096671806776E-11,-94.4999999999866));
#30930=CARTESIAN_POINT('Origin',(-85.,2.24145788735308E-11,-87.4999999999866));
#30931=CARTESIAN_POINT('',(-84.4,4.46250000002306,-82.1068475128048));
#30932=CARTESIAN_POINT('Origin',(-84.9999999999962,3.66340291435563E-11,
-87.4999999999461));
#30933=CARTESIAN_POINT('',(-84.4000000000002,7.00000000002246,-87.4999999999874));
#30934=CARTESIAN_POINT('Origin',(-84.4,2.24700900247621E-11,-87.4999999999866));
#30935=CARTESIAN_POINT('',(-92.4000000000006,7.00000000002176,-87.4999999999874));
#30936=CARTESIAN_POINT('',(-88.4000000000006,7.00000000002211,-87.4999999999874));
#30937=CARTESIAN_POINT('Origin',(-92.4,2.17484450587558E-11,-87.4999999999866));
#30938=CARTESIAN_POINT('',(-84.4,4.46250000002184,-92.8931524871694));
#30939=CARTESIAN_POINT('Origin',(-84.4,2.24700900247621E-11,-87.4999999999866));
#30940=CARTESIAN_POINT('Origin',(-84.9999999999965,2.80445537735029E-11,
-87.4999999999995));
#30941=CARTESIAN_POINT('Origin',(1.11022302462516E-12,-11.1689999999808,
-179.499999999986));
#30942=CARTESIAN_POINT('',(-5.86106217982448E-12,68.8310000000173,-196.499999999995));
#30943=CARTESIAN_POINT('Origin',(1.11022302462516E-12,-11.1689999999827,
-196.499999999986));
#30944=CARTESIAN_POINT('',(-5.86106217982472E-12,68.8310000000201,-172.499999999995));
#30945=CARTESIAN_POINT('',(-5.86106217982465E-12,68.8310000000192,-179.499999999995));
#30946=CARTESIAN_POINT('Origin',(1.11022302462516E-12,-11.16899999998,-172.499999999986));
#30947=CARTESIAN_POINT('Origin',(1.11022302462516E-13,3.92899688478332E-11,
-5.2499999999866));
#30948=CARTESIAN_POINT('',(-3.37462029976237E-12,40.0000000000391,-6.99999999999121));
#30949=CARTESIAN_POINT('Origin',(1.11022302462516E-13,3.90956798185238E-11,
-6.9999999999866));
#30950=CARTESIAN_POINT('',(-3.3746202997624E-12,40.0000000000395,-3.4999999999912));
#30951=CARTESIAN_POINT('',(-3.37462029976239E-12,40.0000000000393,-5.24999999999121));
#30952=CARTESIAN_POINT('Origin',(1.11022302462516E-13,3.94842578771426E-11,
-3.4999999999866));
#30953=CARTESIAN_POINT('Origin',(-45.0000000000069,80.7485954613074,-137.259999999996));
#30954=CARTESIAN_POINT('',(-40.5000000000059,69.6242977306741,-50.1388507296581));
#30955=CARTESIAN_POINT('',(-49.500000000006,69.6242977306733,-50.1388507296581));
#30956=CARTESIAN_POINT('Ctrl Pts',(-49.5000000000044,69.6242977306726,-50.1388507296569));
#30957=CARTESIAN_POINT('Ctrl Pts',(-49.4390982354682,69.5996617539082,-50.0984034235873));
#30958=CARTESIAN_POINT('Ctrl Pts',(-49.3768762455399,69.5750761416804,-50.0591199168394));
#30959=CARTESIAN_POINT('Ctrl Pts',(-49.0593786189297,69.4527670848549,-49.8683860724675));
#30960=CARTESIAN_POINT('Ctrl Pts',(-48.7892136307126,69.3594387044218,-49.7382482521322));
#30961=CARTESIAN_POINT('Ctrl Pts',(-48.0207556703975,69.122587413154,-49.4258938436431));
#30962=CARTESIAN_POINT('Ctrl Pts',(-47.4278637439859,68.980519656034,-49.2670353254958));
#30963=CARTESIAN_POINT('Ctrl Pts',(-46.2057776234041,68.7933356998361,-49.066423146127));
#30964=CARTESIAN_POINT('Ctrl Pts',(-45.5767473719908,68.7485954613172,-49.0233224566437));
#30965=CARTESIAN_POINT('Ctrl Pts',(-44.423252628021,68.7485954613173,-49.0233224566437));
#30966=CARTESIAN_POINT('Ctrl Pts',(-43.7942223766076,68.7933356998363,-49.066423146127));
#30967=CARTESIAN_POINT('Ctrl Pts',(-42.5721362560258,68.9805196560344,-49.2670353254958));
#30968=CARTESIAN_POINT('Ctrl Pts',(-41.9792443296143,69.1225874131545,-49.4258938436431));
#30969=CARTESIAN_POINT('Ctrl Pts',(-41.2107863692992,69.3594387044225,-49.7382482521322));
#30970=CARTESIAN_POINT('Ctrl Pts',(-40.9406213810821,69.4527670848557,-49.8683860724675));
#30971=CARTESIAN_POINT('Ctrl Pts',(-40.6231237544707,69.5750761416816,-50.0591199168402));
#30972=CARTESIAN_POINT('Ctrl Pts',(-40.5609017645412,69.59966175391,-50.0984034235889));
#30973=CARTESIAN_POINT('Ctrl Pts',(-40.5000000000039,69.6242977306749,-50.1388507296593));
#30974=CARTESIAN_POINT('',(-40.5000000000059,69.6242977306647,-134.381149270331));
#30975=CARTESIAN_POINT('',(-40.5000000000059,69.6242977306643,-137.259999999995));
#30976=CARTESIAN_POINT('',(-49.500000000006,69.6242977306639,-134.381149270331));
#30977=CARTESIAN_POINT('Ctrl Pts',(-40.5000000000075,69.624297730664,-134.381149270332));
#30978=CARTESIAN_POINT('Ctrl Pts',(-40.5609017645436,69.5996617538996,-134.421596576402));
#30979=CARTESIAN_POINT('Ctrl Pts',(-40.623123754472,69.5750761416717,-134.46088008315));
#30980=CARTESIAN_POINT('Ctrl Pts',(-40.9406213810821,69.4527670848462,-134.651613927522));
#30981=CARTESIAN_POINT('Ctrl Pts',(-41.2107863692992,69.359438704413,-134.781751747857));
#30982=CARTESIAN_POINT('Ctrl Pts',(-41.9792443296143,69.1225874131449,-135.094106156346));
#30983=CARTESIAN_POINT('Ctrl Pts',(-42.5721362560258,68.9805196560248,-135.252964674493));
#30984=CARTESIAN_POINT('Ctrl Pts',(-43.7942223766076,68.7933356998266,-135.453576853862));
#30985=CARTESIAN_POINT('Ctrl Pts',(-44.4232526280209,68.7485954613077,-135.496677543345));
#30986=CARTESIAN_POINT('Ctrl Pts',(-45.5767473719907,68.7485954613076,-135.496677543345));
#30987=CARTESIAN_POINT('Ctrl Pts',(-46.2057776234041,68.7933356998264,-135.453576853862));
#30988=CARTESIAN_POINT('Ctrl Pts',(-47.4278637439859,68.9805196560244,-135.252964674493));
#30989=CARTESIAN_POINT('Ctrl Pts',(-48.0207556703975,69.1225874131444,-135.094106156346));
#30990=CARTESIAN_POINT('Ctrl Pts',(-48.7892136307126,69.3594387044123,-134.781751747857));
#30991=CARTESIAN_POINT('Ctrl Pts',(-49.0593786189297,69.4527670848454,-134.651613927522));
#30992=CARTESIAN_POINT('Ctrl Pts',(-49.3768762455412,69.5750761416714,-134.460880083149));
#30993=CARTESIAN_POINT('Ctrl Pts',(-49.4390982354707,69.5996617538998,-134.4215965764));
#30994=CARTESIAN_POINT('Ctrl Pts',(-49.5000000000081,69.6242977306647,-134.38114927033));
#30995=CARTESIAN_POINT('',(-49.500000000006,69.6242977306636,-137.259999999995));
#30996=CARTESIAN_POINT('Origin',(-27.000000000007,80.748595461309,-137.259999999996));
#30997=CARTESIAN_POINT('',(-22.500000000006,69.6242977306757,-50.1388507296581));
#30998=CARTESIAN_POINT('',(-31.500000000006,69.6242977306749,-50.1388507296581));
#30999=CARTESIAN_POINT('Ctrl Pts',(-31.5000000000043,69.6242977306742,-50.1388507296569));
#31000=CARTESIAN_POINT('Ctrl Pts',(-31.4390982354682,69.5996617539098,-50.0984034235873));
#31001=CARTESIAN_POINT('Ctrl Pts',(-31.3768762455399,69.5750761416819,-50.0591199168394));
#31002=CARTESIAN_POINT('Ctrl Pts',(-31.0593786189298,69.4527670848565,-49.8683860724675));
#31003=CARTESIAN_POINT('Ctrl Pts',(-30.7892136307126,69.3594387044234,-49.7382482521322));
#31004=CARTESIAN_POINT('Ctrl Pts',(-30.0207556703975,69.1225874131556,-49.4258938436431));
#31005=CARTESIAN_POINT('Ctrl Pts',(-29.4278637439859,68.9805196560356,-49.2670353254958));
#31006=CARTESIAN_POINT('Ctrl Pts',(-28.2057776234042,68.7933356998377,-49.066423146127));
#31007=CARTESIAN_POINT('Ctrl Pts',(-27.5767473719908,68.7485954613188,-49.0233224566438));
#31008=CARTESIAN_POINT('Ctrl Pts',(-26.423252628021,68.7485954613189,-49.0233224566438));
#31009=CARTESIAN_POINT('Ctrl Pts',(-25.7942223766076,68.7933356998379,-49.066423146127));
#31010=CARTESIAN_POINT('Ctrl Pts',(-24.5721362560259,68.980519656036,-49.2670353254958));
#31011=CARTESIAN_POINT('Ctrl Pts',(-23.9792443296144,69.1225874131561,-49.4258938436431));
#31012=CARTESIAN_POINT('Ctrl Pts',(-23.2107863692993,69.3594387044241,-49.7382482521322));
#31013=CARTESIAN_POINT('Ctrl Pts',(-22.9406213810822,69.4527670848572,-49.8683860724675));
#31014=CARTESIAN_POINT('Ctrl Pts',(-22.6231237544708,69.5750761416832,-50.0591199168402));
#31015=CARTESIAN_POINT('Ctrl Pts',(-22.5609017645412,69.5996617539116,-50.0984034235889));
#31016=CARTESIAN_POINT('Ctrl Pts',(-22.5000000000039,69.6242977306765,-50.1388507296593));
#31017=CARTESIAN_POINT('',(-22.500000000006,69.6242977306663,-134.381149270331));
#31018=CARTESIAN_POINT('',(-22.500000000006,69.6242977306659,-137.259999999995));
#31019=CARTESIAN_POINT('',(-31.500000000006,69.6242977306654,-134.381149270331));
#31020=CARTESIAN_POINT('Ctrl Pts',(-22.5000000000075,69.6242977306656,-134.381149270332));
#31021=CARTESIAN_POINT('Ctrl Pts',(-22.5609017645437,69.5996617539012,-134.421596576402));
#31022=CARTESIAN_POINT('Ctrl Pts',(-22.623123754472,69.5750761416733,-134.46088008315));
#31023=CARTESIAN_POINT('Ctrl Pts',(-22.9406213810822,69.4527670848478,-134.651613927522));
#31024=CARTESIAN_POINT('Ctrl Pts',(-23.2107863692993,69.3594387044146,-134.781751747857));
#31025=CARTESIAN_POINT('Ctrl Pts',(-23.9792443296144,69.1225874131465,-135.094106156346));
#31026=CARTESIAN_POINT('Ctrl Pts',(-24.5721362560259,68.9805196560264,-135.252964674493));
#31027=CARTESIAN_POINT('Ctrl Pts',(-25.7942223766076,68.7933356998282,-135.453576853862));
#31028=CARTESIAN_POINT('Ctrl Pts',(-26.423252628021,68.7485954613093,-135.496677543345));
#31029=CARTESIAN_POINT('Ctrl Pts',(-27.5767473719908,68.7485954613092,-135.496677543345));
#31030=CARTESIAN_POINT('Ctrl Pts',(-28.2057776234042,68.793335699828,-135.453576853862));
#31031=CARTESIAN_POINT('Ctrl Pts',(-29.4278637439859,68.980519656026,-135.252964674493));
#31032=CARTESIAN_POINT('Ctrl Pts',(-30.0207556703975,69.122587413146,-135.094106156346));
#31033=CARTESIAN_POINT('Ctrl Pts',(-30.7892136307126,69.3594387044139,-134.781751747857));
#31034=CARTESIAN_POINT('Ctrl Pts',(-31.0593786189298,69.4527670848471,-134.651613927522));
#31035=CARTESIAN_POINT('Ctrl Pts',(-31.3768762455412,69.575076141673,-134.460880083149));
#31036=CARTESIAN_POINT('Ctrl Pts',(-31.4390982354707,69.5996617539014,-134.4215965764));
#31037=CARTESIAN_POINT('Ctrl Pts',(-31.500000000008,69.6242977306663,-134.38114927033));
#31038=CARTESIAN_POINT('',(-31.500000000006,69.6242977306651,-137.259999999995));
#31039=CARTESIAN_POINT('Origin',(-9.00000000000695,80.7485954613106,-137.259999999996));
#31040=CARTESIAN_POINT('',(-6.66025403785028,68.9789060502699,-58.2599999999945));
#31041=CARTESIAN_POINT('',(-11.7870568576517,69.0767355378866,-49.3801170357112));
#31042=CARTESIAN_POINT('Origin',(-9.00000000010824,80.7485954607085,-54.2074411165631));
#31043=CARTESIAN_POINT('',(-4.50000000000594,69.624297730676,-60.85934207678));
#31044=CARTESIAN_POINT('Ctrl Pts',(-4.50000000000591,69.6242977306761,-60.85934207678));
#31045=CARTESIAN_POINT('Ctrl Pts',(-4.57072744769444,69.5956870693737,-60.798846259467));
#31046=CARTESIAN_POINT('Ctrl Pts',(-4.6401768168913,69.5683786357621,-60.7377313283798));
#31047=CARTESIAN_POINT('Ctrl Pts',(-5.44240225889553,69.2611409903921,-60.0120911133602));
#31048=CARTESIAN_POINT('Ctrl Pts',(-6.12426404754931,69.085457750299,-59.1883618955442));
#31049=CARTESIAN_POINT('Ctrl Pts',(-6.66025403785028,68.9789060502699,-58.2599999999945));
#31050=CARTESIAN_POINT('',(-4.50000000000611,69.6242977306689,-123.660657923209));
#31051=CARTESIAN_POINT('',(-4.50000000000594,69.6242977306675,-137.259999999995));
#31052=CARTESIAN_POINT('',(-6.66025403785028,68.9789060502623,-126.259999999995));
#31053=CARTESIAN_POINT('Ctrl Pts',(-6.66025403785036,68.9789060502623,-126.259999999995));
#31054=CARTESIAN_POINT('Ctrl Pts',(-6.12426404754937,69.0854577502916,-125.331638104445));
#31055=CARTESIAN_POINT('Ctrl Pts',(-5.44240225889557,69.2611409903848,-124.507908886629));
#31056=CARTESIAN_POINT('Ctrl Pts',(-4.64017681689139,69.568378635755,-123.782268671609));
#31057=CARTESIAN_POINT('Ctrl Pts',(-4.57072744769462,69.5956870693666,-123.721153740522));
#31058=CARTESIAN_POINT('Ctrl Pts',(-4.50000000000619,69.6242977306689,-123.660657923209));
#31059=CARTESIAN_POINT('',(-11.7870568576531,69.0767355378777,-135.13988296428));
#31060=CARTESIAN_POINT('Origin',(-9.00000000026207,80.7485954590947,-130.312558883691));
#31061=CARTESIAN_POINT('',(-13.5000000000061,69.6242977306671,-134.381149270331));
#31062=CARTESIAN_POINT('Ctrl Pts',(-13.5000000000062,69.6242977306671,-134.381149270331));
#31063=CARTESIAN_POINT('Ctrl Pts',(-13.4390982354695,69.5996617539025,-134.421596576401));
#31064=CARTESIAN_POINT('Ctrl Pts',(-13.3768762455405,69.5750761416743,-134.460880083149));
#31065=CARTESIAN_POINT('Ctrl Pts',(-13.0593786189297,69.4527670848486,-134.651613927522));
#31066=CARTESIAN_POINT('Ctrl Pts',(-12.7892136307126,69.3594387044155,-134.781751747857));
#31067=CARTESIAN_POINT('Ctrl Pts',(-12.2998487382835,69.2086084538895,-134.980663450779));
#31068=CARTESIAN_POINT('Ctrl Pts',(-12.0489093664513,69.13926180491,-135.066126567241));
#31069=CARTESIAN_POINT('Ctrl Pts',(-11.7870568576528,69.0767355378775,-135.139882964279));
#31070=CARTESIAN_POINT('',(-13.5000000000059,69.6242977306765,-50.1388507296581));
#31071=CARTESIAN_POINT('',(-13.5000000000059,69.6242977306667,-137.259999999995));
#31072=CARTESIAN_POINT('Ctrl Pts',(-11.787056857652,69.0767355378869,-49.3801170357097));
#31073=CARTESIAN_POINT('Ctrl Pts',(-12.0489093664508,69.1392618049194,-49.4538734327484));
#31074=CARTESIAN_POINT('Ctrl Pts',(-12.2998487382833,69.208608453899,-49.5393365492105));
#31075=CARTESIAN_POINT('Ctrl Pts',(-12.7892136307126,69.359438704425,-49.7382482521323));
#31076=CARTESIAN_POINT('Ctrl Pts',(-13.0593786189297,69.4527670848581,-49.8683860724675));
#31077=CARTESIAN_POINT('Ctrl Pts',(-13.3768762455404,69.5750761416838,-50.0591199168398));
#31078=CARTESIAN_POINT('Ctrl Pts',(-13.4390982354693,69.5996617539118,-50.0984034235881));
#31079=CARTESIAN_POINT('Ctrl Pts',(-13.500000000006,69.6242977306765,-50.138850729658));
#31080=CARTESIAN_POINT('Origin',(26.9999999999931,80.7485954613137,-137.259999999996));
#31081=CARTESIAN_POINT('',(31.499999999994,69.6242977306804,-50.1388507296581));
#31082=CARTESIAN_POINT('',(22.4999999999941,69.6242977306796,-50.1388507296581));
#31083=CARTESIAN_POINT('Ctrl Pts',(22.4999999999957,69.6242977306789,-50.1388507296569));
#31084=CARTESIAN_POINT('Ctrl Pts',(22.5609017645318,69.5996617539145,-50.0984034235874));
#31085=CARTESIAN_POINT('Ctrl Pts',(22.6231237544602,69.5750761416866,-50.0591199168394));
#31086=CARTESIAN_POINT('Ctrl Pts',(22.9406213810703,69.4527670848612,-49.8683860724675));
#31087=CARTESIAN_POINT('Ctrl Pts',(23.2107863692874,69.3594387044281,-49.7382482521322));
#31088=CARTESIAN_POINT('Ctrl Pts',(23.9792443296025,69.1225874131603,-49.4258938436431));
#31089=CARTESIAN_POINT('Ctrl Pts',(24.5721362560141,68.9805196560403,-49.2670353254958));
#31090=CARTESIAN_POINT('Ctrl Pts',(25.7942223765959,68.7933356998424,-49.066423146127));
#31091=CARTESIAN_POINT('Ctrl Pts',(26.4232526280092,68.7485954613235,-49.0233224566437));
#31092=CARTESIAN_POINT('Ctrl Pts',(27.5767473719791,68.7485954613236,-49.0233224566437));
#31093=CARTESIAN_POINT('Ctrl Pts',(28.2057776233924,68.7933356998426,-49.066423146127));
#31094=CARTESIAN_POINT('Ctrl Pts',(29.4278637439741,68.9805196560407,-49.2670353254958));
#31095=CARTESIAN_POINT('Ctrl Pts',(30.0207556703857,69.1225874131608,-49.4258938436431));
#31096=CARTESIAN_POINT('Ctrl Pts',(30.7892136307008,69.3594387044288,-49.7382482521322));
#31097=CARTESIAN_POINT('Ctrl Pts',(31.0593786189179,69.4527670848619,-49.8683860724675));
#31098=CARTESIAN_POINT('Ctrl Pts',(31.3768762455292,69.5750761416879,-50.0591199168402));
#31099=CARTESIAN_POINT('Ctrl Pts',(31.4390982354588,69.5996617539163,-50.0984034235889));
#31100=CARTESIAN_POINT('Ctrl Pts',(31.4999999999961,69.6242977306811,-50.1388507296593));
#31101=CARTESIAN_POINT('',(31.499999999994,69.6242977306789,-63.2599999999946));
#31102=CARTESIAN_POINT('',(31.499999999994,69.6242977306707,-137.259999999995));
#31103=CARTESIAN_POINT('',(22.4999999999941,69.6242977306781,-63.2599999999946));
#31104=CARTESIAN_POINT('Origin',(26.9999999999931,80.748595461322,-63.2599999999959));
#31105=CARTESIAN_POINT('',(22.4999999999941,69.6242977306698,-137.259999999995));
#31106=CARTESIAN_POINT('Origin',(44.9999999999931,80.7485954613153,-137.259999999996));
#31107=CARTESIAN_POINT('',(49.4999999999941,69.624297730682,-50.1388507296581));
#31108=CARTESIAN_POINT('',(40.499999999994,69.6242977306812,-50.1388507296581));
#31109=CARTESIAN_POINT('Ctrl Pts',(40.4999999999957,69.6242977306805,-50.1388507296569));
#31110=CARTESIAN_POINT('Ctrl Pts',(40.5609017645319,69.5996617539161,-50.0984034235874));
#31111=CARTESIAN_POINT('Ctrl Pts',(40.6231237544602,69.5750761416882,-50.0591199168395));
#31112=CARTESIAN_POINT('Ctrl Pts',(40.9406213810703,69.4527670848628,-49.8683860724675));
#31113=CARTESIAN_POINT('Ctrl Pts',(41.2107863692875,69.3594387044297,-49.7382482521323));
#31114=CARTESIAN_POINT('Ctrl Pts',(41.9792443296026,69.1225874131619,-49.4258938436431));
#31115=CARTESIAN_POINT('Ctrl Pts',(42.5721362560142,68.9805196560419,-49.2670353254958));
#31116=CARTESIAN_POINT('Ctrl Pts',(43.7942223765959,68.793335699844,-49.0664231461271));
#31117=CARTESIAN_POINT('Ctrl Pts',(44.4232526280093,68.7485954613251,-49.0233224566438));
#31118=CARTESIAN_POINT('Ctrl Pts',(45.5767473719791,68.7485954613252,-49.0233224566438));
#31119=CARTESIAN_POINT('Ctrl Pts',(46.2057776233924,68.7933356998442,-49.0664231461271));
#31120=CARTESIAN_POINT('Ctrl Pts',(47.4278637439741,68.9805196560423,-49.2670353254959));
#31121=CARTESIAN_POINT('Ctrl Pts',(48.0207556703856,69.1225874131624,-49.4258938436432));
#31122=CARTESIAN_POINT('Ctrl Pts',(48.7892136307007,69.3594387044304,-49.7382482521323));
#31123=CARTESIAN_POINT('Ctrl Pts',(49.0593786189178,69.4527670848635,-49.8683860724676));
#31124=CARTESIAN_POINT('Ctrl Pts',(49.3768762455292,69.5750761416895,-50.0591199168403));
#31125=CARTESIAN_POINT('Ctrl Pts',(49.4390982354588,69.5996617539179,-50.098403423589));
#31126=CARTESIAN_POINT('Ctrl Pts',(49.4999999999961,69.6242977306828,-50.1388507296594));
#31127=CARTESIAN_POINT('',(49.4999999999941,69.6242977306725,-134.381149270331));
#31128=CARTESIAN_POINT('',(49.4999999999941,69.6242977306722,-137.259999999995));
#31129=CARTESIAN_POINT('',(40.499999999994,69.6242977306718,-134.381149270331));
#31130=CARTESIAN_POINT('Ctrl Pts',(49.4999999999925,69.6242977306719,-134.381149270332));
#31131=CARTESIAN_POINT('Ctrl Pts',(49.4390982354563,69.5996617539075,-134.421596576402));
#31132=CARTESIAN_POINT('Ctrl Pts',(49.376876245528,69.5750761416795,-134.46088008315));
#31133=CARTESIAN_POINT('Ctrl Pts',(49.0593786189179,69.452767084854,-134.651613927522));
#31134=CARTESIAN_POINT('Ctrl Pts',(48.7892136307007,69.3594387044209,-134.781751747857));
#31135=CARTESIAN_POINT('Ctrl Pts',(48.0207556703856,69.1225874131528,-135.094106156346));
#31136=CARTESIAN_POINT('Ctrl Pts',(47.4278637439741,68.9805196560327,-135.252964674493));
#31137=CARTESIAN_POINT('Ctrl Pts',(46.2057776233924,68.7933356998346,-135.453576853862));
#31138=CARTESIAN_POINT('Ctrl Pts',(45.576747371979,68.7485954613156,-135.496677543345));
#31139=CARTESIAN_POINT('Ctrl Pts',(44.4232526280092,68.7485954613155,-135.496677543345));
#31140=CARTESIAN_POINT('Ctrl Pts',(43.7942223765959,68.7933356998343,-135.453576853862));
#31141=CARTESIAN_POINT('Ctrl Pts',(42.5721362560142,68.9805196560323,-135.252964674493));
#31142=CARTESIAN_POINT('Ctrl Pts',(41.9792443296026,69.1225874131523,-135.094106156346));
#31143=CARTESIAN_POINT('Ctrl Pts',(41.2107863692875,69.3594387044202,-134.781751747857));
#31144=CARTESIAN_POINT('Ctrl Pts',(40.9406213810703,69.4527670848533,-134.651613927522));
#31145=CARTESIAN_POINT('Ctrl Pts',(40.6231237544589,69.5750761416793,-134.460880083149));
#31146=CARTESIAN_POINT('Ctrl Pts',(40.5609017645293,69.5996617539077,-134.4215965764));
#31147=CARTESIAN_POINT('Ctrl Pts',(40.499999999992,69.6242977306726,-134.38114927033));
#31148=CARTESIAN_POINT('',(40.499999999994,69.6242977306714,-137.259999999995));
#31149=CARTESIAN_POINT('Origin',(1.11022302462516E-12,-11.1689999999816,
-186.499999999986));
#31150=CARTESIAN_POINT('',(-44.8103167727357,-39.4715707441228,-208.140791933168));
#31151=CARTESIAN_POINT('',(52.999999999995,-11.1689999999795,-208.140791933169));
#31152=CARTESIAN_POINT('Origin',(1.11022302462516E-12,-11.1689999999841,
-208.140791933171));
#31153=CARTESIAN_POINT('',(-51.6986185553089,-22.8417391589202,-208.140791933169));
#31154=CARTESIAN_POINT('Origin',(1.11022302462516E-12,-11.1689999999841,
-208.140791933171));
#31155=CARTESIAN_POINT('',(-51.6986185553089,-22.8417391589189,-196.499999999984));
#31156=CARTESIAN_POINT('',(-51.6986185553089,-22.8417391589189,-196.399999999984));
#31157=CARTESIAN_POINT('',(-44.8103167727357,-39.4715707441215,-196.499999999982));
#31158=CARTESIAN_POINT('Origin',(1.11022302462516E-12,-11.1689999999827,
-196.499999999986));
#31159=CARTESIAN_POINT('',(-44.8103167727357,-39.4715707441215,-196.399999999982));
#31160=CARTESIAN_POINT('Origin',(6.07847105982273E-12,-76.1689999999842,
-209.227922061336));
#31161=CARTESIAN_POINT('',(6.47170803469214E-12,-80.6689999999827,-196.499999999977));
#31162=CARTESIAN_POINT('Origin',(6.07847105982273E-12,-76.1689999999827,
-196.499999999978));
#31163=CARTESIAN_POINT('',(6.47170803469204E-12,-80.6689999999816,-186.499999999977));
#31164=CARTESIAN_POINT('',(6.47170803469227E-12,-80.6689999999842,-209.227922061336));
#31165=CARTESIAN_POINT('Origin',(6.07847105982273E-12,-76.1689999999816,
-186.499999999978));
#31166=CARTESIAN_POINT('Origin',(65.0000000000011,-11.168999999979,-209.227922061344));
#31167=CARTESIAN_POINT('',(65.0000000000015,-15.6689999999776,-196.499999999985));
#31168=CARTESIAN_POINT('Origin',(65.0000000000011,-11.1689999999776,-196.499999999986));
#31169=CARTESIAN_POINT('',(65.0000000000015,-15.6689999999764,-186.499999999985));
#31170=CARTESIAN_POINT('',(65.0000000000015,-15.668999999979,-209.227922061343));
#31171=CARTESIAN_POINT('Origin',(65.0000000000011,-11.1689999999764,-186.499999999986));
#31172=CARTESIAN_POINT('Origin',(-4.35762537165374E-12,53.8310000000158,
-209.227922061351));
#31173=CARTESIAN_POINT('',(-3.96438839678434E-12,49.3310000000173,-196.499999999992));
#31174=CARTESIAN_POINT('Origin',(-4.35762537165374E-12,53.8310000000173,
-196.499999999993));
#31175=CARTESIAN_POINT('',(-3.96438839678444E-12,49.3310000000184,-186.499999999992));
#31176=CARTESIAN_POINT('',(-3.96438839678421E-12,49.3310000000158,-209.227922061351));
#31177=CARTESIAN_POINT('Origin',(-4.35762537165374E-12,53.8310000000184,
-186.499999999993));
#31178=CARTESIAN_POINT('Origin',(-64.9999999999989,-11.1689999999899,-209.227922061344));
#31179=CARTESIAN_POINT('',(-64.9999999999985,-15.6689999999884,-196.499999999985));
#31180=CARTESIAN_POINT('Origin',(-64.9999999999989,-11.1689999999884,-196.499999999986));
#31181=CARTESIAN_POINT('',(-64.9999999999985,-15.6689999999872,-186.499999999985));
#31182=CARTESIAN_POINT('',(-64.9999999999985,-15.6689999999899,-209.227922061343));
#31183=CARTESIAN_POINT('Origin',(-64.9999999999989,-11.1689999999873,-186.499999999986));
#31184=CARTESIAN_POINT('Origin',(1.11022302462516E-13,3.97063024820676E-11,
-1.7499999999866));
#31185=CARTESIAN_POINT('',(-1.63179899864992E-12,20.0000000000395,-3.4999999999889));
#31186=CARTESIAN_POINT('Origin',(1.11022302462516E-13,3.94842578771426E-11,
-3.4999999999866));
#31187=CARTESIAN_POINT('',(-1.63179899864995E-12,20.0000000000399,1.11022302462516E-11));
#31188=CARTESIAN_POINT('',(-1.63179899864994E-12,20.0000000000397,-1.7499999999889));
#31189=CARTESIAN_POINT('Origin',(1.11022302462516E-13,3.99005915113771E-11,
1.34059430223488E-11));
#31190=CARTESIAN_POINT('Origin',(26.9999999999931,80.7485954613137,-137.259999999996));
#31191=CARTESIAN_POINT('',(31.499999999994,69.6242977306724,-121.259999999995));
#31192=CARTESIAN_POINT('',(22.4999999999941,69.6242977306716,-121.259999999995));
#31193=CARTESIAN_POINT('Origin',(26.9999999999931,80.7485954613155,-121.259999999996));
#31194=CARTESIAN_POINT('',(31.499999999994,69.624297730671,-134.381149270331));
#31195=CARTESIAN_POINT('',(31.499999999994,69.6242977306707,-137.259999999995));
#31196=CARTESIAN_POINT('',(22.4999999999941,69.6242977306702,-134.381149270331));
#31197=CARTESIAN_POINT('Ctrl Pts',(31.4999999999925,69.6242977306703,-134.381149270332));
#31198=CARTESIAN_POINT('Ctrl Pts',(31.4390982354563,69.5996617539059,-134.421596576402));
#31199=CARTESIAN_POINT('Ctrl Pts',(31.376876245528,69.575076141678,-134.46088008315));
#31200=CARTESIAN_POINT('Ctrl Pts',(31.0593786189179,69.4527670848525,-134.651613927522));
#31201=CARTESIAN_POINT('Ctrl Pts',(30.7892136307008,69.3594387044192,-134.781751747857));
#31202=CARTESIAN_POINT('Ctrl Pts',(30.0207556703857,69.1225874131512,-135.094106156346));
#31203=CARTESIAN_POINT('Ctrl Pts',(29.4278637439741,68.9805196560311,-135.252964674493));
#31204=CARTESIAN_POINT('Ctrl Pts',(28.2057776233924,68.7933356998329,-135.453576853862));
#31205=CARTESIAN_POINT('Ctrl Pts',(27.576747371979,68.748595461314,-135.496677543345));
#31206=CARTESIAN_POINT('Ctrl Pts',(26.4232526280092,68.7485954613139,-135.496677543345));
#31207=CARTESIAN_POINT('Ctrl Pts',(25.7942223765959,68.7933356998327,-135.453576853862));
#31208=CARTESIAN_POINT('Ctrl Pts',(24.5721362560141,68.9805196560307,-135.252964674493));
#31209=CARTESIAN_POINT('Ctrl Pts',(23.9792443296025,69.1225874131507,-135.094106156346));
#31210=CARTESIAN_POINT('Ctrl Pts',(23.2107863692874,69.3594387044186,-134.781751747857));
#31211=CARTESIAN_POINT('Ctrl Pts',(22.9406213810703,69.4527670848518,-134.651613927522));
#31212=CARTESIAN_POINT('Ctrl Pts',(22.6231237544589,69.5750761416777,-134.460880083149));
#31213=CARTESIAN_POINT('Ctrl Pts',(22.5609017645293,69.5996617539061,-134.4215965764));
#31214=CARTESIAN_POINT('Ctrl Pts',(22.499999999992,69.624297730671,-134.38114927033));
#31215=CARTESIAN_POINT('',(22.4999999999941,69.6242977306698,-137.259999999995));
#31216=CARTESIAN_POINT('Origin',(1.99999999999398,70.5000000000341,-53.2599999999947));
#31217=CARTESIAN_POINT('',(10.6602540378387,66.5000000000341,-58.2599999999942));
#31218=CARTESIAN_POINT('',(-6.66025403785006,66.5000000000326,-58.2599999999943));
#31219=CARTESIAN_POINT('Origin',(1.99999999999431,66.5000000000339,-53.2599999999943));
#31220=CARTESIAN_POINT('',(10.6602540378385,68.8640022192357,-58.2599999999945));
#31221=CARTESIAN_POINT('',(10.6602540378383,70.5000000000341,-58.2599999999947));
#31222=CARTESIAN_POINT('',(4.49999999999401,69.6242977306766,-62.9424583655132));
#31223=CARTESIAN_POINT('Ctrl Pts',(10.6602540378348,68.8640022192353,-58.2600000000009));
#31224=CARTESIAN_POINT('Ctrl Pts',(10.248704850567,68.8065096163321,-58.9728241021613));
#31225=CARTESIAN_POINT('Ctrl Pts',(9.75221352104281,68.7599390932012,-59.6251196466602));
#31226=CARTESIAN_POINT('Ctrl Pts',(8.83757091267963,68.7439037327988,-60.5769028187122));
#31227=CARTESIAN_POINT('Ctrl Pts',(8.39639094390703,68.7544489459965,-60.9689841103285));
#31228=CARTESIAN_POINT('Ctrl Pts',(7.45384509647339,68.8392168199242,-61.6622512795055));
#31229=CARTESIAN_POINT('Ctrl Pts',(6.95262696745016,68.9146735330389,-61.9634865839287));
#31230=CARTESIAN_POINT('Ctrl Pts',(5.86111154267866,69.1490964557957,-62.5104810158789));
#31231=CARTESIAN_POINT('Ctrl Pts',(5.18034932187989,69.3490828791313,-62.766792925962));
#31232=CARTESIAN_POINT('Ctrl Pts',(4.49999999999421,69.6242977306766,-62.9424583655131));
#31233=CARTESIAN_POINT('Ctrl Pts',(4.49999999999909,69.6242977306746,-62.9424583655118));
#31234=CARTESIAN_POINT('Ctrl Pts',(3.6938450265894,69.950403473993,-63.1506066846109));
#31235=CARTESIAN_POINT('Ctrl Pts',(2.8431330228302,70.1896440739217,-63.2599999999947));
#31236=CARTESIAN_POINT('Ctrl Pts',(1.37467804558015,70.4378582683016,-63.2599999999947));
#31237=CARTESIAN_POINT('Ctrl Pts',(0.727224534423085,70.4951788900757,-63.2002681824217));
#31238=CARTESIAN_POINT('Ctrl Pts',(-0.558312959174255,70.5042267042902,
-62.9493716889925));
#31239=CARTESIAN_POINT('Ctrl Pts',(-1.19640226162106,70.4560846742305,-62.7582390058393));
#31240=CARTESIAN_POINT('Ctrl Pts',(-2.80448010483271,70.2113780440741,-62.0965365584756));
#31241=CARTESIAN_POINT('Ctrl Pts',(-3.72705357784681,69.9369699535809,-61.5204719079205));
#31242=CARTESIAN_POINT('Ctrl Pts',(-4.4999999999832,69.6242977306852,-60.8593420767994));
#31243=CARTESIAN_POINT('',(-6.66025403785039,70.5000000000327,-58.2599999999947));
#31244=CARTESIAN_POINT('Origin',(8.99999999999307,80.7485954613122,-137.259999999996));
#31245=CARTESIAN_POINT('',(13.499999999994,69.6242977306784,-53.3414157129525));
#31246=CARTESIAN_POINT('Origin',(9.00000000008001,80.748595461022,-61.1356443468633));
#31247=CARTESIAN_POINT('',(13.499999999994,69.6242977306697,-131.178584287037));
#31248=CARTESIAN_POINT('',(13.4999999999941,69.624297730669,-137.259999999995));
#31249=CARTESIAN_POINT('',(10.6602540378385,68.8640022192282,-126.259999999995));
#31250=CARTESIAN_POINT('Origin',(8.99999999987123,80.7485954618345,-123.384355652776));
#31251=CARTESIAN_POINT('',(4.49999999999396,69.62429773067,-121.577541634476));
#31252=CARTESIAN_POINT('Ctrl Pts',(10.6602540378386,68.8640022192282,-126.259999999995));
#31253=CARTESIAN_POINT('Ctrl Pts',(10.6511405690506,68.8627290857649,-126.24421500902));
#31254=CARTESIAN_POINT('Ctrl Pts',(10.6420002974861,68.8614628960272,-126.228483263499));
#31255=CARTESIAN_POINT('Ctrl Pts',(10.219407479571,68.8034210642394,-125.505671077853));
#31256=CARTESIAN_POINT('Ctrl Pts',(9.67726187597146,68.7512246263665,-124.79116967751));
#31257=CARTESIAN_POINT('Ctrl Pts',(8.4193522322561,68.7461607613385,-123.54131924113));
#31258=CARTESIAN_POINT('Ctrl Pts',(7.70358433234451,68.7975084367052,-123.00596056583));
#31259=CARTESIAN_POINT('Ctrl Pts',(6.26432228327072,69.040788125594,-122.175002234363));
#31260=CARTESIAN_POINT('Ctrl Pts',(5.42432246719667,69.2588498443473,-121.825186221089));
#31261=CARTESIAN_POINT('Ctrl Pts',(4.56168799981022,69.5994929078332,-121.593626545806));
#31262=CARTESIAN_POINT('Ctrl Pts',(4.53083553750895,69.6118241415791,-121.585503336027));
#31263=CARTESIAN_POINT('Ctrl Pts',(4.49999999998978,69.6242977306718,-121.577541634475));
#31264=CARTESIAN_POINT('',(4.49999999999401,69.6242977306683,-137.259999999995));
#31265=CARTESIAN_POINT('Origin',(1.11022302462516E-12,-11.1689999999848,
-213.999999999986));
#31266=CARTESIAN_POINT('',(-59.3192302506006,22.0759834182112,-211.880711975822));
#31267=CARTESIAN_POINT('',(-59.3192302505947,-44.4139834181905,-211.880711975815));
#31268=CARTESIAN_POINT('Origin',(1.11022302462516E-12,-11.1689999999845,
-211.880711975818));
#31269=CARTESIAN_POINT('',(-58.1696747238564,-60.8533933496133,-213.999999999979));
#31270=CARTESIAN_POINT('Ctrl Pts',(-59.3192302505947,-44.4139834181905,
-211.880711975815));
#31271=CARTESIAN_POINT('Ctrl Pts',(-58.7782629438943,-52.1501763270953,
-212.706060413095));
#31272=CARTESIAN_POINT('Ctrl Pts',(-58.1696747238564,-60.8533933496133,
-213.99999999998));
#31273=CARTESIAN_POINT('',(-49.6843933496171,-69.3386747238511,-213.999999999978));
#31274=CARTESIAN_POINT('Origin',(1.11022302462516E-12,-11.1689999999848,
-213.999999999986));
#31275=CARTESIAN_POINT('',(-33.2449834181943,-70.4882302505863,-211.880711975812));
#31276=CARTESIAN_POINT('Ctrl Pts',(-49.684393349617,-69.3386747238512,-213.999999999979));
#31277=CARTESIAN_POINT('Ctrl Pts',(-40.9811763270991,-69.9472629438874,
-212.706060413093));
#31278=CARTESIAN_POINT('Ctrl Pts',(-33.2449834181943,-70.4882302505863,
-211.880711975812));
#31279=CARTESIAN_POINT('',(33.2449834182069,-70.4882302505805,-211.880711975812));
#31280=CARTESIAN_POINT('Origin',(1.11022302462516E-12,-11.1689999999845,
-211.880711975818));
#31281=CARTESIAN_POINT('',(49.6843933496294,-69.3386747238425,-213.999999999978));
#31282=CARTESIAN_POINT('Ctrl Pts',(33.2449834182069,-70.4882302505805,-211.880711975812));
#31283=CARTESIAN_POINT('Ctrl Pts',(40.9811763271116,-69.9472629438803,-212.706060413093));
#31284=CARTESIAN_POINT('Ctrl Pts',(49.6843933496294,-69.3386747238425,-213.999999999979));
#31285=CARTESIAN_POINT('',(58.1696747238672,-60.8533933496032,-213.999999999979));
#31286=CARTESIAN_POINT('Origin',(1.11022302462516E-12,-11.1689999999848,
-213.999999999986));
#31287=CARTESIAN_POINT('',(59.3192302506027,-44.4139834181802,-211.880711975815));
#31288=CARTESIAN_POINT('Ctrl Pts',(58.1696747238672,-60.8533933496032,-213.99999999998));
#31289=CARTESIAN_POINT('Ctrl Pts',(58.7782629439037,-52.1501763270851,-212.706060413095));
#31290=CARTESIAN_POINT('Ctrl Pts',(59.3192302506027,-44.4139834181801,-211.880711975815));
#31291=CARTESIAN_POINT('',(68.0000000000011,-11.1689999999786,-211.880711975818));
#31292=CARTESIAN_POINT('Origin',(1.11022302462516E-12,-11.1689999999845,
-211.880711975818));
#31293=CARTESIAN_POINT('',(76.5000000000011,-11.1689999999781,-213.999999999986));
#31294=CARTESIAN_POINT('',(-52.4384165089406,-42.6312331099945,-210.173502450762));
#31295=CARTESIAN_POINT('Ctrl Pts',(-52.4384165089405,-42.6312331099945,
-210.173502450762));
#31296=CARTESIAN_POINT('Ctrl Pts',(-48.3519683114706,-40.9385708446668,
-209.082698564953));
#31297=CARTESIAN_POINT('Ctrl Pts',(-44.8103167727301,-39.4715707441205,
-208.140791933166));
#31298=CARTESIAN_POINT('',(-59.3267182915137,-26.0014015247919,-210.173502450764));
#31299=CARTESIAN_POINT('Ctrl Pts',(-52.4384165089406,-42.6312331099944,
-210.173502450762));
#31300=CARTESIAN_POINT('Ctrl Pts',(-55.9844712211047,-34.3585272620583,
-209.870455963678));
#31301=CARTESIAN_POINT('Ctrl Pts',(-59.3267182915136,-26.0014015247919,
-210.173502450764));
#31302=CARTESIAN_POINT('Ctrl Pts',(-59.3267182915137,-26.0014015247919,
-210.173502450764));
#31303=CARTESIAN_POINT('Ctrl Pts',(-55.2402700940438,-24.3087392594642,
-209.082698564955));
#31304=CARTESIAN_POINT('Ctrl Pts',(-51.6986185553031,-22.8417391589179,
-208.140791933168));
#31305=CARTESIAN_POINT('',(59.3192302505969,22.0759834182214,-211.880711975822));
#31306=CARTESIAN_POINT('Origin',(1.11022302462516E-12,-11.1689999999845,
-211.880711975818));
#31307=CARTESIAN_POINT('',(58.1696747238586,38.5153933496439,-213.999999999991));
#31308=CARTESIAN_POINT('Ctrl Pts',(59.3192302505969,22.0759834182215,-211.880711975822));
#31309=CARTESIAN_POINT('Ctrl Pts',(58.7782629438965,29.8121763271262,-212.706060413104));
#31310=CARTESIAN_POINT('Ctrl Pts',(58.1696747238585,38.5153933496438,-213.999999999991));
#31311=CARTESIAN_POINT('',(49.6843933496193,47.0006747238816,-213.999999999992));
#31312=CARTESIAN_POINT('Origin',(1.11022302462516E-12,-11.1689999999848,
-213.999999999986));
#31313=CARTESIAN_POINT('',(33.2449834181965,48.1502302506173,-211.880711975825));
#31314=CARTESIAN_POINT('Ctrl Pts',(49.6843933496193,47.0006747238816,-213.999999999992));
#31315=CARTESIAN_POINT('Ctrl Pts',(40.9811763271013,47.6092629439181,-212.706060413106));
#31316=CARTESIAN_POINT('Ctrl Pts',(33.2449834181965,48.1502302506173,-211.880711975825));
#31317=CARTESIAN_POINT('',(-33.2449834182046,48.1502302506115,-211.880711975825));
#31318=CARTESIAN_POINT('Origin',(1.11022302462516E-12,-11.1689999999845,
-211.880711975818));
#31319=CARTESIAN_POINT('',(-49.6843933496272,47.000674723873,-213.999999999992));
#31320=CARTESIAN_POINT('Ctrl Pts',(-33.2449834182046,48.1502302506115,-211.880711975825));
#31321=CARTESIAN_POINT('Ctrl Pts',(-40.9811763271093,47.609262943911,-212.706060413106));
#31322=CARTESIAN_POINT('Ctrl Pts',(-49.6843933496272,47.000674723873,-213.999999999992));
#31323=CARTESIAN_POINT('',(-58.169674723865,38.5153933496337,-213.999999999991));
#31324=CARTESIAN_POINT('Origin',(1.11022302462516E-12,-11.1689999999848,
-213.999999999986));
#31325=CARTESIAN_POINT('Ctrl Pts',(-58.169674723865,38.5153933496337,-213.999999999991));
#31326=CARTESIAN_POINT('Ctrl Pts',(-58.7782629439015,29.8121763271159,-212.706060413104));
#31327=CARTESIAN_POINT('Ctrl Pts',(-59.3192302506005,22.0759834182111,-211.880711975822));
#31328=CARTESIAN_POINT('',(-59.2516966812877,-34.5416704979166,-210.807339776632));
#31329=CARTESIAN_POINT('',(-58.341412086245,-36.6160882438761,-210.796041473035));
#31330=CARTESIAN_POINT('Ctrl Pts',(-59.2516966813201,-34.5416704957383,
-210.807339776229));
#31331=CARTESIAN_POINT('Ctrl Pts',(-59.029454981385,-34.5478031947605,-210.75635515438));
#31332=CARTESIAN_POINT('Ctrl Pts',(-58.7921795388409,-34.5649224930198,
-210.702930314816));
#31333=CARTESIAN_POINT('Ctrl Pts',(-58.4366785026112,-34.6298287310412,
-210.626651867582));
#31334=CARTESIAN_POINT('Ctrl Pts',(-58.312197261563,-34.6607888434274,-210.600732341974));
#31335=CARTESIAN_POINT('Ctrl Pts',(-58.0781686614658,-34.747530321667,-210.554747021162));
#31336=CARTESIAN_POINT('Ctrl Pts',(-57.9682517418723,-34.8022087259218,
-210.534489049959));
#31337=CARTESIAN_POINT('Ctrl Pts',(-57.8331509870804,-34.9164071144292,
-210.514115724432));
#31338=CARTESIAN_POINT('Ctrl Pts',(-57.7935864618605,-34.9574272928331,
-210.508879171898));
#31339=CARTESIAN_POINT('Ctrl Pts',(-57.7287600318386,-35.0494073869723,
-210.502685784877));
#31340=CARTESIAN_POINT('Ctrl Pts',(-57.7036583364591,-35.1004833661575,
-210.501777404252));
#31341=CARTESIAN_POINT('Ctrl Pts',(-57.6694577754129,-35.2056166064024,
-210.503965499983));
#31342=CARTESIAN_POINT('Ctrl Pts',(-57.6596154308036,-35.2682318542073,
-210.507714108404));
#31343=CARTESIAN_POINT('Ctrl Pts',(-57.6582870250246,-35.3939331364455,
-210.519521527325));
#31344=CARTESIAN_POINT('Ctrl Pts',(-57.6664633243023,-35.4570226989156,
-210.527502248886));
#31345=CARTESIAN_POINT('Ctrl Pts',(-57.7016594788991,-35.621513122669,-210.551534754846));
#31346=CARTESIAN_POINT('Ctrl Pts',(-57.7386665647023,-35.7159198006795,
-210.569232984154));
#31347=CARTESIAN_POINT('Ctrl Pts',(-57.8204746085682,-35.8913905023802,
-210.605154351717));
#31348=CARTESIAN_POINT('Ctrl Pts',(-57.8659994434101,-35.9720888655669,
-210.623510416932));
#31349=CARTESIAN_POINT('Ctrl Pts',(-58.0089417708346,-36.2023684566477,
-210.678918981039));
#31350=CARTESIAN_POINT('Ctrl Pts',(-58.1120369384791,-36.3394897776198,
-210.716089360605));
#31351=CARTESIAN_POINT('Ctrl Pts',(-58.2591150958127,-36.5199599816261,
-210.767655854534));
#31352=CARTESIAN_POINT('Ctrl Pts',(-58.3000784572093,-36.5684840123265,
-210.781850056857));
#31353=CARTESIAN_POINT('Ctrl Pts',(-58.3414120848803,-36.6160882451689,
-210.796041472673));
#31354=CARTESIAN_POINT('Ctrl Pts',(-58.3414120868986,-36.616088244313,-210.796041473049));
#31355=CARTESIAN_POINT('Ctrl Pts',(-58.5196070612518,-36.3488442716846,
-210.810126004893));
#31356=CARTESIAN_POINT('Ctrl Pts',(-58.6856862024724,-36.0599520454846,
-210.819863004671));
#31357=CARTESIAN_POINT('Ctrl Pts',(-59.0239120577606,-35.331588505113,-210.827688366328));
#31358=CARTESIAN_POINT('Ctrl Pts',(-59.1566032891731,-34.9319981002169,
-210.82099539984));
#31359=CARTESIAN_POINT('Ctrl Pts',(-59.2516966823843,-34.5416704981807,
-210.807339776699));
#31360=CARTESIAN_POINT('Origin',(-59.506244168816,-35.8520251485972,-203.77397811514));
#31361=CARTESIAN_POINT('',(-54.7302932280859,-40.0172481069749,-207.104324991779));
#31362=CARTESIAN_POINT('',(-61.6687352492389,-30.9288598303485,-199.047872363436));
#31363=CARTESIAN_POINT('Origin',(-58.1950257608775,-35.2740441834793,-203.296733644058));
#31364=CARTESIAN_POINT('',(-61.0274459660746,-28.8726777694807,-203.299999999994));
#31365=CARTESIAN_POINT('Origin',(-58.2040000000275,-35.2780000000021,-203.299999999994));
#31366=CARTESIAN_POINT('',(-63.6319343036514,-30.0207280666708,-204.247956230286));
#31367=CARTESIAN_POINT('',(-62.3296901348632,-29.4467029180758,-203.77397811514));
#31368=CARTESIAN_POINT('Origin',(-60.8084883376043,-36.4260502971922,-204.247956230285));
#31369=CARTESIAN_POINT('Origin',(-60.8084883376043,-36.4260502971922,-204.247956230285));
#31370=CARTESIAN_POINT('Origin',(-58.2040000000275,-35.2780000000021,-203.299999999994));
#31371=CARTESIAN_POINT('Origin',(26.9999999999931,80.7485954613137,-137.259999999996));
#31372=CARTESIAN_POINT('',(31.499999999994,69.6242977306766,-84.2599999999946));
#31373=CARTESIAN_POINT('',(22.4999999999941,69.6242977306758,-84.2599999999946));
#31374=CARTESIAN_POINT('Origin',(26.9999999999931,80.7485954613196,-84.2599999999958));
#31375=CARTESIAN_POINT('',(31.499999999994,69.6242977306748,-100.259999999995));
#31376=CARTESIAN_POINT('',(31.499999999994,69.6242977306707,-137.259999999995));
#31377=CARTESIAN_POINT('',(22.4999999999941,69.624297730674,-100.259999999995));
#31378=CARTESIAN_POINT('Origin',(26.9999999999931,80.7485954613179,-100.259999999996));
#31379=CARTESIAN_POINT('',(22.4999999999941,69.6242977306698,-137.259999999995));
#31380=CARTESIAN_POINT('Origin',(1.11022302462516E-12,-11.1689999999872,
-235.499999999986));
#31381=CARTESIAN_POINT('',(32.4575348647363,48.5847315195132,-232.499999999992));
#31382=CARTESIAN_POINT('',(-32.4575348647446,48.5847315195076,-232.499999999992));
#31383=CARTESIAN_POINT('Origin',(1.11022302462516E-12,-11.1689999999869,
-232.499999999986));
#31384=CARTESIAN_POINT('',(-32.4575348647445,48.5847315195081,-227.499999999992));
#31385=CARTESIAN_POINT('',(-32.4575348647446,48.5847315195072,-235.499999999992));
#31386=CARTESIAN_POINT('',(-33.2449834182046,48.1502302506097,-227.499999999992));
#31387=CARTESIAN_POINT('Origin',(1.11022302462516E-12,-11.1689999999863,
-227.499999999986));
#31388=CARTESIAN_POINT('',(-33.2449834182046,48.150230250612,-207.499999999949));
#31389=CARTESIAN_POINT('',(33.2449834181965,48.1502302506155,-227.499999999992));
#31390=CARTESIAN_POINT('',(33.2449834181965,48.1502302506146,-235.499999999992));
#31391=CARTESIAN_POINT('',(32.4575348647363,48.5847315195138,-227.499999999992));
#31392=CARTESIAN_POINT('Origin',(1.11022302462516E-12,-11.1689999999863,
-227.499999999986));
#31393=CARTESIAN_POINT('',(32.4575348647363,48.5847315195129,-235.499999999992));
#31394=CARTESIAN_POINT('Origin',(-60.8084883376896,-36.4260502972298,-204.247956230316));
#31395=CARTESIAN_POINT('',(-64.0967476590949,-31.3184575319747,-204.563941640371));
#31396=CARTESIAN_POINT('',(-63.6319343036976,-30.0207280667973,-204.247956230317));
#31397=CARTESIAN_POINT('Origin',(-61.6766511167642,-36.8087337295747,-204.56394164037));
#31398=CARTESIAN_POINT('Origin',(6.77236045021346E-12,-76.1689999999813,
-183.999999999978));
#31399=CARTESIAN_POINT('',(7.12190442787529E-12,-80.1689999999816,-186.499999999978));
#31400=CARTESIAN_POINT('Origin',(6.77236045021346E-12,-76.1689999999816,
-186.499999999978));
#31401=CARTESIAN_POINT('',(7.12190442787524E-12,-80.168999999981,-181.499999999978));
#31402=CARTESIAN_POINT('',(7.12190442787527E-12,-80.1689999999813,-183.999999999978));
#31403=CARTESIAN_POINT('Origin',(6.77236045021346E-12,-76.168999999981,
-181.499999999978));
#31404=CARTESIAN_POINT('Origin',(65.0000000000011,-11.1689999999756,-183.999999999986));
#31405=CARTESIAN_POINT('',(65.0000000000014,-15.1689999999759,-186.499999999985));
#31406=CARTESIAN_POINT('Origin',(65.0000000000011,-11.1689999999759,-186.499999999986));
#31407=CARTESIAN_POINT('',(65.0000000000014,-15.1689999999753,-181.499999999985));
#31408=CARTESIAN_POINT('',(65.0000000000014,-15.1689999999756,-183.999999999985));
#31409=CARTESIAN_POINT('Origin',(65.0000000000011,-11.1689999999753,-181.499999999986));
#31410=CARTESIAN_POINT('Origin',(-4.57966997657877E-12,53.8310000000187,
-183.999999999993));
#31411=CARTESIAN_POINT('',(-4.23012599891694E-12,49.8310000000184,-186.499999999993));
#31412=CARTESIAN_POINT('Origin',(-4.57966997657877E-12,53.8310000000184,
-186.499999999993));
#31413=CARTESIAN_POINT('',(-4.23012599891699E-12,49.831000000019,-181.499999999993));
#31414=CARTESIAN_POINT('',(-4.23012599891696E-12,49.8310000000187,-183.999999999993));
#31415=CARTESIAN_POINT('Origin',(-4.57966997657877E-12,53.831000000019,
-181.499999999993));
#31416=CARTESIAN_POINT('Origin',(-64.9999999999989,-11.1689999999869,-183.999999999986));
#31417=CARTESIAN_POINT('',(-64.9999999999986,-15.1689999999872,-186.499999999985));
#31418=CARTESIAN_POINT('Origin',(-64.9999999999989,-11.1689999999873,-186.499999999986));
#31419=CARTESIAN_POINT('',(-64.9999999999986,-15.1689999999867,-181.499999999985));
#31420=CARTESIAN_POINT('',(-64.9999999999986,-15.1689999999869,-183.999999999985));
#31421=CARTESIAN_POINT('Origin',(-64.9999999999989,-11.1689999999867,-181.499999999986));
#31422=CARTESIAN_POINT('Origin',(1.11022302462516E-13,4.3869638824412E-11,
34.5000000000134));
#31423=CARTESIAN_POINT('',(-1.41067854607095E-12,17.4625000000399,1.13953291247526E-11));
#31424=CARTESIAN_POINT('Origin',(1.11022302462516E-13,3.99005915113771E-11,
1.34059430223488E-11));
#31425=CARTESIAN_POINT('',(-1.41067854607102E-12,17.4625000000407,7.0000000000114));
#31426=CARTESIAN_POINT('',(-1.41067854607129E-12,17.4625000000439,34.5000000000114));
#31427=CARTESIAN_POINT('',(3.96999999999864,17.0052346720472,7.00000000001144));
#31428=CARTESIAN_POINT('Origin',(1.11022302462516E-13,4.07055032042302E-11,
7.00000000001341));
#31429=CARTESIAN_POINT('',(3.96999999999864,17.0052346720536,63.0000000000114));
#31430=CARTESIAN_POINT('',(3.96999999999864,17.0052346720503,34.5000000000115));
#31431=CARTESIAN_POINT('',(-1.41067854607158E-12,17.4625000000471,63.0000000000114));
#31432=CARTESIAN_POINT('Origin',(1.11022302462516E-13,4.71447967470562E-11,
63.0000000000134));
#31433=CARTESIAN_POINT('',(-1.41067854607164E-12,17.4625000000478,69.0000000000114));
#31434=CARTESIAN_POINT('',(-1.41067854607129E-12,17.4625000000439,34.5000000000114));
#31435=CARTESIAN_POINT('Origin',(1.11022302462516E-13,4.78386861374469E-11,
69.0000000000134));
#31436=CARTESIAN_POINT('',(-3.97000000000136,17.005234672053,63.0000000000114));
#31437=CARTESIAN_POINT('Origin',(1.11022302462516E-13,4.71447967470562E-11,
63.0000000000134));
#31438=CARTESIAN_POINT('',(-3.97000000000136,17.0052346720466,7.00000000001144));
#31439=CARTESIAN_POINT('',(-3.97000000000136,17.0052346720497,34.5000000000115));
#31440=CARTESIAN_POINT('Origin',(1.11022302462516E-13,4.07055032042302E-11,
7.00000000001341));
#31441=CARTESIAN_POINT('Origin',(26.999999999994,70.5000000000298,-110.759999999995));
#31442=CARTESIAN_POINT('',(26.9999999999943,67.0000000000306,-102.759999999994));
#31443=CARTESIAN_POINT('Origin',(26.9999999999943,67.0000000000297,-110.759999999994));
#31444=CARTESIAN_POINT('',(26.999999999994,70.5000000000306,-102.759999999995));
#31445=CARTESIAN_POINT('',(26.999999999994,70.5000000000307,-102.759999999995));
#31446=CARTESIAN_POINT('Origin',(26.999999999994,70.5000000000297,-110.759999999995));
#31447=CARTESIAN_POINT('Origin',(26.9899999999939,70.5000000000338,-73.7599999999947));
#31448=CARTESIAN_POINT('',(26.9899999999943,67.0000000000347,-65.7599999999943));
#31449=CARTESIAN_POINT('Origin',(26.9899999999942,67.0000000000338,-73.7599999999943));
#31450=CARTESIAN_POINT('',(26.9899999999939,70.5000000000348,-65.7599999999947));
#31451=CARTESIAN_POINT('',(26.9899999999939,70.5000000000347,-65.7599999999947));
#31452=CARTESIAN_POINT('Origin',(26.9899999999939,70.5000000000339,-73.7599999999947));
#31453=CARTESIAN_POINT('Origin',(1.11022302462516E-13,4.78386861374469E-11,
69.0000000000134));
#31454=CARTESIAN_POINT('',(-1.32353748101568E-12,16.4625000000479,70.0000000000115));
#31455=CARTESIAN_POINT('',(-1.41067854607129E-12,17.4625000000478,69.0000000000114));
#31456=CARTESIAN_POINT('Origin',(1.11022302462516E-13,4.79774640155251E-11,
70.0000000000134));
#31457=CARTESIAN_POINT('Origin',(26.9999999999943,67.0000000000295,-110.759999999994));
#31458=CARTESIAN_POINT('',(26.9999999999943,67.0000000000289,-117.759999999994));
#31459=CARTESIAN_POINT('Origin',(26.9999999999943,67.0000000000297,-110.759999999994));
#31460=CARTESIAN_POINT('',(26.9999999999939,71.0000000000287,-117.759999999995));
#31461=CARTESIAN_POINT('',(26.9999999999943,67.0000000000287,-117.759999999994));
#31462=CARTESIAN_POINT('Origin',(26.9999999999939,71.0000000000295,-110.759999999995));
#31463=CARTESIAN_POINT('Origin',(26.9899999999942,67.0000000000338,-73.7599999999943));
#31464=CARTESIAN_POINT('',(26.9899999999942,67.000000000033,-80.7599999999943));
#31465=CARTESIAN_POINT('Origin',(26.9899999999942,67.0000000000338,-73.7599999999943));
#31466=CARTESIAN_POINT('',(26.9899999999939,71.000000000033,-80.7599999999948));
#31467=CARTESIAN_POINT('',(26.9899999999942,67.000000000033,-80.7599999999943));
#31468=CARTESIAN_POINT('Origin',(26.9899999999939,71.0000000000338,-73.7599999999948));
#31469=CARTESIAN_POINT('Origin',(-50.5581348548326,-61.7271348548489,-400.985281374227));
#31470=CARTESIAN_POINT('',(-50.5581348548323,-64.7271348548299,-235.499999999979));
#31471=CARTESIAN_POINT('Origin',(-50.5581348548326,-61.7271348548299,-235.49999999998));
#31472=CARTESIAN_POINT('',(-50.5581348548323,-64.7271348548479,-392.499999999979));
#31473=CARTESIAN_POINT('',(-50.5581348548323,-64.7271348548489,-400.985281374226));
#31474=CARTESIAN_POINT('Origin',(-50.5581348548326,-61.7271348548479,-392.49999999998));
#31475=CARTESIAN_POINT('Origin',(-50.5581348548387,39.3891348548274,-400.985281374238));
#31476=CARTESIAN_POINT('',(-50.5581348548384,36.3891348548434,-235.499999999991));
#31477=CARTESIAN_POINT('Origin',(-50.5581348548387,39.3891348548464,-235.499999999991));
#31478=CARTESIAN_POINT('',(-50.5581348548384,36.3891348548253,-392.499999999991));
#31479=CARTESIAN_POINT('',(-50.5581348548384,36.3891348548243,-400.985281374238));
#31480=CARTESIAN_POINT('Origin',(-50.5581348548387,39.3891348548284,-392.499999999991));
#31481=CARTESIAN_POINT('Origin',(50.5581348548376,39.3891348548335,-400.985281374238));
#31482=CARTESIAN_POINT('',(50.5581348548379,36.3891348548505,-235.499999999991));
#31483=CARTESIAN_POINT('Origin',(50.5581348548376,39.3891348548526,-235.499999999991));
#31484=CARTESIAN_POINT('',(50.5581348548379,36.3891348548324,-392.499999999991));
#31485=CARTESIAN_POINT('',(50.5581348548379,36.3891348548314,-400.985281374238));
#31486=CARTESIAN_POINT('Origin',(50.5581348548376,39.3891348548345,-392.499999999991));
#31487=CARTESIAN_POINT('Origin',(50.5581348548437,-61.7271348548428,-400.985281374227));
#31488=CARTESIAN_POINT('',(50.558134854844,-64.727134854823,-235.499999999979));
#31489=CARTESIAN_POINT('Origin',(50.5581348548437,-61.7271348548237,-235.49999999998));
#31490=CARTESIAN_POINT('',(50.558134854844,-64.7271348548411,-392.499999999979));
#31491=CARTESIAN_POINT('',(50.558134854844,-64.7271348548421,-400.985281374226));
#31492=CARTESIAN_POINT('Origin',(50.5581348548437,-61.7271348548418,-392.49999999998));
#31493=CARTESIAN_POINT('Origin',(1.11022302462516E-12,-11.1690000000053,
-392.499999999986));
#31494=CARTESIAN_POINT('',(32.4575348647468,-70.9227315195001,-395.499999999979));
#31495=CARTESIAN_POINT('',(-32.4575348647341,-70.9227315195058,-395.499999999979));
#31496=CARTESIAN_POINT('Origin',(1.11022302462516E-12,-11.1690000000057,
-395.499999999985));
#31497=CARTESIAN_POINT('',(-32.4575348647341,-70.9227315195064,-400.499999999979));
#31498=CARTESIAN_POINT('',(-32.4575348647342,-70.9227315195055,-392.499999999978));
#31499=CARTESIAN_POINT('',(32.4575348647468,-70.9227315195007,-400.499999999979));
#31500=CARTESIAN_POINT('Origin',(1.11022302462516E-12,-11.1690000000062,
-400.499999999986));
#31501=CARTESIAN_POINT('',(32.4575348647468,-70.9227315194997,-392.499999999978));
#31502=CARTESIAN_POINT('Origin',(1.11022302462516E-13,4.71170411714406E-11,
62.6499999999764));
#31503=CARTESIAN_POINT('',(-4.77179886666E-13,6.75000000008227,60.5000000000126));
#31504=CARTESIAN_POINT('',(-4.77179886666022E-13,6.75000000008252,62.6499999999756));
#31505=CARTESIAN_POINT('',(-6.75000000002784,4.62773855285951E-11,60.5000000000209));
#31506=CARTESIAN_POINT('Origin',(1.11022302462516E-13,4.68672409908999E-11,
60.5000000000134));
#31507=CARTESIAN_POINT('Origin',(1.11022302462516E-13,4.68672409908999E-11,
60.5000000000134));
#31508=CARTESIAN_POINT('Origin',(-871.,-11.1690000000814,-400.499999999982));
#31509=CARTESIAN_POINT('',(72.525443681756,-54.5019036555836,-427.999999999988));
#31510=CARTESIAN_POINT('',(72.5254436817485,32.1639036555757,-428.));
#31511=CARTESIAN_POINT('Origin',(-871.,-11.1690000000845,-427.99999999999));
#31512=CARTESIAN_POINT('',(73.0049525312962,32.1859258606169,-400.499999999992));
#31513=CARTESIAN_POINT('',(73.0049525312962,32.1859258606169,-400.499999999992));
#31514=CARTESIAN_POINT('',(73.004952531304,-54.5239258606185,-400.499999999982));
#31515=CARTESIAN_POINT('Origin',(-871.,-11.1690000000814,-400.499999999979));
#31516=CARTESIAN_POINT('',(73.004952531304,-54.5239258606185,-400.499999999984));
#31517=CARTESIAN_POINT('Origin',(1.11022302462516E-13,4.68672409908999E-11,
60.5000000000038));
#31518=CARTESIAN_POINT('',(5.91645271747417E-13,-5.49999999995327,59.2499999999771));
#31519=CARTESIAN_POINT('',(-5.4999999999835,4.62426359731071E-11,59.2499999999765));
#31520=CARTESIAN_POINT('Origin',(1.11022302462516E-13,4.67284631128218E-11,
59.2499999999765));
#31521=CARTESIAN_POINT('Origin',(1.11022302462516E-13,4.67284631128218E-11,
59.2499999999765));
#31522=CARTESIAN_POINT('',(-6.7500000000108,4.62773855285947E-11,60.5000000000038));
#31523=CARTESIAN_POINT('Origin',(1.11022302462516E-13,4.57570179662747E-11,
50.8000000000134));
#31524=CARTESIAN_POINT('',(-4.06739714446706E-13,5.50000000004478,42.3500000000128));
#31525=CARTESIAN_POINT('',(5.91645271747587E-13,-5.49999999995522,42.350000000014));
#31526=CARTESIAN_POINT('Origin',(1.11022302462516E-13,4.47855728197277E-11,
42.3500000000134));
#31527=CARTESIAN_POINT('Origin',(1.11022302462516E-13,4.47855728197277E-11,
42.3500000000134));
#31528=CARTESIAN_POINT('',(5.91645271747502E-13,-5.49999999995424,50.800000000014));
#31529=CARTESIAN_POINT('Origin',(-871.,-11.1690000000846,-427.999999999983));
#31530=CARTESIAN_POINT('',(70.7822037839096,-15.3837757183187,-439.937224614355));
#31531=CARTESIAN_POINT('',(70.7822037837444,-6.95422428207094,-439.937224614869));
#31532=CARTESIAN_POINT('Ctrl Pts',(70.7822037837443,-15.3837757179392,-439.937224614868));
#31533=CARTESIAN_POINT('Ctrl Pts',(70.7793815670799,-14.7181872564058,-440.26955676224));
#31534=CARTESIAN_POINT('Ctrl Pts',(70.7771136682848,-14.0238576141718,-440.537081066418));
#31535=CARTESIAN_POINT('Ctrl Pts',(70.7740765236161,-12.6025387021907,-440.895543254428));
#31536=CARTESIAN_POINT('Ctrl Pts',(70.773294912811,-11.8913254701458,-440.987905442524));
#31537=CARTESIAN_POINT('Ctrl Pts',(70.7732942454401,-10.4474454821257,-440.987984275525));
#31538=CARTESIAN_POINT('Ctrl Pts',(70.7740755308484,-9.73607650775737,-440.8956604892));
#31539=CARTESIAN_POINT('Ctrl Pts',(70.7771127074938,-8.31443689341987,-440.537194400521));
#31540=CARTESIAN_POINT('Ctrl Pts',(70.7793809661231,-7.61995447243546,-440.269627528263));
#31541=CARTESIAN_POINT('Ctrl Pts',(70.7822037837436,-6.9542242820708,-439.93722461487));
#31542=CARTESIAN_POINT('',(70.7804124467087,-3.96116868056053,-438.999999999988));
#31543=CARTESIAN_POINT('Ctrl Pts',(70.7822037837436,-6.95422428207028,-439.93722461487));
#31544=CARTESIAN_POINT('Ctrl Pts',(70.784260001646,-6.47662207653906,-439.696973540908));
#31545=CARTESIAN_POINT('Ctrl Pts',(70.7852286730449,-5.98180724382513,-439.493770109462));
#31546=CARTESIAN_POINT('Ctrl Pts',(70.7846425695099,-4.97817312280563,-439.179518622343));
#31547=CARTESIAN_POINT('Ctrl Pts',(70.7831704772474,-4.47390580694272,-439.066807118521));
#31548=CARTESIAN_POINT('Ctrl Pts',(70.7804124467078,-3.96116868056048,-438.999999999988));
#31549=CARTESIAN_POINT('',(70.761115158048,-1.77218793995686,-438.999999999987));
#31550=CARTESIAN_POINT('Origin',(-871.000107047341,-11.169000944124,-438.999998579555));
#31551=CARTESIAN_POINT('',(70.7115584312605,1.14064771598034,-439.915842225177));
#31552=CARTESIAN_POINT('Ctrl Pts',(70.7611151580471,-1.772187939957,-438.999999999989));
#31553=CARTESIAN_POINT('Ctrl Pts',(70.7549712858817,-1.2712400283809,-439.065619900641));
#31554=CARTESIAN_POINT('Ctrl Pts',(70.7477342419649,-0.778729462480956,
-439.175730874464));
#31555=CARTESIAN_POINT('Ctrl Pts',(70.7310929468594,0.198249032937304,-439.482912240457));
#31556=CARTESIAN_POINT('Ctrl Pts',(70.7217076382667,0.677934742452566,-439.68092633614));
#31557=CARTESIAN_POINT('Ctrl Pts',(70.7115584312596,1.14064771597983,-439.915842225178));
#31558=CARTESIAN_POINT('',(70.5621815020405,9.72878593023437,-439.798062313339));
#31559=CARTESIAN_POINT('Ctrl Pts',(70.7115584312596,1.14064771598,-439.915842225178));
#31560=CARTESIAN_POINT('Ctrl Pts',(70.6977555438623,1.7722760085199,-440.233574685584));
#31561=CARTESIAN_POINT('Ctrl Pts',(70.6841784180189,2.43135220063798,-440.481498690251));
#31562=CARTESIAN_POINT('Ctrl Pts',(70.6576559190849,3.79836391559058,-440.812682544676));
#31563=CARTESIAN_POINT('Ctrl Pts',(70.6450375971601,4.48847501002298,-440.893489401533));
#31564=CARTESIAN_POINT('Ctrl Pts',(70.6195899340406,5.95683448888694,-440.890104980619));
#31565=CARTESIAN_POINT('Ctrl Pts',(70.6072142402067,6.7166479370343,-440.788838196047));
#31566=CARTESIAN_POINT('Ctrl Pts',(70.5835347472419,8.24335729001911,-440.414736630433));
#31567=CARTESIAN_POINT('Ctrl Pts',(70.5724334125237,9.00060738974511,-440.13655505323));
#31568=CARTESIAN_POINT('Ctrl Pts',(70.5621815020397,9.72878593023391,-439.798062313338));
#31569=CARTESIAN_POINT('',(70.5123942581075,12.4256934496977,-438.999999999989));
#31570=CARTESIAN_POINT('Ctrl Pts',(70.5621815020397,9.72878593023386,-439.798062313338));
#31571=CARTESIAN_POINT('Ctrl Pts',(70.5560935286397,10.1630589717267,-439.594696903278));
#31572=CARTESIAN_POINT('Ctrl Pts',(70.5488623731821,10.6109112971744,-439.422304715381));
#31573=CARTESIAN_POINT('Ctrl Pts',(70.532189399423,11.5143833304763,-439.154979614465));
#31574=CARTESIAN_POINT('Ctrl Pts',(70.5228784997486,11.9667160576192,-439.058298484005));
#31575=CARTESIAN_POINT('Ctrl Pts',(70.5123942581067,12.4256934496978,-438.99999999999));
#31576=CARTESIAN_POINT('',(70.4593636589108,14.4545180952481,-438.999999999989));
#31577=CARTESIAN_POINT('Origin',(-871.000092098264,-11.1690024073961,-438.999997857804));
#31578=CARTESIAN_POINT('',(70.2929704410881,18.8989817281299,-441.000070380918));
#31579=CARTESIAN_POINT('Ctrl Pts',(70.4593636589101,14.454518095248,-438.99999999999));
#31580=CARTESIAN_POINT('Ctrl Pts',(70.4323968085906,15.3696263962396,-439.118003644213));
#31581=CARTESIAN_POINT('Ctrl Pts',(70.402361472674,16.2465973045633,-439.394182358811));
#31582=CARTESIAN_POINT('Ctrl Pts',(70.3451108148425,17.725685099839,-440.131591270883));
#31583=CARTESIAN_POINT('Ctrl Pts',(70.3190794500871,18.3352673501182,-440.536136589015));
#31584=CARTESIAN_POINT('Ctrl Pts',(70.292970440885,18.8989817282384,-441.000070380775));
#31585=CARTESIAN_POINT('',(69.7816652336224,32.0328182762798,-441.000100325617));
#31586=CARTESIAN_POINT('Ctrl Pts',(70.2929704408694,18.8989817281253,-441.000070381875));
#31587=CARTESIAN_POINT('Ctrl Pts',(70.2251073370001,21.0262639243397,-440.994959300743));
#31588=CARTESIAN_POINT('Ctrl Pts',(70.150003220528,23.1528067113153,-440.992592473935));
#31589=CARTESIAN_POINT('Ctrl Pts',(69.9804315445582,27.5309940661356,-440.992609031095));
#31590=CARTESIAN_POINT('Ctrl Pts',(69.8851070136805,29.7820605867228,-440.995276017104));
#31591=CARTESIAN_POINT('Ctrl Pts',(69.7816652336217,32.0328182762798,-441.000100325618));
#31592=CARTESIAN_POINT('',(70.0083439496798,32.0432276337977,-427.999999999994));
#31593=CARTESIAN_POINT('',(70.008342200333,32.0432275534655,-428.000100325617));
#31594=CARTESIAN_POINT('',(70.0083439496875,-54.3812276338044,-427.999999999984));
#31595=CARTESIAN_POINT('Origin',(-871.,-11.1690000000846,-427.999999999982));
#31596=CARTESIAN_POINT('',(69.7816652336299,-54.3708182762896,-441.000100325607));
#31597=CARTESIAN_POINT('',(70.0083439496874,-54.3812276338046,-427.999999999984));
#31598=CARTESIAN_POINT('',(70.2929704406237,-41.2369817304577,-441.000070382643));
#31599=CARTESIAN_POINT('Ctrl Pts',(69.7816652336292,-54.3708182762895,-441.000100325608));
#31600=CARTESIAN_POINT('Ctrl Pts',(69.8851070061175,-52.1200607514469,-440.995276017448));
#31601=CARTESIAN_POINT('Ctrl Pts',(69.9804315306073,-49.8689943957394,-440.992609031477));
#31602=CARTESIAN_POINT('Ctrl Pts',(70.1500033362218,-45.49080375343,-440.992592473549));
#31603=CARTESIAN_POINT('Ctrl Pts',(70.2251072266989,-43.3642673819341,-440.99495929243));
#31604=CARTESIAN_POINT('Ctrl Pts',(70.2929704408003,-41.2369817304615,-441.000070381863));
#31605=CARTESIAN_POINT('',(70.4593636589152,-36.7925180952641,-438.999999999984));
#31606=CARTESIAN_POINT('Ctrl Pts',(70.2929704407877,-41.2369817303642,-441.000070382765));
#31607=CARTESIAN_POINT('Ctrl Pts',(70.317704961237,-40.7029436632141,-440.560560029249));
#31608=CARTESIAN_POINT('Ctrl Pts',(70.3423766984901,-40.1275883461274,-440.17422668545));
#31609=CARTESIAN_POINT('Ctrl Pts',(70.399844103119,-38.6577652909441,-439.417647186168));
#31610=CARTESIAN_POINT('Ctrl Pts',(70.4312604023686,-37.7461955970541,-439.122967454739));
#31611=CARTESIAN_POINT('Ctrl Pts',(70.4593636589143,-36.7925180952639,-438.999999999984));
#31612=CARTESIAN_POINT('',(70.5123942581118,-34.7636934497019,-438.999999999984));
#31613=CARTESIAN_POINT('Origin',(-871.000092221015,-11.1689975899443,-438.99999810262));
#31614=CARTESIAN_POINT('',(70.5621815020439,-32.0667859302444,-439.798062313334));
#31615=CARTESIAN_POINT('Ctrl Pts',(70.5123942581109,-34.763693449702,-438.999999999984));
#31616=CARTESIAN_POINT('Ctrl Pts',(70.5244264243219,-34.2369512725135,-439.066905845301));
#31617=CARTESIAN_POINT('Ctrl Pts',(70.5349061547253,-33.7192548928422,-439.184327052031));
#31618=CARTESIAN_POINT('Ctrl Pts',(70.5508948328608,-32.8218972350616,-439.471919820818));
#31619=CARTESIAN_POINT('Ctrl Pts',(70.5569594113589,-32.4392930119041,-439.623621240154));
#31620=CARTESIAN_POINT('Ctrl Pts',(70.5621815020433,-32.0667859302438,-439.798062313332));
#31621=CARTESIAN_POINT('',(70.7115584312623,-23.4786477159905,-439.915842225175));
#31622=CARTESIAN_POINT('Ctrl Pts',(70.5621815020433,-32.066785930244,-439.798062313333));
#31623=CARTESIAN_POINT('Ctrl Pts',(70.579829006079,-30.8133089561511,-440.380739269272));
#31624=CARTESIAN_POINT('Ctrl Pts',(70.599849431034,-29.4823568207801,-440.780673806023));
#31625=CARTESIAN_POINT('Ctrl Pts',(70.6364529932775,-27.3071756279525,-440.924738336709));
#31626=CARTESIAN_POINT('Ctrl Pts',(70.6505405351955,-26.5176964957163,-440.873145899115));
#31627=CARTESIAN_POINT('Ctrl Pts',(70.6804876960852,-24.9493418204798,-440.547513202668));
#31628=CARTESIAN_POINT('Ctrl Pts',(70.6958611485221,-24.1969646600544,-440.277182292876));
#31629=CARTESIAN_POINT('Ctrl Pts',(70.7115584312618,-23.4786477159904,-439.915842225175));
#31630=CARTESIAN_POINT('',(70.7611151580495,-20.5658120600565,-438.999999999986));
#31631=CARTESIAN_POINT('Ctrl Pts',(70.7115584312618,-23.4786477159902,-439.915842225175));
#31632=CARTESIAN_POINT('Ctrl Pts',(70.7217087916647,-23.0158821579329,-439.680899639368));
#31633=CARTESIAN_POINT('Ctrl Pts',(70.7310950754517,-22.5361402088534,-439.482867337723));
#31634=CARTESIAN_POINT('Ctrl Pts',(70.7477359295614,-21.5591557455211,-439.175705187447));
#31635=CARTESIAN_POINT('Ctrl Pts',(70.7549720035577,-21.0667014551982,-439.065612235486));
#31636=CARTESIAN_POINT('Ctrl Pts',(70.7611151580486,-20.5658120600564,-438.999999999987));
#31637=CARTESIAN_POINT('',(70.7804124467098,-18.3768313194477,-438.999999999986));
#31638=CARTESIAN_POINT('Origin',(-871.000106910411,-11.1689990568951,-438.999998737379));
#31639=CARTESIAN_POINT('Ctrl Pts',(70.780412446709,-18.3768313194477,-438.999999999987));
#31640=CARTESIAN_POINT('Ctrl Pts',(70.7831704612649,-17.8640971645283,-439.066806731352));
#31641=CARTESIAN_POINT('Ctrl Pts',(70.7846425525253,-17.359832709541,-439.179517317669));
#31642=CARTESIAN_POINT('Ctrl Pts',(70.7852286838526,-16.3561982906056,-439.493767837466));
#31643=CARTESIAN_POINT('Ctrl Pts',(70.7842600131655,-15.8613805991198,-439.696972194992));
#31644=CARTESIAN_POINT('Ctrl Pts',(70.7822037837465,-15.383775718449,-439.937224614613));
#31645=CARTESIAN_POINT('Origin',(52.9999999999906,86.831000000001,-377.5));
#31646=CARTESIAN_POINT('',(53.9999999999878,95.6310000000053,-377.500000000001));
#31647=CARTESIAN_POINT('Origin',(53.9999999999885,86.831000000001,-377.5));
#31648=CARTESIAN_POINT('',(51.9999999999918,95.6310000000052,-377.500000000001));
#31649=CARTESIAN_POINT('',(52.9999999999898,95.6310000000053,-377.500000000001));
#31650=CARTESIAN_POINT('Origin',(51.9999999999926,86.831000000001,-377.5));
#31651=CARTESIAN_POINT('Origin',(52.9999999999906,86.8310000000061,-333.499999999996));
#31652=CARTESIAN_POINT('',(53.9999999999878,95.6310000000105,-333.499999999997));
#31653=CARTESIAN_POINT('Origin',(53.9999999999885,86.8310000000061,-333.499999999997));
#31654=CARTESIAN_POINT('',(51.9999999999918,95.6310000000103,-333.499999999997));
#31655=CARTESIAN_POINT('',(52.9999999999898,95.6310000000104,-333.499999999997));
#31656=CARTESIAN_POINT('Origin',(51.9999999999926,86.8310000000061,-333.499999999996));
#31657=CARTESIAN_POINT('Origin',(1.11022302462516E-13,4.46745505172652E-11,
41.4999999999416));
#31658=CARTESIAN_POINT('',(-4.42323460632396E-13,6.34999999994952,41.4999999999768));
#31659=CARTESIAN_POINT('',(-4.42323460635528E-13,6.34999999998547,41.4999999999408));
#31660=CARTESIAN_POINT('Origin',(1.11022302462516E-13,4.46745505172735E-11,
41.5000000000134));
#31661=CARTESIAN_POINT('Origin',(1.11022302462516E-13,4.52574176051934E-11,
46.6250000000134));
#31662=CARTESIAN_POINT('',(-3.68253555343357E-13,5.50000000004467,41.5000000000128));
#31663=CARTESIAN_POINT('Origin',(1.10718178859001E-13,4.46664927267193E-11,
41.5000000000134));
#31664=CARTESIAN_POINT('',(-3.68253555343282E-13,5.5000000000438,34.0000000000128));
#31665=CARTESIAN_POINT('',(-3.68253555343408E-13,5.50000000004526,46.6250000000128));
#31666=CARTESIAN_POINT('',(5.90298160273389E-13,-5.50000000001298,34.000000000014));
#31667=CARTESIAN_POINT('Origin',(1.11022302462516E-13,4.38141276731807E-11,
34.0000000000134));
#31668=CARTESIAN_POINT('Origin',(1.11022302462516E-13,4.38141276731807E-11,
34.0000000000134));
#31669=CARTESIAN_POINT('Origin',(125.,-11.169000000001,-461.499999999986));
#31670=CARTESIAN_POINT('',(-52.1061868616723,-40.3862650211908,-461.499999999981));
#31671=CARTESIAN_POINT('',(-52.1061868616775,18.0482650211561,-461.499999999988));
#31672=CARTESIAN_POINT('Origin',(125.000000000001,-11.1690000000008,-461.499999999987));
#31673=CARTESIAN_POINT('',(-52.1061868616723,-40.3862650211909,-462.499999999981));
#31674=CARTESIAN_POINT('',(-52.1061868616723,-40.3862650211908,-461.499999999982));
#31675=CARTESIAN_POINT('',(-52.1061868616775,18.0482650211559,-462.499999999988));
#31676=CARTESIAN_POINT('Origin',(125.000000000005,-11.1690000000027,-462.499999998938));
#31677=CARTESIAN_POINT('',(-52.1061868616775,18.0482650211561,-461.499999999988));
#31678=CARTESIAN_POINT('Origin',(1.11022302462516E-13,4.38141276731807E-11,
33.9999999998916));
#31679=CARTESIAN_POINT('',(1.11022302462543E-13,4.34973671664388E-11,31.2499999996439));
#31680=CARTESIAN_POINT('',(5.9164527173117E-13,-5.49999999976929,33.9999999998922));
#31681=CARTESIAN_POINT('Ctrl Pts',(-69.7885335814896,32.039936012842,-440.9823476426));
#31682=CARTESIAN_POINT('Ctrl Pts',(-69.7776904941909,32.0305578312519,-441.000027286454));
#31683=CARTESIAN_POINT('Ctrl Pts',(-69.5538754530634,37.1252327578524,-440.982079016193));
#31684=CARTESIAN_POINT('Ctrl Pts',(-69.5425906598027,37.113747189771,-440.99999999999));
#31685=CARTESIAN_POINT('Ctrl Pts',(-67.6435743056599,41.8415378856266,-440.982079016193));
#31686=CARTESIAN_POINT('Ctrl Pts',(-67.6327997693356,41.8281639590277,-440.99999999999));
#31687=CARTESIAN_POINT('Ctrl Pts',(-64.2753290142128,45.652151355614,-440.981957227449));
#31688=CARTESIAN_POINT('Ctrl Pts',(-64.2658958771893,45.637476314079,-440.999637204013));
#31689=CARTESIAN_POINT('',(-69.7776905149964,32.0305573814079,-441.000027286453));
#31690=CARTESIAN_POINT('',(-66.07358548387,43.2921573753126,-440.999810981737));
#31691=CARTESIAN_POINT('Origin',(-47.744837071413,30.9950012145811,-440.998278175537));
#31692=CARTESIAN_POINT('Ctrl Pts',(-66.07358548387,43.2921573753126,-440.999810981737));
#31693=CARTESIAN_POINT('Ctrl Pts',(-67.1868327014352,41.6282336258689,-440.99958021146));
#31694=CARTESIAN_POINT('Ctrl Pts',(-68.0685532114393,39.8205645108678,-440.999180312587));
#31695=CARTESIAN_POINT('Ctrl Pts',(-69.0695679316239,36.7792652847884,-440.998939961127));
#31696=CARTESIAN_POINT('Ctrl Pts',(-69.351131410688,35.6109067469029,-440.998942059551));
#31697=CARTESIAN_POINT('Ctrl Pts',(-69.6602915252648,33.6321769872792,-440.999335940571));
#31698=CARTESIAN_POINT('Ctrl Pts',(-69.7408627779659,32.8326707807528,-440.99959902782));
#31699=CARTESIAN_POINT('Ctrl Pts',(-69.7776892840197,32.0305577767104,-441.000029187691));
#31700=CARTESIAN_POINT('Ctrl Pts',(64.2809593455634,45.6547550552671,-440.98049740866));
#31701=CARTESIAN_POINT('Ctrl Pts',(64.2705054959308,45.6385004273605,-441.000078147052));
#31702=CARTESIAN_POINT('Ctrl Pts',(67.6447335076994,41.8429767487719,-440.980150947971));
#31703=CARTESIAN_POINT('Ctrl Pts',(67.6327997693276,41.8281639590396,-440.999999999992));
#31704=CARTESIAN_POINT('Ctrl Pts',(69.5550895522119,37.1264684578182,-440.980150947971));
#31705=CARTESIAN_POINT('Ctrl Pts',(69.5425906597955,37.1137471897833,-440.999999999992));
#31706=CARTESIAN_POINT('Ctrl Pts',(69.7936785182884,32.0432074888088,-440.980518645148));
#31707=CARTESIAN_POINT('Ctrl Pts',(69.7816652336223,32.0328182762799,-441.000100325617));
#31708=CARTESIAN_POINT('Origin',(47.8350487511125,31.0311022099888,-441.00118582651));
#31709=CARTESIAN_POINT('Ctrl Pts',(69.7816652336224,32.0328182762799,-441.000100325617));
#31710=CARTESIAN_POINT('Ctrl Pts',(69.7518843882855,32.6817941814599,-440.998904011986));
#31711=CARTESIAN_POINT('Ctrl Pts',(69.6934625136204,33.3291394297202,-440.997957204299));
#31712=CARTESIAN_POINT('Ctrl Pts',(69.5231554244232,34.5910307977996,-440.99650408746));
#31713=CARTESIAN_POINT('Ctrl Pts',(69.4135787649794,35.2052865159601,-440.995982544645));
#31714=CARTESIAN_POINT('Ctrl Pts',(69.1056439599675,36.589400265789,-440.995153783906));
#31715=CARTESIAN_POINT('Ctrl Pts',(68.8914233630438,37.3548496771541,-440.994944699506));
#31716=CARTESIAN_POINT('Ctrl Pts',(68.2710180729107,39.1849139644065,-440.994911067285));
#31717=CARTESIAN_POINT('Ctrl Pts',(67.8228059244791,40.2328726275071,-440.995291719939));
#31718=CARTESIAN_POINT('Ctrl Pts',(66.4689261490073,42.8241873584825,-440.996896227121));
#31719=CARTESIAN_POINT('Ctrl Pts',(65.4530647309365,44.3006265039595,-440.998470978792));
#31720=CARTESIAN_POINT('Ctrl Pts',(64.270505495931,45.6385004273601,-441.000078147052));
#31721=CARTESIAN_POINT('Ctrl Pts',(64.2705054959308,45.6385004273605,-441.000078147052));
#31722=CARTESIAN_POINT('Ctrl Pts',(52.7925979348309,27.7915710081813,-462.498943458995));
#31723=CARTESIAN_POINT('Ctrl Pts',(67.6327997693276,41.8281639590396,-440.999999999992));
#31724=CARTESIAN_POINT('Ctrl Pts',(54.7064708585553,25.7833181444813,-462.499999999991));
#31725=CARTESIAN_POINT('Ctrl Pts',(69.5425906597955,37.1137471897833,-440.999999999992));
#31726=CARTESIAN_POINT('Ctrl Pts',(56.0041009291211,23.3343857139696,-462.49999999999));
#31727=CARTESIAN_POINT('Ctrl Pts',(69.7816652336223,32.0328182762799,-441.000100325617));
#31728=CARTESIAN_POINT('Ctrl Pts',(56.5915605594642,20.6258796622937,-462.49999999999));
#31729=CARTESIAN_POINT('',(56.5915605594642,20.6258796622937,-462.49999999999));
#31730=CARTESIAN_POINT('',(69.7816652336224,32.0328182762798,-441.000100325617));
#31731=CARTESIAN_POINT('',(53.0296962895253,27.5362761699812,-462.499535472188));
#31732=CARTESIAN_POINT('Ctrl Pts',(53.0300419063622,27.5365540887963,-462.4990707585));
#31733=CARTESIAN_POINT('Ctrl Pts',(53.2015496317819,27.3480106076271,-462.49915996944));
#31734=CARTESIAN_POINT('Ctrl Pts',(53.3687845536093,27.1545069130794,-462.499240999659));
#31735=CARTESIAN_POINT('Ctrl Pts',(53.5313403519166,26.9563420647616,-462.499314432669));
#31736=CARTESIAN_POINT('Ctrl Pts',(53.6934013451948,26.7587804121745,-462.499387642156));
#31737=CARTESIAN_POINT('Ctrl Pts',(53.850811280172,26.5565861676637,-462.49945330107));
#31738=CARTESIAN_POINT('Ctrl Pts',(54.0031963229347,26.3500987421599,-462.49951205977));
#31739=CARTESIAN_POINT('Ctrl Pts',(54.1597252568381,26.1379961893595,-462.499572416329));
#31740=CARTESIAN_POINT('Ctrl Pts',(54.3109517332303,25.9213638896764,-462.499625492546));
#31741=CARTESIAN_POINT('Ctrl Pts',(54.4565083889137,25.7006130098379,-462.499672064642));
#31742=CARTESIAN_POINT('Ctrl Pts',(54.5976460796388,25.4865639218063,-462.499717222852));
#31743=CARTESIAN_POINT('Ctrl Pts',(54.7334528676258,25.2686430436956,-462.499756266788));
#31744=CARTESIAN_POINT('Ctrl Pts',(54.8636333433693,25.0472601517917,-462.499789960424));
#31745=CARTESIAN_POINT('Ctrl Pts',(54.9937540045974,24.825978979522,-462.499823638579));
#31746=CARTESIAN_POINT('Ctrl Pts',(55.1182532692508,24.6012393380423,-462.499851972027));
#31747=CARTESIAN_POINT('Ctrl Pts',(55.236879250096,24.3734796429302,-462.499875769413));
#31748=CARTESIAN_POINT('Ctrl Pts',(55.3555307652856,24.1456709223478,-462.49989957192));
#31749=CARTESIAN_POINT('Ctrl Pts',(55.4683062680139,23.9148412445512,-462.499918837139));
#31750=CARTESIAN_POINT('Ctrl Pts',(55.5750002656745,23.6814528220458,-462.499934409438));
#31751=CARTESIAN_POINT('Ctrl Pts',(55.6817890000358,23.4478571671789,-462.499949995564));
#31752=CARTESIAN_POINT('Ctrl Pts',(55.7824852825477,23.2116986428949,-462.499961882973));
#31753=CARTESIAN_POINT('Ctrl Pts',(55.8769322876267,22.9734581004061,-462.499970942341));
#31754=CARTESIAN_POINT('Ctrl Pts',(55.971639256022,22.7345618060333,-462.499980026645));
#31755=CARTESIAN_POINT('Ctrl Pts',(56.0600624058537,22.4935724529541,-462.499986268102));
#31756=CARTESIAN_POINT('Ctrl Pts',(56.1420948629952,22.2509859138938,-462.499990557135));
#31757=CARTESIAN_POINT('Ctrl Pts',(56.2242902121949,22.0079176701276,-462.499994854686));
#31758=CARTESIAN_POINT('Ctrl Pts',(56.3000694465316,21.7632463371213,-462.499997192841));
#31759=CARTESIAN_POINT('Ctrl Pts',(56.3693772469459,21.5174751624493,-462.499998468048));
#31760=CARTESIAN_POINT('Ctrl Pts',(56.4389505167557,21.2707626114129,-462.49999974814));
#31761=CARTESIAN_POINT('Ctrl Pts',(56.5020027183568,21.0229422220262,-462.499999957906));
#31762=CARTESIAN_POINT('Ctrl Pts',(56.5585303196142,20.7745207724168,-462.499999992997));
#31763=CARTESIAN_POINT('Ctrl Pts',(56.5697994701431,20.724996316258,-462.499999999993));
#31764=CARTESIAN_POINT('Ctrl Pts',(56.580809477877,20.6754479526699,-462.49999999999));
#31765=CARTESIAN_POINT('Ctrl Pts',(56.5915605594642,20.6258796622937,-462.49999999999));
#31766=CARTESIAN_POINT('Ctrl Pts',(53.030005423924,27.5365939049776,-462.499070944381));
#31767=CARTESIAN_POINT('Ctrl Pts',(53.5773086193955,28.4845508466792,-461.404278299304));
#31768=CARTESIAN_POINT('Ctrl Pts',(54.1393619772859,29.4580558191063,-460.280364313678));
#31769=CARTESIAN_POINT('Ctrl Pts',(55.3016968424015,31.4712788608959,-457.956521108394));
#31770=CARTESIAN_POINT('Ctrl Pts',(55.9376439432745,32.5727715505385,-456.685346754008));
#31771=CARTESIAN_POINT('Ctrl Pts',(56.5529890060882,33.6385804635187,-455.455487085885));
#31772=CARTESIAN_POINT('Ctrl Pts',(57.8778422943977,15.3629606180432,-462.504468150655));
#31773=CARTESIAN_POINT('Ctrl Pts',(57.8804420169269,15.3637472976184,-462.499999999989));
#31774=CARTESIAN_POINT('Ctrl Pts',(71.5535162631277,19.501120323523,-438.999979560409));
#31775=CARTESIAN_POINT('Ctrl Pts',(57.875348319425,15.354802038958,-462.504468081353));
#31776=CARTESIAN_POINT('Ctrl Pts',(57.8779477730967,15.3555885117513,-462.499999999989));
#31777=CARTESIAN_POINT('Ctrl Pts',(71.5498292133137,19.4919801773738,-438.999986373603));
#31778=CARTESIAN_POINT('Ctrl Pts',(57.8728543444523,15.3466434598728,-462.504468012053));
#31779=CARTESIAN_POINT('Ctrl Pts',(57.8754535292664,15.3474297258841,-462.499999999989));
#31780=CARTESIAN_POINT('Ctrl Pts',(71.5461421634996,19.4828400312246,-438.999993186796));
#31781=CARTESIAN_POINT('Ctrl Pts',(57.8703603694796,15.3384848807876,-462.504467942754));
#31782=CARTESIAN_POINT('Ctrl Pts',(57.8729592854362,15.3392709400169,-462.499999999989));
#31783=CARTESIAN_POINT('Ctrl Pts',(71.5424551136857,19.4736998850754,-438.99999999999));
#31784=CARTESIAN_POINT('',(64.5871672591961,17.3700458363661,-450.95723971308));
#31785=CARTESIAN_POINT('',(65.2503505017821,17.5706789545087,-449.81715836622));
#31786=CARTESIAN_POINT('',(64.5871632769409,17.3700261100896,-450.957233845127));
#31787=CARTESIAN_POINT('Ctrl Pts',(65.2503505017068,17.5706789550751,-449.817158366273));
#31788=CARTESIAN_POINT('Ctrl Pts',(65.1399402715371,17.5378213168938,-450.007344522965));
#31789=CARTESIAN_POINT('Ctrl Pts',(65.0294703630796,17.5046773948113,-450.197443704583));
#31790=CARTESIAN_POINT('Ctrl Pts',(64.808407856047,17.4378034358709,-450.577473377674));
#31791=CARTESIAN_POINT('Ctrl Pts',(64.6978178839098,17.4040741936062,-450.767399354003));
#31792=CARTESIAN_POINT('Ctrl Pts',(64.58716725919,17.3700458364086,-450.957239713085));
#31793=CARTESIAN_POINT('Ctrl Pts',(58.315252633502,-29.4505673778293,-462.499999999984));
#31794=CARTESIAN_POINT('Ctrl Pts',(70.9913620171487,-32.1584685094449,-439.002497203513));
#31795=CARTESIAN_POINT('Ctrl Pts',(57.2363227370075,-31.9735001917283,-462.499999999984));
#31796=CARTESIAN_POINT('Ctrl Pts',(70.1312984392538,-35.2664311746943,-438.996844362179));
#31797=CARTESIAN_POINT('Ctrl Pts',(57.0028527821642,-34.8311127366432,-462.499999999984));
#31798=CARTESIAN_POINT('Ctrl Pts',(70.2493774551285,-38.6061780586552,-439.002389441109));
#31799=CARTESIAN_POINT('Ctrl Pts',(57.872959299689,-37.6772709866423,-462.499999999983));
#31800=CARTESIAN_POINT('Ctrl Pts',(71.5424551348726,-41.8116999372577,-438.999999999983));
#31801=CARTESIAN_POINT('',(64.5798198703728,-39.7058474679734,-450.969887422476));
#31802=CARTESIAN_POINT('',(65.2610173681319,-39.9118525359211,-449.798783660325));
#31803=CARTESIAN_POINT('',(64.5798106827944,-39.7058023136291,-450.96987413409));
#31804=CARTESIAN_POINT('',(57.7295804999108,-37.1684431732989,-462.499999999983));
#31805=CARTESIAN_POINT('Ctrl Pts',(57.729580499911,-37.1684431732993,-462.499999999983));
#31806=CARTESIAN_POINT('Ctrl Pts',(58.8199723157923,-37.6567760006761,-460.693530021075));
#31807=CARTESIAN_POINT('Ctrl Pts',(59.923205364492,-38.1000146374347,-458.856471844879));
#31808=CARTESIAN_POINT('Ctrl Pts',(62.2046437952623,-38.9433259685703,-455.022540409383));
#31809=CARTESIAN_POINT('Ctrl Pts',(63.3997482388661,-39.3427460598765,-452.994373238536));
#31810=CARTESIAN_POINT('Ctrl Pts',(64.5798065713121,-39.705781792052,-450.969867971454));
#31811=CARTESIAN_POINT('',(58.315252633502,-29.4505673778293,-462.499999999984));
#31812=CARTESIAN_POINT('Ctrl Pts',(58.3152526334998,-29.4505673778284,-462.499999999988));
#31813=CARTESIAN_POINT('Ctrl Pts',(57.7976276531132,-30.6609639499824,-462.499999999988));
#31814=CARTESIAN_POINT('Ctrl Pts',(57.4826884205137,-31.9483301287851,-462.499999999987));
#31815=CARTESIAN_POINT('Ctrl Pts',(57.2834655596958,-34.5736510331327,-462.499999999987));
#31816=CARTESIAN_POINT('Ctrl Pts',(57.4005339681898,-35.8938034717833,-462.499999999988));
#31817=CARTESIAN_POINT('Ctrl Pts',(57.7295829994487,-37.1684528558765,-462.499999999988));
#31818=CARTESIAN_POINT('',(58.315252633502,-29.4505673778293,-462.499999999984));
#31819=CARTESIAN_POINT('Ctrl Pts',(70.459364073535,-36.7925280866649,-438.999999999984));
#31820=CARTESIAN_POINT('Ctrl Pts',(70.4453273089361,-36.4542715080457,-438.999999999984));
#31821=CARTESIAN_POINT('Ctrl Pts',(70.4427173721536,-36.1156409498122,-438.999999999982));
#31822=CARTESIAN_POINT('Ctrl Pts',(70.4603981657122,-35.4387755921454,-438.999999999983));
#31823=CARTESIAN_POINT('Ctrl Pts',(70.4806827099488,-35.1007537261475,-438.999999999984));
#31824=CARTESIAN_POINT('Ctrl Pts',(70.5123942581111,-34.7636934497019,-438.999999999984));
#31825=CARTESIAN_POINT('Ctrl Pts',(65.2610173681319,-39.9118525359211,-449.798783660325));
#31826=CARTESIAN_POINT('Ctrl Pts',(66.0967783128156,-40.1604407556788,-448.359058582003));
#31827=CARTESIAN_POINT('Ctrl Pts',(66.9275802964328,-40.392196036837,-446.916923734249));
#31828=CARTESIAN_POINT('Ctrl Pts',(68.5997382095796,-40.8322295918434,-443.993321242625));
#31829=CARTESIAN_POINT('Ctrl Pts',(69.4492098945576,-41.0416415242989,-442.496899945137));
#31830=CARTESIAN_POINT('Ctrl Pts',(70.2929704405245,-41.2369817291983,-441.000070382422));
#31831=CARTESIAN_POINT('Ctrl Pts',(69.7946169307026,-54.38201903755,-440.978989030848));
#31832=CARTESIAN_POINT('Ctrl Pts',(69.7816652336298,-54.3708182762895,-441.000100325607));
#31833=CARTESIAN_POINT('Ctrl Pts',(69.5560658976611,-59.4654621740419,-440.978600448059));
#31834=CARTESIAN_POINT('Ctrl Pts',(69.5425906598038,-59.4517471897933,-440.999999999981));
#31835=CARTESIAN_POINT('Ctrl Pts',(67.6456657063917,-64.182133843286,-440.978600448058));
#31836=CARTESIAN_POINT('Ctrl Pts',(67.6327997693368,-64.1661639590497,-440.99999999998));
#31837=CARTESIAN_POINT('Ctrl Pts',(64.2817759434034,-67.9940247783317,-440.978967867946));
#31838=CARTESIAN_POINT('Ctrl Pts',(64.2705054959406,-67.9765004273711,-441.000078147038));
#31839=CARTESIAN_POINT('',(64.2705054959405,-67.9765004273713,-441.000078147038));
#31840=CARTESIAN_POINT('Origin',(47.8350487510253,-53.3691022099654,-441.001185826503));
#31841=CARTESIAN_POINT('Ctrl Pts',(64.2705054959406,-67.9765004273711,-441.000078147038));
#31842=CARTESIAN_POINT('Ctrl Pts',(65.3713757282322,-66.7310443578283,-440.998581998987));
#31843=CARTESIAN_POINT('Ctrl Pts',(66.3280443259402,-65.3652099283856,-440.997113886392));
#31844=CARTESIAN_POINT('Ctrl Pts',(67.7249250139629,-62.7970659610114,-440.99537830064));
#31845=CARTESIAN_POINT('Ctrl Pts',(68.2314861563532,-61.6395247500074,-440.994908924246));
#31846=CARTESIAN_POINT('Ctrl Pts',(68.9087860162404,-59.6416335258256,-440.994945640725));
#31847=CARTESIAN_POINT('Ctrl Pts',(69.1346111078826,-58.8231493981561,-440.995183026277));
#31848=CARTESIAN_POINT('Ctrl Pts',(69.438858496689,-57.4066076677694,-440.996093834534));
#31849=CARTESIAN_POINT('Ctrl Pts',(69.5409437946101,-56.8146091059414,-440.996619383099));
#31850=CARTESIAN_POINT('Ctrl Pts',(69.6989501274562,-55.6056200152367,-440.998047800919));
#31851=CARTESIAN_POINT('Ctrl Pts',(69.7532997046084,-54.9889520016567,-440.998960866044));
#31852=CARTESIAN_POINT('Ctrl Pts',(69.7816652336299,-54.3708182762896,-441.000100325607));
#31853=CARTESIAN_POINT('Ctrl Pts',(69.7816652336298,-54.3708182762895,-441.000100325607));
#31854=CARTESIAN_POINT('Ctrl Pts',(56.5915605594697,-42.9638796623104,-462.499999999983));
#31855=CARTESIAN_POINT('Ctrl Pts',(69.5425906598038,-59.4517471897933,-440.999999999981));
#31856=CARTESIAN_POINT('Ctrl Pts',(56.0041009291271,-45.6723857139866,-462.499999999983));
#31857=CARTESIAN_POINT('Ctrl Pts',(67.6327997693368,-64.1661639590497,-440.99999999998));
#31858=CARTESIAN_POINT('Ctrl Pts',(54.7064708585618,-48.1213181444985,-462.499999999982));
#31859=CARTESIAN_POINT('Ctrl Pts',(64.2705054959406,-67.9765004273711,-441.000078147038));
#31860=CARTESIAN_POINT('Ctrl Pts',(52.7925979348378,-50.1295710081989,-462.498943458986));
#31861=CARTESIAN_POINT('',(56.5915605594697,-42.9638796623104,-462.499999999983));
#31862=CARTESIAN_POINT('',(69.7816652336299,-54.3708182762896,-441.000100325607));
#31863=CARTESIAN_POINT('',(56.5529890060961,-55.9765804635348,-455.455487085874));
#31864=CARTESIAN_POINT('',(64.2705054959405,-67.9765004273713,-441.000078147038));
#31865=CARTESIAN_POINT('',(53.029696289532,-49.8742761699988,-462.499535472179));
#31866=CARTESIAN_POINT('Ctrl Pts',(56.5529890060963,-55.9765804635346,-455.455487085874));
#31867=CARTESIAN_POINT('Ctrl Pts',(55.9381283183532,-54.9116105127872,-456.684378657559));
#31868=CARTESIAN_POINT('Ctrl Pts',(55.3027200270559,-53.8110510686363,-457.954475902198));
#31869=CARTESIAN_POINT('Ctrl Pts',(54.1403899944375,-51.7978363969789,-460.278308627195));
#31870=CARTESIAN_POINT('Ctrl Pts',(53.5778030008828,-50.8234071405388,-461.40328936809));
#31871=CARTESIAN_POINT('Ctrl Pts',(53.0300054239308,-49.8745939049953,-462.499070944372));
#31872=CARTESIAN_POINT('Ctrl Pts',(56.5915605594697,-42.9638796623104,-462.499999999983));
#31873=CARTESIAN_POINT('Ctrl Pts',(56.537631898305,-43.2125199051099,-462.499999999983));
#31874=CARTESIAN_POINT('Ctrl Pts',(56.4771841693873,-43.4606593871229,-462.500000001674));
#31875=CARTESIAN_POINT('Ctrl Pts',(56.4102105416286,-43.7077927013583,-462.499999113015));
#31876=CARTESIAN_POINT('Ctrl Pts',(56.3434676095377,-43.9540747464168,-462.499998227417));
#31877=CARTESIAN_POINT('Ctrl Pts',(56.2702436069996,-44.1993571047456,-462.499996456823));
#31878=CARTESIAN_POINT('Ctrl Pts',(56.1905834176614,-44.4431360043272,-462.49999290506));
#31879=CARTESIAN_POINT('Ctrl Pts',(56.1089402448685,-44.6929832992829,-462.499989264884));
#31880=CARTESIAN_POINT('Ctrl Pts',(56.0205362191533,-44.9412508502421,-462.499983752903));
#31881=CARTESIAN_POINT('Ctrl Pts',(55.9254766389649,-45.1873997239285,-462.499975402613));
#31882=CARTESIAN_POINT('Ctrl Pts',(55.833195263603,-45.4263546673707,-462.499967296368));
#31883=CARTESIAN_POINT('Ctrl Pts',(55.7346419953777,-45.6633125555955,-462.499956514529));
#31884=CARTESIAN_POINT('Ctrl Pts',(55.6299648435093,-45.8977902129081,-462.499942183297));
#31885=CARTESIAN_POINT('Ctrl Pts',(55.5253792494255,-46.1320627800511,-462.4999278646));
#31886=CARTESIAN_POINT('Ctrl Pts',(55.4146806098435,-46.3638590294524,-462.49991000195));
#31887=CARTESIAN_POINT('Ctrl Pts',(55.2980659547443,-46.5927132907045,-462.499887745806));
#31888=CARTESIAN_POINT('Ctrl Pts',(55.1814748250644,-46.8215213837246,-462.499865494152));
#31889=CARTESIAN_POINT('Ctrl Pts',(55.0589702553333,-47.0473882738389,-462.499838850043));
#31890=CARTESIAN_POINT('Ctrl Pts',(54.9307961809409,-47.2698710119221,-462.499806997694));
#31891=CARTESIAN_POINT('Ctrl Pts',(54.8025614231947,-47.4924590833091,-462.499775130265));
#31892=CARTESIAN_POINT('Ctrl Pts',(54.6686520347203,-47.7116594263157,-462.499738048975));
#31893=CARTESIAN_POINT('Ctrl Pts',(54.529356130181,-47.9270567374448,-462.499694980864));
#31894=CARTESIAN_POINT('Ctrl Pts',(54.389759265441,-48.1429194320911,-462.499651819701));
#31895=CARTESIAN_POINT('Ctrl Pts',(54.2447528711453,-48.3549623037771,-462.499602645179));
#31896=CARTESIAN_POINT('Ctrl Pts',(54.0946669651107,-48.5628011065844,-462.499546733495));
#31897=CARTESIAN_POINT('Ctrl Pts',(53.9443335508868,-48.7709826584683,-462.499490729606));
#31898=CARTESIAN_POINT('Ctrl Pts',(53.7889041971722,-48.9749459760321,-462.49942796576));
#31899=CARTESIAN_POINT('Ctrl Pts',(53.6287459504915,-49.1743434635936,-462.499357777847));
#31900=CARTESIAN_POINT('Ctrl Pts',(53.4680465723631,-49.3744146613969,-462.499287352789));
#31901=CARTESIAN_POINT('Ctrl Pts',(53.3025866634557,-49.5698888785735,-462.499209452928));
#31902=CARTESIAN_POINT('Ctrl Pts',(53.1327672630609,-49.7604578043835,-462.499123478914));
#31903=CARTESIAN_POINT('Ctrl Pts',(53.0986997159057,-49.7986879232701,-462.499106231627));
#31904=CARTESIAN_POINT('Ctrl Pts',(53.0644568094535,-49.8367207747998,-462.499088659643));
#31905=CARTESIAN_POINT('Ctrl Pts',(53.0300419063689,-49.8745540888141,-462.499070758491));
#31906=CARTESIAN_POINT('Ctrl Pts',(56.8171268781939,-75.4544783554495,-440.981517358892));
#31907=CARTESIAN_POINT('Ctrl Pts',(56.8017229870639,-75.4445663251619,-441.000077552423));
#31908=CARTESIAN_POINT('Ctrl Pts',(53.0022604651873,-78.8200388563469,-440.981185782947));
#31909=CARTESIAN_POINT('Ctrl Pts',(52.9882277636123,-78.8087212293983,-440.999999999979));
#31910=CARTESIAN_POINT('Ctrl Pts',(48.2867035759484,-80.7296085197381,-440.981185782946));
#31911=CARTESIAN_POINT('Ctrl Pts',(48.274652617608,-80.7177558649672,-440.999999999978));
#31912=CARTESIAN_POINT('Ctrl Pts',(43.2073677667846,-80.9657191524129,-440.981499301018));
#31913=CARTESIAN_POINT('Ctrl Pts',(43.197523751011,-80.9543288413526,-441.000060412176));
#31914=CARTESIAN_POINT('',(56.8017229870589,-75.4445663251663,-441.000077552423));
#31915=CARTESIAN_POINT('',(43.1975237510109,-80.9543288413527,-441.000060412177));
#31916=CARTESIAN_POINT('Origin',(42.2233532178455,-58.9519567778136,-441.000918028327));
#31917=CARTESIAN_POINT('Ctrl Pts',(43.1975237510113,-80.9543288413526,-441.000060412176));
#31918=CARTESIAN_POINT('Ctrl Pts',(44.4031402145552,-80.8989945191125,-440.998726536663));
#31919=CARTESIAN_POINT('Ctrl Pts',(45.6021895814689,-80.7448684887729,-440.997737499632));
#31920=CARTESIAN_POINT('Ctrl Pts',(47.9449883857747,-80.245975858692,-440.996451146542));
#31921=CARTESIAN_POINT('Ctrl Pts',(49.0854799958832,-79.9049726728867,-440.996144855277));
#31922=CARTESIAN_POINT('Ctrl Pts',(51.4454681110207,-78.9862019845966,-440.996145395842));
#31923=CARTESIAN_POINT('Ctrl Pts',(52.6508252985512,-78.3851936817408,-440.996537734672));
#31924=CARTESIAN_POINT('Ctrl Pts',(54.858065396025,-77.0203018770163,-440.997937064421));
#31925=CARTESIAN_POINT('Ctrl Pts',(55.8642654113312,-76.2730348674113,-440.998896997706));
#31926=CARTESIAN_POINT('Ctrl Pts',(56.8017229870589,-75.4445663251663,-441.000077552423));
#31927=CARTESIAN_POINT('Ctrl Pts',(56.8017229870639,-75.4445663251619,-441.000077552423));
#31928=CARTESIAN_POINT('Ctrl Pts',(38.9588941886819,-63.9631388095498,-462.498954222077));
#31929=CARTESIAN_POINT('Ctrl Pts',(52.9882277636123,-78.8087212293983,-440.999999999979));
#31930=CARTESIAN_POINT('Ctrl Pts',(36.9523181444951,-65.8754708585682,-462.499999999979));
#31931=CARTESIAN_POINT('Ctrl Pts',(48.274652617608,-80.7177558649672,-440.999999999978));
#31932=CARTESIAN_POINT('Ctrl Pts',(34.5033857139835,-67.173100929134,-462.499999999979));
#31933=CARTESIAN_POINT('Ctrl Pts',(43.197523751011,-80.9543288413526,-441.000060412176));
#31934=CARTESIAN_POINT('Ctrl Pts',(31.7948796623075,-67.7605605594772,-462.499999999979));
#31935=CARTESIAN_POINT('',(44.7374479017836,-67.6814979527098,-455.536357931381));
#31936=CARTESIAN_POINT('',(56.8017229870589,-75.4445663251663,-441.000077552423));
#31937=CARTESIAN_POINT('',(31.7948796623075,-67.7605605594772,-462.499999999979));
#31938=CARTESIAN_POINT('',(43.1975237510109,-80.9543288413527,-441.000060412177));
#31939=CARTESIAN_POINT('',(38.7052882157426,-64.1987044759212,-462.499539856792));
#31940=CARTESIAN_POINT('Ctrl Pts',(38.7055635736167,-64.1990467954908,-462.499079528891));
#31941=CARTESIAN_POINT('Ctrl Pts',(38.5172275971445,-64.3704105530215,-462.499167854858));
#31942=CARTESIAN_POINT('Ctrl Pts',(38.3239197960279,-64.5375163457007,-462.499248085453));
#31943=CARTESIAN_POINT('Ctrl Pts',(38.1259398426536,-64.699957188765,-462.49932079767));
#31944=CARTESIAN_POINT('Ctrl Pts',(37.9285425865703,-64.8619199337311,-462.49939329588));
#31945=CARTESIAN_POINT('Ctrl Pts',(37.726500868484,-65.0192447705182,-462.499458320352));
#31946=CARTESIAN_POINT('Ctrl Pts',(37.5201548987088,-65.1715569484135,-462.49951651441));
#31947=CARTESIAN_POINT('Ctrl Pts',(37.3080980013927,-65.3280845893609,-462.499576319074));
#31948=CARTESIAN_POINT('Ctrl Pts',(37.0914954019602,-65.4793177024024,-462.499628910257));
#31949=CARTESIAN_POINT('Ctrl Pts',(36.8707598320672,-65.6248872824809,-462.499675056921));
#31950=CARTESIAN_POINT('Ctrl Pts',(36.6567884437342,-65.7659960542278,-462.499719789474));
#31951=CARTESIAN_POINT('Ctrl Pts',(36.4389340209405,-65.9017829622837,-462.499758467341));
#31952=CARTESIAN_POINT('Ctrl Pts',(36.2176075522289,-66.0319513181425,-462.499791846736));
#31953=CARTESIAN_POINT('Ctrl Pts',(35.9963765196386,-66.1620635453191,-462.499825211738));
#31954=CARTESIAN_POINT('Ctrl Pts',(35.7716767996782,-66.2865618098307,-462.499853283506));
#31955=CARTESIAN_POINT('Ctrl Pts',(35.5439481503633,-66.4051928613635,-462.499876862572));
#31956=CARTESIAN_POINT('Ctrl Pts',(35.316169349663,-66.5238500383382,-462.499900446831));
#31957=CARTESIAN_POINT('Ctrl Pts',(35.0853606833263,-66.6366372165729,-462.49991953713));
#31958=CARTESIAN_POINT('Ctrl Pts',(34.8519857935553,-66.7433474955649,-462.499934969413));
#31959=CARTESIAN_POINT('Ctrl Pts',(34.6184080394107,-66.8501505339532,-462.499950415112));
#31960=CARTESIAN_POINT('Ctrl Pts',(34.3822600211211,-66.9508659603753,-462.499962197189));
#31961=CARTESIAN_POINT('Ctrl Pts',(34.1440240563708,-67.0453355257903,-462.499971177619));
#31962=CARTESIAN_POINT('Ctrl Pts',(33.9051482369425,-67.1400588177718,-462.499980182168));
#31963=CARTESIAN_POINT('Ctrl Pts',(33.664173678481,-67.2285025608647,-462.499986370777));
#31964=CARTESIAN_POINT('Ctrl Pts',(33.4215976713632,-67.3105584616105,-462.499990624821));
#31965=CARTESIAN_POINT('Ctrl Pts',(33.1785544871469,-67.3927723938042,-462.499994887057));
#31966=CARTESIAN_POINT('Ctrl Pts',(32.9339041272313,-67.4685738375367,-462.49999720805));
#31967=CARTESIAN_POINT('Ctrl Pts',(32.6881511913545,-67.5379060565884,-462.499998475006));
#31968=CARTESIAN_POINT('Ctrl Pts',(32.4414818006612,-67.6074968273676,-462.499999746687));
#31969=CARTESIAN_POINT('Ctrl Pts',(32.1937020411489,-67.6705700690391,-462.499999957227));
#31970=CARTESIAN_POINT('Ctrl Pts',(31.9453199033596,-67.7271208240112,-462.499999992803));
#31971=CARTESIAN_POINT('Ctrl Pts',(31.8951963275913,-67.7385327801076,-462.499999999982));
#31972=CARTESIAN_POINT('Ctrl Pts',(31.8450482010303,-67.7496792874214,-462.499999999979));
#31973=CARTESIAN_POINT('Ctrl Pts',(31.7948796623075,-67.7605605594772,-462.499999999979));
#31974=CARTESIAN_POINT('Ctrl Pts',(38.7056029900764,-64.1990106692133,-462.4990797136));
#31975=CARTESIAN_POINT('Ctrl Pts',(39.6432579745448,-64.7403660269029,-461.416170705934));
#31976=CARTESIAN_POINT('Ctrl Pts',(40.6056781462348,-65.296019572104,-460.305037237873));
#31977=CARTESIAN_POINT('Ctrl Pts',(42.5961675836127,-66.4452291845927,-458.007400411776));
#31978=CARTESIAN_POINT('Ctrl Pts',(43.6839808596153,-67.0732784723181,-456.751993534114));
#31979=CARTESIAN_POINT('Ctrl Pts',(44.7374479017911,-67.6814979527005,-455.536357931383));
#31980=CARTESIAN_POINT('Ctrl Pts',(-43.2047136373585,-80.966056949464,-440.981137741313));
#31981=CARTESIAN_POINT('Ctrl Pts',(-43.1946805031653,-80.9544448157854,
-441.000060157993));
#31982=CARTESIAN_POINT('Ctrl Pts',(-48.2869381564542,-80.7298392401449,
-440.980819550762));
#31983=CARTESIAN_POINT('Ctrl Pts',(-48.2746526175946,-80.7177558649757,
-440.999999999976));
#31984=CARTESIAN_POINT('Ctrl Pts',(-53.0025336217422,-78.8202591620554,
-440.980819550762));
#31985=CARTESIAN_POINT('Ctrl Pts',(-52.9882277635993,-78.8087212294075,
-440.999999999977));
#31986=CARTESIAN_POINT('Ctrl Pts',(-56.8142200441329,-75.4551560531967,
-440.98112498298));
#31987=CARTESIAN_POINT('Ctrl Pts',(-56.7985201760894,-75.4450502563038,
-441.000046863259));
#31988=CARTESIAN_POINT('',(-43.1946805031654,-80.9544448157855,-441.000060157993));
#31989=CARTESIAN_POINT('',(-56.7985201761028,-75.4450502562919,-441.000046863259));
#31990=CARTESIAN_POINT('Origin',(-42.1888478026556,-58.9666575781096,-441.000711744184));
#31991=CARTESIAN_POINT('Ctrl Pts',(-56.7985201760894,-75.4450502563038,
-441.000046863259));
#31992=CARTESIAN_POINT('Ctrl Pts',(-56.4263535406146,-75.7739272521541,
-440.99977882747));
#31993=CARTESIAN_POINT('Ctrl Pts',(-56.0431930051001,-76.090149626701,-440.999512160104));
#31994=CARTESIAN_POINT('Ctrl Pts',(-53.724908457157,-77.8754202087466,-440.997991790387));
#31995=CARTESIAN_POINT('Ctrl Pts',(-51.5685554398738,-79.0297799655311,
-440.996935620165));
#31996=CARTESIAN_POINT('Ctrl Pts',(-48.2083577710306,-80.1686711508664,
-440.996972642525));
#31997=CARTESIAN_POINT('Ctrl Pts',(-47.123200326989,-80.4466850673039,-440.997215533442));
#31998=CARTESIAN_POINT('Ctrl Pts',(-45.087048397782,-80.8063142609533,-440.998282797664));
#31999=CARTESIAN_POINT('Ctrl Pts',(-44.1427605555334,-80.9109332077313,
-440.999012122082));
#32000=CARTESIAN_POINT('Ctrl Pts',(-43.1946805031653,-80.9544448157854,
-441.000060157993));
#32001=CARTESIAN_POINT('Ctrl Pts',(-64.2743506444738,-67.9925839239085,
-440.983888214158));
#32002=CARTESIAN_POINT('Ctrl Pts',(-64.2657293397397,-67.9791674266158,
-441.000046512357));
#32003=CARTESIAN_POINT('Ctrl Pts',(-67.6426474509325,-64.1783874243697,
-440.983620627614));
#32004=CARTESIAN_POINT('Ctrl Pts',(-67.6327997693264,-64.1661639590615,
-440.999999999978));
#32005=CARTESIAN_POINT('Ctrl Pts',(-69.552904704657,-59.4622447382962,-440.983620627615));
#32006=CARTESIAN_POINT('Ctrl Pts',(-69.5425906597941,-59.4517471898053,
-440.999999999979));
#32007=CARTESIAN_POINT('Ctrl Pts',(-69.7876243621201,-54.3811153516783,
-440.983874019661));
#32008=CARTESIAN_POINT('Ctrl Pts',(-69.7777140088065,-54.3725409130246,
-441.000032808645));
#32009=CARTESIAN_POINT('',(-64.2657293397398,-67.9791674266157,-441.000046512357));
#32010=CARTESIAN_POINT('',(-69.7777140088065,-54.3725409130246,-441.000032808645));
#32011=CARTESIAN_POINT('Origin',(-47.7498816680565,-53.384540451435,-441.000527747256));
#32012=CARTESIAN_POINT('Ctrl Pts',(-69.7777140088065,-54.3725409130246,
-441.000032808645));
#32013=CARTESIAN_POINT('Ctrl Pts',(-69.7165990727465,-55.7037291462961,
-440.999228486668));
#32014=CARTESIAN_POINT('Ctrl Pts',(-69.535056842701,-57.026651696731,-440.99862757642));
#32015=CARTESIAN_POINT('Ctrl Pts',(-68.9483190906072,-59.5682977466865,
-440.997891639565));
#32016=CARTESIAN_POINT('Ctrl Pts',(-68.5540700559461,-60.7842796997571,
-440.997738224173));
#32017=CARTESIAN_POINT('Ctrl Pts',(-67.6191319824325,-62.9944922976845,
-440.997830589012));
#32018=CARTESIAN_POINT('Ctrl Pts',(-67.1028440820214,-63.9946589547973,
-440.998030525737));
#32019=CARTESIAN_POINT('Ctrl Pts',(-65.8514110837686,-66.0227249818099,
-440.99876113321));
#32020=CARTESIAN_POINT('Ctrl Pts',(-65.0996976290768,-67.0357638306388,
-440.999327438968));
#32021=CARTESIAN_POINT('Ctrl Pts',(-64.2657293397398,-67.9791674266157,
-441.000046512357));
#32022=CARTESIAN_POINT('Origin',(45.9999999999903,112.830999999998,-401.5));
#32023=CARTESIAN_POINT('',(49.9999999999903,112.830999999998,-399.1905989232));
#32024=CARTESIAN_POINT('',(45.9999999999903,112.830999999998,-396.8811978465));
#32025=CARTESIAN_POINT('',(47.9999999999903,112.830999999998,-398.03589838485));
#32026=CARTESIAN_POINT('',(49.9999999999903,112.830999999998,-403.8094010768));
#32027=CARTESIAN_POINT('',(49.9999999999903,112.830999999998,-401.5));
#32028=CARTESIAN_POINT('',(45.9999999999903,112.830999999997,-406.118802153499));
#32029=CARTESIAN_POINT('',(47.9999999999903,112.830999999997,-404.96410161515));
#32030=CARTESIAN_POINT('',(41.9999999999903,112.830999999997,-403.8094010768));
#32031=CARTESIAN_POINT('',(43.9999999999903,112.830999999997,-404.96410161515));
#32032=CARTESIAN_POINT('',(41.9999999999903,112.830999999998,-399.1905989232));
#32033=CARTESIAN_POINT('',(41.9999999999903,112.830999999997,-401.5));
#32034=CARTESIAN_POINT('',(43.9999999999903,112.830999999998,-398.03589838485));
#32035=CARTESIAN_POINT('Origin',(-49.0000000000097,112.830999999989,-401.5));
#32036=CARTESIAN_POINT('',(-45.0000000000097,112.83099999999,-399.1905989232));
#32037=CARTESIAN_POINT('',(-49.0000000000097,112.83099999999,-396.8811978465));
#32038=CARTESIAN_POINT('',(-47.0000000000097,112.83099999999,-398.03589838485));
#32039=CARTESIAN_POINT('',(-45.0000000000097,112.830999999989,-403.8094010768));
#32040=CARTESIAN_POINT('',(-45.0000000000097,112.83099999999,-401.5));
#32041=CARTESIAN_POINT('',(-49.0000000000097,112.830999999989,-406.118802153499));
#32042=CARTESIAN_POINT('',(-47.0000000000097,112.830999999989,-404.96410161515));
#32043=CARTESIAN_POINT('',(-53.0000000000097,112.830999999989,-403.8094010768));
#32044=CARTESIAN_POINT('',(-51.0000000000097,112.830999999989,-404.96410161515));
#32045=CARTESIAN_POINT('',(-53.0000000000097,112.830999999989,-399.1905989232));
#32046=CARTESIAN_POINT('',(-53.0000000000097,112.830999999989,-401.5));
#32047=CARTESIAN_POINT('',(-51.0000000000097,112.83099999999,-398.03589838485));
#32048=CARTESIAN_POINT('Origin',(45.9999999999903,112.831000000008,-309.5));
#32049=CARTESIAN_POINT('',(49.9999999999903,112.831000000009,-307.1905989232));
#32050=CARTESIAN_POINT('',(45.9999999999903,112.831000000009,-304.881197846499));
#32051=CARTESIAN_POINT('',(47.9999999999903,112.831000000009,-306.035898384849));
#32052=CARTESIAN_POINT('',(49.9999999999903,112.831000000008,-311.809401076799));
#32053=CARTESIAN_POINT('',(49.9999999999903,112.831000000009,-309.5));
#32054=CARTESIAN_POINT('',(45.9999999999903,112.831000000008,-314.118802153499));
#32055=CARTESIAN_POINT('',(47.9999999999903,112.831000000008,-312.96410161515));
#32056=CARTESIAN_POINT('',(41.9999999999903,112.831000000008,-311.809401076799));
#32057=CARTESIAN_POINT('',(43.9999999999903,112.831000000008,-312.96410161515));
#32058=CARTESIAN_POINT('',(41.9999999999903,112.831000000008,-307.1905989232));
#32059=CARTESIAN_POINT('',(41.9999999999903,112.831000000008,-309.5));
#32060=CARTESIAN_POINT('',(43.9999999999903,112.831000000008,-306.035898384849));
#32061=CARTESIAN_POINT('Origin',(-49.0000000000097,112.831,-309.5));
#32062=CARTESIAN_POINT('',(-45.0000000000097,112.831,-307.1905989232));
#32063=CARTESIAN_POINT('',(-49.0000000000097,112.831,-304.881197846499));
#32064=CARTESIAN_POINT('',(-47.0000000000097,112.831,-306.035898384849));
#32065=CARTESIAN_POINT('',(-45.0000000000097,112.831,-311.809401076799));
#32066=CARTESIAN_POINT('',(-45.0000000000097,112.831,-309.5));
#32067=CARTESIAN_POINT('',(-49.0000000000097,112.831,-314.118802153499));
#32068=CARTESIAN_POINT('',(-47.0000000000097,112.831,-312.96410161515));
#32069=CARTESIAN_POINT('',(-53.0000000000097,112.831,-311.809401076799));
#32070=CARTESIAN_POINT('',(-51.0000000000097,112.831,-312.96410161515));
#32071=CARTESIAN_POINT('',(-53.0000000000097,112.831,-307.1905989232));
#32072=CARTESIAN_POINT('',(-53.0000000000097,112.831,-309.5));
#32073=CARTESIAN_POINT('',(-51.0000000000097,112.831,-306.035898384849));
#32074=CARTESIAN_POINT('Origin',(26.6129405624652,-47.4885629631521,-461.499999999981));
#32075=CARTESIAN_POINT('',(52.1061868616782,-40.3862650211815,-461.499999999983));
#32076=CARTESIAN_POINT('',(47.6332714621302,-49.0956490614551,-461.499999999982));
#32077=CARTESIAN_POINT('Origin',(36.3195629631445,-37.7819405624712,-461.500000000005));
#32078=CARTESIAN_POINT('',(37.9266490614509,-58.802271462136,-461.49999999998));
#32079=CARTESIAN_POINT('',(47.6332714621302,-49.0956490614551,-461.499999999982));
#32080=CARTESIAN_POINT('',(29.2172650211785,-63.2751868616856,-461.499999999979));
#32081=CARTESIAN_POINT('Origin',(26.6129405624651,-47.488562963152,-461.499999999982));
#32082=CARTESIAN_POINT('',(-29.2172650211685,-63.2751868616907,-461.499999999979));
#32083=CARTESIAN_POINT('Origin',(-1.19904086659517E-11,113.830999999992,
-461.500000000043));
#32084=CARTESIAN_POINT('',(-37.9266490614418,-58.8022714621425,-461.49999999998));
#32085=CARTESIAN_POINT('Origin',(-26.612940562458,-47.4885629631569,-461.499999999995));
#32086=CARTESIAN_POINT('',(-47.6332714621227,-49.0956490614631,-461.49999999998));
#32087=CARTESIAN_POINT('',(-37.9266490614418,-58.8022714621425,-461.49999999998));
#32088=CARTESIAN_POINT('Origin',(-36.3195629631389,-37.7819405624775,-461.499999999979));
#32089=CARTESIAN_POINT('',(-47.6332714621292,26.7576490614296,-461.499999999989));
#32090=CARTESIAN_POINT('Origin',(-36.3195629631435,15.4439405624457,-461.49999999999));
#32091=CARTESIAN_POINT('',(-37.9266490614499,36.4642714621104,-461.49999999999));
#32092=CARTESIAN_POINT('',(-47.6332714621292,26.7576490614295,-461.499999999989));
#32093=CARTESIAN_POINT('',(-29.2172650211774,40.93718686166,-461.499999999991));
#32094=CARTESIAN_POINT('Origin',(-26.6129405624642,25.1505629631267,-461.499999999994));
#32095=CARTESIAN_POINT('',(29.2172650211694,40.9371868616653,-461.499999999991));
#32096=CARTESIAN_POINT('Origin',(1.30295774170008E-11,-136.169000000019,
-461.500000000151));
#32097=CARTESIAN_POINT('',(37.9266490614429,36.4642714621169,-461.499999999991));
#32098=CARTESIAN_POINT('Origin',(26.6129405624589,25.1505629631313,-461.49999999999));
#32099=CARTESIAN_POINT('',(47.6332714621237,26.7576490614377,-461.49999999999));
#32100=CARTESIAN_POINT('',(37.9266490614429,36.4642714621169,-461.499999999991));
#32101=CARTESIAN_POINT('',(52.1061868616731,18.0482650211652,-461.499999999989));
#32102=CARTESIAN_POINT('Origin',(36.31956296314,15.4439405624519,-461.499999999992));
#32103=CARTESIAN_POINT('Origin',(-125.,-11.1690000000242,-461.500000000023));
#32104=CARTESIAN_POINT('Origin',(52.4999999999926,86.8310000000061,-333.499999999996));
#32105=CARTESIAN_POINT('',(52.4999999999928,83.9442486541067,-328.499999999996));
#32106=CARTESIAN_POINT('',(52.4999999999931,81.0574973081061,-333.499999999996));
#32107=CARTESIAN_POINT('',(52.4999999999929,82.5008729811064,-330.999999999996));
#32108=CARTESIAN_POINT('',(52.4999999999928,83.9442486541055,-338.499999999996));
#32109=CARTESIAN_POINT('',(52.4999999999929,82.5008729811058,-335.999999999996));
#32110=CARTESIAN_POINT('',(52.4999999999923,89.7177513459055,-338.5));
#32111=CARTESIAN_POINT('',(52.4999999999927,85.3876243270555,-338.499999999996));
#32112=CARTESIAN_POINT('',(52.499999999992,92.6045026919061,-333.5));
#32113=CARTESIAN_POINT('',(52.4999999999922,91.1611270189058,-336.));
#32114=CARTESIAN_POINT('',(52.4999999999923,89.7177513459067,-328.5));
#32115=CARTESIAN_POINT('',(52.4999999999922,91.1611270189064,-331.));
#32116=CARTESIAN_POINT('',(52.4999999999926,86.8310000000067,-328.499999999996));
#32117=CARTESIAN_POINT('Origin',(52.4999999999926,86.831000000001,-377.5));
#32118=CARTESIAN_POINT('',(52.4999999999928,83.9442486541016,-372.5));
#32119=CARTESIAN_POINT('',(52.4999999999931,81.057497308101,-377.5));
#32120=CARTESIAN_POINT('',(52.4999999999929,82.5008729811013,-375.));
#32121=CARTESIAN_POINT('',(52.4999999999928,83.9442486541005,-382.5));
#32122=CARTESIAN_POINT('',(52.4999999999929,82.5008729811008,-380.));
#32123=CARTESIAN_POINT('',(52.4999999999923,89.7177513459005,-382.5));
#32124=CARTESIAN_POINT('',(52.4999999999927,85.3876243270505,-382.5));
#32125=CARTESIAN_POINT('',(52.499999999992,92.604502691901,-377.5));
#32126=CARTESIAN_POINT('',(52.4999999999922,91.1611270189007,-380.));
#32127=CARTESIAN_POINT('',(52.4999999999923,89.7177513459016,-372.5));
#32128=CARTESIAN_POINT('',(52.4999999999922,91.1611270189013,-375.));
#32129=CARTESIAN_POINT('',(52.4999999999926,86.8310000000016,-372.5));
#32130=CARTESIAN_POINT('Origin',(43.9999999999906,109.330999999997,-404.964101615149));
#32131=CARTESIAN_POINT('',(45.9999999999906,109.330999999997,-406.118802153499));
#32132=CARTESIAN_POINT('',(41.9999999999906,109.330999999997,-403.809401076799));
#32133=CARTESIAN_POINT('',(45.9999999999906,109.330999999997,-406.118802153499));
#32134=CARTESIAN_POINT('',(41.9999999999906,109.330999999997,-403.809401076799));
#32135=CARTESIAN_POINT('',(45.9999999999906,109.330999999997,-406.118802153499));
#32136=CARTESIAN_POINT('Origin',(41.9999999999906,109.330999999997,-401.5));
#32137=CARTESIAN_POINT('',(41.9999999999906,109.330999999998,-399.190598923199));
#32138=CARTESIAN_POINT('',(41.9999999999906,109.330999999997,-402.957368983363));
#32139=CARTESIAN_POINT('',(41.9999999999906,109.330999999998,-399.190598923199));
#32140=CARTESIAN_POINT('Origin',(43.9999999999906,109.330999999998,-398.035898384849));
#32141=CARTESIAN_POINT('',(45.9999999999906,109.330999999998,-396.881197846499));
#32142=CARTESIAN_POINT('',(41.9999999999906,109.330999999998,-399.190598923199));
#32143=CARTESIAN_POINT('',(45.9999999999906,109.330999999998,-396.881197846499));
#32144=CARTESIAN_POINT('Origin',(47.9999999999906,109.330999999998,-398.035898384849));
#32145=CARTESIAN_POINT('',(49.9999999999906,109.330999999998,-399.190598923199));
#32146=CARTESIAN_POINT('',(45.9999999999906,109.330999999998,-396.881197846499));
#32147=CARTESIAN_POINT('',(49.9999999999906,109.330999999998,-399.190598923199));
#32148=CARTESIAN_POINT('Origin',(49.9999999999906,109.330999999998,-401.5));
#32149=CARTESIAN_POINT('',(49.9999999999906,109.330999999998,-403.809401076799));
#32150=CARTESIAN_POINT('',(49.9999999999906,109.330999999998,-402.957368983363));
#32151=CARTESIAN_POINT('',(49.9999999999906,109.330999999998,-403.809401076799));
#32152=CARTESIAN_POINT('Origin',(47.9999999999906,109.330999999997,-404.964101615149));
#32153=CARTESIAN_POINT('',(49.9999999999906,109.330999999998,-403.809401076799));
#32154=CARTESIAN_POINT('Origin',(50.4999999999899,117.331,-393.5));
#32155=CARTESIAN_POINT('',(54.9999999999906,109.331,-393.5));
#32156=CARTESIAN_POINT('',(54.9999999999905,110.331,-393.5));
#32157=CARTESIAN_POINT('',(54.9999999999899,117.331,-393.5));
#32158=CARTESIAN_POINT('',(44.9999999999906,109.330999999998,-393.5));
#32159=CARTESIAN_POINT('',(47.4573689833543,109.330999999999,-393.5));
#32160=CARTESIAN_POINT('',(44.9999999999899,117.330999999998,-393.5));
#32161=CARTESIAN_POINT('',(44.9999999999899,117.330999999998,-393.5));
#32162=CARTESIAN_POINT('',(47.9999999999899,117.330999999999,-393.5));
#32163=CARTESIAN_POINT('',(-1.50000000001011,117.330999999994,-393.5));
#32164=CARTESIAN_POINT('Origin',(47.9999999999905,110.330999999999,-393.5));
#32165=CARTESIAN_POINT('Origin',(44.9999999999899,117.330999999998,-400.5));
#32166=CARTESIAN_POINT('',(37.9999999999905,109.330999999997,-400.5));
#32167=CARTESIAN_POINT('',(37.9999999999899,117.330999999997,-400.5));
#32168=CARTESIAN_POINT('',(37.9999999999899,117.330999999997,-400.5));
#32169=CARTESIAN_POINT('Origin',(44.99999999999,117.330999999997,-400.5));
#32170=CARTESIAN_POINT('Origin',(44.9999999999907,109.330999999998,-400.499999999999));
#32171=CARTESIAN_POINT('Origin',(37.9999999999899,117.330999999996,-406.));
#32172=CARTESIAN_POINT('',(37.9999999999899,117.330999999997,-403.5));
#32173=CARTESIAN_POINT('',(37.9999999999899,117.331000000002,-355.5));
#32174=CARTESIAN_POINT('',(37.9999999999905,109.330999999996,-410.5));
#32175=CARTESIAN_POINT('',(37.9999999999905,109.330999999997,-402.957368983363));
#32176=CARTESIAN_POINT('',(37.9999999999905,110.330999999996,-410.5));
#32177=CARTESIAN_POINT('',(37.9999999999899,117.330999999996,-410.5));
#32178=CARTESIAN_POINT('Origin',(37.9999999999905,110.330999999997,-403.5));
#32179=CARTESIAN_POINT('Origin',(-47.0000000000094,109.330999999989,-404.964101615149));
#32180=CARTESIAN_POINT('',(-49.0000000000094,109.330999999989,-406.118802153499));
#32181=CARTESIAN_POINT('',(-45.0000000000094,109.330999999989,-403.809401076799));
#32182=CARTESIAN_POINT('',(-49.0000000000094,109.330999999989,-406.118802153499));
#32183=CARTESIAN_POINT('',(-49.0000000000094,109.330999999989,-406.118802153499));
#32184=CARTESIAN_POINT('',(-45.0000000000094,109.330999999989,-403.809401076799));
#32185=CARTESIAN_POINT('Origin',(-45.0000000000094,109.33099999999,-401.5));
#32186=CARTESIAN_POINT('',(-45.0000000000094,109.33099999999,-399.190598923199));
#32187=CARTESIAN_POINT('',(-45.0000000000094,109.330999999989,-402.957368983363));
#32188=CARTESIAN_POINT('',(-45.0000000000094,109.33099999999,-399.190598923199));
#32189=CARTESIAN_POINT('Origin',(-47.0000000000094,109.33099999999,-398.035898384849));
#32190=CARTESIAN_POINT('',(-49.0000000000094,109.33099999999,-396.881197846499));
#32191=CARTESIAN_POINT('',(-45.0000000000094,109.33099999999,-399.190598923199));
#32192=CARTESIAN_POINT('',(-49.0000000000094,109.33099999999,-396.881197846499));
#32193=CARTESIAN_POINT('Origin',(-51.0000000000094,109.33099999999,-398.035898384849));
#32194=CARTESIAN_POINT('',(-53.0000000000094,109.330999999989,-399.190598923199));
#32195=CARTESIAN_POINT('',(-49.0000000000094,109.33099999999,-396.881197846499));
#32196=CARTESIAN_POINT('',(-53.0000000000094,109.330999999989,-399.190598923199));
#32197=CARTESIAN_POINT('Origin',(-53.0000000000094,109.330999999989,-401.5));
#32198=CARTESIAN_POINT('',(-53.0000000000094,109.330999999989,-403.809401076799));
#32199=CARTESIAN_POINT('',(-53.0000000000094,109.330999999989,-402.957368983363));
#32200=CARTESIAN_POINT('',(-53.0000000000094,109.330999999989,-403.809401076799));
#32201=CARTESIAN_POINT('Origin',(-51.0000000000094,109.330999999989,-404.964101615149));
#32202=CARTESIAN_POINT('',(-53.0000000000094,109.330999999989,-403.809401076799));
#32203=CARTESIAN_POINT('Origin',(-53.5000000000094,109.33099999999,-393.5));
#32204=CARTESIAN_POINT('',(-48.0000000000101,117.33099999999,-393.5));
#32205=CARTESIAN_POINT('',(-51.0000000000101,117.33099999999,-393.5));
#32206=CARTESIAN_POINT('',(-1.50000000001011,117.330999999994,-393.5));
#32207=CARTESIAN_POINT('',(-48.0000000000094,109.33099999999,-393.5));
#32208=CARTESIAN_POINT('',(-48.0000000000094,109.33099999999,-393.5));
#32209=CARTESIAN_POINT('',(-58.0000000000094,109.330999999989,-393.5));
#32210=CARTESIAN_POINT('',(-50.4573689833731,109.33099999999,-393.5));
#32211=CARTESIAN_POINT('',(-58.0000000000095,110.330999999989,-393.5));
#32212=CARTESIAN_POINT('',(-58.0000000000094,109.330999999989,-393.5));
#32213=CARTESIAN_POINT('Origin',(-51.0000000000095,110.33099999999,-393.5));
#32214=CARTESIAN_POINT('Origin',(-48.0000000000094,109.33099999999,-400.5));
#32215=CARTESIAN_POINT('',(-41.0000000000101,117.33099999999,-400.5));
#32216=CARTESIAN_POINT('',(-41.0000000000094,109.33099999999,-400.5));
#32217=CARTESIAN_POINT('',(-41.0000000000094,109.33099999999,-400.5));
#32218=CARTESIAN_POINT('Origin',(-48.0000000000095,109.33099999999,-400.5));
#32219=CARTESIAN_POINT('Origin',(-48.0000000000101,117.33099999999,-400.500000000001));
#32220=CARTESIAN_POINT('Origin',(-41.0000000000094,109.33099999999,-406.));
#32221=CARTESIAN_POINT('',(-41.0000000000094,109.330999999989,-410.5));
#32222=CARTESIAN_POINT('',(-41.0000000000095,110.330999999989,-410.5));
#32223=CARTESIAN_POINT('',(-41.0000000000094,109.330999999989,-410.5));
#32224=CARTESIAN_POINT('',(-41.0000000000094,109.33099999999,-402.957368983363));
#32225=CARTESIAN_POINT('',(-41.0000000000101,117.33099999999,-403.5));
#32226=CARTESIAN_POINT('',(-41.0000000000101,117.330999999995,-355.5));
#32227=CARTESIAN_POINT('Origin',(-41.0000000000095,110.33099999999,-403.5));
#32228=CARTESIAN_POINT('Origin',(47.9999999999906,109.331000000008,-312.964101615149));
#32229=CARTESIAN_POINT('',(45.9999999999906,109.331000000008,-314.118802153499));
#32230=CARTESIAN_POINT('',(49.9999999999906,109.331000000008,-311.809401076799));
#32231=CARTESIAN_POINT('',(45.9999999999906,109.331000000008,-314.118802153499));
#32232=CARTESIAN_POINT('',(45.9999999999906,109.331000000008,-314.118802153499));
#32233=CARTESIAN_POINT('',(49.9999999999906,109.331000000008,-311.809401076799));
#32234=CARTESIAN_POINT('Origin',(49.9999999999906,109.331000000009,-309.5));
#32235=CARTESIAN_POINT('',(49.9999999999906,109.331000000009,-307.190598923199));
#32236=CARTESIAN_POINT('',(49.9999999999906,109.331000000009,-308.042631016635));
#32237=CARTESIAN_POINT('',(49.9999999999906,109.331000000009,-307.190598923199));
#32238=CARTESIAN_POINT('Origin',(47.9999999999906,109.331000000009,-306.035898384849));
#32239=CARTESIAN_POINT('',(45.9999999999906,109.331000000009,-304.881197846499));
#32240=CARTESIAN_POINT('',(49.9999999999906,109.331000000009,-307.190598923199));
#32241=CARTESIAN_POINT('',(45.9999999999906,109.331000000009,-304.881197846499));
#32242=CARTESIAN_POINT('Origin',(43.9999999999906,109.331000000008,-306.035898384849));
#32243=CARTESIAN_POINT('',(41.9999999999906,109.331000000008,-307.190598923199));
#32244=CARTESIAN_POINT('',(45.9999999999906,109.331000000009,-304.881197846499));
#32245=CARTESIAN_POINT('',(41.9999999999906,109.331000000008,-307.190598923199));
#32246=CARTESIAN_POINT('Origin',(41.9999999999906,109.331000000008,-309.5));
#32247=CARTESIAN_POINT('',(41.9999999999906,109.331000000008,-311.809401076799));
#32248=CARTESIAN_POINT('',(41.9999999999906,109.331000000008,-308.042631016635));
#32249=CARTESIAN_POINT('',(41.9999999999906,109.331000000008,-311.809401076799));
#32250=CARTESIAN_POINT('Origin',(43.9999999999906,109.331000000008,-312.964101615149));
#32251=CARTESIAN_POINT('',(41.9999999999906,109.331000000008,-311.809401076799));
#32252=CARTESIAN_POINT('Origin',(50.4999999999906,109.331000000008,-317.5));
#32253=CARTESIAN_POINT('',(44.9999999999899,117.331000000007,-317.5));
#32254=CARTESIAN_POINT('',(47.9999999999899,117.331000000007,-317.5));
#32255=CARTESIAN_POINT('',(-1.50000000001011,117.331000000003,-317.5));
#32256=CARTESIAN_POINT('',(44.9999999999906,109.331000000007,-317.5));
#32257=CARTESIAN_POINT('',(44.9999999999906,109.331000000007,-317.5));
#32258=CARTESIAN_POINT('',(54.9999999999906,109.331000000008,-317.5));
#32259=CARTESIAN_POINT('',(47.4573689833543,109.331000000007,-317.5));
#32260=CARTESIAN_POINT('',(54.9999999999905,110.331000000008,-317.5));
#32261=CARTESIAN_POINT('',(54.9999999999906,109.331000000008,-317.5));
#32262=CARTESIAN_POINT('Origin',(47.9999999999905,110.331000000007,-317.5));
#32263=CARTESIAN_POINT('Origin',(44.9999999999906,109.331000000008,-310.5));
#32264=CARTESIAN_POINT('',(37.9999999999899,117.331000000007,-310.5));
#32265=CARTESIAN_POINT('',(37.9999999999905,109.331000000007,-310.5));
#32266=CARTESIAN_POINT('',(37.9999999999905,109.331000000007,-310.5));
#32267=CARTESIAN_POINT('Origin',(44.9999999999906,109.331000000008,-310.5));
#32268=CARTESIAN_POINT('Origin',(44.9999999999899,117.331000000008,-310.500000000001));
#32269=CARTESIAN_POINT('Origin',(37.9999999999905,109.331000000008,-305.));
#32270=CARTESIAN_POINT('',(37.9999999999905,109.331000000009,-300.5));
#32271=CARTESIAN_POINT('',(37.9999999999905,110.331000000009,-300.5));
#32272=CARTESIAN_POINT('',(37.9999999999905,109.331000000009,-300.5));
#32273=CARTESIAN_POINT('',(37.9999999999905,109.331000000008,-308.042631016635));
#32274=CARTESIAN_POINT('',(37.9999999999899,117.331000000008,-307.5));
#32275=CARTESIAN_POINT('',(37.9999999999899,117.331000000002,-355.5));
#32276=CARTESIAN_POINT('Origin',(37.9999999999905,110.331000000008,-307.5));
#32277=CARTESIAN_POINT('Origin',(-1.50000000001011,117.330999999999,-355.5));
#32278=CARTESIAN_POINT('',(-58.0000000000101,117.330999999988,-403.5));
#32279=CARTESIAN_POINT('',(-51.0000000000101,117.331,-317.5));
#32280=CARTESIAN_POINT('',(-51.0000000000101,117.330999999988,-410.5));
#32281=CARTESIAN_POINT('',(-48.0000000000101,117.331,-317.5));
#32282=CARTESIAN_POINT('',(-53.5000000000101,117.330999999999,-317.5));
#32283=CARTESIAN_POINT('',(-41.0000000000101,117.331,-310.5));
#32284=CARTESIAN_POINT('Origin',(-48.0000000000101,117.331,-310.500000000001));
#32285=CARTESIAN_POINT('',(-41.0000000000101,117.331,-307.5));
#32286=CARTESIAN_POINT('',(-41.0000000000101,117.331000000001,-305.));
#32287=CARTESIAN_POINT('',(-58.0000000000101,117.331,-307.5));
#32288=CARTESIAN_POINT('',(47.9999999999899,117.331000000009,-300.5));
#32289=CARTESIAN_POINT('Origin',(-47.0000000000094,109.331,-312.964101615149));
#32290=CARTESIAN_POINT('',(-49.0000000000094,109.331,-314.118802153499));
#32291=CARTESIAN_POINT('',(-45.0000000000094,109.331,-311.809401076799));
#32292=CARTESIAN_POINT('',(-49.0000000000094,109.331,-314.118802153499));
#32293=CARTESIAN_POINT('',(-49.0000000000095,109.331,-314.118802153499));
#32294=CARTESIAN_POINT('',(-45.0000000000094,109.331,-311.809401076799));
#32295=CARTESIAN_POINT('Origin',(-45.0000000000094,109.331,-309.5));
#32296=CARTESIAN_POINT('',(-45.0000000000094,109.331,-307.190598923199));
#32297=CARTESIAN_POINT('',(-45.0000000000094,109.331,-308.042631016635));
#32298=CARTESIAN_POINT('',(-45.0000000000094,109.331,-307.190598923199));
#32299=CARTESIAN_POINT('Origin',(-47.0000000000094,109.331,-306.035898384849));
#32300=CARTESIAN_POINT('',(-49.0000000000094,109.331,-304.881197846499));
#32301=CARTESIAN_POINT('',(-45.0000000000094,109.331,-307.190598923199));
#32302=CARTESIAN_POINT('',(-49.0000000000094,109.331,-304.881197846499));
#32303=CARTESIAN_POINT('Origin',(-51.0000000000094,109.331,-306.035898384849));
#32304=CARTESIAN_POINT('',(-53.0000000000094,109.331,-307.190598923199));
#32305=CARTESIAN_POINT('',(-49.0000000000094,109.331,-304.881197846499));
#32306=CARTESIAN_POINT('',(-53.0000000000094,109.331,-307.190598923199));
#32307=CARTESIAN_POINT('Origin',(-53.0000000000094,109.331,-309.5));
#32308=CARTESIAN_POINT('',(-53.0000000000094,109.331,-311.809401076799));
#32309=CARTESIAN_POINT('',(-53.0000000000094,109.331,-308.042631016635));
#32310=CARTESIAN_POINT('',(-53.0000000000094,109.331,-311.809401076799));
#32311=CARTESIAN_POINT('Origin',(-51.0000000000094,109.331,-312.964101615149));
#32312=CARTESIAN_POINT('',(-53.0000000000094,109.331,-311.809401076799));
#32313=CARTESIAN_POINT('Origin',(-41.0000000000094,109.331000000001,-305.));
#32314=CARTESIAN_POINT('',(-41.0000000000094,109.331,-310.5));
#32315=CARTESIAN_POINT('',(-41.0000000000094,109.331,-310.5));
#32316=CARTESIAN_POINT('',(-41.0000000000094,109.331000000002,-300.5));
#32317=CARTESIAN_POINT('',(-41.0000000000094,109.331,-308.042631016635));
#32318=CARTESIAN_POINT('',(-41.0000000000095,110.331000000002,-300.5));
#32319=CARTESIAN_POINT('',(-41.0000000000094,109.331000000002,-300.5));
#32320=CARTESIAN_POINT('Origin',(-41.0000000000095,110.331000000001,-307.5));
#32321=CARTESIAN_POINT('Origin',(-48.0000000000094,109.331,-310.5));
#32322=CARTESIAN_POINT('',(-48.0000000000094,109.331,-317.5));
#32323=CARTESIAN_POINT('',(-48.0000000000094,109.331,-317.5));
#32324=CARTESIAN_POINT('Origin',(-48.0000000000094,109.331000000001,-310.5));
#32325=CARTESIAN_POINT('Origin',(-53.5000000000094,109.330999999999,-317.5));
#32326=CARTESIAN_POINT('',(-58.0000000000094,109.330999999998,-317.5));
#32327=CARTESIAN_POINT('',(-58.0000000000095,110.330999999998,-317.5));
#32328=CARTESIAN_POINT('',(-58.0000000000094,109.330999999998,-317.5));
#32329=CARTESIAN_POINT('',(-50.4573689833731,109.331,-317.5));
#32330=CARTESIAN_POINT('Origin',(-51.0000000000095,110.330999999999,-317.499999999999));
#32331=CARTESIAN_POINT('Origin',(26.6129405624652,-47.4885629631521,-461.499999999981));
#32332=CARTESIAN_POINT('',(29.2172650211785,-63.2751868616857,-462.49999999998));
#32333=CARTESIAN_POINT('',(29.2172650211786,-63.2751868616856,-461.49999999998));
#32334=CARTESIAN_POINT('',(37.9266490614509,-58.8022714621361,-462.49999999998));
#32335=CARTESIAN_POINT('',(37.9266490614509,-58.802271462136,-461.499999999981));
#32336=CARTESIAN_POINT('Origin',(26.6129405624651,-47.4885629631522,-462.499999999891));
#32337=CARTESIAN_POINT('Origin',(47.6332714621302,-49.0956490614551,-461.499999999982));
#32338=CARTESIAN_POINT('',(47.6332714621302,-49.0956490614552,-462.499999999982));
#32339=CARTESIAN_POINT('',(47.6332714621302,-49.0956490614551,-461.499999999981));
#32340=CARTESIAN_POINT('',(37.9266490614509,-58.8022714621361,-462.49999999998));
#32341=CARTESIAN_POINT('Origin',(36.3195629631445,-37.7819405624712,-461.499999999982));
#32342=CARTESIAN_POINT('',(52.1061868616782,-40.3862650211816,-462.499999999983));
#32343=CARTESIAN_POINT('',(52.1061868616778,-40.3862650211815,-461.499999999983));
#32344=CARTESIAN_POINT('Origin',(36.3195629631445,-37.7819405624713,-462.499999999905));
#32345=CARTESIAN_POINT('Origin',(-125.,-11.1690000000246,-461.499999999984));
#32346=CARTESIAN_POINT('',(52.1061868616731,18.0482650211651,-462.49999999999));
#32347=CARTESIAN_POINT('',(52.1061868616733,18.0482650211652,-461.499999999989));
#32348=CARTESIAN_POINT('Origin',(-125.000000000001,-11.1690000000256,-462.49999999969));
#32349=CARTESIAN_POINT('Origin',(36.3195629631399,15.4439405624519,-461.499999999988));
#32350=CARTESIAN_POINT('',(47.6332714621237,26.7576490614375,-462.49999999999));
#32351=CARTESIAN_POINT('',(47.6332714621237,26.7576490614377,-461.49999999999));
#32352=CARTESIAN_POINT('Origin',(36.3195629631398,15.4439405624517,-462.499999999907));
#32353=CARTESIAN_POINT('Origin',(37.9266490614429,36.4642714621169,-461.499999999991));
#32354=CARTESIAN_POINT('',(37.9266490614428,36.4642714621168,-462.499999999991));
#32355=CARTESIAN_POINT('',(37.9266490614428,36.4642714621169,-461.499999999991));
#32356=CARTESIAN_POINT('',(47.6332714621237,26.7576490614375,-462.49999999999));
#32357=CARTESIAN_POINT('Origin',(26.6129405624589,25.1505629631313,-461.499999999989));
#32358=CARTESIAN_POINT('',(29.2172650211694,40.9371868616652,-462.499999999991));
#32359=CARTESIAN_POINT('',(29.2172650211694,40.9371868616654,-461.499999999992));
#32360=CARTESIAN_POINT('Origin',(26.6129405624589,25.1505629631313,-462.499999999889));
#32361=CARTESIAN_POINT('Origin',(1.22402088464923E-11,-136.169000000013,
-461.499999999971));
#32362=CARTESIAN_POINT('',(-29.2172650211774,40.9371868616598,-462.499999999991));
#32363=CARTESIAN_POINT('',(-29.2172650211774,40.9371868616601,-461.499999999991));
#32364=CARTESIAN_POINT('Origin',(1.38211769938405E-11,-136.16900000002,
-462.499999998645));
#32365=CARTESIAN_POINT('Origin',(-26.6129405624642,25.1505629631266,-461.499999999989));
#32366=CARTESIAN_POINT('',(-37.9266490614499,36.4642714621103,-462.499999999991));
#32367=CARTESIAN_POINT('',(-37.9266490614499,36.4642714621104,-461.49999999999));
#32368=CARTESIAN_POINT('Origin',(-26.6129405624642,25.1505629631265,-462.499999999905));
#32369=CARTESIAN_POINT('Origin',(-47.6332714621292,26.7576490614295,-461.499999999989));
#32370=CARTESIAN_POINT('',(-47.6332714621292,26.7576490614294,-462.499999999989));
#32371=CARTESIAN_POINT('',(-47.6332714621292,26.7576490614296,-461.49999999999));
#32372=CARTESIAN_POINT('',(-37.9266490614499,36.4642714621103,-462.49999999999));
#32373=CARTESIAN_POINT('Origin',(-36.3195629631435,15.4439405624457,-461.499999999988));
#32374=CARTESIAN_POINT('Origin',(-36.3195629631436,15.4439405624456,-462.499999999891));
#32375=CARTESIAN_POINT('Origin',(-36.3195629631389,-37.7819405624774,-461.499999999982));
#32376=CARTESIAN_POINT('',(-47.6332714621227,-49.0956490614632,-462.49999999998));
#32377=CARTESIAN_POINT('',(-47.6332714621227,-49.0956490614631,-461.499999999981));
#32378=CARTESIAN_POINT('Origin',(-36.3195629631389,-37.7819405624776,-462.499999999884));
#32379=CARTESIAN_POINT('Origin',(-37.9266490614418,-58.8022714621425,-461.49999999998));
#32380=CARTESIAN_POINT('',(-37.9266490614418,-58.8022714621426,-462.49999999998));
#32381=CARTESIAN_POINT('',(-37.9266490614418,-58.8022714621425,-461.49999999998));
#32382=CARTESIAN_POINT('',(-47.6332714621227,-49.0956490614632,-462.49999999998));
#32383=CARTESIAN_POINT('Origin',(-26.612940562458,-47.4885629631568,-461.499999999981));
#32384=CARTESIAN_POINT('',(-29.2172650211685,-63.2751868616909,-462.499999999979));
#32385=CARTESIAN_POINT('',(-29.2172650211685,-63.2751868616907,-461.499999999979));
#32386=CARTESIAN_POINT('Origin',(-26.612940562458,-47.488562963157,-462.499999999894));
#32387=CARTESIAN_POINT('Origin',(-1.04360964314765E-11,113.830999999987,
-461.5));
#32388=CARTESIAN_POINT('Origin',(-1.14310418010589E-11,113.830999999992,
-462.499999998675));
#32389=CARTESIAN_POINT('Origin',(52.4999999999929,82.5008729811058,-335.999999999996));
#32390=CARTESIAN_POINT('',(55.1642481716112,83.9442486541057,-338.499999999996));
#32391=CARTESIAN_POINT('',(52.4999999999928,83.9442486541055,-338.499999999996));
#32392=CARTESIAN_POINT('',(55.1642481716032,81.0574973081063,-333.499999999996));
#32393=CARTESIAN_POINT('',(52.4999999999931,81.0574973081061,-333.499999999996));
#32394=CARTESIAN_POINT('Origin',(35.6399999999928,82.5008729811182,-336.00000000002));
#32395=CARTESIAN_POINT('Origin',(52.4999999999929,82.5008729811064,-330.999999999996));
#32396=CARTESIAN_POINT('',(55.1642481716112,83.9442486541069,-328.499999999996));
#32397=CARTESIAN_POINT('',(52.4999999999928,83.9442486541067,-328.499999999996));
#32398=CARTESIAN_POINT('Origin',(35.6399999999928,82.5008729811189,-330.999999999972));
#32399=CARTESIAN_POINT('Origin',(52.4999999999926,86.8310000000067,-328.499999999996));
#32400=CARTESIAN_POINT('',(55.1642481716107,89.7177513459069,-328.5));
#32401=CARTESIAN_POINT('',(52.4999999999923,89.7177513459067,-328.5));
#32402=CARTESIAN_POINT('Origin',(35.6399999998842,86.8310000000025,-328.500000000393));
#32403=CARTESIAN_POINT('Origin',(52.4999999999922,91.1611270189064,-331.));
#32404=CARTESIAN_POINT('',(55.1642481716022,92.6045026919063,-333.5));
#32405=CARTESIAN_POINT('',(52.499999999992,92.6045026919061,-333.5));
#32406=CARTESIAN_POINT('Origin',(35.639999999992,91.1611270188897,-330.999999999974));
#32407=CARTESIAN_POINT('Origin',(52.4999999999922,91.1611270189058,-336.));
#32408=CARTESIAN_POINT('',(55.1642481716107,89.7177513459057,-338.5));
#32409=CARTESIAN_POINT('',(52.4999999999923,89.7177513459055,-338.5));
#32410=CARTESIAN_POINT('Origin',(35.639999999992,91.1611270188918,-336.000000000022));
#32411=CARTESIAN_POINT('Origin',(52.4999999999927,85.3876243270555,-338.499999999996));
#32412=CARTESIAN_POINT('Origin',(35.6400000000029,86.8310000000037,-338.500000000075));
#32413=CARTESIAN_POINT('Origin',(52.4999999999929,82.5008729811008,-380.));
#32414=CARTESIAN_POINT('',(55.1642481716112,83.9442486541007,-382.5));
#32415=CARTESIAN_POINT('',(52.4999999999928,83.9442486541005,-382.5));
#32416=CARTESIAN_POINT('',(55.1642481716032,81.0574973081013,-377.5));
#32417=CARTESIAN_POINT('',(52.4999999999931,81.057497308101,-377.5));
#32418=CARTESIAN_POINT('Origin',(35.6399999999927,82.5008729811131,-380.000000000024));
#32419=CARTESIAN_POINT('Origin',(52.4999999999929,82.5008729811013,-375.));
#32420=CARTESIAN_POINT('',(55.1642481716112,83.9442486541018,-372.5));
#32421=CARTESIAN_POINT('',(52.4999999999928,83.9442486541016,-372.5));
#32422=CARTESIAN_POINT('Origin',(35.6399999999927,82.5008729811141,-374.999999999975));
#32423=CARTESIAN_POINT('Origin',(52.4999999999926,86.8310000000016,-372.5));
#32424=CARTESIAN_POINT('',(55.1642481716107,89.7177513459018,-372.5));
#32425=CARTESIAN_POINT('',(52.4999999999923,89.7177513459016,-372.5));
#32426=CARTESIAN_POINT('Origin',(35.6400000000052,86.8310000000011,-372.499999999934));
#32427=CARTESIAN_POINT('Origin',(52.4999999999922,91.1611270189013,-375.));
#32428=CARTESIAN_POINT('',(55.1642481716022,92.6045026919012,-377.5));
#32429=CARTESIAN_POINT('',(52.499999999992,92.604502691901,-377.5));
#32430=CARTESIAN_POINT('Origin',(35.639999999992,91.1611270188862,-374.999999999976));
#32431=CARTESIAN_POINT('Origin',(52.4999999999922,91.1611270189007,-380.));
#32432=CARTESIAN_POINT('',(55.1642481716107,89.7177513459007,-382.5));
#32433=CARTESIAN_POINT('',(52.4999999999923,89.7177513459005,-382.5));
#32434=CARTESIAN_POINT('Origin',(35.639999999992,91.1611270188853,-380.000000000024));
#32435=CARTESIAN_POINT('Origin',(52.4999999999927,85.3876243270505,-382.5));
#32436=CARTESIAN_POINT('Origin',(35.6400000000109,86.8309999999987,-382.500000000053));
#32437=CARTESIAN_POINT('Origin',(47.9999999999905,110.331000000009,-300.5));
#32438=CARTESIAN_POINT('',(54.9999999999905,110.331000000004,-355.5));
#32439=CARTESIAN_POINT('Origin',(-58.0000000000095,110.330999999988,-403.5));
#32440=CARTESIAN_POINT('',(-1.5000000000095,110.330999999992,-410.5));
#32441=CARTESIAN_POINT('Origin',(47.4573689833543,109.330999999998,-402.957368983363));
#32442=CARTESIAN_POINT('',(47.9999999999906,109.330999999997,-410.5));
#32443=CARTESIAN_POINT('',(54.9999999999906,109.330999999998,-403.5));
#32444=CARTESIAN_POINT('Origin',(47.9999999999906,109.330999999998,-403.500000000001));
#32445=CARTESIAN_POINT('',(-1.50000000000941,109.330999999992,-410.5));
#32446=CARTESIAN_POINT('',(54.9999999999906,109.331000000004,-355.5));
#32447=CARTESIAN_POINT('Origin',(-51.0000000000095,110.330999999988,-410.5));
#32448=CARTESIAN_POINT('',(-58.0000000000095,110.330999999994,-355.5));
#32449=CARTESIAN_POINT('Origin',(-50.4573689833731,109.330999999989,-402.957368983363));
#32450=CARTESIAN_POINT('',(-51.0000000000094,109.330999999988,-410.5));
#32451=CARTESIAN_POINT('',(-1.50000000000941,109.330999999992,-410.5));
#32452=CARTESIAN_POINT('',(-58.0000000000094,109.330999999988,-403.5));
#32453=CARTESIAN_POINT('Origin',(-51.0000000000094,109.330999999989,-403.500000000001));
#32454=CARTESIAN_POINT('',(-58.0000000000094,109.330999999994,-355.5));
#32455=CARTESIAN_POINT('Origin',(47.4573689833543,109.331000000009,-308.042631016635));
#32456=CARTESIAN_POINT('',(47.9999999999906,109.331000000009,-300.5));
#32457=CARTESIAN_POINT('',(-26.2500000000094,109.331000000003,-300.5));
#32458=CARTESIAN_POINT('',(54.9999999999906,109.331000000009,-307.5));
#32459=CARTESIAN_POINT('Origin',(47.9999999999906,109.331000000009,-307.500000000001));
#32460=CARTESIAN_POINT('',(54.9999999999906,109.331000000004,-355.5));
#32461=CARTESIAN_POINT('Origin',(-58.0000000000095,110.331,-307.5));
#32462=CARTESIAN_POINT('',(-26.2500000000095,110.331000000003,-300.5));
#32463=CARTESIAN_POINT('Origin',(-50.4573689833731,109.331,-308.042631016635));
#32464=CARTESIAN_POINT('',(-58.0000000000094,109.331,-307.5));
#32465=CARTESIAN_POINT('',(-58.0000000000094,109.330999999994,-355.5));
#32466=CARTESIAN_POINT('',(-51.0000000000094,109.331,-300.5));
#32467=CARTESIAN_POINT('Origin',(-51.0000000000095,109.331,-307.500000000001));
#32468=CARTESIAN_POINT('',(-26.2500000000094,109.331000000003,-300.5));
#32469=CARTESIAN_POINT('Origin',(-61.0064055375887,-63.6901241633721,-442.499999999978));
#32470=CARTESIAN_POINT('',(-53.0300791427081,-49.8747215894684,-462.499718596329));
#32471=CARTESIAN_POINT('',(-56.5529890060881,-55.976580463545,-455.455487085872));
#32472=CARTESIAN_POINT('Ctrl Pts',(-53.0302197456166,-49.8749651210668,
-462.499437315867));
#32473=CARTESIAN_POINT('Ctrl Pts',(-53.5772253220562,-50.8224065714837,
-461.405135361616));
#32474=CARTESIAN_POINT('Ctrl Pts',(-54.1391093421611,-51.7956182422464,
-460.281440602366));
#32475=CARTESIAN_POINT('Ctrl Pts',(-55.3014638055348,-53.8088752292143,
-457.95729552662));
#32476=CARTESIAN_POINT('Ctrl Pts',(-55.9378134738743,-54.9110651861781,
-456.685162782456));
#32477=CARTESIAN_POINT('Ctrl Pts',(-56.5529890060879,-55.9765804635453,
-455.455487085872));
#32478=CARTESIAN_POINT('',(-61.0064055375889,-63.6901241633744,-462.499999999978));
#32479=CARTESIAN_POINT('',(-61.0064055375889,-63.6901241633744,-462.499999999979));
#32480=CARTESIAN_POINT('',(-61.0064055375888,-63.6901241633726,-446.555000365155));
#32481=CARTESIAN_POINT('',(-61.0064055375887,-63.6901241633722,-442.499999999978));
#32482=CARTESIAN_POINT('Ctrl Pts',(-56.5529890060879,-55.9765804635452,
-455.455487085872));
#32483=CARTESIAN_POINT('Ctrl Pts',(-57.3037589083373,-57.2769520790348,
-453.954027830977));
#32484=CARTESIAN_POINT('Ctrl Pts',(-58.1291756986755,-58.7066158973974,
-452.303717577715));
#32485=CARTESIAN_POINT('Ctrl Pts',(-59.614164504551,-61.2786919578449,-449.335876617764));
#32486=CARTESIAN_POINT('Ctrl Pts',(-60.3130716773339,-62.4892346908032,
-447.93954461762));
#32487=CARTESIAN_POINT('Ctrl Pts',(-61.0064055375887,-63.6901241633725,
-446.555000365155));
#32488=CARTESIAN_POINT('Origin',(6.66133814775094E-13,-11.1690000000111,
-442.499999999986));
#32489=CARTESIAN_POINT('',(-52.5211241633496,-72.1754055376122,-462.499999999977));
#32490=CARTESIAN_POINT('Origin',(3.5527136788005E-13,-11.1690000000144,
-462.49999999999));
#32491=CARTESIAN_POINT('',(-52.5211241633495,-72.1754055376103,-446.554850154037));
#32492=CARTESIAN_POINT('',(-52.5211241633495,-72.1754055376099,-442.499999999978));
#32493=CARTESIAN_POINT('Ctrl Pts',(-61.0064055375888,-63.6901241633725,
-446.555000365155));
#32494=CARTESIAN_POINT('Ctrl Pts',(-59.7028303851691,-65.2043041369367,
-446.489771872832));
#32495=CARTESIAN_POINT('Ctrl Pts',(-58.3409919033042,-66.6719343927154,
-446.458142664235));
#32496=CARTESIAN_POINT('Ctrl Pts',(-55.5103141820403,-69.5031427304158,
-446.457920540329));
#32497=CARTESIAN_POINT('Ctrl Pts',(-54.0391111582702,-70.8685528762214,
-446.489484908003));
#32498=CARTESIAN_POINT('Ctrl Pts',(-52.5211241633495,-72.1754055376103,
-446.554850154037));
#32499=CARTESIAN_POINT('Origin',(-52.5211241633494,-72.1754055376099,-442.499999999978));
#32500=CARTESIAN_POINT('',(-38.7057432251289,-64.1990916340934,-462.499726017634));
#32501=CARTESIAN_POINT('',(-38.705506016167,-64.1989546813131,-462.499999999979));
#32502=CARTESIAN_POINT('',(-44.7374479018055,-67.6814979526866,-455.53635793138));
#32503=CARTESIAN_POINT('Ctrl Pts',(-44.7374479017809,-67.6814979527087,
-455.536357931381));
#32504=CARTESIAN_POINT('Ctrl Pts',(-43.6857872701621,-67.0743214039474,
-456.750069874714));
#32505=CARTESIAN_POINT('Ctrl Pts',(-42.5978914217962,-66.446224443087,-458.005729087235));
#32506=CARTESIAN_POINT('Ctrl Pts',(-40.6077271815802,-65.2972025832667,
-460.30325547882));
#32507=CARTESIAN_POINT('Ctrl Pts',(-39.6441515550798,-64.7408819358782,
-461.415842174298));
#32508=CARTESIAN_POINT('Ctrl Pts',(-38.7059803294307,-64.1992285262037,
-462.499452156896));
#32509=CARTESIAN_POINT('Ctrl Pts',(-52.5211241633495,-72.1754055376104,
-446.554850154037));
#32510=CARTESIAN_POINT('Ctrl Pts',(-51.309846368319,-71.4760739765861,-447.951355698663));
#32511=CARTESIAN_POINT('Ctrl Pts',(-50.0887918485801,-70.7710978208717,
-449.359814919897));
#32512=CARTESIAN_POINT('Ctrl Pts',(-47.4933387038742,-69.2726122491067,
-452.354661179647));
#32513=CARTESIAN_POINT('Ctrl Pts',(-46.0497544858338,-68.439158512271,-454.021075738748));
#32514=CARTESIAN_POINT('Ctrl Pts',(-44.7374479017856,-67.6814979527114,
-455.536357931375));
#32515=CARTESIAN_POINT('Origin',(52.5211241633613,-72.1754055376007,-442.49999999998));
#32516=CARTESIAN_POINT('',(52.5211241633611,-72.175405537603,-462.499999999979));
#32517=CARTESIAN_POINT('',(52.5211241633611,-72.175405537603,-462.499999999979));
#32518=CARTESIAN_POINT('',(52.5211241633613,-72.1754055376012,-446.555918723113));
#32519=CARTESIAN_POINT('',(52.5211241633614,-72.1754055376007,-442.499999999979));
#32520=CARTESIAN_POINT('Ctrl Pts',(44.737447901791,-67.6814979527004,-455.536357931383));
#32521=CARTESIAN_POINT('Ctrl Pts',(46.0484136650392,-68.4383843890099,-454.022827080102));
#32522=CARTESIAN_POINT('Ctrl Pts',(47.4933110155619,-69.2725962632375,-452.355109735904));
#32523=CARTESIAN_POINT('Ctrl Pts',(50.0889455884469,-70.7711865826099,-449.360409943347));
#32524=CARTESIAN_POINT('Ctrl Pts',(51.3099391726234,-71.4761275571605,-447.952177252778));
#32525=CARTESIAN_POINT('Ctrl Pts',(52.5211241633614,-72.1754055376012,-446.555918723113));
#32526=CARTESIAN_POINT('Origin',(6.66133814775094E-13,-11.1690000000111,
-442.499999999986));
#32527=CARTESIAN_POINT('',(61.006405537599,-63.6901241633638,-462.49999999998));
#32528=CARTESIAN_POINT('Origin',(-2.93098878501041E-13,-11.1690000000144,
-462.499999999992));
#32529=CARTESIAN_POINT('',(61.0064055375993,-63.6901241633619,-446.556015654869));
#32530=CARTESIAN_POINT('',(61.0064055375992,-63.6901241633614,-442.49999999998));
#32531=CARTESIAN_POINT('Ctrl Pts',(52.5211241633613,-72.1754055376012,-446.555918723113));
#32532=CARTESIAN_POINT('Ctrl Pts',(54.0377808744736,-70.8696981330166,-446.490122433087));
#32533=CARTESIAN_POINT('Ctrl Pts',(55.5077540668189,-69.5055188910036,-446.458279670062));
#32534=CARTESIAN_POINT('Ctrl Pts',(58.3386174884044,-66.6744930634029,-446.458344295615));
#32535=CARTESIAN_POINT('Ctrl Pts',(59.7017006172735,-65.2056164294591,-446.490203981457));
#32536=CARTESIAN_POINT('Ctrl Pts',(61.0064055375992,-63.6901241633618,-446.55601565487));
#32537=CARTESIAN_POINT('Origin',(61.0064055375992,-63.6901241633614,-442.49999999998));
#32538=CARTESIAN_POINT('Ctrl Pts',(61.0064055375992,-63.690124163362,-446.55601565487));
#32539=CARTESIAN_POINT('Ctrl Pts',(60.3129264164325,-62.4889830915135,-447.94070717192));
#32540=CARTESIAN_POINT('Ctrl Pts',(59.6139369007277,-61.2782977364298,-449.337050349079));
#32541=CARTESIAN_POINT('Ctrl Pts',(58.1287483302424,-58.7058756735295,-452.304951999478));
#32542=CARTESIAN_POINT('Ctrl Pts',(57.3027210262701,-57.2751544145364,-453.956286633532));
#32543=CARTESIAN_POINT('Ctrl Pts',(56.5529890060965,-55.9765804635349,-455.455487085874));
#32544=CARTESIAN_POINT('',(53.0295409752009,-49.8737894561974,-462.499999999981));
#32545=CARTESIAN_POINT('Origin',(61.0064055375901,41.3521241633499,-442.499999999992));
#32546=CARTESIAN_POINT('',(61.0064055375899,41.3521241633477,-462.499999999992));
#32547=CARTESIAN_POINT('',(61.0064055375899,41.3521241633477,-462.499999999992));
#32548=CARTESIAN_POINT('',(61.00640553759,41.3521241633499,-442.499999999992));
#32549=CARTESIAN_POINT('Origin',(6.66133814775094E-13,-11.1690000000111,
-442.499999999986));
#32550=CARTESIAN_POINT('',(52.5211241633506,49.8374055375854,-462.499999999993));
#32551=CARTESIAN_POINT('Origin',(2.91322521661641E-12,-11.1690000000106,
-462.49999999998));
#32552=CARTESIAN_POINT('',(52.5211241633507,49.8374055375877,-442.499999999993));
#32553=CARTESIAN_POINT('Origin',(52.5211241633508,49.8374055375877,-442.499999999993));
#32554=CARTESIAN_POINT('',(38.7052701169132,41.8608184847882,-462.499999999992));
#32555=CARTESIAN_POINT('Origin',(-52.5211241633601,49.8374055375786,-442.499999999991));
#32556=CARTESIAN_POINT('',(-43.5419127712896,44.6532698807934,-456.914899800777));
#32557=CARTESIAN_POINT('',(-38.7066184322078,41.8615969349749,-462.499999999991));
#32558=CARTESIAN_POINT('Ctrl Pts',(-43.5419565207299,44.6532806820063,-456.914942914046));
#32559=CARTESIAN_POINT('Ctrl Pts',(-43.3888210609314,44.5648678830691,-457.092282683389));
#32560=CARTESIAN_POINT('Ctrl Pts',(-43.260269592342,44.4906486580742,-457.241800248498));
#32561=CARTESIAN_POINT('Ctrl Pts',(-42.7372899671077,44.1887062306645,-457.847255790856));
#32562=CARTESIAN_POINT('Ctrl Pts',(-42.535915318321,44.0724425229795,-458.080116830013));
#32563=CARTESIAN_POINT('Ctrl Pts',(-41.9435098505755,43.7304170667072,-458.764642376408));
#32564=CARTESIAN_POINT('Ctrl Pts',(-41.4886182402114,43.4677852730115,-459.289573202535));
#32565=CARTESIAN_POINT('Ctrl Pts',(-40.3188335853071,42.7924097876085,-460.639149869349));
#32566=CARTESIAN_POINT('Ctrl Pts',(-39.5123048656016,42.3267602141773,-461.569029335436));
#32567=CARTESIAN_POINT('Ctrl Pts',(-38.7066184322079,41.861596934975,-462.499999999991));
#32568=CARTESIAN_POINT('',(-52.5211241633603,49.8374055375763,-462.499999999992));
#32569=CARTESIAN_POINT('',(-52.5211241633602,49.8374055375763,-462.499999999992));
#32570=CARTESIAN_POINT('',(-52.5211241633601,49.837405537578,-446.550390587012));
#32571=CARTESIAN_POINT('',(-52.5211241633601,49.8374055375786,-442.499999999991));
#32572=CARTESIAN_POINT('Ctrl Pts',(-43.5418850933958,44.6532394434158,-456.91486058488));
#32573=CARTESIAN_POINT('Ctrl Pts',(-45.0572774506985,45.5281516288324,-455.163894143534));
#32574=CARTESIAN_POINT('Ctrl Pts',(-46.7377899355917,46.4983959641712,-453.222925656717));
#32575=CARTESIAN_POINT('Ctrl Pts',(-49.7321482182746,48.2271895247285,-449.766679504493));
#32576=CARTESIAN_POINT('Ctrl Pts',(-51.1321942398983,49.0355064723819,-448.151530117407));
#32577=CARTESIAN_POINT('Ctrl Pts',(-52.5211241633599,49.837405537578,-446.550390587012));
#32578=CARTESIAN_POINT('Origin',(6.66133814775094E-13,-11.1690000000111,
-442.499999999986));
#32579=CARTESIAN_POINT('',(-61.0064055375982,41.352124163337,-462.499999999991));
#32580=CARTESIAN_POINT('Origin',(-2.38031816479634E-12,-11.1690000000101,
-462.499999999979));
#32581=CARTESIAN_POINT('',(-61.0064055375979,41.3521241633388,-446.553488658841));
#32582=CARTESIAN_POINT('',(-61.0064055375979,41.3521241633393,-442.49999999999));
#32583=CARTESIAN_POINT('Ctrl Pts',(-52.5211241633601,49.8374055375781,-446.550390587012));
#32584=CARTESIAN_POINT('Ctrl Pts',(-54.0643256331624,48.5088454414645,-446.486213866141));
#32585=CARTESIAN_POINT('Ctrl Pts',(-55.5591057416034,47.1198261279319,-446.455982678674));
#32586=CARTESIAN_POINT('Ctrl Pts',(-58.3862727598194,44.2851113555294,-446.459187956062));
#32587=CARTESIAN_POINT('Ctrl Pts',(-59.7244711699984,42.8411670798447,-446.490453383587));
#32588=CARTESIAN_POINT('Ctrl Pts',(-61.006405537598,41.3521241633388,-446.553488658841));
#32589=CARTESIAN_POINT('Origin',(-61.0064055375979,41.3521241633393,-442.49999999999));
#32590=CARTESIAN_POINT('',(-56.5529890060949,33.6385804635094,-455.455487085884));
#32591=CARTESIAN_POINT('Ctrl Pts',(-61.0064055375978,41.3521241633387,-446.553488658841));
#32592=CARTESIAN_POINT('Ctrl Pts',(-60.3110035926517,40.1476526630098,-447.942369697286));
#32593=CARTESIAN_POINT('Ctrl Pts',(-59.6106476791202,38.9346006374547,-449.341816313449));
#32594=CARTESIAN_POINT('Ctrl Pts',(-58.1300841047959,36.3701893028892,-452.30131448445));
#32595=CARTESIAN_POINT('Ctrl Pts',(-57.3381109788292,34.9984516104232,-453.885022424417));
#32596=CARTESIAN_POINT('Ctrl Pts',(-56.5529890060949,33.6385804635089,-455.455487085883));
#32597=CARTESIAN_POINT('',(-53.0305574330481,27.5375500128072,-462.499999999989));
#32598=CARTESIAN_POINT('',(-53.030557433048,27.537550012807,-462.499999999989));
#32599=CARTESIAN_POINT('Ctrl Pts',(-56.5529890060952,33.6385804635093,-455.455487085884));
#32600=CARTESIAN_POINT('Ctrl Pts',(-55.9412708023145,32.5790534546464,-456.678496830178));
#32601=CARTESIAN_POINT('Ctrl Pts',(-55.3067518807507,31.4800344443309,-457.947209569429));
#32602=CARTESIAN_POINT('Ctrl Pts',(-54.1447199575835,29.4673361133885,-460.271113052516));
#32603=CARTESIAN_POINT('Ctrl Pts',(-53.5798271593038,28.4889130857417,-461.401007474302));
#32604=CARTESIAN_POINT('Ctrl Pts',(-53.0305574330482,27.5375500128075,-462.499999999989));
#32605=CARTESIAN_POINT('Origin',(-104.132690000718,86.3051835969643,-462.5));
#32606=CARTESIAN_POINT('',(12.0150531445647,47.9060664143426,-462.499999999992));
#32607=CARTESIAN_POINT('',(18.8780323271008,47.6380911509506,-462.499968784806));
#32608=CARTESIAN_POINT('Ctrl Pts',(12.0150531445629,47.906066414339,-462.499999999997));
#32609=CARTESIAN_POINT('Ctrl Pts',(12.3401897703731,47.7470231052897,-462.499999999997));
#32610=CARTESIAN_POINT('Ctrl Pts',(13.4663873030089,47.1961341237507,-462.499999999997));
#32611=CARTESIAN_POINT('Ctrl Pts',(15.7097574528983,47.0181411184891,-462.499999999997));
#32612=CARTESIAN_POINT('Ctrl Pts',(16.3411029419287,47.0389120836614,-462.499999999997));
#32613=CARTESIAN_POINT('Ctrl Pts',(17.8946098878202,47.2634700470991,-462.499999999997));
#32614=CARTESIAN_POINT('Ctrl Pts',(18.3628654099176,47.4345106517495,-462.499999999997));
#32615=CARTESIAN_POINT('Ctrl Pts',(18.8780355053135,47.6380912035477,-462.499999999997));
#32616=CARTESIAN_POINT('Ctrl Pts',(31.7952304123374,45.4237242247432,-462.499999999997));
#32617=CARTESIAN_POINT('Ctrl Pts',(25.3169775513725,46.8233621997,-462.499999999997));
#32618=CARTESIAN_POINT('Ctrl Pts',(18.8780323213069,47.6380669487686,-462.499999999997));
#32619=CARTESIAN_POINT('Ctrl Pts',(56.5915605594614,20.625879662293,-462.499999999994));
#32620=CARTESIAN_POINT('Ctrl Pts',(56.3136127711561,21.9073690239263,-462.499999999994));
#32621=CARTESIAN_POINT('Ctrl Pts',(55.8688443804651,23.1467900735692,-462.500000000367));
#32622=CARTESIAN_POINT('Ctrl Pts',(54.6666325419165,25.4805815867024,-462.500000000368));
#32623=CARTESIAN_POINT('Ctrl Pts',(53.9138954951052,26.5642794410027,-462.499999999995));
#32624=CARTESIAN_POINT('Ctrl Pts',(53.0293871551266,27.5359584349847,-462.499999999995));
#32625=CARTESIAN_POINT('',(57.7295804999065,14.830443173281,-462.499999999989));
#32626=CARTESIAN_POINT('Origin',(-90.0000000001335,-11.1690000000447,-462.499999999809));
#32627=CARTESIAN_POINT('',(58.3152526334991,7.11256737781201,-462.499999999988));
#32628=CARTESIAN_POINT('Ctrl Pts',(57.7295804999045,14.8304431732815,-462.499999999993));
#32629=CARTESIAN_POINT('Ctrl Pts',(57.4005325308538,13.5557935149812,-462.499999999993));
#32630=CARTESIAN_POINT('Ctrl Pts',(57.283465559692,12.2356510331148,-462.499999999992));
#32631=CARTESIAN_POINT('Ctrl Pts',(57.4826884205102,9.61033012876741,-462.499999999992));
#32632=CARTESIAN_POINT('Ctrl Pts',(57.7976276531099,8.32296394996483,-462.499999999993));
#32633=CARTESIAN_POINT('Ctrl Pts',(58.3152526334968,7.11256737781103,-462.499999999993));
#32634=CARTESIAN_POINT('',(59.0902650976006,-0.703506953302192,-462.499999999987));
#32635=CARTESIAN_POINT('Ctrl Pts',(58.3152526334968,7.11256737781104,-462.499999999993));
#32636=CARTESIAN_POINT('Ctrl Pts',(58.8390772674901,5.88767374744325,-462.499999999992));
#32637=CARTESIAN_POINT('Ctrl Pts',(59.1725049660372,4.58984165948011,-462.499999999988));
#32638=CARTESIAN_POINT('Ctrl Pts',(59.435407607139,1.93844399318233,-462.499999999988));
#32639=CARTESIAN_POINT('Ctrl Pts',(59.3633429804589,0.600404665165133,-462.499999999992));
#32640=CARTESIAN_POINT('Ctrl Pts',(59.0902650975989,-0.703506953301665,
-462.499999999992));
#32641=CARTESIAN_POINT('',(59.406405003267,-7.27543664706474,-462.499999999987));
#32642=CARTESIAN_POINT('Ctrl Pts',(59.0902650975988,-0.703506953301827,
-462.499999999992));
#32643=CARTESIAN_POINT('Ctrl Pts',(58.8627320990774,-1.78994763186904,-462.499999999992));
#32644=CARTESIAN_POINT('Ctrl Pts',(58.7745669265647,-2.90096756015087,-462.499999999988));
#32645=CARTESIAN_POINT('Ctrl Pts',(58.8812368083505,-5.11842556204558,-462.499999999987));
#32646=CARTESIAN_POINT('Ctrl Pts',(59.0756383970967,-6.21585273547284,-462.499999999991));
#32647=CARTESIAN_POINT('Ctrl Pts',(59.4064050032652,-7.27543664706531,-462.499999999991));
#32648=CARTESIAN_POINT('',(59.4064050032676,-15.0625633529524,-462.499999999986));
#32649=CARTESIAN_POINT('Ctrl Pts',(59.4064050032652,-7.27543664706531,-462.499999999991));
#32650=CARTESIAN_POINT('Ctrl Pts',(59.7998586504781,-8.53583339440735,-462.499999999991));
#32651=CARTESIAN_POINT('Ctrl Pts',(60.0000000000047,-9.84861909545626,-462.499999999987));
#32652=CARTESIAN_POINT('Ctrl Pts',(59.9999999999965,-12.4893809046158,-462.499999999986));
#32653=CARTESIAN_POINT('Ctrl Pts',(59.7998586504701,-13.8021666056362,-462.49999999999));
#32654=CARTESIAN_POINT('Ctrl Pts',(59.4064050032657,-15.0625633529518,-462.49999999999));
#32655=CARTESIAN_POINT('',(59.0902650976022,-21.6344930467149,-462.499999999985));
#32656=CARTESIAN_POINT('Ctrl Pts',(59.4064050032657,-15.0625633529518,-462.49999999999));
#32657=CARTESIAN_POINT('Ctrl Pts',(59.0756383970974,-16.1221472645443,-462.49999999999));
#32658=CARTESIAN_POINT('Ctrl Pts',(58.8812368083515,-17.2195744379716,-462.499999999986));
#32659=CARTESIAN_POINT('Ctrl Pts',(58.7745669265659,-19.4370324398664,-462.499999999985));
#32660=CARTESIAN_POINT('Ctrl Pts',(58.8627320990786,-20.5480523681482,-462.499999999989));
#32661=CARTESIAN_POINT('Ctrl Pts',(59.0902650976002,-21.6344930467154,-462.499999999989));
#32662=CARTESIAN_POINT('Ctrl Pts',(59.0902650976002,-21.6344930467154,-462.499999999989));
#32663=CARTESIAN_POINT('Ctrl Pts',(59.3633429804669,-22.9384046652121,-462.499999999989));
#32664=CARTESIAN_POINT('Ctrl Pts',(59.4354076071443,-24.2764439932607,-462.499999999985));
#32665=CARTESIAN_POINT('Ctrl Pts',(59.1725049660245,-26.9278416595568,-462.499999999984));
#32666=CARTESIAN_POINT('Ctrl Pts',(58.8390772674808,-28.2256737474886,-462.499999999989));
#32667=CARTESIAN_POINT('Ctrl Pts',(58.3152526334998,-29.4505673778284,-462.499999999988));
#32668=CARTESIAN_POINT('Origin',(-89.9999999999107,-11.1690000000371,-462.499999999983));
#32669=CARTESIAN_POINT('Ctrl Pts',(53.0293871551332,-49.8739584350024,-462.499999999986));
#32670=CARTESIAN_POINT('Ctrl Pts',(53.9138954951112,-48.9022794410202,-462.499999999986));
#32671=CARTESIAN_POINT('Ctrl Pts',(54.6666325419227,-47.8185815867197,-462.500000000359));
#32672=CARTESIAN_POINT('Ctrl Pts',(55.8688443804717,-45.4847900735855,-462.50000000036));
#32673=CARTESIAN_POINT('Ctrl Pts',(56.3136127711626,-44.2453690239416,-462.499999999987));
#32674=CARTESIAN_POINT('Ctrl Pts',(56.5915605594671,-42.9638796623099,-462.499999999987));
#32675=CARTESIAN_POINT('Ctrl Pts',(31.7948796623067,-67.7605605594739,-462.499999999984));
#32676=CARTESIAN_POINT('Ctrl Pts',(33.0765842486482,-67.4825660901477,-462.499999999984));
#32677=CARTESIAN_POINT('Ctrl Pts',(34.3163262618311,-67.0376689797928,-462.500000000349));
#32678=CARTESIAN_POINT('Ctrl Pts',(36.650042374503,-65.8354478699916,-462.500000000349));
#32679=CARTESIAN_POINT('Ctrl Pts',(37.7336254438657,-65.082830891689,-462.499999999984));
#32680=CARTESIAN_POINT('Ctrl Pts',(38.7049734414089,-64.1983982826292,-462.499999999984));
#32681=CARTESIAN_POINT('',(25.9994431732944,-68.8985804999195,-462.499999999979));
#32682=CARTESIAN_POINT('Origin',(-5.05551156493311E-11,78.8310000002275,
-462.500000000346));
#32683=CARTESIAN_POINT('',(18.2815673778257,-69.4842526335121,-462.499999999979));
#32684=CARTESIAN_POINT('Ctrl Pts',(25.999443173295,-68.8985804999172,-462.499999999984));
#32685=CARTESIAN_POINT('Ctrl Pts',(24.7247935149947,-68.5695325308664,-462.499999999984));
#32686=CARTESIAN_POINT('Ctrl Pts',(23.4046510331284,-68.4524655597047,-462.499999999982));
#32687=CARTESIAN_POINT('Ctrl Pts',(20.779330128781,-68.6516884205231,-462.499999999982));
#32688=CARTESIAN_POINT('Ctrl Pts',(19.4919639499785,-68.9666276531229,-462.499999999983));
#32689=CARTESIAN_POINT('Ctrl Pts',(18.2815673778248,-69.4842526335099,-462.499999999983));
#32690=CARTESIAN_POINT('',(10.4654930467115,-70.2592650976135,-462.499999999979));
#32691=CARTESIAN_POINT('Ctrl Pts',(18.2815673778248,-69.4842526335099,-462.499999999983));
#32692=CARTESIAN_POINT('Ctrl Pts',(17.056673747458,-70.0080772675025,-462.499999999983));
#32693=CARTESIAN_POINT('Ctrl Pts',(15.7588416594962,-70.3415049660496,-462.499999999978));
#32694=CARTESIAN_POINT('Ctrl Pts',(13.1074439931985,-70.604407607152,-462.499999999978));
#32695=CARTESIAN_POINT('Ctrl Pts',(11.7694046651801,-70.5323429804717,-462.499999999983));
#32696=CARTESIAN_POINT('Ctrl Pts',(10.4654930467121,-70.2592650976111,-462.499999999983));
#32697=CARTESIAN_POINT('',(3.89356335294888,-70.5754050032799,-462.499999999978));
#32698=CARTESIAN_POINT('Ctrl Pts',(10.465493046712,-70.2592650976111,-462.499999999983));
#32699=CARTESIAN_POINT('Ctrl Pts',(9.37905236814473,-70.0317320990898,-462.499999999983));
#32700=CARTESIAN_POINT('Ctrl Pts',(8.26803243986281,-69.9435669265776,-462.499999999978));
#32701=CARTESIAN_POINT('Ctrl Pts',(6.05057443796808,-70.0502368083634,-462.499999999978));
#32702=CARTESIAN_POINT('Ctrl Pts',(4.95314726454063,-70.2446383971091,-462.499999999983));
#32703=CARTESIAN_POINT('Ctrl Pts',(3.89356335294815,-70.5754050032776,-462.499999999983));
#32704=CARTESIAN_POINT('',(-3.89356335293881,-70.5754050032805,-462.499999999978));
#32705=CARTESIAN_POINT('Ctrl Pts',(3.89356335294815,-70.5754050032776,-462.499999999983));
#32706=CARTESIAN_POINT('Ctrl Pts',(2.63316660560615,-70.9688586504905,-462.499999999983));
#32707=CARTESIAN_POINT('Ctrl Pts',(1.32038090455743,-71.1690000000175,-462.499999999978));
#32708=CARTESIAN_POINT('Ctrl Pts',(-1.32038090460214,-71.1690000000094,
-462.499999999978));
#32709=CARTESIAN_POINT('Ctrl Pts',(-2.63316660562244,-70.9688586504828,
-462.499999999983));
#32710=CARTESIAN_POINT('Ctrl Pts',(-3.89356335293808,-70.5754050032782,
-462.499999999983));
#32711=CARTESIAN_POINT('',(-10.4654930467012,-70.2592650976151,-462.499999999978));
#32712=CARTESIAN_POINT('Ctrl Pts',(-3.89356335293809,-70.5754050032782,
-462.499999999983));
#32713=CARTESIAN_POINT('Ctrl Pts',(-4.9531472645306,-70.24463839711,-462.499999999983));
#32714=CARTESIAN_POINT('Ctrl Pts',(-6.05057443795802,-70.0502368083644,
-462.499999999979));
#32715=CARTESIAN_POINT('Ctrl Pts',(-8.26803243985268,-69.9435669265789,
-462.499999999979));
#32716=CARTESIAN_POINT('Ctrl Pts',(-9.37905236813454,-70.0317320990914,
-462.499999999983));
#32717=CARTESIAN_POINT('Ctrl Pts',(-10.4654930467017,-70.2592650976128,
-462.499999999983));
#32718=CARTESIAN_POINT('',(-18.2815673778157,-69.4842526335148,-462.499999999978));
#32719=CARTESIAN_POINT('Ctrl Pts',(-10.4654930467017,-70.2592650976128,
-462.499999999983));
#32720=CARTESIAN_POINT('Ctrl Pts',(-11.7694046651997,-70.5323429804799,
-462.499999999983));
#32721=CARTESIAN_POINT('Ctrl Pts',(-13.1074439932496,-70.6044076071573,
-462.499999999978));
#32722=CARTESIAN_POINT('Ctrl Pts',(-15.7588416595456,-70.3415049660368,
-462.499999999978));
#32723=CARTESIAN_POINT('Ctrl Pts',(-17.0566737474761,-70.0080772674932,
-462.499999999983));
#32724=CARTESIAN_POINT('Ctrl Pts',(-18.2815673778148,-69.4842526335129,
-462.499999999983));
#32725=CARTESIAN_POINT('',(-25.9994431732854,-68.8985804999237,-462.499999999979));
#32726=CARTESIAN_POINT('Ctrl Pts',(-18.2815673778149,-69.4842526335129,
-462.499999999983));
#32727=CARTESIAN_POINT('Ctrl Pts',(-19.4919639499688,-68.966627653126,-462.499999999983));
#32728=CARTESIAN_POINT('Ctrl Pts',(-20.7793301287716,-68.6516884205264,
-462.499999999982));
#32729=CARTESIAN_POINT('Ctrl Pts',(-23.4046510331192,-68.4524655597085,
-462.499999999982));
#32730=CARTESIAN_POINT('Ctrl Pts',(-24.7247935149856,-68.5695325308705,
-462.499999999983));
#32731=CARTESIAN_POINT('Ctrl Pts',(-25.9994431732859,-68.8985804999215,
-462.499999999983));
#32732=CARTESIAN_POINT('',(-31.7948796622966,-67.7605605594826,-462.499999999979));
#32733=CARTESIAN_POINT('Origin',(-1.99706917669573E-11,78.8309999999131,
-462.500000001079));
#32734=CARTESIAN_POINT('Ctrl Pts',(-38.7057432251289,-64.1990916340934,
-462.499726017634));
#32735=CARTESIAN_POINT('Ctrl Pts',(-36.7423174004781,-65.9851579023194,
-462.499999999979));
#32736=CARTESIAN_POINT('Ctrl Pts',(-34.3848293251332,-67.1988151387573,
-462.499999999979));
#32737=CARTESIAN_POINT('Ctrl Pts',(-31.7948796622966,-67.7605605594826,
-462.499999999979));
#32738=CARTESIAN_POINT('',(-56.5915605594633,-42.9638796623205,-462.499999999981));
#32739=CARTESIAN_POINT('Ctrl Pts',(-56.5915605594633,-42.9638796623205,
-462.499999999981));
#32740=CARTESIAN_POINT('Ctrl Pts',(-56.029715455103,-45.5542889205284,-462.49999999998));
#32741=CARTESIAN_POINT('Ctrl Pts',(-54.8157369429699,-47.9121350536181,
-462.49999999998));
#32742=CARTESIAN_POINT('Ctrl Pts',(-53.0300791427081,-49.8747215894684,
-462.499718596329));
#32743=CARTESIAN_POINT('',(-57.7295804999055,-37.1684431733084,-462.499999999981));
#32744=CARTESIAN_POINT('Origin',(90.0000000000961,-11.1689999999847,-462.499999999614));
#32745=CARTESIAN_POINT('',(-58.315252633498,-29.4505673778391,-462.499999999982));
#32746=CARTESIAN_POINT('Ctrl Pts',(-57.7295804999029,-37.1684431733091,
-462.499999999986));
#32747=CARTESIAN_POINT('Ctrl Pts',(-57.4005325308522,-35.8937935150087,
-462.499999999986));
#32748=CARTESIAN_POINT('Ctrl Pts',(-57.2834655596905,-34.5736510331422,
-462.499999999985));
#32749=CARTESIAN_POINT('Ctrl Pts',(-57.4826884205089,-31.9483301287947,
-462.499999999986));
#32750=CARTESIAN_POINT('Ctrl Pts',(-57.7976276531085,-30.6609639499919,
-462.499999999987));
#32751=CARTESIAN_POINT('Ctrl Pts',(-58.3152526334954,-29.4505673778381,
-462.499999999987));
#32752=CARTESIAN_POINT('',(-59.0902650975996,-21.6344930467249,-462.499999999983));
#32753=CARTESIAN_POINT('Ctrl Pts',(-58.3152526334954,-29.4505673778381,
-462.499999999987));
#32754=CARTESIAN_POINT('Ctrl Pts',(-58.8390772674878,-28.2256737474723,
-462.499999999987));
#32755=CARTESIAN_POINT('Ctrl Pts',(-59.1725049660351,-26.9278416595116,
-462.499999999982));
#32756=CARTESIAN_POINT('Ctrl Pts',(-59.4354076071382,-24.2764439932139,
-462.499999999982));
#32757=CARTESIAN_POINT('Ctrl Pts',(-59.3633429804578,-22.9384046651945,
-462.499999999988));
#32758=CARTESIAN_POINT('Ctrl Pts',(-59.0902650975972,-21.6344930467255,
-462.499999999988));
#32759=CARTESIAN_POINT('',(-59.4064050032661,-15.0625633529624,-462.499999999984));
#32760=CARTESIAN_POINT('Ctrl Pts',(-59.0902650975972,-21.6344930467254,
-462.499999999988));
#32761=CARTESIAN_POINT('Ctrl Pts',(-58.8627320990759,-20.5480523681582,
-462.499999999988));
#32762=CARTESIAN_POINT('Ctrl Pts',(-58.7745669265638,-19.4370324398763,
-462.499999999983));
#32763=CARTESIAN_POINT('Ctrl Pts',(-58.8812368083496,-17.2195744379816,
-462.499999999984));
#32764=CARTESIAN_POINT('Ctrl Pts',(-59.0756383970952,-16.1221472645542,
-462.499999999989));
#32765=CARTESIAN_POINT('Ctrl Pts',(-59.4064050032639,-15.0625633529618,
-462.499999999989));
#32766=CARTESIAN_POINT('',(-59.4064050032667,-7.27543664707476,-462.499999999985));
#32767=CARTESIAN_POINT('Ctrl Pts',(-59.4064050032639,-15.0625633529618,
-462.499999999989));
#32768=CARTESIAN_POINT('Ctrl Pts',(-59.7998586504767,-13.8021666056197,
-462.499999999989));
#32769=CARTESIAN_POINT('Ctrl Pts',(-60.0000000000037,-12.489380904571,-462.499999999984));
#32770=CARTESIAN_POINT('Ctrl Pts',(-59.9999999999956,-9.84861909541142,
-462.499999999985));
#32771=CARTESIAN_POINT('Ctrl Pts',(-59.7998586504689,-8.53583339439112,
-462.49999999999));
#32772=CARTESIAN_POINT('Ctrl Pts',(-59.4064050032645,-7.27543664707546,
-462.49999999999));
#32773=CARTESIAN_POINT('',(-59.0902650976014,-0.703506953312267,-462.499999999986));
#32774=CARTESIAN_POINT('Ctrl Pts',(-59.4064050032645,-7.27543664707543,
-462.49999999999));
#32775=CARTESIAN_POINT('Ctrl Pts',(-59.0756383970961,-6.21585273548295,
-462.49999999999));
#32776=CARTESIAN_POINT('Ctrl Pts',(-58.8812368083507,-5.11842556205552,
-462.499999999985));
#32777=CARTESIAN_POINT('Ctrl Pts',(-58.7745669265651,-2.90096756016081,
-462.499999999985));
#32778=CARTESIAN_POINT('Ctrl Pts',(-58.8627320990773,-1.7899476318789,-462.49999999999));
#32779=CARTESIAN_POINT('Ctrl Pts',(-59.0902650975988,-0.703506953311725,
-462.49999999999));
#32780=CARTESIAN_POINT('',(-58.3152526335012,7.11256737780218,-462.499999999987));
#32781=CARTESIAN_POINT('Ctrl Pts',(-59.0902650975988,-0.703506953311577,
-462.49999999999));
#32782=CARTESIAN_POINT('Ctrl Pts',(-59.3633429804661,0.600404665187346,
-462.499999999991));
#32783=CARTESIAN_POINT('Ctrl Pts',(-59.4354076071438,1.93844399323813,-462.499999999986));
#32784=CARTESIAN_POINT('Ctrl Pts',(-59.1725049660226,4.58984165953402,-462.499999999986));
#32785=CARTESIAN_POINT('Ctrl Pts',(-58.8390772674787,5.88767374746334,-462.499999999991));
#32786=CARTESIAN_POINT('Ctrl Pts',(-58.3152526334986,7.11256737780097,-462.499999999991));
#32787=CARTESIAN_POINT('',(-57.7295804999101,14.8304431732717,-462.499999999987));
#32788=CARTESIAN_POINT('Ctrl Pts',(-58.3152526334985,7.11256737780111,-462.499999999991));
#32789=CARTESIAN_POINT('Ctrl Pts',(-57.7976276531118,8.32296394995511,-462.499999999991));
#32790=CARTESIAN_POINT('Ctrl Pts',(-57.4826884205125,9.61033012875785,-462.499999999991));
#32791=CARTESIAN_POINT('Ctrl Pts',(-57.2834655596947,12.2356510331055,-462.499999999991));
#32792=CARTESIAN_POINT('Ctrl Pts',(-57.4005325308566,13.555793514972,-462.499999999992));
#32793=CARTESIAN_POINT('Ctrl Pts',(-57.7295804999076,14.8304431732723,-462.499999999992));
#32794=CARTESIAN_POINT('',(-56.5915605594688,20.6258796622837,-462.499999999988));
#32795=CARTESIAN_POINT('Origin',(90.0000000001139,-11.1690000000374,-462.499999998157));
#32796=CARTESIAN_POINT('Ctrl Pts',(-53.0305574330451,27.5375500128045,-462.499999999994));
#32797=CARTESIAN_POINT('Ctrl Pts',(-53.9136598402457,26.5661625983044,-462.499999999994));
#32798=CARTESIAN_POINT('Ctrl Pts',(-54.6654949545811,25.4831869345778,-462.500000000018));
#32799=CARTESIAN_POINT('Ctrl Pts',(-55.867938981057,23.1493254197733,-462.500000000018));
#32800=CARTESIAN_POINT('Ctrl Pts',(-56.3133319485292,21.9086637678552,-462.499999999993));
#32801=CARTESIAN_POINT('Ctrl Pts',(-56.5915605594654,20.625879662283,-462.499999999993));
#32802=CARTESIAN_POINT('',(-31.7948796623065,45.4225605594505,-462.499999999992));
#32803=CARTESIAN_POINT('Ctrl Pts',(-38.7066184322078,41.8615969349749,-462.499999999991));
#32804=CARTESIAN_POINT('Ctrl Pts',(-38.3840553815676,42.1548781377002,-462.499999999991));
#32805=CARTESIAN_POINT('Ctrl Pts',(-38.0485358858946,42.4342626183073,-462.49999999999));
#32806=CARTESIAN_POINT('Ctrl Pts',(-37.7015139289768,42.6984598857191,-462.499999999992));
#32807=CARTESIAN_POINT('Ctrl Pts',(-37.6313113290433,42.751907037111,-462.499999999992));
#32808=CARTESIAN_POINT('Ctrl Pts',(-37.5606381983877,42.8047320086185,-462.499999999992));
#32809=CARTESIAN_POINT('Ctrl Pts',(-37.4895054223497,42.8569273733703,-462.499999999992));
#32810=CARTESIAN_POINT('Ctrl Pts',(-37.2083128059277,43.0632591376727,-462.499999999992));
#32811=CARTESIAN_POINT('Ctrl Pts',(-36.9199317767795,43.2597666774808,-462.499999999992));
#32812=CARTESIAN_POINT('Ctrl Pts',(-36.6250350054762,43.44599737661,-462.499999999992));
#32813=CARTESIAN_POINT('Ctrl Pts',(-36.4766084300011,43.5397304642866,-462.499999999992));
#32814=CARTESIAN_POINT('Ctrl Pts',(-36.3265298420472,43.6308599885747,-462.499999999992));
#32815=CARTESIAN_POINT('Ctrl Pts',(-36.1748926818072,43.719331120904,-462.499999999992));
#32816=CARTESIAN_POINT('Ctrl Pts',(-35.9475629882934,43.8519642786695,-462.499999999992));
#32817=CARTESIAN_POINT('Ctrl Pts',(-35.7167344653798,43.9786237267065,-462.499999999992));
#32818=CARTESIAN_POINT('Ctrl Pts',(-35.4827207341128,44.0991249603451,-462.499999999992));
#32819=CARTESIAN_POINT('Ctrl Pts',(-35.0926443215359,44.2999879125929,-462.499999999992));
#32820=CARTESIAN_POINT('Ctrl Pts',(-34.6937162549713,44.4837348679316,-462.499999999992));
#32821=CARTESIAN_POINT('Ctrl Pts',(-34.2872595209354,44.6497527723323,-462.499999999992));
#32822=CARTESIAN_POINT('Ctrl Pts',(-34.2870189837742,44.6498510128264,-462.499999999991));
#32823=CARTESIAN_POINT('Ctrl Pts',(-33.882499227078,44.8150532196688,-462.499999999992));
#32824=CARTESIAN_POINT('Ctrl Pts',(-33.4710017122312,44.9624982997247,-462.499999999992));
#32825=CARTESIAN_POINT('Ctrl Pts',(-33.0533836161765,45.091854154172,-462.499999999992));
#32826=CARTESIAN_POINT('Ctrl Pts',(-33.0529806979711,45.0919789381448,-462.499999999992));
#32827=CARTESIAN_POINT('Ctrl Pts',(-32.6383541991618,45.2203697961812,-462.499999999991));
#32828=CARTESIAN_POINT('Ctrl Pts',(-32.2184964333868,45.3306825375905,-462.499999999992));
#32829=CARTESIAN_POINT('Ctrl Pts',(-31.7948796623065,45.4225605594505,-462.499999999992));
#32830=CARTESIAN_POINT('',(-18.8785077902573,47.6382644181355,-462.499999999992));
#32831=CARTESIAN_POINT('Origin',(1.8061108164602E-11,-101.169000000086,
-462.499999999992));
#32832=CARTESIAN_POINT('',(-12.0150531445829,47.9060664143362,-462.499999999992));
#32833=CARTESIAN_POINT('Ctrl Pts',(-18.8785077902579,47.638264418134,-462.499999999996));
#32834=CARTESIAN_POINT('Ctrl Pts',(-18.5525168649589,47.5094378392464,-462.499999999996));
#32835=CARTESIAN_POINT('Ctrl Pts',(-17.4086215538667,47.057388076463,-462.499999999996));
#32836=CARTESIAN_POINT('Ctrl Pts',(-15.1447493101886,47.0351751898152,-462.499999999996));
#32837=CARTESIAN_POINT('Ctrl Pts',(-14.4547291834694,47.1123036398729,-462.499999999996));
#32838=CARTESIAN_POINT('Ctrl Pts',(-12.9164507181125,47.4785763558462,-462.499999999996));
#32839=CARTESIAN_POINT('Ctrl Pts',(-12.4871383760148,47.6751419616563,-462.499999999997));
#32840=CARTESIAN_POINT('Ctrl Pts',(-12.0150531445812,47.9060664143328,-462.499999999997));
#32841=CARTESIAN_POINT('',(-7.17826498482574,48.1389160151703,-462.499999999992));
#32842=CARTESIAN_POINT('Ctrl Pts',(-12.0150531445813,47.9060664143328,-462.499999999997));
#32843=CARTESIAN_POINT('Ctrl Pts',(-11.8254498398673,47.9988124619773,-462.499999999997));
#32844=CARTESIAN_POINT('Ctrl Pts',(-11.2182438109275,48.2958323869455,-462.499999999998));
#32845=CARTESIAN_POINT('Ctrl Pts',(-9.75062554367071,48.5431074753305,-462.499999999998));
#32846=CARTESIAN_POINT('Ctrl Pts',(-9.15039604630952,48.55483428605,-462.499999999998));
#32847=CARTESIAN_POINT('Ctrl Pts',(-7.88961170229352,48.3954373452753,-462.499999999998));
#32848=CARTESIAN_POINT('Ctrl Pts',(-7.55090612168781,48.2786384356784,-462.499999999997));
#32849=CARTESIAN_POINT('Ctrl Pts',(-7.17826498481883,48.1389160151649,-462.499999999997));
#32850=CARTESIAN_POINT('',(-2.51503960160435,48.2902113213028,-462.499999999992));
#32851=CARTESIAN_POINT('Ctrl Pts',(-7.17826498482668,48.1389160151678,-462.499999999997));
#32852=CARTESIAN_POINT('Ctrl Pts',(-6.93633745397943,48.0482048809024,-462.499999999997));
#32853=CARTESIAN_POINT('Ctrl Pts',(-6.04322837503661,47.7133321303008,-462.499999999995));
#32854=CARTESIAN_POINT('Ctrl Pts',(-3.62010262056583,47.7919488650083,-462.499999999995));
#32855=CARTESIAN_POINT('Ctrl Pts',(-2.75057840885255,48.1840091023979,-462.499999999997));
#32856=CARTESIAN_POINT('Ctrl Pts',(-2.51503960160297,48.2902113212998,-462.499999999997));
#32857=CARTESIAN_POINT('',(2.51503960159695,48.2902113215691,-462.499999999685));
#32858=CARTESIAN_POINT('Ctrl Pts',(-2.51503960160305,48.2902113212997,-462.499999999997));
#32859=CARTESIAN_POINT('Ctrl Pts',(-2.31486538455667,48.3804679811915,-462.499999999997));
#32860=CARTESIAN_POINT('Ctrl Pts',(-1.67033819224985,48.6710791924356,-462.5));
#32861=CARTESIAN_POINT('Ctrl Pts',(-0.126674917807384,48.8617608677135,
-462.5));
#32862=CARTESIAN_POINT('Ctrl Pts',(0.500972562625843,48.8421778966588,-462.5));
#32863=CARTESIAN_POINT('Ctrl Pts',(1.79880408278553,48.6019577853086,-462.5));
#32864=CARTESIAN_POINT('Ctrl Pts',(2.14046119294517,48.4591051805071,-462.499999999997));
#32865=CARTESIAN_POINT('Ctrl Pts',(2.51503960150293,48.290211321341,-462.499999999997));
#32866=CARTESIAN_POINT('',(7.17826498479954,48.1389160151653,-462.499999999992));
#32867=CARTESIAN_POINT('Ctrl Pts',(2.5150396014956,48.2902113213443,-462.499999999997));
#32868=CARTESIAN_POINT('Ctrl Pts',(3.01635259829434,48.0641740358177,-462.499999999997));
#32869=CARTESIAN_POINT('Ctrl Pts',(3.81474900505418,47.785633690015,-462.499999999995));
#32870=CARTESIAN_POINT('Ctrl Pts',(6.04322837400998,47.7133321303346,-462.499999999995));
#32871=CARTESIAN_POINT('Ctrl Pts',(6.93633745247155,48.0482048803425,-462.499999999997));
#32872=CARTESIAN_POINT('Ctrl Pts',(7.17826498480051,48.1389160151627,-462.499999999997));
#32873=CARTESIAN_POINT('Ctrl Pts',(7.17826498479326,48.13891601516,-462.499999999997));
#32874=CARTESIAN_POINT('Ctrl Pts',(7.57867402073054,48.289050056096,-462.499999999997));
#32875=CARTESIAN_POINT('Ctrl Pts',(7.94324496867089,48.4139972953879,-462.500000000092));
#32876=CARTESIAN_POINT('Ctrl Pts',(9.18080504777323,48.548614052163,-462.500000000092));
#32877=CARTESIAN_POINT('Ctrl Pts',(9.70223236095501,48.5392006175157,-462.500000000092));
#32878=CARTESIAN_POINT('Ctrl Pts',(11.0123813546909,48.3457034074005,-462.500000000092));
#32879=CARTESIAN_POINT('Ctrl Pts',(11.6260991509692,48.0963265243883,-462.499999999997));
#32880=CARTESIAN_POINT('Ctrl Pts',(12.0150531445265,47.9060664143568,-462.499999999997));
#32881=CARTESIAN_POINT('Origin',(3.88578058618805E-13,-3.17499999995531,
41.5000000000138));
#32882=CARTESIAN_POINT('Origin',(35.6399999999924,86.8310000000046,-333.499999999996));
#32883=CARTESIAN_POINT('Origin',(35.6399999999924,86.831,-377.5));
#32884=CARTESIAN_POINT('Origin',(47.999999999991,104.331000000009,-307.5));
#32885=CARTESIAN_POINT('',(47.999999999991,104.331000000009,-300.5));
#32886=CARTESIAN_POINT('',(54.999999999991,104.331000000009,-307.5));
#32887=CARTESIAN_POINT('Origin',(47.999999999991,104.331000000009,-307.5));
#32888=CARTESIAN_POINT('',(54.999999999991,104.331000000009,-307.5));
#32889=CARTESIAN_POINT('',(47.999999999991,104.331000000009,-300.5));
#32890=CARTESIAN_POINT('Origin',(54.999999999991,104.331000000004,-355.5));
#32891=CARTESIAN_POINT('',(54.999999999991,104.330999999998,-403.5));
#32892=CARTESIAN_POINT('',(54.999999999991,104.331000000004,-355.5));
#32893=CARTESIAN_POINT('',(54.999999999991,104.330999999998,-403.5));
#32894=CARTESIAN_POINT('Origin',(47.999999999991,104.330999999998,-403.5));
#32895=CARTESIAN_POINT('',(47.999999999991,104.330999999997,-410.5));
#32896=CARTESIAN_POINT('Origin',(47.999999999991,104.330999999998,-403.5));
#32897=CARTESIAN_POINT('',(47.999999999991,104.330999999997,-410.5));
#32898=CARTESIAN_POINT('Origin',(-1.500000000009,104.330999999992,-410.5));
#32899=CARTESIAN_POINT('',(-51.000000000009,104.330999999988,-410.5));
#32900=CARTESIAN_POINT('',(-1.50000000000897,104.330999999992,-410.5));
#32901=CARTESIAN_POINT('',(-51.000000000009,104.330999999988,-410.5));
#32902=CARTESIAN_POINT('Origin',(-51.000000000009,104.330999999989,-403.5));
#32903=CARTESIAN_POINT('',(-58.000000000009,104.330999999988,-403.5));
#32904=CARTESIAN_POINT('Origin',(-51.000000000009,104.330999999989,-403.5));
#32905=CARTESIAN_POINT('',(-58.000000000009,104.330999999988,-403.5));
#32906=CARTESIAN_POINT('Origin',(-58.000000000009,104.330999999994,-355.5));
#32907=CARTESIAN_POINT('',(-58.000000000009,104.331,-307.5));
#32908=CARTESIAN_POINT('',(-58.000000000009,104.330999999994,-355.5));
#32909=CARTESIAN_POINT('',(-58.000000000009,104.331,-307.5));
#32910=CARTESIAN_POINT('Origin',(-51.000000000009,104.331,-307.5));
#32911=CARTESIAN_POINT('',(-51.000000000009,104.331,-300.5));
#32912=CARTESIAN_POINT('Origin',(-51.000000000009,104.331,-307.5));
#32913=CARTESIAN_POINT('',(-51.000000000009,104.331,-300.5));
#32914=CARTESIAN_POINT('Origin',(-26.250000000009,104.331000000003,-300.5));
#32915=CARTESIAN_POINT('',(-1.50000000000897,104.331000000005,-300.5));
#32916=CARTESIAN_POINT('Ctrl Pts',(-64.2657293397397,-67.9791674266158,
-441.000046512357));
#32917=CARTESIAN_POINT('Ctrl Pts',(-52.7947107433608,-50.1279378633292,
-462.499360694393));
#32918=CARTESIAN_POINT('Ctrl Pts',(-67.6327997693264,-64.1661639590615,
-440.999999999978));
#32919=CARTESIAN_POINT('Ctrl Pts',(-54.7064708585543,-48.1213181445082,
-462.49999999998));
#32920=CARTESIAN_POINT('Ctrl Pts',(-69.5425906597941,-59.4517471898053,
-440.999999999979));
#32921=CARTESIAN_POINT('Ctrl Pts',(-56.0041009291202,-45.6723857139965,
-462.49999999998));
#32922=CARTESIAN_POINT('Ctrl Pts',(-69.7777140088065,-54.3725409130246,
-441.000032808645));
#32923=CARTESIAN_POINT('Ctrl Pts',(-56.5915605594633,-42.9638796623204,
-462.499999999981));
#32924=CARTESIAN_POINT('',(-64.2657293397398,-67.9791674266157,-441.000046512357));
#32925=CARTESIAN_POINT('',(-56.5915605594633,-42.9638796623205,-462.499999999981));
#32926=CARTESIAN_POINT('Ctrl Pts',(-56.8068436844474,-75.458414074715,-440.983703173492));
#32927=CARTESIAN_POINT('Ctrl Pts',(-56.7932797691753,-75.4496884498354,
-441.000046956267));
#32928=CARTESIAN_POINT('Ctrl Pts',(-44.7294130526197,-67.6890459439958,
-455.536347976562));
#32929=CARTESIAN_POINT('Ctrl Pts',(-44.7287959283668,-67.6886489496926,
-455.537091577965));
#32930=CARTESIAN_POINT('Ctrl Pts',(-56.8085894473236,-75.4568691036499,
-440.983703130936));
#32931=CARTESIAN_POINT('Ctrl Pts',(-56.79502657148,-75.4481423853249,-441.000046925264));
#32932=CARTESIAN_POINT('Ctrl Pts',(-44.7320913356736,-67.6865299469002,
-455.536351294835));
#32933=CARTESIAN_POINT('Ctrl Pts',(-44.7314742592658,-67.6861329032623,
-455.537094896055));
#32934=CARTESIAN_POINT('Ctrl Pts',(-56.8103352101999,-75.4553241325848,
-440.98370308838));
#32935=CARTESIAN_POINT('Ctrl Pts',(-56.7967733737847,-75.4465963208143,
-441.000046894262));
#32936=CARTESIAN_POINT('Ctrl Pts',(-44.7347696187276,-67.6840139498046,
-455.536354613108));
#32937=CARTESIAN_POINT('Ctrl Pts',(-44.7341525901647,-67.6836168568319,
-455.537098214144));
#32938=CARTESIAN_POINT('Ctrl Pts',(-56.8120809730762,-75.4537791615197,
-440.983703045824));
#32939=CARTESIAN_POINT('Ctrl Pts',(-56.7985201760894,-75.4450502563038,
-441.000046863259));
#32940=CARTESIAN_POINT('Ctrl Pts',(-44.7374479017815,-67.681497952709,-455.53635793138));
#32941=CARTESIAN_POINT('Ctrl Pts',(-44.7368309210637,-67.6811008104016,
-455.537101532234));
#32942=CARTESIAN_POINT('Ctrl Pts',(-59.4509723336889,-73.11840426527,-440.983638717812));
#32943=CARTESIAN_POINT('Ctrl Pts',(-59.4389827344453,-73.1080225102961,
-440.999999999977));
#32944=CARTESIAN_POINT('Ctrl Pts',(-48.7830207157301,-63.8810596701001,
-455.541370214754));
#32945=CARTESIAN_POINT('Ctrl Pts',(-48.7824760053808,-63.8805880071809,
-455.542113538993));
#32946=CARTESIAN_POINT('Ctrl Pts',(-61.940843357604,-70.6288920335432,-440.983638717812));
#32947=CARTESIAN_POINT('Ctrl Pts',(-61.9304681124401,-70.6168956516598,
-440.999999999977));
#32948=CARTESIAN_POINT('Ctrl Pts',(-52.7092909776335,-59.9549054455687,
-455.541370214755));
#32949=CARTESIAN_POINT('Ctrl Pts',(-52.7088196104674,-59.9543604270711,
-455.542113538993));
#32950=CARTESIAN_POINT('Ctrl Pts',(-64.2744496288301,-67.9927379636265,
-440.983702694819));
#32951=CARTESIAN_POINT('Ctrl Pts',(-64.2657293397397,-67.9791674266158,
-441.000046512357));
#32952=CARTESIAN_POINT('Ctrl Pts',(-56.5098402813215,-55.9094323036241,
-455.536357671384));
#32953=CARTESIAN_POINT('Ctrl Pts',(-56.5094435310252,-55.9088148797607,
-455.537101272242));
#32954=CARTESIAN_POINT('Ctrl Pts',(-64.2759934183429,-67.990994024618,-440.983702737144));
#32955=CARTESIAN_POINT('Ctrl Pts',(-64.267274224083,-67.9774224462302,-441.000046543128));
#32956=CARTESIAN_POINT('Ctrl Pts',(-56.512356333148,-55.9067541065334,-455.536354352964));
#32957=CARTESIAN_POINT('Ctrl Pts',(-56.5119596322498,-55.906136634736,-455.537097954005));
#32958=CARTESIAN_POINT('Ctrl Pts',(-64.2775372078555,-67.9892500856095,
-440.983702779468));
#32959=CARTESIAN_POINT('Ctrl Pts',(-64.2688191084264,-67.9756774658445,
-441.000046573897));
#32960=CARTESIAN_POINT('Ctrl Pts',(-56.5148723849746,-55.9040759094427,
-455.536351034544));
#32961=CARTESIAN_POINT('Ctrl Pts',(-56.5144757334745,-55.9034583897113,
-455.537094635768));
#32962=CARTESIAN_POINT('Ctrl Pts',(-64.2790809973682,-67.987506146601,-440.983702821791));
#32963=CARTESIAN_POINT('Ctrl Pts',(-64.2703639927698,-67.9739324854589,
-441.000046604668));
#32964=CARTESIAN_POINT('Ctrl Pts',(-56.5173884368011,-55.9013977123521,
-455.536347716124));
#32965=CARTESIAN_POINT('Ctrl Pts',(-56.5169918346991,-55.9007801446866,
-455.537091317531));
#32966=CARTESIAN_POINT('',(-56.7985201761028,-75.4450502562919,-441.000046863259));
#32967=CARTESIAN_POINT('Ctrl Pts',(-64.2657293397398,-67.9791674266157,
-441.000046512357));
#32968=CARTESIAN_POINT('Ctrl Pts',(-64.2379686007189,-68.0105725380733,
-441.000011935885));
#32969=CARTESIAN_POINT('Ctrl Pts',(-64.2006833472475,-68.0527069711186,
-440.999965951545));
#32970=CARTESIAN_POINT('Ctrl Pts',(-64.1198226715104,-68.1438289318397,
-440.999868753421));
#32971=CARTESIAN_POINT('Ctrl Pts',(-64.0832738799935,-68.1849360569023,
-440.999825609413));
#32972=CARTESIAN_POINT('Ctrl Pts',(-63.9735042890578,-68.3081570525,-440.999698381965));
#32973=CARTESIAN_POINT('Ctrl Pts',(-63.9001649872347,-68.3901652114701,
-440.99961650872));
#32974=CARTESIAN_POINT('Ctrl Pts',(-63.6796564581205,-68.6357853866767,
-440.999379598168));
#32975=CARTESIAN_POINT('Ctrl Pts',(-63.5320150171305,-68.7989722880318,
-440.999233289074));
#32976=CARTESIAN_POINT('Ctrl Pts',(-63.0871465110819,-69.2868934672009,
-440.998828453101));
#32977=CARTESIAN_POINT('Ctrl Pts',(-62.7880452046029,-69.6099093149823,
-440.99860404548));
#32978=CARTESIAN_POINT('Ctrl Pts',(-61.8831162212809,-70.5722204933488,
-440.998063183776));
#32979=CARTESIAN_POINT('Ctrl Pts',(-61.2699123367798,-71.2045014479794,
-440.997878501315));
#32980=CARTESIAN_POINT('Ctrl Pts',(-60.0244121795718,-72.4497779568237,
-440.997860569593));
#32981=CARTESIAN_POINT('Ctrl Pts',(-59.3921928542818,-73.0627068426545,
-440.998027192544));
#32982=CARTESIAN_POINT('Ctrl Pts',(-58.429873872212,-73.9673320492948,-440.998561014861));
#32983=CARTESIAN_POINT('Ctrl Pts',(-58.1067820084529,-74.2664003494679,
-440.998786485406));
#32984=CARTESIAN_POINT('Ctrl Pts',(-57.6187183951671,-74.7112440254951,
-440.999200642983));
#32985=CARTESIAN_POINT('Ctrl Pts',(-57.4554648297677,-74.8588940789512,
-440.999351364043));
#32986=CARTESIAN_POINT('Ctrl Pts',(-57.2097371052446,-75.0794213981712,
-440.999597178664));
#32987=CARTESIAN_POINT('Ctrl Pts',(-57.1276881746811,-75.1527711803181,
-440.99968240501));
#32988=CARTESIAN_POINT('Ctrl Pts',(-57.0044040747093,-75.2625579230306,
-440.999815278954));
#32989=CARTESIAN_POINT('Ctrl Pts',(-56.9632746672463,-75.2991134864768,
-440.999860408936));
#32990=CARTESIAN_POINT('Ctrl Pts',(-56.8721271094273,-75.3799679631664,
-440.999962214462));
#32991=CARTESIAN_POINT('Ctrl Pts',(-56.8299684290529,-75.4172613726013,
-441.000010497298));
#32992=CARTESIAN_POINT('Ctrl Pts',(-56.7985201761028,-75.4450502562919,
-441.000046863259));
#32993=CARTESIAN_POINT('Ctrl Pts',(-43.1946805031653,-80.9544448157854,
-441.000060157993));
#32994=CARTESIAN_POINT('Ctrl Pts',(-31.7948796622966,-67.7605605594826,
-462.499999999979));
#32995=CARTESIAN_POINT('Ctrl Pts',(-48.2746526175946,-80.7177558649757,
-440.999999999976));
#32996=CARTESIAN_POINT('Ctrl Pts',(-34.5033857139727,-67.17310092914,-462.499999999979));
#32997=CARTESIAN_POINT('Ctrl Pts',(-52.9882277635993,-78.8087212294075,
-440.999999999977));
#32998=CARTESIAN_POINT('Ctrl Pts',(-36.9523181444846,-65.8754708585745,
-462.499999999979));
#32999=CARTESIAN_POINT('Ctrl Pts',(-56.7985201760894,-75.4450502563038,
-441.000046863259));
#33000=CARTESIAN_POINT('Ctrl Pts',(-38.9600894847066,-63.9626889424092,
-462.499377237841));
#33001=CARTESIAN_POINT('',(-43.1946805031654,-80.9544448157855,-441.000060157993));
#33002=CARTESIAN_POINT('Ctrl Pts',(-30.0724252391789,-81.4699528747219,
-440.991833214076));
#33003=CARTESIAN_POINT('Ctrl Pts',(-30.0694361726661,-81.4653775066517,
-441.00006022933));
#33004=CARTESIAN_POINT('Ctrl Pts',(-22.2580066308467,-69.5084119606299,
-462.499999999978));
#33005=CARTESIAN_POINT('Ctrl Pts',(-22.2501512995082,-69.4963877945455,
-462.521620773711));
#33006=CARTESIAN_POINT('Ctrl Pts',(-34.4491834215995,-81.3268370384189,
-440.991760309822));
#33007=CARTESIAN_POINT('Ctrl Pts',(-34.4457390924923,-81.3221254984248,
-440.999999999977));
#33008=CARTESIAN_POINT('Ctrl Pts',(-25.4583773817378,-69.0282032793835,
-462.499999999979));
#33009=CARTESIAN_POINT('Ctrl Pts',(-25.4493533867006,-69.0158592459884,
-462.521587635987));
#33010=CARTESIAN_POINT('Ctrl Pts',(-38.8247825005319,-81.1566899975232,
-440.991744896788));
#33011=CARTESIAN_POINT('Ctrl Pts',(-38.8208728590296,-81.1518111816476,
-440.999999999977));
#33012=CARTESIAN_POINT('Ctrl Pts',(-28.6384087051628,-68.4451812419869,
-462.499999999979));
#33013=CARTESIAN_POINT('Ctrl Pts',(-28.628203825419,-68.4324466397802,-462.521547329895));
#33014=CARTESIAN_POINT('Ctrl Pts',(-43.1990671867739,-80.959521869026,-440.99178690524));
#33015=CARTESIAN_POINT('Ctrl Pts',(-43.1946805031653,-80.9544448157854,
-441.000060157993));
#33016=CARTESIAN_POINT('Ctrl Pts',(-31.7948796622966,-67.7605605594826,
-462.499999999979));
#33017=CARTESIAN_POINT('Ctrl Pts',(-31.7834798614557,-67.7473666752263,
-462.521499939821));
#33018=CARTESIAN_POINT('',(-30.0769139794115,-81.465138787044,-441.000049420363));
#33019=CARTESIAN_POINT('Ctrl Pts',(-25.9994431732858,-68.8985804999237,
-462.499999999979));
#33020=CARTESIAN_POINT('Ctrl Pts',(-26.7964799308327,-70.6751920159385,
-459.557188447894));
#33021=CARTESIAN_POINT('Ctrl Pts',(-27.479108889254,-72.495769348422,-456.514213204788));
#33022=CARTESIAN_POINT('Ctrl Pts',(-28.4752491269335,-75.495938283277,-451.414006370867));
#33023=CARTESIAN_POINT('Ctrl Pts',(-28.8452960300499,-76.7249502701369,
-449.301561414758));
#33024=CARTESIAN_POINT('Ctrl Pts',(-29.5081306533979,-79.1196286730972,
-445.139987269977));
#33025=CARTESIAN_POINT('Ctrl Pts',(-29.8061604421476,-80.2987054845064,
-443.068993354753));
#33026=CARTESIAN_POINT('Ctrl Pts',(-30.0769139781574,-81.4651387869444,
-441.000049420142));
#33027=CARTESIAN_POINT('Ctrl Pts',(-43.1946805031653,-80.9544448157855,
-441.000060157993));
#33028=CARTESIAN_POINT('Ctrl Pts',(-40.9465691514988,-81.0577146082457,
-440.997167465374));
#33029=CARTESIAN_POINT('Ctrl Pts',(-38.6981106838266,-81.1529027064473,
-440.995568194053));
#33030=CARTESIAN_POINT('Ctrl Pts',(-34.3253844906309,-81.3222673217518,
-440.995559720608));
#33031=CARTESIAN_POINT('Ctrl Pts',(-32.2013690465366,-81.3973097918519,
-440.99698028376));
#33032=CARTESIAN_POINT('Ctrl Pts',(-30.076913979416,-81.465138787221,-441.000049419583));
#33033=CARTESIAN_POINT('Origin',(5.02375918642883E-12,-65.4426315587606,
-438.999999999979));
#33034=CARTESIAN_POINT('',(-25.7039045353314,-81.6296264484025,-438.999999999976));
#33035=CARTESIAN_POINT('',(-23.5144780620957,-81.6868555254876,-438.999999999977));
#33036=CARTESIAN_POINT('Origin',(0.000161522130812664,859.827648708006,
-438.999999684644));
#33037=CARTESIAN_POINT('Ctrl Pts',(-25.7039045353315,-81.6296264484023,
-438.999999999977));
#33038=CARTESIAN_POINT('Ctrl Pts',(-25.338907423015,-81.6125050746809,-438.999999999977));
#33039=CARTESIAN_POINT('Ctrl Pts',(-24.9734197856892,-81.608705495081,-438.999999999974));
#33040=CARTESIAN_POINT('Ctrl Pts',(-24.2428714081309,-81.6277925001813,
-438.999999999974));
#33041=CARTESIAN_POINT('Ctrl Pts',(-23.8780813890794,-81.6506720610301,
-438.999999999977));
#33042=CARTESIAN_POINT('Ctrl Pts',(-23.5144780620957,-81.6868555254874,
-438.999999999977));
#33043=CARTESIAN_POINT('Ctrl Pts',(-18.2815673778157,-69.4842526335149,
-462.499999999979));
#33044=CARTESIAN_POINT('Ctrl Pts',(-20.9895259839786,-82.1584973191859,
-439.001498361858));
#33045=CARTESIAN_POINT('Ctrl Pts',(-20.8066529721932,-68.4044021024295,
-462.499999999979));
#33046=CARTESIAN_POINT('Ctrl Pts',(-24.0993037835529,-81.2970472206573,
-438.998064517714));
#33047=CARTESIAN_POINT('Ctrl Pts',(-23.6668225473958,-68.1714685993807,
-462.499999999979));
#33048=CARTESIAN_POINT('Ctrl Pts',(-27.4436430653255,-81.41563992135,-439.00145091813));
#33049=CARTESIAN_POINT('Ctrl Pts',(-26.5149982528597,-69.0440180664332,
-462.499999999978));
#33050=CARTESIAN_POINT('Ctrl Pts',(-30.6502301549084,-82.7145147968836,
-438.999999999977));
#33051=CARTESIAN_POINT('Ctrl Pts',(-30.0769139793183,-81.4651387872084,
-441.000049420484));
#33052=CARTESIAN_POINT('Ctrl Pts',(-29.551680891548,-81.4895072998655,-440.565682691273));
#33053=CARTESIAN_POINT('Ctrl Pts',(-28.9861515269315,-81.513823687901,-440.18289056592));
#33054=CARTESIAN_POINT('Ctrl Pts',(-27.540804130675,-81.5705690446153,-439.428837284769));
#33055=CARTESIAN_POINT('Ctrl Pts',(-26.6435506045776,-81.6016843613183,
-439.131000321948));
#33056=CARTESIAN_POINT('Ctrl Pts',(-25.7039045353331,-81.6296264484023,
-438.999999999977));
#33057=CARTESIAN_POINT('',(-20.8989998873753,-81.7348018106293,-439.787044944617));
#33058=CARTESIAN_POINT('',(-18.2815673778157,-69.4842526335148,-462.499999999978));
#33059=CARTESIAN_POINT('Ctrl Pts',(-23.5144780620922,-81.6868555254877,
-438.999999999977));
#33060=CARTESIAN_POINT('Ctrl Pts',(-23.0030694413233,-81.6984039047958,
-439.070113764198));
#33061=CARTESIAN_POINT('Ctrl Pts',(-22.5005158148452,-81.7084840649418,
-439.187699311006));
#33062=CARTESIAN_POINT('Ctrl Pts',(-21.6305049523498,-81.7238853085043,
-439.470420490408));
#33063=CARTESIAN_POINT('Ctrl Pts',(-21.2600040239069,-81.729739132405,-439.618066172395));
#33064=CARTESIAN_POINT('Ctrl Pts',(-20.8989998873755,-81.7348018106293,
-439.787044944617));
#33065=CARTESIAN_POINT('Ctrl Pts',(-10.4654930467012,-70.2592650976151,
-462.499999999978));
#33066=CARTESIAN_POINT('Ctrl Pts',(-12.3200202973713,-81.9438009571564,
-439.788405446002));
#33067=CARTESIAN_POINT('Ctrl Pts',(-13.1095347614995,-70.8130060900615,
-462.499999999978));
#33068=CARTESIAN_POINT('Ctrl Pts',(-15.1681070338602,-82.5994409013717,
-439.778955852854));
#33069=CARTESIAN_POINT('Ctrl Pts',(-15.7977562350973,-70.5464521833251,
-462.499999999978));
#33070=CARTESIAN_POINT('Ctrl Pts',(-18.0885677400365,-82.5280608755568,
-439.778955852854));
#33071=CARTESIAN_POINT('Ctrl Pts',(-18.2815673778157,-69.4842526335149,
-462.499999999979));
#33072=CARTESIAN_POINT('Ctrl Pts',(-20.8989998873753,-81.7348018106291,
-439.787044944617));
#33073=CARTESIAN_POINT('',(-12.3105614915023,-81.8842053074701,-439.904243357679));
#33074=CARTESIAN_POINT('',(-10.4654930467012,-70.2592650976151,-462.499999999978));
#33075=CARTESIAN_POINT('Ctrl Pts',(-20.8989998873751,-81.7348018106294,
-439.787044944617));
#33076=CARTESIAN_POINT('Ctrl Pts',(-19.6456374495956,-81.7524189300427,
-440.37142096878));
#33077=CARTESIAN_POINT('Ctrl Pts',(-18.3143448116165,-81.7724261674984,
-440.772667881321));
#33078=CARTESIAN_POINT('Ctrl Pts',(-16.1385805324535,-81.809038794424,-440.916888546948));
#33079=CARTESIAN_POINT('Ctrl Pts',(-15.3491371083455,-81.8231310310214,
-440.865014920264));
#33080=CARTESIAN_POINT('Ctrl Pts',(-13.7808037670599,-81.8531011884192,
-440.538114526936));
#33081=CARTESIAN_POINT('Ctrl Pts',(-13.0285402685663,-81.8684908169203,
-440.266775657381));
#33082=CARTESIAN_POINT('Ctrl Pts',(-12.3105614915036,-81.8842053074704,
-439.904243357677));
#33083=CARTESIAN_POINT('Origin',(5.02375918642883E-12,-65.4426315587606,
-438.999999999979));
#33084=CARTESIAN_POINT('',(-9.48352202361111,-81.9327028027076,-438.999999999976));
#33085=CARTESIAN_POINT('',(-7.12117861053857,-81.9535288684061,-438.999999999977));
#33086=CARTESIAN_POINT('Origin',(0.000159838139652813,859.827666094174,
-438.999999728954));
#33087=CARTESIAN_POINT('Ctrl Pts',(-9.48352202361107,-81.9327028027073,
-438.999999999977));
#33088=CARTESIAN_POINT('Ctrl Pts',(-9.08970639030352,-81.9095180552699,
-438.999999999977));
#33089=CARTESIAN_POINT('Ctrl Pts',(-8.69522724576118,-81.8996692479367,
-438.999999999977));
#33090=CARTESIAN_POINT('Ctrl Pts',(-7.90709887115381,-81.9066737233761,
-438.999999999977));
#33091=CARTESIAN_POINT('Ctrl Pts',(-7.51369125012755,-81.9234683536681,
-438.999999999977));
#33092=CARTESIAN_POINT('Ctrl Pts',(-7.12117861053855,-81.9535288684059,
-438.999999999977));
#33093=CARTESIAN_POINT('Ctrl Pts',(-3.89356335293881,-70.5754050032805,
-462.499999999978));
#33094=CARTESIAN_POINT('Ctrl Pts',(-4.22808633459723,-82.4205871416874,
-439.001458640508));
#33095=CARTESIAN_POINT('Ctrl Pts',(-6.03305280327815,-69.9075280596242,
-462.499999999979));
#33096=CARTESIAN_POINT('Ctrl Pts',(-6.91662420919795,-81.7519577109097,
-438.999332051806));
#33097=CARTESIAN_POINT('Ctrl Pts',(-8.27177497984179,-69.7998352736863,
-462.499999999979));
#33098=CARTESIAN_POINT('Ctrl Pts',(-9.68449268817595,-81.7275714335143,
-438.99931906013));
#33099=CARTESIAN_POINT('Ctrl Pts',(-10.4654930467012,-70.2592650976151,
-462.499999999978));
#33100=CARTESIAN_POINT('Ctrl Pts',(-12.3842779267235,-82.3486591624718,
-439.001470002309));
#33101=CARTESIAN_POINT('',(-4.21493383398708,-81.95486797187,-439.925355043788));
#33102=CARTESIAN_POINT('',(-3.89356335293881,-70.5754050032805,-462.499999999978));
#33103=CARTESIAN_POINT('Ctrl Pts',(-7.12117861053848,-81.9535288684062,
-438.999999999976));
#33104=CARTESIAN_POINT('Ctrl Pts',(-6.62324952873175,-81.9560718440252,
-439.070014738437));
#33105=CARTESIAN_POINT('Ctrl Pts',(-6.13364118294728,-81.9574020359696,
-439.183225075406));
#33106=CARTESIAN_POINT('Ctrl Pts',(-5.15947229064142,-81.9578371438549,
-439.493384596533));
#33107=CARTESIAN_POINT('Ctrl Pts',(-4.67905024494302,-81.9568662510572,
-439.691871923607));
#33108=CARTESIAN_POINT('Ctrl Pts',(-4.21493383398643,-81.9548679718702,
-439.925355043786));
#33109=CARTESIAN_POINT('Ctrl Pts',(-12.3105614915033,-81.8842053074704,
-439.904243357676));
#33110=CARTESIAN_POINT('Ctrl Pts',(-11.8610189703665,-81.8940670193849,
-439.675963799339));
#33111=CARTESIAN_POINT('Ctrl Pts',(-11.3953934000695,-81.9032084453796,
-439.482522031307));
#33112=CARTESIAN_POINT('Ctrl Pts',(-10.4475434646805,-81.9194866185534,
-439.179364695647));
#33113=CARTESIAN_POINT('Ctrl Pts',(-9.96967424536579,-81.9266070176389,
-439.068753183443));
#33114=CARTESIAN_POINT('Ctrl Pts',(-9.48352202361117,-81.9327028027076,
-438.999999999976));
#33115=CARTESIAN_POINT('Ctrl Pts',(3.89356335294888,-70.5754050032799,-462.499999999978));
#33116=CARTESIAN_POINT('Ctrl Pts',(4.21493383919102,-81.9548693923795,-439.925355068582));
#33117=CARTESIAN_POINT('Ctrl Pts',(1.33838929652316,-71.3730447574958,-462.499999999978));
#33118=CARTESIAN_POINT('Ctrl Pts',(1.43390756316856,-82.6552216731943,-439.915749851982));
#33119=CARTESIAN_POINT('Ctrl Pts',(-1.33838929651297,-71.3730447574961,
-462.499999999978));
#33120=CARTESIAN_POINT('Ctrl Pts',(-1.43390756315624,-82.6552216731946,
-439.915749851982));
#33121=CARTESIAN_POINT('Ctrl Pts',(-3.89356335293881,-70.5754050032805,
-462.499999999978));
#33122=CARTESIAN_POINT('Ctrl Pts',(-4.21493383398708,-81.95486797187,-439.925355043787));
#33123=CARTESIAN_POINT('',(4.21493383919094,-81.9548693923797,-439.925355068582));
#33124=CARTESIAN_POINT('',(3.89356335294888,-70.5754050032799,-462.499999999978));
#33125=CARTESIAN_POINT('Ctrl Pts',(4.21493383919057,-81.9548693923798,-439.925355068582));
#33126=CARTESIAN_POINT('Ctrl Pts',(3.54934499941135,-81.9520270095361,-440.25884255782));
#33127=CARTESIAN_POINT('Ctrl Pts',(2.8548204219887,-81.9497427021224,-440.52735679615));
#33128=CARTESIAN_POINT('Ctrl Pts',(1.43300534097921,-81.9466845475377,-440.88703829099));
#33129=CARTESIAN_POINT('Ctrl Pts',(0.721578194027332,-81.9458978792099,
-440.979675755148));
#33130=CARTESIAN_POINT('Ctrl Pts',(-0.722493479587384,-81.9458984309402,
-440.979581995565));
#33131=CARTESIAN_POINT('Ctrl Pts',(-1.43373571979195,-81.9466852459727,
-440.886898928913));
#33132=CARTESIAN_POINT('Ctrl Pts',(-2.85517004898937,-81.9497428822133,
-440.527222128221));
#33133=CARTESIAN_POINT('Ctrl Pts',(-3.54951323389898,-81.9520265269081,
-440.258758519013));
#33134=CARTESIAN_POINT('Ctrl Pts',(-4.2149338339865,-81.9548679718702,-439.925355043787));
#33135=CARTESIAN_POINT('Origin',(5.02375918642883E-12,-65.4426315587606,
-438.999999999979));
#33136=CARTESIAN_POINT('',(7.12117862753353,-81.9535312690186,-438.999999999978));
#33137=CARTESIAN_POINT('',(9.48352205464678,-81.9327059996163,-438.999999999978));
#33138=CARTESIAN_POINT('Origin',(0.000157662688085036,859.827665975351,
-439.000000180659));
#33139=CARTESIAN_POINT('Ctrl Pts',(7.12117862753352,-81.9535312690185,-438.999999999978));
#33140=CARTESIAN_POINT('Ctrl Pts',(7.51410779327789,-81.9234389742552,-438.999999999978));
#33141=CARTESIAN_POINT('Ctrl Pts',(7.90793370256448,-81.9066407489514,-438.999999999977));
#33142=CARTESIAN_POINT('Ctrl Pts',(8.69606258685533,-81.8996930223353,-438.999999999977));
#33143=CARTESIAN_POINT('Ctrl Pts',(9.09012343726988,-81.9095456552935,-438.999999999978));
#33144=CARTESIAN_POINT('Ctrl Pts',(9.48352205464679,-81.9327059996161,-438.999999999978));
#33145=CARTESIAN_POINT('Ctrl Pts',(10.4654930467115,-70.2592650976135,-462.499999999978));
#33146=CARTESIAN_POINT('Ctrl Pts',(12.3842778439454,-82.3486626074551,-439.001471767375));
#33147=CARTESIAN_POINT('Ctrl Pts',(8.27177497985184,-69.7998352736849,-462.499999999978));
#33148=CARTESIAN_POINT('Ctrl Pts',(9.68449198910565,-81.7275751837853,-438.999317851236));
#33149=CARTESIAN_POINT('Ctrl Pts',(6.03305280328818,-69.9075280596233,-462.499999999978));
#33150=CARTESIAN_POINT('Ctrl Pts',(6.91662493113332,-81.7519599718325,-438.999332171566));
#33151=CARTESIAN_POINT('Ctrl Pts',(3.89356335294888,-70.5754050032799,-462.499999999978));
#33152=CARTESIAN_POINT('Ctrl Pts',(4.22808633184835,-82.4205883312023,-439.001459239898));
#33153=CARTESIAN_POINT('',(12.3105615445815,-81.8842094560395,-439.904243430097));
#33154=CARTESIAN_POINT('',(10.4654930467115,-70.2592650976135,-462.499999999979));
#33155=CARTESIAN_POINT('Ctrl Pts',(9.48352205464689,-81.9327059996164,-438.999999999977));
#33156=CARTESIAN_POINT('Ctrl Pts',(9.96970255654653,-81.9266100234847,-439.068757204431));
#33157=CARTESIAN_POINT('Ctrl Pts',(10.4475989576107,-81.919489312792,-439.179377597763));
#33158=CARTESIAN_POINT('Ctrl Pts',(11.3954460472368,-81.9032112524941,-439.482543979102));
#33159=CARTESIAN_POINT('Ctrl Pts',(11.8610444462678,-81.8940704579246,-439.675976824542));
#33160=CARTESIAN_POINT('Ctrl Pts',(12.3105615445817,-81.8842094560397,-439.904243430096));
#33161=CARTESIAN_POINT('Ctrl Pts',(4.21493383919116,-81.9548693923798,-439.925355068582));
#33162=CARTESIAN_POINT('Ctrl Pts',(4.67904816069443,-81.956867818085,-439.691873053696));
#33163=CARTESIAN_POINT('Ctrl Pts',(5.15946796055897,-81.9578388730233,-439.49338646958));
#33164=CARTESIAN_POINT('Ctrl Pts',(6.13363661544826,-81.9574041152318,-439.183226185497));
#33165=CARTESIAN_POINT('Ctrl Pts',(6.62324720515649,-81.9560740883707,-439.070015088001));
#33166=CARTESIAN_POINT('Ctrl Pts',(7.12117862753345,-81.9535312690188,-438.999999999977));
#33167=CARTESIAN_POINT('Ctrl Pts',(18.2815673778257,-69.4842526335121,-462.499999999979));
#33168=CARTESIAN_POINT('Ctrl Pts',(20.8990000425199,-81.7348088522914,-439.787045067561));
#33169=CARTESIAN_POINT('Ctrl Pts',(15.7977562351075,-70.5464521833227,-462.499999999978));
#33170=CARTESIAN_POINT('Ctrl Pts',(18.0885677400489,-82.5280608755536,-439.778955852855));
#33171=CARTESIAN_POINT('Ctrl Pts',(13.1095347615097,-70.8130060900595,-462.499999999978));
#33172=CARTESIAN_POINT('Ctrl Pts',(15.1681070338725,-82.599440901369,-439.778955852855));
#33173=CARTESIAN_POINT('Ctrl Pts',(10.4654930467115,-70.2592650976135,-462.499999999978));
#33174=CARTESIAN_POINT('Ctrl Pts',(12.3200202173657,-81.9438042867714,-439.788407151959));
#33175=CARTESIAN_POINT('',(20.8990000425197,-81.7348088522915,-439.787045067561));
#33176=CARTESIAN_POINT('',(18.2815673778257,-69.4842526335121,-462.499999999979));
#33177=CARTESIAN_POINT('Ctrl Pts',(12.3105615445817,-81.8842094560396,-439.904243430097));
#33178=CARTESIAN_POINT('Ctrl Pts',(12.9424829255709,-81.8703787725802,-440.223319792049));
#33179=CARTESIAN_POINT('Ctrl Pts',(13.6020736939311,-81.8567751181056,-440.472315085927));
#33180=CARTESIAN_POINT('Ctrl Pts',(14.9703535636644,-81.8302081245194,-440.804754741935));
#33181=CARTESIAN_POINT('Ctrl Pts',(15.6610816623562,-81.8175741397569,-440.885758233786));
#33182=CARTESIAN_POINT('Ctrl Pts',(17.1296347509788,-81.7921241598419,-440.881946716635));
#33183=CARTESIAN_POINT('Ctrl Pts',(17.8889355257091,-81.7797619763488,-440.780290522576));
#33184=CARTESIAN_POINT('Ctrl Pts',(19.4146607479418,-81.7561159296533,-440.405153968589));
#33185=CARTESIAN_POINT('Ctrl Pts',(20.1714264871945,-81.7450353487284,-440.126270879395));
#33186=CARTESIAN_POINT('Ctrl Pts',(20.8990000425196,-81.7348088522916,-439.787045067561));
#33187=CARTESIAN_POINT('Origin',(5.02375918642883E-12,-65.4426315587606,
-438.999999999979));
#33188=CARTESIAN_POINT('',(23.5144782588677,-81.6868634501823,-438.999999999977));
#33189=CARTESIAN_POINT('',(25.7039047706638,-81.6296351104369,-438.999999999978));
#33190=CARTESIAN_POINT('Origin',(0.000155981030567354,859.827648586247,
-438.999999842311));
#33191=CARTESIAN_POINT('Ctrl Pts',(23.5144782588677,-81.686863450182,-438.999999999977));
#33192=CARTESIAN_POINT('Ctrl Pts',(23.8779552573195,-81.6506927118015,-438.999999999977));
#33193=CARTESIAN_POINT('Ctrl Pts',(24.2426281344593,-81.6278161321225,-438.999999999973));
#33194=CARTESIAN_POINT('Ctrl Pts',(24.9731693890883,-81.608711524059,-438.999999999973));
#33195=CARTESIAN_POINT('Ctrl Pts',(25.3387874851401,-81.6125080570722,-438.999999999977));
#33196=CARTESIAN_POINT('Ctrl Pts',(25.7039047706638,-81.6296351104367,-438.999999999977));
#33197=CARTESIAN_POINT('Ctrl Pts',(26.5149982231106,-69.0440180573124,-462.499999999979));
#33198=CARTESIAN_POINT('Ctrl Pts',(30.6502301216108,-82.7145147833341,-438.999999999977));
#33199=CARTESIAN_POINT('Ctrl Pts',(23.6668225265683,-68.171468601074,-462.499999999979));
#33200=CARTESIAN_POINT('Ctrl Pts',(27.4436392089424,-81.415652603698,-439.001453877264));
#33201=CARTESIAN_POINT('Ctrl Pts',(20.8066529626785,-68.4044021064994,-462.499999999979));
#33202=CARTESIAN_POINT('Ctrl Pts',(24.0993065058744,-81.29705577815,-438.998060570033));
#33203=CARTESIAN_POINT('Ctrl Pts',(18.2815673778257,-69.4842526335121,-462.499999999979));
#33204=CARTESIAN_POINT('Ctrl Pts',(20.9895258069676,-82.1585030246664,-439.001501417916));
#33205=CARTESIAN_POINT('',(30.0769364718121,-81.4651482118546,-441.000049527067));
#33206=CARTESIAN_POINT('Ctrl Pts',(30.0769364733382,-81.4651482119768,-441.000049527336));
#33207=CARTESIAN_POINT('Ctrl Pts',(29.8061861881463,-80.2987458269529,-443.068934798007));
#33208=CARTESIAN_POINT('Ctrl Pts',(29.5081626488663,-79.1197036090261,-445.139865574628));
#33209=CARTESIAN_POINT('Ctrl Pts',(28.8453460499946,-76.7250958481571,-449.301315287558));
#33210=CARTESIAN_POINT('Ctrl Pts',(28.4753114889536,-75.4961210030392,-451.41369731436));
#33211=CARTESIAN_POINT('Ctrl Pts',(27.4791729678182,-72.4959292673654,-456.513948240452));
#33212=CARTESIAN_POINT('Ctrl Pts',(26.7965164718484,-70.6752595300762,-459.55708022097));
#33213=CARTESIAN_POINT('Ctrl Pts',(25.9994431732941,-68.8985804999194,-462.499999999979));
#33214=CARTESIAN_POINT('Ctrl Pts',(25.7039047706639,-81.6296351104371,-438.999999999977));
#33215=CARTESIAN_POINT('Ctrl Pts',(26.6066393041569,-81.6027909675482,-439.125853859304));
#33216=CARTESIAN_POINT('Ctrl Pts',(27.4708379293598,-81.5730007420501,-439.405781130766));
#33217=CARTESIAN_POINT('Ctrl Pts',(28.9250644802948,-81.5164546086103,-440.141784715098));
#33218=CARTESIAN_POINT('Ctrl Pts',(29.5233073521062,-81.4908339430079,-440.542202709549));
#33219=CARTESIAN_POINT('Ctrl Pts',(30.0769364719202,-81.4651482116506,-441.000049526925));
#33220=CARTESIAN_POINT('Ctrl Pts',(20.8990000425198,-81.7348088522916,-439.787045067561));
#33221=CARTESIAN_POINT('Ctrl Pts',(21.3204957294972,-81.7288979936655,-439.58975120819));
#33222=CARTESIAN_POINT('Ctrl Pts',(21.7548089567099,-81.7219103005923,-439.421599055221));
#33223=CARTESIAN_POINT('Ctrl Pts',(22.6307047917946,-81.7058594459475,-439.158050593173));
#33224=CARTESIAN_POINT('Ctrl Pts',(23.0693369665686,-81.6969152647404,-439.061028459663));
#33225=CARTESIAN_POINT('Ctrl Pts',(23.5144782588676,-81.6868634501824,-438.999999999977));
#33226=CARTESIAN_POINT('Ctrl Pts',(43.201920988198,-80.9594167953459,-440.991769323448));
#33227=CARTESIAN_POINT('Ctrl Pts',(43.197523751011,-80.9543288413526,-441.000060412176));
#33228=CARTESIAN_POINT('Ctrl Pts',(31.7948796623075,-67.7605605594772,-462.499999999979));
#33229=CARTESIAN_POINT('Ctrl Pts',(31.7834770182188,-67.7473667911953,-462.521499939567));
#33230=CARTESIAN_POINT('Ctrl Pts',(38.8247909292306,-81.1567005156185,-440.991727099844));
#33231=CARTESIAN_POINT('Ctrl Pts',(38.8208728590421,-81.151811181641,-440.999999999977));
#33232=CARTESIAN_POINT('Ctrl Pts',(28.638408705173,-68.4451812419819,-462.499999999979));
#33233=CARTESIAN_POINT('Ctrl Pts',(28.6282038254292,-68.4324466397753,-462.521547329896));
#33234=CARTESIAN_POINT('Ctrl Pts',(34.4491908471433,-81.3268471958895,-440.991742546106));
#33235=CARTESIAN_POINT('Ctrl Pts',(34.4457390925038,-81.3221254984189,-440.999999999977));
#33236=CARTESIAN_POINT('Ctrl Pts',(25.4583773817474,-69.0282032793794,-462.499999999978));
#33237=CARTESIAN_POINT('Ctrl Pts',(25.4493533867103,-69.0158592459841,-462.521587635989));
#33238=CARTESIAN_POINT('Ctrl Pts',(30.0724320076141,-81.4699728715382,-440.991815654647));
#33239=CARTESIAN_POINT('Ctrl Pts',(30.0694364969325,-81.4653876356763,-441.000060406224));
#33240=CARTESIAN_POINT('Ctrl Pts',(22.2580066308556,-69.5084119606264,-462.499999999979));
#33241=CARTESIAN_POINT('Ctrl Pts',(22.250151299191,-69.496387784356,-462.521620773535));
#33242=CARTESIAN_POINT('Ctrl Pts',(30.0769364718065,-81.465148211635,-441.000049528026));
#33243=CARTESIAN_POINT('Ctrl Pts',(32.2034419211209,-81.3972545994429,-440.996967120045));
#33244=CARTESIAN_POINT('Ctrl Pts',(34.329571566688,-81.3221311807446,-440.995540157727));
#33245=CARTESIAN_POINT('Ctrl Pts',(38.703204763265,-81.1527038540004,-440.995547974776));
#33246=CARTESIAN_POINT('Ctrl Pts',(40.9505527826719,-81.0575526448392,-440.997149115757));
#33247=CARTESIAN_POINT('Ctrl Pts',(43.1975237510106,-80.9543288413528,-441.000060412176));
#33248=CARTESIAN_POINT('Ctrl Pts',(38.9588941886819,-63.9631388095498,-462.498954222077));
#33249=CARTESIAN_POINT('Ctrl Pts',(38.9383104029384,-63.9498936427278,-462.523755685796));
#33250=CARTESIAN_POINT('Ctrl Pts',(36.9523181444951,-65.8754708585682,-462.499999999979));
#33251=CARTESIAN_POINT('Ctrl Pts',(36.934067668895,-65.8607515207863,-462.52446915918));
#33252=CARTESIAN_POINT('Ctrl Pts',(34.5033857139835,-67.173100929134,-462.499999999979));
#33253=CARTESIAN_POINT('Ctrl Pts',(34.487712629227,-67.1576857515551,-462.52446915918));
#33254=CARTESIAN_POINT('Ctrl Pts',(31.7948796623075,-67.7605605594772,-462.499999999979));
#33255=CARTESIAN_POINT('Ctrl Pts',(31.7817253813645,-67.7453400077063,-462.524802689899));
#33256=CARTESIAN_POINT('Ctrl Pts',(64.2844510030596,-67.9859312604405,-440.982510346491));
#33257=CARTESIAN_POINT('Ctrl Pts',(64.2750751909262,-67.9713441846113,-441.000078299647));
#33258=CARTESIAN_POINT('Ctrl Pts',(56.5172406812969,-55.9015414418543,-455.536347698364));
#33259=CARTESIAN_POINT('Ctrl Pts',(56.5171259388062,-55.9013629232716,-455.536562697357));
#33260=CARTESIAN_POINT('Ctrl Pts',(64.2829289255942,-67.9876489086986,-440.982510283378));
#33261=CARTESIAN_POINT('Ctrl Pts',(64.2735519592642,-67.9730629321979,-441.000078248778));
#33262=CARTESIAN_POINT('Ctrl Pts',(56.5147649746143,-55.9041767025935,-455.536350963711));
#33263=CARTESIAN_POINT('Ctrl Pts',(56.5146502181162,-55.9039981976221,-455.536565962653));
#33264=CARTESIAN_POINT('Ctrl Pts',(64.2814068481288,-67.9893665569567,-440.982510220263));
#33265=CARTESIAN_POINT('Ctrl Pts',(64.2720287276024,-67.9747816797845,-441.000078197908));
#33266=CARTESIAN_POINT('Ctrl Pts',(56.5122892679318,-55.9068119633328,-455.536354229059));
#33267=CARTESIAN_POINT('Ctrl Pts',(56.5121744974262,-55.9066334719727,-455.536569227948));
#33268=CARTESIAN_POINT('Ctrl Pts',(64.2798847706634,-67.9910842052148,-440.982510157149));
#33269=CARTESIAN_POINT('Ctrl Pts',(64.2705054959406,-67.9765004273711,-441.000078147038));
#33270=CARTESIAN_POINT('Ctrl Pts',(56.5098135612492,-55.909447224072,-455.536357494406));
#33271=CARTESIAN_POINT('Ctrl Pts',(56.5096987767362,-55.9092687463232,-455.536572493243));
#33272=CARTESIAN_POINT('Ctrl Pts',(61.9416205008464,-70.629790605742,-440.982413198853));
#33273=CARTESIAN_POINT('Ctrl Pts',(61.9304681124519,-70.6168956516489,-440.999999999979));
#33274=CARTESIAN_POINT('Ctrl Pts',(52.7092909776432,-59.9549054455595,-455.541370214756));
#33275=CARTESIAN_POINT('Ctrl Pts',(52.7091546899917,-59.9547478629012,-455.541585134084));
#33276=CARTESIAN_POINT('Ctrl Pts',(59.4518703978667,-73.1191818960986,-440.982413198852));
#33277=CARTESIAN_POINT('Ctrl Pts',(59.4389827344574,-73.1080225102857,-440.999999999979));
#33278=CARTESIAN_POINT('Ctrl Pts',(48.7830207157406,-63.8810596700917,-455.541370214754));
#33279=CARTESIAN_POINT('Ctrl Pts',(48.782863222178,-63.8809232969282,-455.541585134083));
#33280=CARTESIAN_POINT('Ctrl Pts',(56.8163034073806,-75.4539484719562,-440.982509561286));
#33281=CARTESIAN_POINT('Ctrl Pts',(56.8017229870639,-75.4445663251619,-441.000077552423));
#33282=CARTESIAN_POINT('Ctrl Pts',(44.7374479017925,-67.6814979527012,-455.536357931381));
#33283=CARTESIAN_POINT('Ctrl Pts',(44.7372694651336,-67.6813831330396,-455.536572930234));
#33284=CARTESIAN_POINT('Ctrl Pts',(56.8145878317028,-75.4554682469289,-440.982509624012));
#33285=CARTESIAN_POINT('Ctrl Pts',(56.800006309516,-75.4460872569967,-441.000077602904));
#33286=CARTESIAN_POINT('Ctrl Pts',(44.734812610957,-67.6839735626181,-455.536354666374));
#33287=CARTESIAN_POINT('Ctrl Pts',(44.7346341606556,-67.6838587569965,-455.536569665279));
#33288=CARTESIAN_POINT('Ctrl Pts',(56.8128722560251,-75.4569880219015,-440.982509686737));
#33289=CARTESIAN_POINT('Ctrl Pts',(56.798289631968,-75.4476081888316,-441.000077653386));
#33290=CARTESIAN_POINT('Ctrl Pts',(44.7321773201212,-67.686449172535,-455.536351401367));
#33291=CARTESIAN_POINT('Ctrl Pts',(44.7319988561776,-67.6863343809532,-455.536566400323));
#33292=CARTESIAN_POINT('Ctrl Pts',(56.8111566803473,-75.4585077968741,-440.982509749462));
#33293=CARTESIAN_POINT('Ctrl Pts',(56.7965729544201,-75.4491291206665,-441.000077703867));
#33294=CARTESIAN_POINT('Ctrl Pts',(44.7295420292855,-67.6889247824519,-455.536348136359));
#33295=CARTESIAN_POINT('Ctrl Pts',(44.7293635516996,-67.6888100049102,-455.536563135368));
#33296=CARTESIAN_POINT('Ctrl Pts',(56.8017229870589,-75.4445663251663,-441.000077552423));
#33297=CARTESIAN_POINT('Ctrl Pts',(56.8648198811864,-75.3888096554507,-440.999961040072));
#33298=CARTESIAN_POINT('Ctrl Pts',(56.9490629520645,-75.3142041475122,-440.99980826392));
#33299=CARTESIAN_POINT('Ctrl Pts',(57.1309026962115,-75.1522669958779,-440.999493603969));
#33300=CARTESIAN_POINT('Ctrl Pts',(57.2129563206459,-75.0789104508246,-440.999356367237));
#33301=CARTESIAN_POINT('Ctrl Pts',(57.4587061305076,-74.8583554202793,-440.998959410034));
#33302=CARTESIAN_POINT('Ctrl Pts',(57.6219769384721,-74.7106841995689,-440.998714462169));
#33303=CARTESIAN_POINT('Ctrl Pts',(58.1101297576784,-74.2657415537038,-440.998037197435));
#33304=CARTESIAN_POINT('Ctrl Pts',(58.4332925903842,-73.9665939710789,-440.997662466009));
#33305=CARTESIAN_POINT('Ctrl Pts',(59.3960169304096,-73.0615413671499,-440.996760635968));
#33306=CARTESIAN_POINT('Ctrl Pts',(60.0285620594009,-72.4482523252744,-440.996454799799));
#33307=CARTESIAN_POINT('Ctrl Pts',(61.2742044918225,-71.2027168180214,-440.996429126657));
#33308=CARTESIAN_POINT('Ctrl Pts',(61.8872423624114,-70.5705492064193,-440.996708949208));
#33309=CARTESIAN_POINT('Ctrl Pts',(62.7920842157113,-69.6082439366836,-440.997600483858));
#33310=CARTESIAN_POINT('Ctrl Pts',(63.091261927389,-69.2851139850578,-440.997976729447));
#33311=CARTESIAN_POINT('Ctrl Pts',(63.536287614412,-68.7969688084124,-440.998667403033));
#33312=CARTESIAN_POINT('Ctrl Pts',(63.6840113457327,-68.6336726425307,-440.998918717446));
#33313=CARTESIAN_POINT('Ctrl Pts',(63.9046541692162,-68.3878737184406,-440.999328524882));
#33314=CARTESIAN_POINT('Ctrl Pts',(63.9780461765651,-68.3057965653884,-440.999470605172));
#33315=CARTESIAN_POINT('Ctrl Pts',(64.1400134581583,-68.1239584591725,-440.999797190977));
#33316=CARTESIAN_POINT('Ctrl Pts',(64.2146497815168,-68.0396973166364,-440.999956381979));
#33317=CARTESIAN_POINT('Ctrl Pts',(64.2705054959405,-67.9765004273713,-441.000078147039));
#33318=CARTESIAN_POINT('Ctrl Pts',(56.5915605594697,-42.9638796623104,-462.499999999983));
#33319=CARTESIAN_POINT('Ctrl Pts',(56.5747906715002,-42.9493768901674,-462.527334954314));
#33320=CARTESIAN_POINT('Ctrl Pts',(56.0041009291271,-45.6723857139866,-462.499999999983));
#33321=CARTESIAN_POINT('Ctrl Pts',(55.9871198863777,-45.6551025508765,-462.52696699751));
#33322=CARTESIAN_POINT('Ctrl Pts',(54.7064708585618,-48.1213181444985,-462.499999999982));
#33323=CARTESIAN_POINT('Ctrl Pts',(54.6902576362458,-48.1011934320598,-462.52696699751));
#33324=CARTESIAN_POINT('Ctrl Pts',(52.7925979348378,-50.1295710081989,-462.498943458986));
#33325=CARTESIAN_POINT('Ctrl Pts',(52.7780049328352,-50.1068804371721,-462.52627709823));
#33326=CARTESIAN_POINT('Origin',(54.2736315587506,-11.1690000000061,-438.999999999986));
#33327=CARTESIAN_POINT('Ctrl Pts',(70.512394258107,12.4256934496976,-438.999999999989));
#33328=CARTESIAN_POINT('Ctrl Pts',(70.4806962609452,12.7626097179399,-438.999999999989));
#33329=CARTESIAN_POINT('Ctrl Pts',(70.4604150062139,13.1004968020805,-438.999999999987));
#33330=CARTESIAN_POINT('Ctrl Pts',(70.4427152853469,13.7773550845288,-438.999999999987));
#33331=CARTESIAN_POINT('Ctrl Pts',(70.4453211759903,14.1161237170503,-438.99999999999));
#33332=CARTESIAN_POINT('Ctrl Pts',(70.4593636589103,14.4545180952481,-438.99999999999));
#33333=CARTESIAN_POINT('Ctrl Pts',(69.7886736272828,32.0388792074281,-440.988676628513));
#33334=CARTESIAN_POINT('Ctrl Pts',(69.7816652336223,32.0328182762799,-441.000100325617));
#33335=CARTESIAN_POINT('Ctrl Pts',(56.5915605594642,20.6258796622937,-462.49999999999));
#33336=CARTESIAN_POINT('Ctrl Pts',(56.5783704547901,20.6144727236797,-462.521499899664));
#33337=CARTESIAN_POINT('Ctrl Pts',(69.9838203851238,27.6573003811947,-440.988601378206));
#33338=CARTESIAN_POINT('Ctrl Pts',(69.9770872889492,27.6518995318566,-440.999999999991));
#33339=CARTESIAN_POINT('Ctrl Pts',(57.2771687825099,17.4648556101157,-462.499999999989));
#33340=CARTESIAN_POINT('Ctrl Pts',(57.2644408666264,17.4546461085292,-462.521547397428));
#33341=CARTESIAN_POINT('Ctrl Pts',(70.1541602115504,23.274511221385,-440.988622685345));
#33342=CARTESIAN_POINT('Ctrl Pts',(70.1476583281893,23.2697541556268,-440.99999999999));
#33343=CARTESIAN_POINT('Ctrl Pts',(57.8608844602741,14.2802063587041,-462.49999999999));
#33344=CARTESIAN_POINT('Ctrl Pts',(57.8485475387408,14.2711801206548,-462.521587750835));
#33345=CARTESIAN_POINT('Ctrl Pts',(70.2996831943332,18.890636417085,-440.988740602151));
#33346=CARTESIAN_POINT('Ctrl Pts',(70.2933682482186,18.8865091831852,-441.000100380184));
#33347=CARTESIAN_POINT('Ctrl Pts',(58.3414879230458,11.0751668932784,-462.499999999988));
#33348=CARTESIAN_POINT('Ctrl Pts',(58.3294687920448,11.0673115982351,-462.521620874947));
#33349=CARTESIAN_POINT('Ctrl Pts',(70.2997304533948,18.8892127394985,-440.988740640445));
#33350=CARTESIAN_POINT('Ctrl Pts',(70.2934155679886,18.8850857101388,-441.000100412783));
#33351=CARTESIAN_POINT('Ctrl Pts',(58.3416442407962,11.0741244443621,-462.499999999988));
#33352=CARTESIAN_POINT('Ctrl Pts',(58.3296252131575,11.0662695301716,-462.521620885722));
#33353=CARTESIAN_POINT('Ctrl Pts',(70.2997777124563,18.887789061912,-440.988740678739));
#33354=CARTESIAN_POINT('Ctrl Pts',(70.2934628877585,18.8836622370922,-441.000100445382));
#33355=CARTESIAN_POINT('Ctrl Pts',(58.3418005585465,11.0730819954458,-462.499999999988));
#33356=CARTESIAN_POINT('Ctrl Pts',(58.32978163427,11.0652274621081,-462.521620896496));
#33357=CARTESIAN_POINT('Ctrl Pts',(70.2998249715178,18.8863653843256,-440.988740717032));
#33358=CARTESIAN_POINT('Ctrl Pts',(70.2935102075285,18.8822387640455,-441.00010047798));
#33359=CARTESIAN_POINT('Ctrl Pts',(58.3419568762969,11.0720395465295,-462.499999999988));
#33360=CARTESIAN_POINT('Ctrl Pts',(58.3299380553828,11.0641853940446,-462.521620907269));
#33361=CARTESIAN_POINT('Ctrl Pts',(70.2929704412094,18.89898172966,-441.000070381186));
#33362=CARTESIAN_POINT('Ctrl Pts',(69.4478798152777,18.703333595985,-442.499259503123));
#33363=CARTESIAN_POINT('Ctrl Pts',(68.5970566354322,18.4935685970824,-443.998044926457));
#33364=CARTESIAN_POINT('Ctrl Pts',(66.921371690547,18.0525189012106,-446.927744712079));
#33365=CARTESIAN_POINT('Ctrl Pts',(66.0883452949664,17.8200628885466,-448.373677904118));
#33366=CARTESIAN_POINT('Ctrl Pts',(65.2503505017821,17.5706789545087,-449.81715836622));
#33367=CARTESIAN_POINT('Ctrl Pts',(64.5871672591961,17.3700458363661,-450.95723971308));
#33368=CARTESIAN_POINT('Ctrl Pts',(63.402389223456,17.0056913908832,-452.989932143487));
#33369=CARTESIAN_POINT('Ctrl Pts',(62.210822170982,16.6072491489963,-455.011995086995));
#33370=CARTESIAN_POINT('Ctrl Pts',(59.9333797132287,15.7661053116544,-458.839522722581));
#33371=CARTESIAN_POINT('Ctrl Pts',(58.8249846736614,15.3210207890733,-460.685225965698));
#33372=CARTESIAN_POINT('Ctrl Pts',(57.7295804999066,14.8304431732807,-462.499999999989));
#33373=CARTESIAN_POINT('Ctrl Pts',(70.2996831378601,-41.2286363801844,-440.988740703741));
#33374=CARTESIAN_POINT('Ctrl Pts',(70.2933682482237,-41.2245091831969,-441.000100380177));
#33375=CARTESIAN_POINT('Ctrl Pts',(58.3414879230496,-33.4131668932962,-462.499999999984));
#33376=CARTESIAN_POINT('Ctrl Pts',(58.3294687920485,-33.4053115982529,-462.521620874943));
#33377=CARTESIAN_POINT('Ctrl Pts',(70.1541601534062,-45.6125111788507,-440.988622787091));
#33378=CARTESIAN_POINT('Ctrl Pts',(70.1476583281953,-45.607754155638,-440.999999999982));
#33379=CARTESIAN_POINT('Ctrl Pts',(57.8608844602783,-36.6182063587215,-462.499999999984));
#33380=CARTESIAN_POINT('Ctrl Pts',(57.8485475387452,-36.6091801206722,-462.521587750829));
#33381=CARTESIAN_POINT('Ctrl Pts',(69.9838203249125,-49.9953003329024,-440.988601480142));
#33382=CARTESIAN_POINT('Ctrl Pts',(69.977087288956,-49.9898995318672,-440.999999999982));
#33383=CARTESIAN_POINT('Ctrl Pts',(57.2771687825149,-39.8028556101327,-462.499999999983));
#33384=CARTESIAN_POINT('Ctrl Pts',(57.2644408666313,-39.7926461085464,-462.521547397421));
#33385=CARTESIAN_POINT('Ctrl Pts',(69.7886735646101,-54.3768791532312,-440.988676730672));
#33386=CARTESIAN_POINT('Ctrl Pts',(69.7816652336298,-54.3708182762895,-441.000100325607));
#33387=CARTESIAN_POINT('Ctrl Pts',(56.5915605594697,-42.9638796623104,-462.499999999983));
#33388=CARTESIAN_POINT('Ctrl Pts',(56.5783704547956,-42.9524727236964,-462.521499899657));
#33389=CARTESIAN_POINT('Origin',(22.4991425263181,166.837401348805,-389.327908649814));
#33390=CARTESIAN_POINT('Origin',(54.2736315587506,-11.1690000000061,-438.999999999986));
#33391=CARTESIAN_POINT('Ctrl Pts',(57.867944997635,-37.6757543779957,-462.508620368993));
#33392=CARTESIAN_POINT('Ctrl Pts',(57.872959299689,-37.6772709866423,-462.499999999983));
#33393=CARTESIAN_POINT('Ctrl Pts',(71.5424551348726,-41.8116999372577,-438.999999999983));
#33394=CARTESIAN_POINT('Ctrl Pts',(71.5463747327639,-41.8128854454279,-438.993261598541));
#33395=CARTESIAN_POINT('Ctrl Pts',(57.8719099587016,-37.6887260106591,-462.508620581582));
#33396=CARTESIAN_POINT('Ctrl Pts',(57.8769250855219,-37.6902432536445,-462.499999999983));
#33397=CARTESIAN_POINT('Ctrl Pts',(71.5483174526145,-41.8262325427425,-438.999989167174));
#33398=CARTESIAN_POINT('Ctrl Pts',(71.5522375084354,-41.8274184918791,-438.993250925682));
#33399=CARTESIAN_POINT('Ctrl Pts',(57.8758749197681,-37.7016976433226,-462.508620794173));
#33400=CARTESIAN_POINT('Ctrl Pts',(57.8808908713546,-37.7032155206467,-462.499999999983));
#33401=CARTESIAN_POINT('Ctrl Pts',(71.5541797703564,-41.8407651482274,-438.999978334365));
#33402=CARTESIAN_POINT('Ctrl Pts',(71.5581002841068,-41.8419515383303,-438.993240252822));
#33403=CARTESIAN_POINT('Ctrl Pts',(57.8798398808347,-37.7146692759861,-462.508621006763));
#33404=CARTESIAN_POINT('Ctrl Pts',(57.8848566571874,-37.7161877876489,-462.499999999983));
#33405=CARTESIAN_POINT('Ctrl Pts',(71.5600420880984,-41.8552977537122,-438.999967501557));
#33406=CARTESIAN_POINT('Ctrl Pts',(71.5639630597783,-41.8564845847815,-438.993229579963));
#33407=CARTESIAN_POINT('Ctrl Pts',(59.0902650976022,-21.634493046715,-462.499999999985));
#33408=CARTESIAN_POINT('Ctrl Pts',(70.7709995585468,-23.4880802833718,-439.80032773308));
#33409=CARTESIAN_POINT('Ctrl Pts',(59.6440060900487,-24.2785347615132,-462.499999999984));
#33410=CARTESIAN_POINT('Ctrl Pts',(71.4248025866704,-26.3361222680391,-439.789824991753));
#33411=CARTESIAN_POINT('Ctrl Pts',(59.3774521833123,-26.966756235111,-462.499999999984));
#33412=CARTESIAN_POINT('Ctrl Pts',(71.353329194899,-29.2564718771875,-439.789824991753));
#33413=CARTESIAN_POINT('Ctrl Pts',(58.315252633502,-29.4505673778293,-462.499999999984));
#33414=CARTESIAN_POINT('Ctrl Pts',(70.5621815020438,-32.0667859302444,-439.798062313332));
#33415=CARTESIAN_POINT('',(59.0902650976022,-21.6344930467149,-462.499999999985));
#33416=CARTESIAN_POINT('Origin',(54.2736315587506,-11.1690000000061,-438.999999999986));
#33417=CARTESIAN_POINT('Ctrl Pts',(70.7611151580493,-20.5658120600565,-438.999999999985));
#33418=CARTESIAN_POINT('Ctrl Pts',(70.7414378019089,-20.2008497257058,-438.999999999986));
#33419=CARTESIAN_POINT('Ctrl Pts',(70.7332146113695,-19.8353710262216,-438.999999999986));
#33420=CARTESIAN_POINT('Ctrl Pts',(70.7396988669432,-19.1051660456595,-438.999999999986));
#33421=CARTESIAN_POINT('Ctrl Pts',(70.754357444811,-18.7406409415397,-438.999999999986));
#33422=CARTESIAN_POINT('Ctrl Pts',(70.7804124467093,-18.3768313194476,-438.999999999986));
#33423=CARTESIAN_POINT('Ctrl Pts',(59.4064050032676,-15.0625633529524,-462.499999999986));
#33424=CARTESIAN_POINT('Ctrl Pts',(71.2535130610729,-15.3970838267174,-439.002429127845));
#33425=CARTESIAN_POINT('Ctrl Pts',(58.7385280596113,-17.2020528032917,-462.499999999986));
#33426=CARTESIAN_POINT('Ctrl Pts',(70.5853951815301,-18.0862311145172,-438.998932713963));
#33427=CARTESIAN_POINT('Ctrl Pts',(58.6308352736733,-19.4407749798555,-462.499999999985));
#33428=CARTESIAN_POINT('Ctrl Pts',(70.5610300866927,-20.8529288319753,-438.998910332345));
#33429=CARTESIAN_POINT('Ctrl Pts',(59.0902650976022,-21.634493046715,-462.499999999985));
#33430=CARTESIAN_POINT('Ctrl Pts',(71.1815697946312,-23.5532326718541,-439.002448983861));
#33431=CARTESIAN_POINT('',(59.4064050032676,-15.0625633529524,-462.499999999986));
#33432=CARTESIAN_POINT('Ctrl Pts',(59.406405003267,-7.27543664706474,-462.499999999987));
#33433=CARTESIAN_POINT('Ctrl Pts',(70.7822037837443,-6.95422428207083,-439.937224614869));
#33434=CARTESIAN_POINT('Ctrl Pts',(60.204044757483,-9.83061070349041,-462.499999999987));
#33435=CARTESIAN_POINT('Ctrl Pts',(71.4803706009395,-9.73514197376118,-439.927462314949));
#33436=CARTESIAN_POINT('Ctrl Pts',(60.2040447574833,-12.5073892965266,-462.499999999986));
#33437=CARTESIAN_POINT('Ctrl Pts',(71.4803706009397,-12.602858026249,-439.927462314949));
#33438=CARTESIAN_POINT('Ctrl Pts',(59.4064050032676,-15.0625633529524,-462.499999999986));
#33439=CARTESIAN_POINT('Ctrl Pts',(70.782203783745,-15.3837757179391,-439.937224614867));
#33440=CARTESIAN_POINT('',(59.406405003267,-7.27543664706474,-462.499999999987));
#33441=CARTESIAN_POINT('Origin',(54.2736315587506,-11.1690000000061,-438.999999999986));
#33442=CARTESIAN_POINT('Ctrl Pts',(70.7804124467082,-3.96116868056056,-438.999999999988));
#33443=CARTESIAN_POINT('Ctrl Pts',(70.7543859912015,-3.59775765571275,-438.999999999988));
#33444=CARTESIAN_POINT('Ctrl Pts',(70.7397309932481,-3.23363260618974,-438.999999999988));
#33445=CARTESIAN_POINT('Ctrl Pts',(70.7331966490285,-2.50342807144109,-438.999999999988));
#33446=CARTESIAN_POINT('Ctrl Pts',(70.7414162872563,-2.1375493135523,-438.999999999987));
#33447=CARTESIAN_POINT('Ctrl Pts',(70.7611151580477,-1.77218793995684,-438.999999999987));
#33448=CARTESIAN_POINT('Ctrl Pts',(59.0902650976006,-0.703506953302192,
-462.499999999988));
#33449=CARTESIAN_POINT('Ctrl Pts',(71.1815697946293,1.21523267184444,-439.002448983864));
#33450=CARTESIAN_POINT('Ctrl Pts',(58.630835273672,-2.8972250201618,-462.499999999987));
#33451=CARTESIAN_POINT('Ctrl Pts',(70.5610300866923,-1.48507116802909,-438.998910332348));
#33452=CARTESIAN_POINT('Ctrl Pts',(58.7385280596104,-5.13594719672545,-462.499999999987));
#33453=CARTESIAN_POINT('Ctrl Pts',(70.585395181528,-4.25176888548718,-438.998932713964));
#33454=CARTESIAN_POINT('Ctrl Pts',(59.406405003267,-7.27543664706474,-462.499999999987));
#33455=CARTESIAN_POINT('Ctrl Pts',(71.2535130610722,-6.94091617329225,-439.002429127846));
#33456=CARTESIAN_POINT('',(59.0902650976006,-0.703506953302192,-462.499999999987));
#33457=CARTESIAN_POINT('Ctrl Pts',(58.3152526334991,7.11256737781201,-462.499999999988));
#33458=CARTESIAN_POINT('Ctrl Pts',(70.5621815020404,9.72878593023445,-439.798062313337));
#33459=CARTESIAN_POINT('Ctrl Pts',(59.3774521833097,4.6287562350939,-462.499999999988));
#33460=CARTESIAN_POINT('Ctrl Pts',(71.353329194896,6.91847187717748,-439.789824991758));
#33461=CARTESIAN_POINT('Ctrl Pts',(59.6440060900465,1.94053476149611,-462.499999999987));
#33462=CARTESIAN_POINT('Ctrl Pts',(71.4248025866678,3.99812226802909,-439.789824991758));
#33463=CARTESIAN_POINT('Ctrl Pts',(59.0902650976006,-0.703506953302192,
-462.499999999988));
#33464=CARTESIAN_POINT('Ctrl Pts',(70.7709995585447,1.15008028336193,-439.800327733084));
#33465=CARTESIAN_POINT('',(58.3152526334991,7.11256737781201,-462.499999999988));
#33466=CARTESIAN_POINT('Ctrl Pts',(57.8729592854362,15.3392709400169,-462.499999999989));
#33467=CARTESIAN_POINT('Ctrl Pts',(71.5424551136857,19.4736998850754,-438.99999999999));
#33468=CARTESIAN_POINT('Ctrl Pts',(57.002852784826,12.4931127039992,-462.499999999989));
#33469=CARTESIAN_POINT('Ctrl Pts',(70.2493774538459,16.2681780209163,-439.002389441071));
#33470=CARTESIAN_POINT('Ctrl Pts',(57.2363227433815,9.63550017679799,-462.499999999989));
#33471=CARTESIAN_POINT('Ctrl Pts',(70.1312984442438,12.9284311565945,-438.996844362213));
#33472=CARTESIAN_POINT('Ctrl Pts',(58.3152526334991,7.11256737781201,-462.499999999988));
#33473=CARTESIAN_POINT('Ctrl Pts',(70.9913620171455,9.8204685094352,-439.002497203518));
#33474=CARTESIAN_POINT('Ctrl Pts',(52.7925979348309,27.7915710081813,-462.498943458995));
#33475=CARTESIAN_POINT('Ctrl Pts',(52.7792868797399,27.7708737286954,-462.523875928528));
#33476=CARTESIAN_POINT('Ctrl Pts',(54.7064708585553,25.7833181444813,-462.499999999991));
#33477=CARTESIAN_POINT('Ctrl Pts',(54.6916819141412,25.7649613214017,-462.524598036068));
#33478=CARTESIAN_POINT('Ctrl Pts',(56.0041009291211,23.3343857139696,-462.49999999999));
#33479=CARTESIAN_POINT('Ctrl Pts',(55.9886116147567,23.318620819518,-462.524598036068));
#33480=CARTESIAN_POINT('Ctrl Pts',(56.5915605594642,20.6258796622937,-462.49999999999));
#33481=CARTESIAN_POINT('Ctrl Pts',(56.5762638506312,20.6126509106678,-462.524933669083));
#33482=CARTESIAN_POINT('Ctrl Pts',(56.6115466725153,53.2965039304289,-440.982369050107));
#33483=CARTESIAN_POINT('Ctrl Pts',(56.597010807163,53.2869057865868,-441.00007767524));
#33484=CARTESIAN_POINT('Ctrl Pts',(56.6133279334121,53.2949358941234,-440.982368985934));
#33485=CARTESIAN_POINT('Ctrl Pts',(56.5987931490312,53.2853365991255,-441.000077624278));
#33486=CARTESIAN_POINT('Ctrl Pts',(56.6151091943089,53.2933678578181,-440.982368921762));
#33487=CARTESIAN_POINT('Ctrl Pts',(56.6005754908994,53.2837674116641,-441.000077573315));
#33488=CARTESIAN_POINT('Ctrl Pts',(56.6168904552057,53.2917998215128,-440.98236885759));
#33489=CARTESIAN_POINT('Ctrl Pts',(56.6023578327675,53.2821982242028,-441.000077522351));
#33490=CARTESIAN_POINT('Ctrl Pts',(59.3264760633801,50.9065632659512,-440.982271241517));
#33491=CARTESIAN_POINT('Ctrl Pts',(59.3135877730366,50.8952105744222,-440.999999999993));
#33492=CARTESIAN_POINT('Ctrl Pts',(61.8829281942602,48.3583918787876,-440.982271241516));
#33493=CARTESIAN_POINT('Ctrl Pts',(61.8717342174682,48.3453380510862,-440.999999999993));
#33494=CARTESIAN_POINT('Ctrl Pts',(64.2799598697074,45.6532009762712,-440.982369491764));
#33495=CARTESIAN_POINT('Ctrl Pts',(64.2705054959308,45.6385004273605,-441.000078147052));
#33496=CARTESIAN_POINT('Ctrl Pts',(64.2815357486139,45.6514225044533,-440.982369556356));
#33497=CARTESIAN_POINT('Ctrl Pts',(64.2720825185032,45.6367208729398,-441.000078198428));
#33498=CARTESIAN_POINT('Ctrl Pts',(64.2831116275205,45.6496440326354,-440.982369620949));
#33499=CARTESIAN_POINT('Ctrl Pts',(64.2736595410759,45.6349413185191,-441.000078249804));
#33500=CARTESIAN_POINT('Ctrl Pts',(64.2846875064269,45.6478655608175,-440.982369685541));
#33501=CARTESIAN_POINT('Ctrl Pts',(64.2752365636483,45.6331617640984,-441.000078301181));
#33502=CARTESIAN_POINT('Ctrl Pts',(64.2705054959311,45.6385004273602,-441.000078147052));
#33503=CARTESIAN_POINT('Ctrl Pts',(64.2132896438939,45.7032361413531,-440.999956345651));
#33504=CARTESIAN_POINT('Ctrl Pts',(64.1367868626771,45.789599828806,-440.999797014702));
#33505=CARTESIAN_POINT('Ctrl Pts',(63.9707562357255,45.9759636633542,-440.999470182454));
#33506=CARTESIAN_POINT('Ctrl Pts',(63.8955272911772,46.0600707364969,-440.99932802141));
#33507=CARTESIAN_POINT('Ctrl Pts',(63.6693479463854,46.3119401271007,-440.998918002061));
#33508=CARTESIAN_POINT('Ctrl Pts',(63.5179009198511,46.4792552858216,-440.998666591105));
#33509=CARTESIAN_POINT('Ctrl Pts',(63.061604480683,46.9793778842359,-440.9979756921));
#33510=CARTESIAN_POINT('Ctrl Pts',(62.7547855853059,47.3103786533786,-440.997599393785));
#33511=CARTESIAN_POINT('Ctrl Pts',(61.8266329871262,48.2959593976243,-440.99670763129));
#33512=CARTESIAN_POINT('Ctrl Pts',(61.1975600856359,48.9431704863275,-440.996427551129));
#33513=CARTESIAN_POINT('Ctrl Pts',(59.9186211802959,50.218080636068,-440.996452059618));
#33514=CARTESIAN_POINT('Ctrl Pts',(59.2688114468007,50.8456859164495,-440.996757235888));
#33515=CARTESIAN_POINT('Ctrl Pts',(58.2795110232487,51.7714152778138,-440.997659002473));
#33516=CARTESIAN_POINT('Ctrl Pts',(57.9473806255298,52.0773186454005,-440.99803387866));
#33517=CARTESIAN_POINT('Ctrl Pts',(57.4456133245308,52.5321901467099,-440.998711889762));
#33518=CARTESIAN_POINT('Ctrl Pts',(57.2777787398507,52.6831355444427,-440.998957173669));
#33519=CARTESIAN_POINT('Ctrl Pts',(57.0251433367402,52.9085499906903,-440.999354813187));
#33520=CARTESIAN_POINT('Ctrl Pts',(56.9407883129355,52.9835173208311,-440.9994923065));
#33521=CARTESIAN_POINT('Ctrl Pts',(56.8140360711639,53.0957164489069,-440.999706086766));
#33522=CARTESIAN_POINT('Ctrl Pts',(56.7717497004109,53.1330733071561,-440.999778601897));
#33523=CARTESIAN_POINT('Ctrl Pts',(56.6780978857083,53.2156432553775,-440.999941865624));
#33524=CARTESIAN_POINT('Ctrl Pts',(56.6347709042445,53.2537341362971,-441.00001916926));
#33525=CARTESIAN_POINT('Ctrl Pts',(56.6023578328018,53.2821982241729,-441.000077522351));
#33526=CARTESIAN_POINT('Ctrl Pts',(41.9546679377988,60.6647702916318,-440.977450556666));
#33527=CARTESIAN_POINT('Ctrl Pts',(41.9445347128706,60.6495679335285,-440.998916834174));
#33528=CARTESIAN_POINT('Ctrl Pts',(47.4212267268272,59.4923192195593,-440.97860778164));
#33529=CARTESIAN_POINT('Ctrl Pts',(47.4083864201783,59.4777499755747,-440.999999999994));
#33530=CARTESIAN_POINT('Ctrl Pts',(52.4160636430517,56.9796669347799,-440.97860778164));
#33531=CARTESIAN_POINT('Ctrl Pts',(52.4006927127278,56.9663054203067,-440.999999999994));
#33532=CARTESIAN_POINT('Ctrl Pts',(56.6199725617386,53.2938361467473,-440.978613169889));
#33533=CARTESIAN_POINT('Ctrl Pts',(56.6023578327675,53.2821982242028,-441.000077522351));
#33534=CARTESIAN_POINT('Ctrl Pts',(56.6023578327673,53.2821982242029,-441.000077522352));
#33535=CARTESIAN_POINT('Ctrl Pts',(54.630099851199,55.0143046797825,-440.997830128999));
#33536=CARTESIAN_POINT('Ctrl Pts',(52.4556758675906,56.5016643215144,-440.996476847209));
#33537=CARTESIAN_POINT('Ctrl Pts',(47.6685347341379,58.9889857335417,-440.994366068387));
#33538=CARTESIAN_POINT('Ctrl Pts',(45.0577394529488,59.947352817005,-440.993641905209));
#33539=CARTESIAN_POINT('Ctrl Pts',(42.2210187024469,60.5949101226765,-440.992100692275));
#33540=CARTESIAN_POINT('Ctrl Pts',(42.08451707017,60.6251470261161,-440.992024703487));
#33541=CARTESIAN_POINT('Ctrl Pts',(41.9478250221979,60.654504216007,-440.991946625419));
#33542=CARTESIAN_POINT('Origin',(0.583570446910677,-20.4591843142083,-487.927777712865));
#33543=CARTESIAN_POINT('',(33.4816044331148,62.276074524876,-440.9999972802));
#33544=CARTESIAN_POINT('Ctrl Pts',(18.8780323328947,47.6381153531325,-462.499937569615));
#33545=CARTESIAN_POINT('Ctrl Pts',(20.9284013294519,49.6296583969895,-459.596795658369));
#33546=CARTESIAN_POINT('Ctrl Pts',(22.9543862194209,51.628750133794,-456.668452986475));
#33547=CARTESIAN_POINT('Ctrl Pts',(27.8203525467718,56.4898863340891,-449.530713795769));
#33548=CARTESIAN_POINT('Ctrl Pts',(30.6950354236204,59.4116076064736,-445.226004279766));
#33549=CARTESIAN_POINT('Ctrl Pts',(33.4816127180597,62.2760728748087,-441.00000162475));
#33550=CARTESIAN_POINT('Ctrl Pts',(41.9449609251821,60.6486156188608,-441.000894783878));
#33551=CARTESIAN_POINT('Ctrl Pts',(39.1229463094741,61.2547168564534,-440.998260847152));
#33552=CARTESIAN_POINT('Ctrl Pts',(36.3000689160198,61.7969223748677,-440.998848881191));
#33553=CARTESIAN_POINT('Ctrl Pts',(33.4816044833662,62.2760748116437,-441.000000948612));
#33554=CARTESIAN_POINT('Origin',(29.9999999999753,83.0468894509273,-439.));
#33555=CARTESIAN_POINT('',(28.3882740955986,63.1097913591115,-438.999999999994));
#33556=CARTESIAN_POINT('',(26.1596537758254,63.4168994820682,-438.999999999994));
#33557=CARTESIAN_POINT('Origin',(-0.00176539235111073,-134.670997806539,
-438.999999999971));
#33558=CARTESIAN_POINT('Ctrl Pts',(28.3882740955984,63.1097913591091,-438.999999999998));
#33559=CARTESIAN_POINT('Ctrl Pts',(28.0150890543069,63.1396553617187,-438.999999999998));
#33560=CARTESIAN_POINT('Ctrl Pts',(27.6425418332694,63.1800897025264,-438.999999999998));
#33561=CARTESIAN_POINT('Ctrl Pts',(26.8985866816018,63.2826197832723,-438.999999999998));
#33562=CARTESIAN_POINT('Ctrl Pts',(26.528147392113,63.3445453679781,-438.999999999998));
#33563=CARTESIAN_POINT('Ctrl Pts',(26.1596537758248,63.4168994820655,-438.999999999998));
#33564=CARTESIAN_POINT('Ctrl Pts',(12.0088324072726,47.904965729667,-462.504463162543));
#33565=CARTESIAN_POINT('Ctrl Pts',(12.0109810190255,47.9080583287232,-462.499999999992));
#33566=CARTESIAN_POINT('Ctrl Pts',(23.3245997914203,64.1922877582739,-438.999002412958));
#33567=CARTESIAN_POINT('Ctrl Pts',(23.3284217331517,64.1977888607304,-438.991063357806));
#33568=CARTESIAN_POINT('Ctrl Pts',(12.0101894276276,47.9043018479569,-462.50446316207));
#33569=CARTESIAN_POINT('Ctrl Pts',(12.0123383942081,47.9073943572616,-462.499999999992));
#33570=CARTESIAN_POINT('Ctrl Pts',(23.3278255288872,64.1911511953027,-438.999004902713));
#33571=CARTESIAN_POINT('Ctrl Pts',(23.3316481017846,64.1966521381094,-438.991065848401));
#33572=CARTESIAN_POINT('Ctrl Pts',(12.0115464479826,47.9036379662469,-462.504463161597));
#33573=CARTESIAN_POINT('Ctrl Pts',(12.0136957693908,47.9067303858,-462.499999999992));
#33574=CARTESIAN_POINT('Ctrl Pts',(23.3310512663538,64.1900146323315,-438.999007392467));
#33575=CARTESIAN_POINT('Ctrl Pts',(23.3348744704173,64.1955154154884,-438.991068338997));
#33576=CARTESIAN_POINT('Ctrl Pts',(12.0129034683376,47.9029740845369,-462.504463161124));
#33577=CARTESIAN_POINT('Ctrl Pts',(12.0150531445734,47.9060664143383,-462.499999999992));
#33578=CARTESIAN_POINT('Ctrl Pts',(23.3342770038207,64.1888780693604,-438.999009882221));
#33579=CARTESIAN_POINT('Ctrl Pts',(23.3381008390501,64.1943786928674,-438.991070829592));
#33580=CARTESIAN_POINT('Ctrl Pts',(12.5525590984298,47.6389636728949,-462.504462973087));
#33581=CARTESIAN_POINT('Ctrl Pts',(12.554849881435,47.6420203105494,-462.499999999992));
#33582=CARTESIAN_POINT('Ctrl Pts',(24.6170782372489,63.7368932453292,-438.999999999994));
#33583=CARTESIAN_POINT('Ctrl Pts',(24.621153072618,63.7423303797924,-438.992061281844));
#33584=CARTESIAN_POINT('Ctrl Pts',(13.1531317256866,47.4164397049396,-462.504462963041));
#33585=CARTESIAN_POINT('Ctrl Pts',(13.1555740488351,47.4194722561805,-462.499999999992));
#33586=CARTESIAN_POINT('Ctrl Pts',(26.0157443355876,63.3875170188384,-439.000052901838));
#33587=CARTESIAN_POINT('Ctrl Pts',(26.0200887299393,63.3929113084884,-438.992114201559));
#33588=CARTESIAN_POINT('Ctrl Pts',(14.4571112437118,47.110317095545,-462.504462977168));
#33589=CARTESIAN_POINT('Ctrl Pts',(14.4598710640546,47.1133367987093,-462.499999999992));
#33590=CARTESIAN_POINT('Ctrl Pts',(28.9918381339846,63.0137293945006,-438.999978514899));
#33591=CARTESIAN_POINT('Ctrl Pts',(28.996747291037,63.0191008300449,-438.992039789491));
#33592=CARTESIAN_POINT('Ctrl Pts',(15.1606676247628,47.0274060982099,-462.504462973087));
#33593=CARTESIAN_POINT('Ctrl Pts',(15.1635931228085,47.0304369741072,-462.499999999992));
#33594=CARTESIAN_POINT('Ctrl Pts',(30.567944125466,62.9896601345561,-438.999999999994));
#33595=CARTESIAN_POINT('Ctrl Pts',(30.5731479893337,62.9950514441119,-438.992061281845));
#33596=CARTESIAN_POINT('Ctrl Pts',(16.619483413463,47.0519242799615,-462.504462973087));
#33597=CARTESIAN_POINT('Ctrl Pts',(16.622742373222,47.0550172977492,-462.499999999992));
#33598=CARTESIAN_POINT('Ctrl Pts',(33.7829521032227,63.3414515780021,-438.999999999994));
#33599=CARTESIAN_POINT('Ctrl Pts',(33.7887491274116,63.3469534252964,-438.992061281845));
#33600=CARTESIAN_POINT('Ctrl Pts',(17.3742915801458,47.1601346920495,-462.504462973087));
#33601=CARTESIAN_POINT('Ctrl Pts',(17.3777182257977,47.1632792121951,-462.499999999992));
#33602=CARTESIAN_POINT('Ctrl Pts',(35.4208861093652,63.7209016414656,-438.999999999994));
#33603=CARTESIAN_POINT('Ctrl Pts',(35.4269814125295,63.726495100942,-438.992061281845));
#33604=CARTESIAN_POINT('Ctrl Pts',(18.3703780276748,47.4490597509409,-462.504462973087));
#33605=CARTESIAN_POINT('Ctrl Pts',(18.374021594636,47.4523013789519,-462.499999999992));
#33606=CARTESIAN_POINT('Ctrl Pts',(37.5593990902821,64.5212499547191,-438.999999999994));
#33607=CARTESIAN_POINT('Ctrl Pts',(37.5658802521772,64.5270161492662,-438.992061281845));
#33608=CARTESIAN_POINT('Ctrl Pts',(18.6243186430052,47.5360060921983,-462.504462973087));
#33609=CARTESIAN_POINT('Ctrl Pts',(18.6280171263085,47.5392751251161,-462.499999999992));
#33610=CARTESIAN_POINT('Ctrl Pts',(38.1025592692013,64.7525255585329,-438.999999999994));
#33611=CARTESIAN_POINT('Ctrl Pts',(38.1091381160596,64.7583405008152,-438.992061281845));
#33612=CARTESIAN_POINT('Ctrl Pts',(18.8747298962646,47.6349689278609,-462.504462973087));
#33613=CARTESIAN_POINT('Ctrl Pts',(18.8784821989614,47.6382677383812,-462.499999999992));
#33614=CARTESIAN_POINT('Ctrl Pts',(38.6364129536412,65.0083135741065,-438.999999999994));
#33615=CARTESIAN_POINT('Ctrl Pts',(38.643087534215,65.0141814846656,-438.992061281845));
#33616=CARTESIAN_POINT('Ctrl Pts',(18.8758942609649,47.6354290862244,-462.504462973087));
#33617=CARTESIAN_POINT('Ctrl Pts',(18.8796468139118,47.6387280352049,-462.499999999992));
#33618=CARTESIAN_POINT('Ctrl Pts',(38.6388952717369,65.009502939729,-438.999999999994));
#33619=CARTESIAN_POINT('Ctrl Pts',(38.6455702974543,65.0153710965805,-438.992061281845));
#33620=CARTESIAN_POINT('Ctrl Pts',(18.8770586256651,47.6358892445878,-462.504462973087));
#33621=CARTESIAN_POINT('Ctrl Pts',(18.8808114288619,47.6391883320286,-462.499999999992));
#33622=CARTESIAN_POINT('Ctrl Pts',(38.6413775898324,65.0106923053514,-438.999999999994));
#33623=CARTESIAN_POINT('Ctrl Pts',(38.6480530606934,65.0165607084954,-438.992061281845));
#33624=CARTESIAN_POINT('Ctrl Pts',(18.8782229903656,47.6363494029513,-462.504462973087));
#33625=CARTESIAN_POINT('Ctrl Pts',(18.8819760438123,47.6396486288522,-462.499999999992));
#33626=CARTESIAN_POINT('Ctrl Pts',(38.643859907928,65.0118816709739,-438.999999999994));
#33627=CARTESIAN_POINT('Ctrl Pts',(38.6505358239326,65.0177503204103,-438.992061281845));
#33628=CARTESIAN_POINT('Ctrl Pts',(33.481598779729,62.2760760009175,-440.999988546436));
#33629=CARTESIAN_POINT('Ctrl Pts',(32.9601399465216,62.3726871929236,-440.550584444613));
#33630=CARTESIAN_POINT('Ctrl Pts',(32.2006722009084,62.5100376689964,-440.020332322067));
#33631=CARTESIAN_POINT('Ctrl Pts',(30.2339613237229,62.8331222144803,-439.276987649111));
#33632=CARTESIAN_POINT('Ctrl Pts',(29.3151615709777,62.9752775583384,-439.083114041147));
#33633=CARTESIAN_POINT('Ctrl Pts',(28.3882740955986,63.1097913591118,-438.999999999994));
#33634=CARTESIAN_POINT('',(23.0582397346304,63.7917958206442,-439.572118888214));
#33635=CARTESIAN_POINT('',(17.5310972153034,55.8409485053149,-451.047580752227));
#33636=CARTESIAN_POINT('Ctrl Pts',(26.1596537758254,63.4168994820685,-438.999999999994));
#33637=CARTESIAN_POINT('Ctrl Pts',(25.6361238202445,63.4852733932441,-439.043651690291));
#33638=CARTESIAN_POINT('Ctrl Pts',(25.113664820537,63.5508806641982,-439.115892043974));
#33639=CARTESIAN_POINT('Ctrl Pts',(23.8409192092728,63.7045947738492,-439.353351910025));
#33640=CARTESIAN_POINT('Ctrl Pts',(23.2599644625544,63.7693502441533,-439.515584934503));
#33641=CARTESIAN_POINT('Ctrl Pts',(23.0582397346378,63.7917958206654,-439.572118888232));
#33642=CARTESIAN_POINT('Ctrl Pts',(7.15508637657014,48.1002682270745,-462.548358098884));
#33643=CARTESIAN_POINT('Ctrl Pts',(7.16823209133649,48.1351541649005,-462.499999999992));
#33644=CARTESIAN_POINT('Ctrl Pts',(13.4012367324298,64.6762260078797,-439.571139897255));
#33645=CARTESIAN_POINT('Ctrl Pts',(13.4078662789118,64.6938194176329,-439.546752310115));
#33646=CARTESIAN_POINT('Ctrl Pts',(7.15842286648213,48.1015224334375,-462.548358080388));
#33647=CARTESIAN_POINT('Ctrl Pts',(7.17157638915753,48.1364081149888,-462.499999999992));
#33648=CARTESIAN_POINT('Ctrl Pts',(13.4082831289197,64.6773584460546,-439.571148667243));
#33649=CARTESIAN_POINT('Ctrl Pts',(13.4149166130267,64.6949517265655,-439.546761089431));
#33650=CARTESIAN_POINT('Ctrl Pts',(7.16175935639413,48.1027766398004,-462.548358061891));
#33651=CARTESIAN_POINT('Ctrl Pts',(7.17492068697853,48.1376620650771,-462.499999999992));
#33652=CARTESIAN_POINT('Ctrl Pts',(13.4153295254096,64.6784908842296,-439.571157437231));
#33653=CARTESIAN_POINT('Ctrl Pts',(13.4219669471417,64.6960840354981,-439.546769868747));
#33654=CARTESIAN_POINT('Ctrl Pts',(7.16509584630612,48.1040308461633,-462.548358043395));
#33655=CARTESIAN_POINT('Ctrl Pts',(7.17826498479954,48.1389160151653,-462.499999999992));
#33656=CARTESIAN_POINT('Ctrl Pts',(13.4223759218995,64.6796233224046,-439.571166207219));
#33657=CARTESIAN_POINT('Ctrl Pts',(13.4290172812566,64.6972163444305,-439.546778648063));
#33658=CARTESIAN_POINT('Ctrl Pts',(7.54205893122661,48.2457335073907,-462.548355953643));
#33659=CARTESIAN_POINT('Ctrl Pts',(7.55611022238567,48.2805897219893,-462.499999999992));
#33660=CARTESIAN_POINT('Ctrl Pts',(14.2184914290542,64.8075683781938,-439.572157057449));
#33661=CARTESIAN_POINT('Ctrl Pts',(14.225577668907,64.8251467981561,-439.547770552181));
#33662=CARTESIAN_POINT('Ctrl Pts',(7.94106123049321,48.3526724298479,-462.548355953643));
#33663=CARTESIAN_POINT('Ctrl Pts',(7.95597858418204,48.3874670903331,-462.499999999992));
#33664=CARTESIAN_POINT('Ctrl Pts',(15.0290009665914,64.8852600322751,-439.572157057449));
#33665=CARTESIAN_POINT('Ctrl Pts',(15.0365239724854,64.902807409737,-439.547770552181));
#33666=CARTESIAN_POINT('Ctrl Pts',(8.76160672396958,48.4833667221507,-462.548355953643));
#33667=CARTESIAN_POINT('Ctrl Pts',(8.77822932150332,48.5180010759625,-462.499999999992));
#33668=CARTESIAN_POINT('Ctrl Pts',(16.6597884011092,64.9397850479198,-439.572157057449));
#33669=CARTESIAN_POINT('Ctrl Pts',(16.6681713825567,64.9572515807444,-439.547770552181));
#33670=CARTESIAN_POINT('Ctrl Pts',(9.18299691544561,48.5070252542725,-462.548355953643));
#33671=CARTESIAN_POINT('Ctrl Pts',(9.20045900848171,48.5415610543782,-462.499999999992));
#33672=CARTESIAN_POINT('Ctrl Pts',(17.4800625805652,64.9166160566062,-439.572157057449));
#33673=CARTESIAN_POINT('Ctrl Pts',(17.4888689299737,64.9340328875783,-439.547770552181));
#33674=CARTESIAN_POINT('Ctrl Pts',(10.0217589312659,48.4668037795237,-462.548355953643));
#33675=CARTESIAN_POINT('Ctrl Pts',(10.0408892417922,48.5011082063693,-462.499999999992));
#33676=CARTESIAN_POINT('Ctrl Pts',(19.1114735664401,64.7664582111772,-439.572157057449));
#33677=CARTESIAN_POINT('Ctrl Pts',(19.1211212185536,64.7837583577536,-439.547770552181));
#33678=CARTESIAN_POINT('Ctrl Pts',(10.4389441100322,48.4029194680995,-462.548355953643));
#33679=CARTESIAN_POINT('Ctrl Pts',(10.4589027392674,48.4370911577441,-462.499999999992));
#33680=CARTESIAN_POINT('Ctrl Pts',(19.9222321103595,64.6395041823741,-439.572157057449));
#33681=CARTESIAN_POINT('Ctrl Pts',(19.9322974938387,64.6567373879391,-439.547770552181));
#33682=CARTESIAN_POINT('Ctrl Pts',(11.2431920479856,48.194304008609,-462.548355953643));
#33683=CARTESIAN_POINT('Ctrl Pts',(11.2648118978999,48.2281753266975,-462.499999999992));
#33684=CARTESIAN_POINT('Ctrl Pts',(21.5158045027278,64.288168000919,-439.572157057449));
#33685=CARTESIAN_POINT('Ctrl Pts',(21.5267076603337,64.3052497253947,-439.547770552181));
#33686=CARTESIAN_POINT('Ctrl Pts',(11.6301113843655,48.0496773411552,-462.548355953643));
#33687=CARTESIAN_POINT('Ctrl Pts',(11.6525644307871,48.0833808106781,-462.499999999992));
#33688=CARTESIAN_POINT('Ctrl Pts',(22.2986148768613,64.063788547369,-439.572157057449));
#33689=CARTESIAN_POINT('Ctrl Pts',(22.309938225767,64.0807856237378,-439.547770552181));
#33690=CARTESIAN_POINT('Ctrl Pts',(11.9917615758797,47.8725612702661,-462.548357991009));
#33691=CARTESIAN_POINT('Ctrl Pts',(12.0150531445734,47.9060664143383,-462.499999999992));
#33692=CARTESIAN_POINT('Ctrl Pts',(23.0586866286725,63.7924386819717,-439.571191046182));
#33693=CARTESIAN_POINT('Ctrl Pts',(23.0704328547269,63.8093357403638,-439.546803513444));
#33694=CARTESIAN_POINT('Ctrl Pts',(11.9948085870571,47.8710690143228,-462.548358008174));
#33695=CARTESIAN_POINT('Ctrl Pts',(12.0181072205521,47.9045724874437,-462.499999999992));
#33696=CARTESIAN_POINT('Ctrl Pts',(23.0650904608222,63.7901524780867,-439.571182907248));
#33697=CARTESIAN_POINT('Ctrl Pts',(23.0768402497433,63.8070486937973,-439.546795365853));
#33698=CARTESIAN_POINT('Ctrl Pts',(11.9978555982345,47.8695767583794,-462.548358025339));
#33699=CARTESIAN_POINT('Ctrl Pts',(12.0211612965308,47.903078560549,-462.499999999992));
#33700=CARTESIAN_POINT('Ctrl Pts',(23.0714942929719,63.7878662742018,-439.571174768313));
#33701=CARTESIAN_POINT('Ctrl Pts',(23.0832476447597,63.804761647231,-439.546787218263));
#33702=CARTESIAN_POINT('Ctrl Pts',(12.0009026094119,47.8680845024361,-462.548358042505));
#33703=CARTESIAN_POINT('Ctrl Pts',(12.0242153725094,47.9015846336544,-462.499999999992));
#33704=CARTESIAN_POINT('Ctrl Pts',(23.0778981251217,63.7855800703168,-439.571166629379));
#33705=CARTESIAN_POINT('Ctrl Pts',(23.0896550397761,63.8024746006646,-439.546779070672));
#33706=CARTESIAN_POINT('',(13.4208374317807,64.67554784793,-439.576815655849));
#33707=CARTESIAN_POINT('',(10.3755396625017,56.6085260457139,-450.759372645136));
#33708=CARTESIAN_POINT('Ctrl Pts',(23.0582397346381,63.7917958206654,-439.572118888233));
#33709=CARTESIAN_POINT('Ctrl Pts',(22.4761301356798,63.8565139964938,-439.738227128177));
#33710=CARTESIAN_POINT('Ctrl Pts',(20.5413879799313,64.0689664196242,-440.29417568351));
#33711=CARTESIAN_POINT('Ctrl Pts',(15.6870770962244,64.5124744893397,-440.37072762596));
#33712=CARTESIAN_POINT('Ctrl Pts',(13.9510385373826,64.6366301639263,-439.760738129923));
#33713=CARTESIAN_POINT('Ctrl Pts',(13.4208374317689,64.6755478479304,-439.576815655883));
#33714=CARTESIAN_POINT('Origin',(29.9999999999753,83.0468894509273,-439.));
#33715=CARTESIAN_POINT('',(10.6589034715959,64.8523969232218,-438.999999999994));
#33716=CARTESIAN_POINT('',(8.41281223346166,64.9597357704683,-438.999999999994));
#33717=CARTESIAN_POINT('Origin',(-0.00176539235111073,-134.670997806539,
-438.999999999971));
#33718=CARTESIAN_POINT('Ctrl Pts',(10.6589034715959,64.852396923219,-438.999999999998));
#33719=CARTESIAN_POINT('Ctrl Pts',(10.2791741653356,64.850135258153,-438.999999999998));
#33720=CARTESIAN_POINT('Ctrl Pts',(9.88830466079304,64.8595052145251,-438.999999999997));
#33721=CARTESIAN_POINT('Ctrl Pts',(9.15135256034744,64.8946619872636,-438.999999999997));
#33722=CARTESIAN_POINT('Ctrl Pts',(8.78144427771419,64.921756709229,-438.999999999998));
#33723=CARTESIAN_POINT('Ctrl Pts',(8.41281223346138,64.9597357704656,-438.999999999998));
#33724=CARTESIAN_POINT('Ctrl Pts',(2.49780576443942,48.2570143438195,-462.551779730762));
#33725=CARTESIAN_POINT('Ctrl Pts',(2.50499543252761,48.2947401420713,-462.499999999992));
#33726=CARTESIAN_POINT('Ctrl Pts',(5.76813712223451,65.4171752173726,-438.998971011752));
#33727=CARTESIAN_POINT('Ctrl Pts',(5.77258297236757,65.4405035884631,-438.966952159128));
#33728=CARTESIAN_POINT('Ctrl Pts',(2.50114805249965,48.2555045618294,-462.551779709936));
#33729=CARTESIAN_POINT('Ctrl Pts',(2.50834348888334,48.2932305351486,-462.499999999992));
#33730=CARTESIAN_POINT('Ctrl Pts',(5.77410320843019,65.4157450675561,-438.998980463695));
#33731=CARTESIAN_POINT('Ctrl Pts',(5.77855262548419,65.4390735469024,-438.966961623949));
#33732=CARTESIAN_POINT('Ctrl Pts',(2.50449034055988,48.253994779839,-462.551779689111));
#33733=CARTESIAN_POINT('Ctrl Pts',(2.51169154523912,48.2917209282259,-462.499999999992));
#33734=CARTESIAN_POINT('Ctrl Pts',(5.78006929462591,65.4143149177398,-438.998989915638));
#33735=CARTESIAN_POINT('Ctrl Pts',(5.7845222786008,65.4376435053419,-438.966971088769));
#33736=CARTESIAN_POINT('Ctrl Pts',(2.50783262862012,48.2524849978489,-462.551779668285));
#33737=CARTESIAN_POINT('Ctrl Pts',(2.51503960159485,48.2902113213033,-462.499999999992));
#33738=CARTESIAN_POINT('Ctrl Pts',(5.78603538082159,65.4128847679232,-438.99899936758));
#33739=CARTESIAN_POINT('Ctrl Pts',(5.79049193171741,65.4362134637813,-438.966980553589));
#33740=CARTESIAN_POINT('Ctrl Pts',(2.86166483944225,48.0926515275304,-462.551777463596));
#33741=CARTESIAN_POINT('Ctrl Pts',(2.86948247455032,48.1303963845574,-462.499999999992));
#33742=CARTESIAN_POINT('Ctrl Pts',(6.41763667626308,65.2614815787759,-438.999999999994));
#33743=CARTESIAN_POINT('Ctrl Pts',(6.42247084018541,65.2848217351751,-438.967982549309));
#33744=CARTESIAN_POINT('Ctrl Pts',(3.23771592613298,47.963840025296,-462.551777463596));
#33745=CARTESIAN_POINT('Ctrl Pts',(3.24611879784553,48.001598882328,-462.499999999992));
#33746=CARTESIAN_POINT('Ctrl Pts',(7.05989165386403,65.1390381946537,-438.999999999994));
#33747=CARTESIAN_POINT('Ctrl Pts',(7.0650877085168,65.1623870081876,-438.967982549309));
#33748=CARTESIAN_POINT('Ctrl Pts',(4.01580172662955,47.7814773668558,-462.551777463596));
#33749=CARTESIAN_POINT('Ctrl Pts',(4.02534345872193,47.8192291909888,-462.499999999992));
#33750=CARTESIAN_POINT('Ctrl Pts',(8.35600565353464,64.9534765136393,-438.999999999994));
#33751=CARTESIAN_POINT('Ctrl Pts',(8.36190594133271,64.9768209782635,-438.967982549309));
#33752=CARTESIAN_POINT('Ctrl Pts',(4.41771393105522,47.7279968672351,-462.551777463596));
#33753=CARTESIAN_POINT('Ctrl Pts',(4.42781120502764,47.7657432867869,-462.499999999992));
#33754=CARTESIAN_POINT('Ctrl Pts',(9.01061464568725,64.8975376569562,-438.999999999994));
#33755=CARTESIAN_POINT('Ctrl Pts',(9.01685846199188,64.9208787795684,-438.967982549309));
#33756=CARTESIAN_POINT('Ctrl Pts',(5.22431302604201,47.7018523564368,-462.551777463596));
#33757=CARTESIAN_POINT('Ctrl Pts',(5.23551978937467,47.7395377085665,-462.499999999992));
#33758=CARTESIAN_POINT('Ctrl Pts',(10.321882078837,64.8436156878735,-438.999999999994));
#33759=CARTESIAN_POINT('Ctrl Pts',(10.3288119662314,64.8669190484356,-438.967982549309));
#33760=CARTESIAN_POINT('Ctrl Pts',(5.62884640341604,47.7291960960751,-462.551777463596));
#33761=CARTESIAN_POINT('Ctrl Pts',(5.6406081038935,47.7668229830741,-462.499999999992));
#33762=CARTESIAN_POINT('Ctrl Pts',(10.9788371708056,64.8443656615973,-438.999999999994));
#33763=CARTESIAN_POINT('Ctrl Pts',(10.9861102127585,64.8676328692792,-438.967982549309));
#33764=CARTESIAN_POINT('Ctrl Pts',(6.41711316528365,47.8607864731195,-462.551777463596));
#33765=CARTESIAN_POINT('Ctrl Pts',(6.43001529825674,47.8982994369536,-462.499999999992));
#33766=CARTESIAN_POINT('Ctrl Pts',(12.2858472329501,64.9241363309766,-438.999999999994));
#33767=CARTESIAN_POINT('Ctrl Pts',(12.2938254801921,64.947333092386,-438.967982549309));
#33768=CARTESIAN_POINT('Ctrl Pts',(6.80072015482547,47.9649760744569,-462.551777463596));
#33769=CARTESIAN_POINT('Ctrl Pts',(6.8142082474083,48.0024123296618,-462.499999999992));
#33770=CARTESIAN_POINT('Ctrl Pts',(12.9359869834827,64.9934338298192,-438.999999999994));
#33771=CARTESIAN_POINT('Ctrl Pts',(12.9443275685373,65.0165831571792,-438.967982549309));
#33772=CARTESIAN_POINT('Ctrl Pts',(7.16416404091255,48.1015624851047,-462.551779701212));
#33773=CARTESIAN_POINT('Ctrl Pts',(7.17826498479954,48.1389160151653,-462.499999999992));
#33774=CARTESIAN_POINT('Ctrl Pts',(13.5781957322997,65.0923914334237,-438.998984423411));
#33775=CARTESIAN_POINT('Ctrl Pts',(13.5869152840909,65.1154896063231,-438.966965589059));
#33776=CARTESIAN_POINT('Ctrl Pts',(7.1675971205597,48.1028526760927,-462.551779722348));
#33777=CARTESIAN_POINT('Ctrl Pts',(7.18170385342104,48.1402054247342,-462.499999999992));
#33778=CARTESIAN_POINT('Ctrl Pts',(13.5842620161724,65.0933261838704,-438.998974830306));
#33779=CARTESIAN_POINT('Ctrl Pts',(13.5929851476715,65.1164238735664,-438.966955982884));
#33780=CARTESIAN_POINT('Ctrl Pts',(7.17103020020685,48.1041428670807,-462.551779743485));
#33781=CARTESIAN_POINT('Ctrl Pts',(7.18514272204257,48.1414948343031,-462.499999999992));
#33782=CARTESIAN_POINT('Ctrl Pts',(13.5903283000451,65.0942609343171,-438.998965237201));
#33783=CARTESIAN_POINT('Ctrl Pts',(13.5990550112522,65.1173581408096,-438.966946376709));
#33784=CARTESIAN_POINT('Ctrl Pts',(7.17446327985399,48.1054330580687,-462.551779764621));
#33785=CARTESIAN_POINT('Ctrl Pts',(7.18858159066407,48.1427842438719,-462.499999999992));
#33786=CARTESIAN_POINT('Ctrl Pts',(13.5963945839176,65.0951956847637,-438.998955644096));
#33787=CARTESIAN_POINT('Ctrl Pts',(13.6051248748329,65.1182924080529,-438.966936770534));
#33788=CARTESIAN_POINT('',(5.71602529916582,65.0464031681007,-439.501998174119));
#33789=CARTESIAN_POINT('',(4.11418572738962,56.6612575572247,-451.010674837211));
#33790=CARTESIAN_POINT('Ctrl Pts',(8.41281223346166,64.9597357704684,-438.999999999994));
#33791=CARTESIAN_POINT('Ctrl Pts',(8.00411492382587,64.9763677702042,-439.034050589004));
#33792=CARTESIAN_POINT('Ctrl Pts',(7.55093882802567,64.9931974319874,-439.093081656777));
#33793=CARTESIAN_POINT('Ctrl Pts',(6.38200340706734,65.0306627918092,-439.312440980534));
#33794=CARTESIAN_POINT('Ctrl Pts',(5.8858057335339,65.0423882666263,-439.453561504873));
#33795=CARTESIAN_POINT('Ctrl Pts',(5.71602529917806,65.0464031680998,-439.501998174162));
#33796=CARTESIAN_POINT('Ctrl Pts',(13.4208374317689,64.6755478479304,-439.576815655884));
#33797=CARTESIAN_POINT('Ctrl Pts',(13.1739140243162,64.6936335881493,-439.493381620575));
#33798=CARTESIAN_POINT('Ctrl Pts',(12.7545818536148,64.7244359742643,-439.352615648631));
#33799=CARTESIAN_POINT('Ctrl Pts',(11.6032651386067,64.7982807678147,-439.110697841396));
#33800=CARTESIAN_POINT('Ctrl Pts',(11.1446275207669,64.8257325793285,-439.040719881605));
#33801=CARTESIAN_POINT('Ctrl Pts',(10.658903471596,64.8523969232225,-438.999999999993));
#33802=CARTESIAN_POINT('Ctrl Pts',(-2.51803865109287,48.2556786139059,-462.541918531101));
#33803=CARTESIAN_POINT('Ctrl Pts',(-2.52389605211168,48.286218031592,-462.499999999992));
#33804=CARTESIAN_POINT('Ctrl Pts',(-5.7376033488292,65.0419001405148,-439.501081391007));
#33805=CARTESIAN_POINT('Ctrl Pts',(-5.74062486656665,65.0576537814102,-439.479457878315));
#33806=CARTESIAN_POINT('Ctrl Pts',(-2.51509415222326,48.2570089424155,-462.541918517992));
#33807=CARTESIAN_POINT('Ctrl Pts',(-2.52094390194258,48.2875491281623,-462.499999999992));
#33808=CARTESIAN_POINT('Ctrl Pts',(-5.73045325541913,65.0436526393717,-439.501088582933));
#33809=CARTESIAN_POINT('Ctrl Pts',(-5.73347082626322,65.0594066764682,-439.479465077003));
#33810=CARTESIAN_POINT('Ctrl Pts',(-2.51214965335364,48.2583392709251,-462.541918504884));
#33811=CARTESIAN_POINT('Ctrl Pts',(-2.51799175177345,48.2888802247325,-462.499999999992));
#33812=CARTESIAN_POINT('Ctrl Pts',(-5.72330316200906,65.0454051382286,-439.50109577486));
#33813=CARTESIAN_POINT('Ctrl Pts',(-5.72631678595981,65.0611595715262,-439.479472275692));
#33814=CARTESIAN_POINT('Ctrl Pts',(-2.50920515448402,48.2596695994346,-462.541918491776));
#33815=CARTESIAN_POINT('Ctrl Pts',(-2.51503960160435,48.2902113213028,-462.499999999992));
#33816=CARTESIAN_POINT('Ctrl Pts',(-5.71615306859899,65.0471576370855,-439.501102966786));
#33817=CARTESIAN_POINT('Ctrl Pts',(-5.7191627456564,65.0629124665843,-439.47947947438));
#33818=CARTESIAN_POINT('Ctrl Pts',(-2.12806987109674,48.4318670279101,-462.54191679505));
#33819=CARTESIAN_POINT('Ctrl Pts',(-2.1329139357002,48.4625081673819,-462.499999999992));
#33820=CARTESIAN_POINT('Ctrl Pts',(-4.79064655670577,65.2740007020806,-439.502033888159));
#33821=CARTESIAN_POINT('Ctrl Pts',(-4.79314534875941,65.2898068157669,-439.480411271002));
#33822=CARTESIAN_POINT('Ctrl Pts',(-1.72039652650194,48.5683071422839,-462.54191679505));
#33823=CARTESIAN_POINT('Ctrl Pts',(-1.72426166237677,48.5990124033193,-462.499999999992));
#33824=CARTESIAN_POINT('Ctrl Pts',(-3.84489764477392,65.4456857180531,-439.502033888159));
#33825=CARTESIAN_POINT('Ctrl Pts',(-3.8468914602163,65.4615249086009,-439.480411271002));
#33826=CARTESIAN_POINT('Ctrl Pts',(-0.875068093851045,48.7525347307723,
-462.54191679505));
#33827=CARTESIAN_POINT('Ctrl Pts',(-0.876992489635159,48.7833242476379,
-462.499999999992));
#33828=CARTESIAN_POINT('Ctrl Pts',(-1.93282676721124,65.6762251597991,-439.502033888159));
#33829=CARTESIAN_POINT('Ctrl Pts',(-1.93381945935864,65.6921078133922,-439.480411271002));
#33830=CARTESIAN_POINT('Ctrl Pts',(-0.437591237771207,48.8001901136637,
-462.54191679505));
#33831=CARTESIAN_POINT('Ctrl Pts',(-0.43855350484806,48.8309999999866,-462.499999999992));
#33832=CARTESIAN_POINT('Ctrl Pts',(-0.966508602396304,65.7350767687133,
-439.502033888159));
#33833=CARTESIAN_POINT('Ctrl Pts',(-0.96700498415872,65.7509699298123,-439.480411271002));
#33834=CARTESIAN_POINT('Ctrl Pts',(0.437591237761631,48.8001901136638,-462.54191679505));
#33835=CARTESIAN_POINT('Ctrl Pts',(0.438553504838485,48.8309999999867,-462.499999999992));
#33836=CARTESIAN_POINT('Ctrl Pts',(0.966508602384286,65.7350767687136,-439.502033888159));
#33837=CARTESIAN_POINT('Ctrl Pts',(0.967004984146674,65.7509699298127,-439.480411271002));
#33838=CARTESIAN_POINT('Ctrl Pts',(0.875068093841497,48.7525347307725,-462.54191679505));
#33839=CARTESIAN_POINT('Ctrl Pts',(0.876992489625583,48.7833242476381,-462.499999999992));
#33840=CARTESIAN_POINT('Ctrl Pts',(1.93282676719919,65.6762251597994,-439.502033888159));
#33841=CARTESIAN_POINT('Ctrl Pts',(1.93381945934659,65.6921078133925,-439.480411271002));
#33842=CARTESIAN_POINT('Ctrl Pts',(1.72039652649242,48.5683071422842,-462.54191679505));
#33843=CARTESIAN_POINT('Ctrl Pts',(1.72426166236725,48.5990124033196,-462.499999999992));
#33844=CARTESIAN_POINT('Ctrl Pts',(3.84489764476192,65.4456857180537,-439.502033888159));
#33845=CARTESIAN_POINT('Ctrl Pts',(3.84689146020431,65.4615249086015,-439.480411271002));
#33846=CARTESIAN_POINT('Ctrl Pts',(2.12806987108721,48.4318670279105,-462.54191679505));
#33847=CARTESIAN_POINT('Ctrl Pts',(2.1329139356907,48.4625081673823,-462.499999999992));
#33848=CARTESIAN_POINT('Ctrl Pts',(4.79064655669381,65.2740007020815,-439.502033888159));
#33849=CARTESIAN_POINT('Ctrl Pts',(4.79314534874745,65.2898068157678,-439.480411271002));
#33850=CARTESIAN_POINT('Ctrl Pts',(2.50920514799,48.2596697215709,-462.541918579872));
#33851=CARTESIAN_POINT('Ctrl Pts',(2.51503960159485,48.2902113213033,-462.499999999992));
#33852=CARTESIAN_POINT('Ctrl Pts',(5.71615662638683,65.0470906263832,-439.5010546324));
#33853=CARTESIAN_POINT('Ctrl Pts',(5.71916630678926,65.0628453928787,-439.47943109455));
#33854=CARTESIAN_POINT('Ctrl Pts',(2.5120017951438,48.2584061935381,-462.541918592968));
#33855=CARTESIAN_POINT('Ctrl Pts',(2.51784351590223,48.2889470628801,-462.499999999992));
#33856=CARTESIAN_POINT('Ctrl Pts',(5.72294771936374,65.0454256337786,-439.501047446939));
#33857=CARTESIAN_POINT('Ctrl Pts',(5.72596114849933,65.0611800235051,-439.479423902333));
#33858=CARTESIAN_POINT('Ctrl Pts',(2.51479844229763,48.2571426655051,-462.541918606065));
#33859=CARTESIAN_POINT('Ctrl Pts',(2.52064743020961,48.2876828044569,-462.499999999992));
#33860=CARTESIAN_POINT('Ctrl Pts',(5.72973881234068,65.0437606411741,-439.501040261477));
#33861=CARTESIAN_POINT('Ctrl Pts',(5.73275599020939,65.0595146541315,-439.479416710115));
#33862=CARTESIAN_POINT('Ctrl Pts',(2.51759508945143,48.2558791374724,-462.541918619161));
#33863=CARTESIAN_POINT('Ctrl Pts',(2.52345134451698,48.2864185460337,-462.499999999992));
#33864=CARTESIAN_POINT('Ctrl Pts',(5.73652990531762,65.0420956485695,-439.501033076016));
#33865=CARTESIAN_POINT('Ctrl Pts',(5.73955083191949,65.0578492847579,-439.479409517898));
#33866=CARTESIAN_POINT('',(-5.71602822336162,65.0465041066898,-439.501999936783));
#33867=CARTESIAN_POINT('',(-4.14907673705054,56.8439451514172,-450.760006334025));
#33868=CARTESIAN_POINT('Ctrl Pts',(5.71602529917836,65.0464031680999,-439.501998174162));
#33869=CARTESIAN_POINT('Ctrl Pts',(5.03832061887466,65.0623545154082,-439.699621167922));
#33870=CARTESIAN_POINT('Ctrl Pts',(2.84424303022636,65.1134462912443,-440.347752071002));
#33871=CARTESIAN_POINT('Ctrl Pts',(-2.84329574129294,65.1134990067166,-440.347698281527));
#33872=CARTESIAN_POINT('Ctrl Pts',(-5.03709134550615,65.0624738964574,-439.699899735949));
#33873=CARTESIAN_POINT('Ctrl Pts',(-5.71602822336464,65.0465041066898,-439.501999936793));
#33874=CARTESIAN_POINT('Origin',(29.9999999999753,83.0468894509273,-439.));
#33875=CARTESIAN_POINT('',(-8.41281803607202,64.9598843197978,-438.999999999994));
#33876=CARTESIAN_POINT('',(-10.6587895159293,64.8525916307611,-438.999999999994));
#33877=CARTESIAN_POINT('Origin',(-0.00176539235111073,-134.670997806539,
-438.999999999971));
#33878=CARTESIAN_POINT('Ctrl Pts',(-8.41281803607176,64.9598843197952,-438.999999999998));
#33879=CARTESIAN_POINT('Ctrl Pts',(-8.78383622403301,64.9216210322276,-438.999999999998));
#33880=CARTESIAN_POINT('Ctrl Pts',(-9.15614215981989,64.8943339071276,-438.999999999998));
#33881=CARTESIAN_POINT('Ctrl Pts',(-9.89456730134841,64.8593136998998,-438.999999999998));
#33882=CARTESIAN_POINT('Ctrl Pts',(-10.2814664621786,64.8502517844627,-438.999999999998));
#33883=CARTESIAN_POINT('Ctrl Pts',(-10.6587895159293,64.8525916307586,-438.999999999998));
#33884=CARTESIAN_POINT('Ctrl Pts',(-7.17446331057034,48.1054326881418,-462.551779506093));
#33885=CARTESIAN_POINT('Ctrl Pts',(-7.18858159067015,48.1427842438694,-462.499999999992));
#33886=CARTESIAN_POINT('Ctrl Pts',(-13.5963806453087,65.0953635799082,-438.999072982214));
#33887=CARTESIAN_POINT('Ctrl Pts',(-13.6047828789584,65.1175926684504,-438.968257365478));
#33888=CARTESIAN_POINT('Ctrl Pts',(-7.1710302306422,48.1041425005522,-462.551779487331));
#33889=CARTESIAN_POINT('Ctrl Pts',(-7.18514272204976,48.1414948343009,-462.499999999992));
#33890=CARTESIAN_POINT('Ctrl Pts',(-13.5903144894735,65.0944272872329,-438.99908149749));
#33891=CARTESIAN_POINT('Ctrl Pts',(-13.5987132780899,65.1166568388001,-438.96826589192));
#33892=CARTESIAN_POINT('Ctrl Pts',(-7.16759715071408,48.1028523129626,-462.551779468569));
#33893=CARTESIAN_POINT('Ctrl Pts',(-7.18170385342937,48.1402054247325,-462.499999999992));
#33894=CARTESIAN_POINT('Ctrl Pts',(-13.5842483336382,65.0934909945578,-438.999090012766));
#33895=CARTESIAN_POINT('Ctrl Pts',(-13.5926436772213,65.1157210091498,-438.968274418361));
#33896=CARTESIAN_POINT('Ctrl Pts',(-7.16416407078593,48.101562125373,-462.551779449808));
#33897=CARTESIAN_POINT('Ctrl Pts',(-7.17826498480897,48.138916015164,-462.499999999992));
#33898=CARTESIAN_POINT('Ctrl Pts',(-13.578182177803,65.0925547018826,-438.999098528042));
#33899=CARTESIAN_POINT('Ctrl Pts',(-13.5865740763529,65.1147851794995,-438.968282944803));
#33900=CARTESIAN_POINT('Ctrl Pts',(-6.80072015483429,47.9649760744541,-462.551777463598));
#33901=CARTESIAN_POINT('Ctrl Pts',(-6.81420824741771,48.0024123296606,-462.499999999992));
#33902=CARTESIAN_POINT('Ctrl Pts',(-12.9359869834945,64.9934338298169,-438.999999999994));
#33903=CARTESIAN_POINT('Ctrl Pts',(-12.9440141726828,65.0157133256896,-438.969185598811));
#33904=CARTESIAN_POINT('Ctrl Pts',(-6.41711316529248,47.8607864731167,-462.551777463598));
#33905=CARTESIAN_POINT('Ctrl Pts',(-6.43001529826615,47.8982994369525,-462.499999999992));
#33906=CARTESIAN_POINT('Ctrl Pts',(-12.2858472329619,64.9241363309746,-438.999999999994));
#33907=CARTESIAN_POINT('Ctrl Pts',(-12.2935256991105,64.9464614785712,-438.969185598811));
#33908=CARTESIAN_POINT('Ctrl Pts',(-5.62884641196265,47.7291951231673,-462.551777463598));
#33909=CARTESIAN_POINT('Ctrl Pts',(-5.64060810390288,47.7668229830731,-462.499999999992));
#33910=CARTESIAN_POINT('Ctrl Pts',(-10.9788332958342,64.844807229598,-438.999999999994));
#33911=CARTESIAN_POINT('Ctrl Pts',(-10.9858330495647,64.8672007554688,-438.969185598811));
#33912=CARTESIAN_POINT('Ctrl Pts',(-5.22431302605086,47.7018523564343,-462.551777463598));
#33913=CARTESIAN_POINT('Ctrl Pts',(-5.23551978938402,47.7395377085656,-462.499999999992));
#33914=CARTESIAN_POINT('Ctrl Pts',(-10.3218820788488,64.8436156878717,-438.999999999994));
#33915=CARTESIAN_POINT('Ctrl Pts',(-10.3285515770679,64.8660434291788,-438.969185598811));
#33916=CARTESIAN_POINT('Ctrl Pts',(-4.41771393106416,47.7279968672327,-462.551777463598));
#33917=CARTESIAN_POINT('Ctrl Pts',(-4.42781120503702,47.7657432867861,-462.499999999992));
#33918=CARTESIAN_POINT('Ctrl Pts',(-9.01061464569913,64.8975376569547,-438.999999999994));
#33919=CARTESIAN_POINT('Ctrl Pts',(-9.01662385181665,64.92000174141,-438.969185598811));
#33920=CARTESIAN_POINT('Ctrl Pts',(-4.01580166730864,47.7814767988564,-462.551777463598));
#33921=CARTESIAN_POINT('Ctrl Pts',(-4.02534345873132,47.8192291909881,-462.499999999992));
#33922=CARTESIAN_POINT('Ctrl Pts',(-8.35603258132023,64.9537343079005,-438.999999999994));
#33923=CARTESIAN_POINT('Ctrl Pts',(-8.36171120225726,64.9762019468255,-438.969185598811));
#33924=CARTESIAN_POINT('Ctrl Pts',(-3.237715926142,47.9638400252938,-462.551777463598));
#33925=CARTESIAN_POINT('Ctrl Pts',(-3.24611879785494,48.0015988823275,-462.499999999992));
#33926=CARTESIAN_POINT('Ctrl Pts',(-7.05989165387597,65.1390381946525,-438.999999999994));
#33927=CARTESIAN_POINT('Ctrl Pts',(-7.06489246778255,65.1615096810445,-438.969185598811));
#33928=CARTESIAN_POINT('Ctrl Pts',(-2.86166483945136,48.0926515275283,-462.551777463598));
#33929=CARTESIAN_POINT('Ctrl Pts',(-2.86948247455976,48.1303963845569,-462.499999999992));
#33930=CARTESIAN_POINT('Ctrl Pts',(-6.41763667627501,65.2614815787748,-438.999999999994));
#33931=CARTESIAN_POINT('Ctrl Pts',(-6.42228919742521,65.2839447333224,-438.969185598811));
#33932=CARTESIAN_POINT('Ctrl Pts',(-2.50783263663928,48.2524848469793,-462.551779559468));
#33933=CARTESIAN_POINT('Ctrl Pts',(-2.51503960160435,48.2902113213028,-462.499999999992));
#33934=CARTESIAN_POINT('Ctrl Pts',(-5.78603174536888,65.4129532414351,-438.999048757082));
#33935=CARTESIAN_POINT('Ctrl Pts',(-5.79032083746175,65.4354054558553,-438.968233108581));
#33936=CARTESIAN_POINT('Ctrl Pts',(-2.50449034865332,48.253994627545,-462.551779579265));
#33937=CARTESIAN_POINT('Ctrl Pts',(-2.51169154524722,48.2917209282261,-462.499999999992));
#33938=CARTESIAN_POINT('Ctrl Pts',(-5.78006562483024,65.4143840380509,-438.999039771671));
#33939=CARTESIAN_POINT('Ctrl Pts',(-5.78435128398358,65.4368361491308,-438.968224111388));
#33940=CARTESIAN_POINT('Ctrl Pts',(-2.5011480606674,48.2555044081108,-462.551779599063));
#33941=CARTESIAN_POINT('Ctrl Pts',(-2.50834348889009,48.2932305351494,-462.499999999992));
#33942=CARTESIAN_POINT('Ctrl Pts',(-5.77409950429161,65.4158148346665,-438.99903078626));
#33943=CARTESIAN_POINT('Ctrl Pts',(-5.77838173050535,65.4382668424065,-438.968215114195));
#33944=CARTESIAN_POINT('Ctrl Pts',(-2.49780577268147,48.2570141886766,-462.551779618861));
#33945=CARTESIAN_POINT('Ctrl Pts',(-2.50499543253297,48.2947401420728,-462.499999999992));
#33946=CARTESIAN_POINT('Ctrl Pts',(-5.76813338375298,65.4172456312822,-438.999021800849));
#33947=CARTESIAN_POINT('Ctrl Pts',(-5.77241217702715,65.4396975356821,-438.968206117001));
#33948=CARTESIAN_POINT('',(-13.4208533932044,64.6757844080299,-439.576819794402));
#33949=CARTESIAN_POINT('',(-10.2970852952296,56.400796767239,-451.047494191925));
#33950=CARTESIAN_POINT('Ctrl Pts',(-10.6587895159293,64.8525916307614,-438.999999999994));
#33951=CARTESIAN_POINT('Ctrl Pts',(-11.1431746641298,64.8260069038297,-439.040765404272));
#33952=CARTESIAN_POINT('Ctrl Pts',(-11.6025803817587,64.7985306170646,-439.11052042917));
#33953=CARTESIAN_POINT('Ctrl Pts',(-12.7544621947915,64.7246760613877,-439.352217793466));
#33954=CARTESIAN_POINT('Ctrl Pts',(-13.1700622987402,64.6941515478973,-439.491932720156));
#33955=CARTESIAN_POINT('Ctrl Pts',(-13.4208533931901,64.6757844080304,-439.576819794444));
#33956=CARTESIAN_POINT('Ctrl Pts',(-5.71602822336486,65.0465041066897,-439.501999936794));
#33957=CARTESIAN_POINT('Ctrl Pts',(-5.88573707745702,65.04249459091,-439.45354399244));
#33958=CARTESIAN_POINT('Ctrl Pts',(-6.38201999480569,65.0307778175158,-439.312278964639));
#33959=CARTESIAN_POINT('Ctrl Pts',(-7.55211977412035,64.993294425775,-439.092788088094));
#33960=CARTESIAN_POINT('Ctrl Pts',(-8.00524379523663,64.9764622470322,-439.034023415792));
#33961=CARTESIAN_POINT('Ctrl Pts',(-8.41281803607201,64.9598843197981,-438.999999999994));
#33962=CARTESIAN_POINT('Ctrl Pts',(-12.001137535198,47.8672571975149,-462.54912382016));
#33963=CARTESIAN_POINT('Ctrl Pts',(-12.0248210021412,47.9012883848401,-462.499999999992));
#33964=CARTESIAN_POINT('Ctrl Pts',(-23.079130834684,63.7854192666133,-439.571349832351));
#33965=CARTESIAN_POINT('Ctrl Pts',(-23.0913829153359,63.8030244953067,-439.545936787544));
#33966=CARTESIAN_POINT('Ctrl Pts',(-11.9978892331025,47.8688480698695,-462.549123805034));
#33967=CARTESIAN_POINT('Ctrl Pts',(-12.0215650496218,47.9028810613388,-462.499999999992));
#33968=CARTESIAN_POINT('Ctrl Pts',(-23.0723040300149,63.787854031318,-439.571356892768));
#33969=CARTESIAN_POINT('Ctrl Pts',(-23.0845521529011,63.8054601933426,-439.545943855786));
#33970=CARTESIAN_POINT('Ctrl Pts',(-11.9946409310072,47.8704389422241,-462.549123789907));
#33971=CARTESIAN_POINT('Ctrl Pts',(-12.0183090971022,47.9044737378375,-462.499999999992));
#33972=CARTESIAN_POINT('Ctrl Pts',(-23.065477225346,63.7902887960227,-439.571363953185));
#33973=CARTESIAN_POINT('Ctrl Pts',(-23.0777213904665,63.8078958913785,-439.545950924028));
#33974=CARTESIAN_POINT('Ctrl Pts',(-11.9913926289119,47.8720298145787,-462.54912377478));
#33975=CARTESIAN_POINT('Ctrl Pts',(-12.0150531445829,47.9060664143362,-462.499999999992));
#33976=CARTESIAN_POINT('Ctrl Pts',(-23.0586504206769,63.7927235607274,-439.571371013602));
#33977=CARTESIAN_POINT('Ctrl Pts',(-23.0708906280318,63.8103315894145,-439.545957992271));
#33978=CARTESIAN_POINT('Ctrl Pts',(-11.6297556451161,48.0491433536022,-462.549122090709));
#33979=CARTESIAN_POINT('Ctrl Pts',(-11.6525644307966,48.083380810676,-462.499999999992));
#33980=CARTESIAN_POINT('Ctrl Pts',(-22.2986148768729,64.0637885473651,-439.572157057449));
#33981=CARTESIAN_POINT('Ctrl Pts',(-22.3104144618915,64.0815004848273,-439.546744907332));
#33982=CARTESIAN_POINT('Ctrl Pts',(-11.242849509649,48.1937673617144,-462.549122090709));
#33983=CARTESIAN_POINT('Ctrl Pts',(-11.2648118979094,48.2281753266956,-462.499999999992));
#33984=CARTESIAN_POINT('Ctrl Pts',(-21.5158045027396,64.2881680009153,-439.572157057449));
#33985=CARTESIAN_POINT('Ctrl Pts',(-21.5271662241007,64.3059681466046,-439.546744907332));
#33986=CARTESIAN_POINT('Ctrl Pts',(-10.4386278915723,48.4023780622091,-462.549122090709));
#33987=CARTESIAN_POINT('Ctrl Pts',(-10.4589027392768,48.4370911577423,-462.499999999992));
#33988=CARTESIAN_POINT('Ctrl Pts',(-19.9222321103714,64.6395041823707,-439.572157057449));
#33989=CARTESIAN_POINT('Ctrl Pts',(-19.9327208225974,64.6574621801238,-439.546744907332));
#33990=CARTESIAN_POINT('Ctrl Pts',(-10.0214566187051,48.4662722784951,-462.549122090709));
#33991=CARTESIAN_POINT('Ctrl Pts',(-10.040890022398,48.5011201886057,-462.499999999992));
#33992=CARTESIAN_POINT('Ctrl Pts',(-19.111473566452,64.7664582111738,-439.572157057449));
#33993=CARTESIAN_POINT('Ctrl Pts',(-19.1215269775492,64.7844859520552,-439.546744907332));
#33994=CARTESIAN_POINT('Ctrl Pts',(-9.18272025134817,48.5064780795265,-462.549122090709));
#33995=CARTESIAN_POINT('Ctrl Pts',(-9.2004590084912,48.5415610543766,-462.499999999992));
#33996=CARTESIAN_POINT('Ctrl Pts',(-17.4800625805772,64.9166160566032,-439.572157057449));
#33997=CARTESIAN_POINT('Ctrl Pts',(-17.4892393064215,64.9347654026598,-439.546744907332));
#33998=CARTESIAN_POINT('Ctrl Pts',(-8.76134336058432,48.4828179859497,-462.549122090709));
#33999=CARTESIAN_POINT('Ctrl Pts',(-8.77822932151279,48.518001075961,-462.499999999992));
#34000=CARTESIAN_POINT('Ctrl Pts',(-16.6597884011211,64.9397850479169,-439.572157057449));
#34001=CARTESIAN_POINT('Ctrl Pts',(-16.6685239530432,64.9579861861807,-439.546744907332));
#34002=CARTESIAN_POINT('Ctrl Pts',(-7.94082488447429,48.3521211537968,-462.549122090709));
#34003=CARTESIAN_POINT('Ctrl Pts',(-7.95597858419148,48.3874670903318,-462.499999999992));
#34004=CARTESIAN_POINT('Ctrl Pts',(-15.0290009666032,64.8852600322724,-439.572157057449));
#34005=CARTESIAN_POINT('Ctrl Pts',(-15.0368403742184,64.903545415328,-439.546744907332));
#34006=CARTESIAN_POINT('Ctrl Pts',(-7.5418363068398,48.2451812560949,-462.549122090709));
#34007=CARTESIAN_POINT('Ctrl Pts',(-7.55611022239511,48.280589721988,-462.499999999992));
#34008=CARTESIAN_POINT('Ctrl Pts',(-14.218491429066,64.8075683781914,-439.572157057449));
#34009=CARTESIAN_POINT('Ctrl Pts',(-14.2258757011838,64.8258861093293,-439.546744907332));
#34010=CARTESIAN_POINT('Ctrl Pts',(-7.16488722681163,48.1034777948425,-462.549123975058));
#34011=CARTESIAN_POINT('Ctrl Pts',(-7.17826498480897,48.138916015164,-462.499999999992));
#34012=CARTESIAN_POINT('Ctrl Pts',(-13.4223626974158,64.6797826157486,-439.571277533733));
#34013=CARTESIAN_POINT('Ctrl Pts',(-13.4292833636476,64.6981157396354,-439.545864408792));
#34014=CARTESIAN_POINT('Ctrl Pts',(-7.16167302984563,48.1022695074123,-462.549123991125));
#34015=CARTESIAN_POINT('Ctrl Pts',(-7.1750431464212,48.1377079814461,-462.499999999992));
#34016=CARTESIAN_POINT('Ctrl Pts',(-13.4155742087594,64.6786930027698,-439.571270034146));
#34017=CARTESIAN_POINT('Ctrl Pts',(-13.4224909218826,64.6970262579086,-439.545856900893));
#34018=CARTESIAN_POINT('Ctrl Pts',(-7.15845883287963,48.101061219982,-462.549124007193));
#34019=CARTESIAN_POINT('Ctrl Pts',(-7.17182130803346,48.1364999477281,-462.499999999992));
#34020=CARTESIAN_POINT('Ctrl Pts',(-13.408785720103,64.677603389791,-439.571262534558));
#34021=CARTESIAN_POINT('Ctrl Pts',(-13.4156984801177,64.6959367761818,-439.545849392994));
#34022=CARTESIAN_POINT('Ctrl Pts',(-7.15524463591363,48.0998529325518,-462.54912402326));
#34023=CARTESIAN_POINT('Ctrl Pts',(-7.16859946964568,48.1352919140101,-462.499999999992));
#34024=CARTESIAN_POINT('Ctrl Pts',(-13.4019972314466,64.6765137768122,-439.571255034971));
#34025=CARTESIAN_POINT('Ctrl Pts',(-13.4089060383527,64.6948472944551,-439.545841885095));
#34026=CARTESIAN_POINT('',(-23.0582867813677,63.7922004510104,-439.572125998435));
#34027=CARTESIAN_POINT('',(-17.67449156409,56.0473953277366,-450.749918885292));
#34028=CARTESIAN_POINT('Ctrl Pts',(-13.4208533931897,64.6757844080304,-439.576819794444));
#34029=CARTESIAN_POINT('Ctrl Pts',(-13.9566749456381,64.6364685998891,-439.76241002145));
#34030=CARTESIAN_POINT('Ctrl Pts',(-15.6979001875856,64.5119662151012,-440.373416758168));
#34031=CARTESIAN_POINT('Ctrl Pts',(-20.5490919569703,64.0684585284553,-440.290614638996));
#34032=CARTESIAN_POINT('Ctrl Pts',(-22.4739368675365,63.8571630490881,-439.738547054618));
#34033=CARTESIAN_POINT('Ctrl Pts',(-23.0582867814246,63.7922004510004,-439.572125998638));
#34034=CARTESIAN_POINT('Origin',(29.9999999999753,83.0468894509273,-439.));
#34035=CARTESIAN_POINT('',(-26.1597137411461,63.4173578413804,-438.999999999994));
#34036=CARTESIAN_POINT('',(-28.3882768422949,63.1102977520074,-438.999999999994));
#34037=CARTESIAN_POINT('Origin',(-0.00176539235111073,-134.670997806539,
-438.999999999971));
#34038=CARTESIAN_POINT('Ctrl Pts',(-26.1597137411455,63.4173578413776,-438.999999999997));
#34039=CARTESIAN_POINT('Ctrl Pts',(-26.5275732374657,63.3451801861953,-438.999999999997));
#34040=CARTESIAN_POINT('Ctrl Pts',(-26.8973783983544,63.2833853100965,-438.999999999934));
#34041=CARTESIAN_POINT('Ctrl Pts',(-27.6412583367134,63.1808107453415,-438.999999999934));
#34042=CARTESIAN_POINT('Ctrl Pts',(-28.0144149229582,63.140261967893,-438.999999999997));
#34043=CARTESIAN_POINT('Ctrl Pts',(-28.3882768422946,63.1102977520047,-438.999999999997));
#34044=CARTESIAN_POINT('Ctrl Pts',(-18.8775059186204,47.6342738478878,-462.508833269478));
#34045=CARTESIAN_POINT('Ctrl Pts',(-18.8849353455675,47.6408044887233,-462.499999999992));
#34046=CARTESIAN_POINT('Ctrl Pts',(-38.6501574445149,65.0148990831144,-438.999999999994));
#34047=CARTESIAN_POINT('Ctrl Pts',(-38.6570457183015,65.0209540376077,-438.991810138368));
#34048=CARTESIAN_POINT('Ctrl Pts',(-18.8753643113511,47.6334276618779,-462.508833269478));
#34049=CARTESIAN_POINT('Ctrl Pts',(-18.8827928271309,47.6399577985274,-462.499999999992));
#34050=CARTESIAN_POINT('Ctrl Pts',(-38.6455908591808,65.0127110581453,-438.999999999994));
#34051=CARTESIAN_POINT('Ctrl Pts',(-38.6524782881685,65.0187655451771,-438.991810138368));
#34052=CARTESIAN_POINT('Ctrl Pts',(-18.873222704082,47.632581475868,-462.508833269478));
#34053=CARTESIAN_POINT('Ctrl Pts',(-18.8806503086941,47.6391111083315,-462.499999999992));
#34054=CARTESIAN_POINT('Ctrl Pts',(-38.6410242738467,65.0105230331761,-438.999999999994));
#34055=CARTESIAN_POINT('Ctrl Pts',(-38.6479108580357,65.0165770527465,-438.991810138368));
#34056=CARTESIAN_POINT('Ctrl Pts',(-18.8710810968126,47.6317352898581,-462.508833269478));
#34057=CARTESIAN_POINT('Ctrl Pts',(-18.8785077902573,47.6382644181355,-462.499999999992));
#34058=CARTESIAN_POINT('Ctrl Pts',(-38.6364576885126,65.008335008207,-438.999999999994));
#34059=CARTESIAN_POINT('Ctrl Pts',(-38.6433434279027,65.0143885603157,-438.991810138368));
#34060=CARTESIAN_POINT('Ctrl Pts',(-18.6207111444172,47.5328097986826,-462.508833269478));
#34061=CARTESIAN_POINT('Ctrl Pts',(-18.6280313155475,47.5392799838325,-462.499999999992));
#34062=CARTESIAN_POINT('Ctrl Pts',(-38.1025896123615,64.7525384785492,-438.999999999994));
#34063=CARTESIAN_POINT('Ctrl Pts',(-38.1093765884324,64.7585373808978,-438.991810138368));
#34064=CARTESIAN_POINT('Ctrl Pts',(-18.3668172652831,47.4458875093331,-462.508833269478));
#34065=CARTESIAN_POINT('Ctrl Pts',(-18.3740287411124,47.4523034520998,-462.499999999992));
#34066=CARTESIAN_POINT('Ctrl Pts',(-37.5594144298113,64.5212556955974,-438.999999999994));
#34067=CARTESIAN_POINT('Ctrl Pts',(-37.5661006278547,64.527204306532,-438.991810138368));
#34068=CARTESIAN_POINT('Ctrl Pts',(-17.3709360911557,47.1570554700231,-462.508833269478));
#34069=CARTESIAN_POINT('Ctrl Pts',(-17.377718225807,47.1632792121921,-462.499999999992));
#34070=CARTESIAN_POINT('Ctrl Pts',(-35.420886109377,63.7209016414593,-438.999999999994));
#34071=CARTESIAN_POINT('Ctrl Pts',(-35.4271742390897,63.7266720515249,-438.991810138368));
#34072=CARTESIAN_POINT('Ctrl Pts',(-16.616292128253,47.0488954908114,-462.508833269478));
#34073=CARTESIAN_POINT('Ctrl Pts',(-16.6227423732312,47.0550172977463,-462.499999999992));
#34074=CARTESIAN_POINT('Ctrl Pts',(-33.7829521032343,63.3414515779963,-438.999999999994));
#34075=CARTESIAN_POINT('Ctrl Pts',(-33.7889325178365,63.3471274777037,-438.991810138368));
#34076=CARTESIAN_POINT('Ctrl Pts',(-15.1578028767041,47.0244381605313,-462.508833269478));
#34077=CARTESIAN_POINT('Ctrl Pts',(-15.1635931228177,47.0304369741045,-462.499999999992));
#34078=CARTESIAN_POINT('Ctrl Pts',(-30.5679441254776,62.9896601345508,-438.999999999994));
#34079=CARTESIAN_POINT('Ctrl Pts',(-30.5733126149729,62.9952219996288,-438.991810138368));
#34080=CARTESIAN_POINT('Ctrl Pts',(-14.4544087306705,47.1073598914834,-462.50883327605));
#34081=CARTESIAN_POINT('Ctrl Pts',(-14.4598710640638,47.1133367987068,-462.499999999992));
#34082=CARTESIAN_POINT('Ctrl Pts',(-28.9918441848079,63.0142803808168,-438.999982515861));
#34083=CARTESIAN_POINT('Ctrl Pts',(-28.9969086464675,63.0198219351849,-438.991792648143));
#34084=CARTESIAN_POINT('Ctrl Pts',(-13.1507400659786,47.4134699086769,-462.508833253297));
#34085=CARTESIAN_POINT('Ctrl Pts',(-13.1555740488444,47.4194722561782,-462.499999999992));
#34086=CARTESIAN_POINT('Ctrl Pts',(-26.0158855700949,63.3880970670556,-439.000043049088));
#34087=CARTESIAN_POINT('Ctrl Pts',(-26.0203674497467,63.3936622086534,-438.991853202466));
#34088=CARTESIAN_POINT('Ctrl Pts',(-12.5503158851177,47.6359705084204,-462.508833269478));
#34089=CARTESIAN_POINT('Ctrl Pts',(-12.5548498814442,47.6420203105473,-462.499999999992));
#34090=CARTESIAN_POINT('Ctrl Pts',(-24.6170782372607,63.7368932453249,-438.999999999994));
#34091=CARTESIAN_POINT('Ctrl Pts',(-24.6212819811383,63.7425023849935,-438.991810138368));
#34092=CARTESIAN_POINT('Ctrl Pts',(-12.0107984455655,47.899945859334,-462.508833572313));
#34093=CARTESIAN_POINT('Ctrl Pts',(-12.0150531445829,47.9060664143362,-462.499999999992));
#34094=CARTESIAN_POINT('Ctrl Pts',(-23.3342398922659,64.1891700571751,-438.999194340672));
#34095=CARTESIAN_POINT('Ctrl Pts',(-23.3381846826136,64.1948447961396,-438.99100419827));
#34096=CARTESIAN_POINT('Ctrl Pts',(-12.0091656235255,47.9007447672828,-462.508833573229));
#34097=CARTESIAN_POINT('Ctrl Pts',(-12.0134194772637,47.906865536415,-462.499999999992));
#34098=CARTESIAN_POINT('Ctrl Pts',(-23.3303574473811,64.1905388499007,-438.999191902385));
#34099=CARTESIAN_POINT('Ctrl Pts',(-23.3343014540193,64.1962137873981,-438.991001759134));
#34100=CARTESIAN_POINT('Ctrl Pts',(-12.0075328014854,47.9015436752317,-462.508833574146));
#34101=CARTESIAN_POINT('Ctrl Pts',(-12.0117858099447,47.9076646584938,-462.499999999992));
#34102=CARTESIAN_POINT('Ctrl Pts',(-23.3264750024962,64.1919076426262,-438.999189464098));
#34103=CARTESIAN_POINT('Ctrl Pts',(-23.3304182254248,64.1975827786566,-438.990999319997));
#34104=CARTESIAN_POINT('Ctrl Pts',(-12.0058999794455,47.9023425831805,-462.508833575062));
#34105=CARTESIAN_POINT('Ctrl Pts',(-12.0101521426257,47.9084637805726,-462.499999999992));
#34106=CARTESIAN_POINT('Ctrl Pts',(-23.3225925576115,64.1932764353518,-438.999187025811));
#34107=CARTESIAN_POINT('Ctrl Pts',(-23.3265349968304,64.198951769915,-438.99099688086));
#34108=CARTESIAN_POINT('',(-33.4829940324908,62.2764393526616,-440.999972026227));
#34109=CARTESIAN_POINT('Ctrl Pts',(-33.4829940630133,62.2764393583309,-440.9999720502));
#34110=CARTESIAN_POINT('Ctrl Pts',(-31.1113726356467,59.8388581046014,-444.596060591447));
#34111=CARTESIAN_POINT('Ctrl Pts',(-28.6868186804599,57.3709516983183,-448.232584923789));
#34112=CARTESIAN_POINT('Ctrl Pts',(-23.4113303313584,52.0741661663874,-456.017611271358));
#34113=CARTESIAN_POINT('Ctrl Pts',(-21.3792166372997,50.0678629208131,-458.957669002678));
#34114=CARTESIAN_POINT('Ctrl Pts',(-18.878507790257,47.6382644181356,-462.499999999992));
#34115=CARTESIAN_POINT('Ctrl Pts',(-28.3882768422949,63.1102977520076,-438.999999999993));
#34116=CARTESIAN_POINT('Ctrl Pts',(-29.3116124609106,62.9763196718963,-439.082600088505));
#34117=CARTESIAN_POINT('Ctrl Pts',(-30.2271255160582,62.8347324864127,-439.274916650434));
#34118=CARTESIAN_POINT('Ctrl Pts',(-32.180534929123,62.5140220534877,-440.010156560329));
#34119=CARTESIAN_POINT('Ctrl Pts',(-32.9450987460992,62.3760920008183,-440.536273886144));
#34120=CARTESIAN_POINT('Ctrl Pts',(-33.482994016876,62.2764393498852,-440.999972043744));
#34121=CARTESIAN_POINT('Ctrl Pts',(-23.0582867814239,63.7922004510005,-439.572125998639));
#34122=CARTESIAN_POINT('Ctrl Pts',(-23.2597393793474,63.7697900102401,-439.515595788428));
#34123=CARTESIAN_POINT('Ctrl Pts',(-23.8404446999355,63.7050803487465,-439.353219756612));
#34124=CARTESIAN_POINT('Ctrl Pts',(-25.1137024112667,63.5513262928731,-439.115720930552));
#34125=CARTESIAN_POINT('Ctrl Pts',(-25.6361613101107,63.4857267740936,-439.04357303287));
#34126=CARTESIAN_POINT('Ctrl Pts',(-26.1597137411461,63.4173578413807,-438.999999999993));
#34127=CARTESIAN_POINT('Ctrl Pts',(-42.0325401995064,60.6377891214161,-440.991114438282));
#34128=CARTESIAN_POINT('Ctrl Pts',(-42.0285040216223,60.6317485621414,-440.999646067766));
#34129=CARTESIAN_POINT('Ctrl Pts',(-31.8570244760066,45.4090817011473,-462.499999999992));
#34130=CARTESIAN_POINT('Ctrl Pts',(-31.8468530089389,45.3938590466631,-462.521500335317));
#34131=CARTESIAN_POINT('Ctrl Pts',(-42.0051853072238,60.6436503983426,-440.99111632347));
#34132=CARTESIAN_POINT('Ctrl Pts',(-42.0011517636324,60.6376092981949,-440.999647949747));
#34133=CARTESIAN_POINT('Ctrl Pts',(-31.8363095381066,45.413574653915,-462.499999999992));
#34134=CARTESIAN_POINT('Ctrl Pts',(-31.8261447041996,45.3983506275219,-462.521500339637));
#34135=CARTESIAN_POINT('Ctrl Pts',(-41.9778304149411,60.6495116752692,-440.991118208659));
#34136=CARTESIAN_POINT('Ctrl Pts',(-41.9737995056426,60.6434700342484,-440.999649831728));
#34137=CARTESIAN_POINT('Ctrl Pts',(-31.8155946002065,45.4180676066827,-462.499999999992));
#34138=CARTESIAN_POINT('Ctrl Pts',(-31.8054363994604,45.4028422083807,-462.521500343958));
#34139=CARTESIAN_POINT('Ctrl Pts',(-41.9504755226585,60.6553729521959,-440.991120093849));
#34140=CARTESIAN_POINT('Ctrl Pts',(-41.9464472476527,60.6493307703021,-440.999651713709));
#34141=CARTESIAN_POINT('Ctrl Pts',(-31.7948796623065,45.4225605594505,-462.499999999992));
#34142=CARTESIAN_POINT('Ctrl Pts',(-31.7847280947211,45.4073337892395,-462.521500348278));
#34143=CARTESIAN_POINT('Ctrl Pts',(-36.316732701322,61.8625035257008,-440.991508348712));
#34144=CARTESIAN_POINT('Ctrl Pts',(-36.3132469591819,61.8563499509359,-441.000039307893));
#34145=CARTESIAN_POINT('Ctrl Pts',(-27.5283826319057,46.3479396136299,-462.499999999992));
#34146=CARTESIAN_POINT('Ctrl Pts',(-27.519597245617,46.332430281845,-462.521501238125));
#34147=CARTESIAN_POINT('Ctrl Pts',(-30.6323582333801,62.8326921119377,-440.991469430236));
#34148=CARTESIAN_POINT('Ctrl Pts',(-30.6294184953645,62.8264473376596,-440.999999999994));
#34149=CARTESIAN_POINT('Ctrl Pts',(-23.220257192727,47.0874462155727,-462.499999999992));
#34150=CARTESIAN_POINT('Ctrl Pts',(-23.2128472394025,47.0717055319886,-462.521502298291));
#34151=CARTESIAN_POINT('Ctrl Pts',(-24.9038049544188,63.5523580409965,-440.99146973189));
#34152=CARTESIAN_POINT('Ctrl Pts',(-24.9014153257654,63.5460465225645,-440.999999999994));
#34153=CARTESIAN_POINT('Ctrl Pts',(-18.8785077896217,47.6382644182162,-462.499999999992));
#34154=CARTESIAN_POINT('Ctrl Pts',(-18.8724840252419,47.622354373005,-462.52150305867));
#34155=CARTESIAN_POINT('Ctrl Pts',(-24.8758540410355,63.5558694546237,-440.991469733362));
#34156=CARTESIAN_POINT('Ctrl Pts',(-24.8734670964907,63.5495576105319,-440.999999999994));
#34157=CARTESIAN_POINT('Ctrl Pts',(-18.8573226583922,47.6409520804515,-462.499999999992));
#34158=CARTESIAN_POINT('Ctrl Pts',(-18.8513056577824,47.6250412088575,-462.521503062381));
#34159=CARTESIAN_POINT('Ctrl Pts',(-24.8479031276521,63.5593808682511,-440.991469734834));
#34160=CARTESIAN_POINT('Ctrl Pts',(-24.8455188672159,63.5530686984991,-440.999999999994));
#34161=CARTESIAN_POINT('Ctrl Pts',(-18.8361375271626,47.6436397426871,-462.499999999992));
#34162=CARTESIAN_POINT('Ctrl Pts',(-18.8301272903229,47.6277280447099,-462.521503066091));
#34163=CARTESIAN_POINT('Ctrl Pts',(-24.8199522142688,63.5628922818783,-440.991469736305));
#34164=CARTESIAN_POINT('Ctrl Pts',(-24.8175706379412,63.5565797864666,-440.999999999994));
#34165=CARTESIAN_POINT('Ctrl Pts',(-18.814952395933,47.6463274049225,-462.499999999992));
#34166=CARTESIAN_POINT('Ctrl Pts',(-18.8089489228634,47.6304148805623,-462.521503069801));
#34167=CARTESIAN_POINT('',(-41.9462958339113,60.6491036583583,-440.999972397992));
#34168=CARTESIAN_POINT('Ctrl Pts',(-31.7948796623065,45.4225605594505,-462.499999999992));
#34169=CARTESIAN_POINT('Ctrl Pts',(-32.3589367582276,46.2685042102034,-461.305499732182));
#34170=CARTESIAN_POINT('Ctrl Pts',(-32.9230130678469,47.114453047541,-460.110987971848));
#34171=CARTESIAN_POINT('Ctrl Pts',(-33.4870955758511,47.9604022194252,-458.916474195592));
#34172=CARTESIAN_POINT('Ctrl Pts',(-33.5108390027484,47.9960100109033,-458.866194582021));
#34173=CARTESIAN_POINT('Ctrl Pts',(-33.5345824407334,48.0316178027276,-458.815914965151));
#34174=CARTESIAN_POINT('Ctrl Pts',(-33.5583258888888,48.0672255944517,-458.765635345777));
#34175=CARTESIAN_POINT('Ctrl Pts',(-33.8316335282801,48.4771020974939,-458.186873407305));
#34176=CARTESIAN_POINT('Ctrl Pts',(-34.1049416910635,48.8869789136655,-457.608110953941));
#34177=CARTESIAN_POINT('Ctrl Pts',(-34.3782537048231,49.2968534751887,-457.029350268047));
#34178=CARTESIAN_POINT('Ctrl Pts',(-34.5132877509722,49.4993583694842,-456.743404560452));
#34179=CARTESIAN_POINT('Ctrl Pts',(-34.648322925422,49.7018626398917,-456.457459324899));
#34180=CARTESIAN_POINT('Ctrl Pts',(-34.7833597254613,49.9043659276223,-456.171514872232));
#34181=CARTESIAN_POINT('Ctrl Pts',(-34.9151745034667,50.1020374209471,-455.892393147345));
#34182=CARTESIAN_POINT('Ctrl Pts',(-35.0469908795589,50.2997079600871,-455.613272177396));
#34183=CARTESIAN_POINT('Ctrl Pts',(-35.1788083996884,50.4973775420908,-455.334152087624));
#34184=CARTESIAN_POINT('Ctrl Pts',(-35.348615406454,50.752015013769,-454.974590271215));
#34185=CARTESIAN_POINT('Ctrl Pts',(-35.5184242304502,51.0066509291891,-454.615029897676));
#34186=CARTESIAN_POINT('Ctrl Pts',(-35.6882312710722,51.2612862178012,-454.255470778926));
#34187=CARTESIAN_POINT('Ctrl Pts',(-36.0826190404626,51.8526930470817,-453.420371608195));
#34188=CARTESIAN_POINT('Ctrl Pts',(-36.4769941306178,52.4440976990883,-452.585278532376));
#34189=CARTESIAN_POINT('Ctrl Pts',(-36.87136162915,53.0354928881843,-451.750199183157));
#34190=CARTESIAN_POINT('Ctrl Pts',(-36.8713782411473,53.0355177996066,-451.750164006993));
#34191=CARTESIAN_POINT('Ctrl Pts',(-36.8713948531446,53.035542711029,-451.750128830828));
#34192=CARTESIAN_POINT('Ctrl Pts',(-36.8714114651419,53.0355676224513,-451.750093654664));
#34193=CARTESIAN_POINT('Ctrl Pts',(-37.1088992326438,53.3917052969764,-451.247209588678));
#34194=CARTESIAN_POINT('Ctrl Pts',(-37.3463820495311,53.7478476179124,-450.744321111962));
#34195=CARTESIAN_POINT('Ctrl Pts',(-37.5838553593534,54.1039950517835,-450.241428853719));
#34196=CARTESIAN_POINT('Ctrl Pts',(-37.9100804261045,54.5932467511626,-449.550588857272));
#34197=CARTESIAN_POINT('Ctrl Pts',(-38.2363414682279,55.0824885214636,-448.859751561661));
#34198=CARTESIAN_POINT('Ctrl Pts',(-38.5627017963576,55.5716951867403,-448.168931295036));
#34199=CARTESIAN_POINT('Ctrl Pts',(-38.5630166981229,55.5721672172823,-448.168264729578));
#34200=CARTESIAN_POINT('Ctrl Pts',(-38.5633315999745,55.5726392477937,-448.167598164135));
#34201=CARTESIAN_POINT('Ctrl Pts',(-38.5636465019127,55.5731112782747,-448.166931598707));
#34202=CARTESIAN_POINT('Ctrl Pts',(-38.5760051462592,55.5916365908502,-448.140771565806));
#34203=CARTESIAN_POINT('Ctrl Pts',(-38.5883639239044,55.6101618563835,-448.11461155567));
#34204=CARTESIAN_POINT('Ctrl Pts',(-38.6007228216993,55.6286870798238,-448.088451565684));
#34205=CARTESIAN_POINT('Ctrl Pts',(-38.6160934753,55.6517267389508,-448.055916613866));
#34206=CARTESIAN_POINT('Ctrl Pts',(-38.6314643147417,55.6747663329655,-448.023381693218));
#34207=CARTESIAN_POINT('Ctrl Pts',(-38.6468353147218,55.6978058713775,-447.990846798726));
#34208=CARTESIAN_POINT('Ctrl Pts',(-38.8979459656751,56.0741947527639,-447.459335605872));
#34209=CARTESIAN_POINT('Ctrl Pts',(-39.1490995352716,56.4505687718856,-446.927831437525));
#34210=CARTESIAN_POINT('Ctrl Pts',(-39.4001855850623,56.8269694640148,-446.396312247445));
#34211=CARTESIAN_POINT('Ctrl Pts',(-39.4034915843839,56.8319254559302,-446.389313841586));
#34212=CARTESIAN_POINT('Ctrl Pts',(-39.4072720742608,56.8375927809872,-446.381310960185));
#34213=CARTESIAN_POINT('Ctrl Pts',(-39.4101046309297,56.841837216879,-446.375317027575));
#34214=CARTESIAN_POINT('Ctrl Pts',(-39.5913882577387,57.1134811139516,-445.99170534054));
#34215=CARTESIAN_POINT('Ctrl Pts',(-39.7877372632166,57.4079275655785,-445.575932518066));
#34216=CARTESIAN_POINT('Ctrl Pts',(-39.9991450289739,57.7251779818922,-445.127998595665));
#34217=CARTESIAN_POINT('Ctrl Pts',(-40.0793695533942,57.8455674277563,-444.958017678609));
#34218=CARTESIAN_POINT('Ctrl Pts',(-40.1617685171492,57.9692393496446,-444.78340557784));
#34219=CARTESIAN_POINT('Ctrl Pts',(-40.2463321871013,58.0961960812351,-444.604161989806));
#34220=CARTESIAN_POINT('Ctrl Pts',(-40.2490197084776,58.1002308981986,-444.598465442166));
#34221=CARTESIAN_POINT('Ctrl Pts',(-40.2517094161308,58.1042690329628,-444.592764216566));
#34222=CARTESIAN_POINT('Ctrl Pts',(-40.2544013097201,58.108310485609,-444.587058312992));
#34223=CARTESIAN_POINT('Ctrl Pts',(-40.2547914092775,58.1088961584213,-444.586231433925));
#34224=CARTESIAN_POINT('Ctrl Pts',(-40.2551815547414,58.1094819009116,-444.585404456617));
#34225=CARTESIAN_POINT('Ctrl Pts',(-40.2555717461105,58.1100677130802,-444.584577381068));
#34226=CARTESIAN_POINT('Ctrl Pts',(-40.2557149406528,58.1102826976032,-444.584273856402));
#34227=CARTESIAN_POINT('Ctrl Pts',(-40.2558581413776,58.1104976915104,-444.583970318506));
#34228=CARTESIAN_POINT('Ctrl Pts',(-40.2560013482848,58.1107126948018,-444.583666767379));
#34229=CARTESIAN_POINT('Ctrl Pts',(-40.2796849784717,58.1462700470485,-444.533465329607));
#34230=CARTESIAN_POINT('Ctrl Pts',(-40.303537699453,58.1820840635307,-444.482902015482));
#34231=CARTESIAN_POINT('Ctrl Pts',(-40.3275595667118,58.2181546889882,-444.431976878569));
#34232=CARTESIAN_POINT('Ctrl Pts',(-40.4124840726278,58.3456751690598,-444.251941245018));
#34233=CARTESIAN_POINT('Ctrl Pts',(-40.499520101303,58.4764037568062,-444.067382958364));
#34234=CARTESIAN_POINT('Ctrl Pts',(-40.5886753472471,58.6103388069207,-443.878302012751));
#34235=CARTESIAN_POINT('Ctrl Pts',(-40.6165363616047,58.6521935100814,-443.819214217247));
#34236=CARTESIAN_POINT('Ctrl Pts',(-40.6446043519804,58.6943613397393,-443.759684755887));
#34237=CARTESIAN_POINT('Ctrl Pts',(-40.6728796563084,58.7368422234442,-443.699713628641));
#34238=CARTESIAN_POINT('Ctrl Pts',(-40.6747646765969,58.7396742823579,-443.695715553492));
#34239=CARTESIAN_POINT('Ctrl Pts',(-40.6760795623318,58.7416497712972,-443.692926715857));
#34240=CARTESIAN_POINT('Ctrl Pts',(-40.678537478369,58.7453425748796,-443.687713514316));
#34241=CARTESIAN_POINT('Ctrl Pts',(-40.8368925478841,58.9832571981406,-443.351844884157));
#34242=CARTESIAN_POINT('Ctrl Pts',(-40.9821297055412,59.2015062105175,-443.043746120084));
#34243=CARTESIAN_POINT('Ctrl Pts',(-41.114288823774,59.400066662282,-442.763435022771));
#34244=CARTESIAN_POINT('Ctrl Pts',(-41.2700380822643,59.6340697605274,-442.433088951029));
#34245=CARTESIAN_POINT('Ctrl Pts',(-41.4076231632199,59.8407285235985,-442.141335825954));
#34246=CARTESIAN_POINT('Ctrl Pts',(-41.5270507342642,60.0200390015437,-441.888178771391));
#34247=CARTESIAN_POINT('Ctrl Pts',(-41.6954461091794,60.2728705286002,-441.531222025617));
#34248=CARTESIAN_POINT('Ctrl Pts',(-41.8277387540249,60.4713302688281,-441.250999947206));
#34249=CARTESIAN_POINT('Ctrl Pts',(-41.9238600911249,60.6154630592316,-441.047475323372));
#34250=CARTESIAN_POINT('Ctrl Pts',(-41.929943127075,60.6245844985714,-441.034595273626));
#34251=CARTESIAN_POINT('Ctrl Pts',(-41.9358812893885,60.6334883672191,-441.022022388381));
#34252=CARTESIAN_POINT('Ctrl Pts',(-41.9416745594323,60.6421746787551,-441.009756655798));
#34253=CARTESIAN_POINT('Ctrl Pts',(-41.94322536715,60.6444999283752,-441.006473226472));
#34254=CARTESIAN_POINT('Ctrl Pts',(-41.9447657920937,60.6468095881562,-441.003211807279));
#34255=CARTESIAN_POINT('Ctrl Pts',(-41.9462958339113,60.6491036583582,-440.999972397991));
#34256=CARTESIAN_POINT('Ctrl Pts',(-33.4829940317438,62.2764393483424,-440.999971988125));
#34257=CARTESIAN_POINT('Ctrl Pts',(-35.2473688614902,61.9765046694296,-440.999378147116));
#34258=CARTESIAN_POINT('Ctrl Pts',(-37.0072017317725,61.652949072738,-440.998941663519));
#34259=CARTESIAN_POINT('Ctrl Pts',(-38.7624945086218,61.3057812102067,-440.999059709867));
#34260=CARTESIAN_POINT('Ctrl Pts',(-39.8254271432111,61.0955507257929,-440.999131193848));
#34261=CARTESIAN_POINT('Ctrl Pts',(-40.8866947611648,60.876660597413,-440.999406024634));
#34262=CARTESIAN_POINT('Ctrl Pts',(-41.9462958339112,60.6491036583585,-440.999972397992));
#34263=CARTESIAN_POINT('Ctrl Pts',(-38.7647784196973,41.8087166343715,-462.499999999991));
#34264=CARTESIAN_POINT('Ctrl Pts',(-39.7995127746359,42.4001734346326,-461.308933337928));
#34265=CARTESIAN_POINT('Ctrl Pts',(-40.8357048397936,42.9924662438129,-460.119580355696));
#34266=CARTESIAN_POINT('Ctrl Pts',(-41.8710255300635,43.5843887879793,-458.928944911376));
#34267=CARTESIAN_POINT('Ctrl Pts',(-41.9145943466774,43.6092983305189,-458.878840071576));
#34268=CARTESIAN_POINT('Ctrl Pts',(-41.9581616507534,43.6342072350156,-458.828732976872));
#34269=CARTESIAN_POINT('Ctrl Pts',(-42.0017269585341,43.6591152324882,-458.778623239637));
#34270=CARTESIAN_POINT('Ctrl Pts',(-42.5030969739151,43.9457681614373,-458.201936857561));
#34271=CARTESIAN_POINT('Ctrl Pts',(-43.0041933315388,44.2322956141741,-457.624895577444));
#34272=CARTESIAN_POINT('Ctrl Pts',(-43.5042383164771,44.5182643009072,-457.046887196222));
#34273=CARTESIAN_POINT('Ctrl Pts',(-43.7512069378789,44.659502178406,-456.761413014161));
#34274=CARTESIAN_POINT('Ctrl Pts',(-43.9936639707697,44.8077097666099,-456.475636259694));
#34275=CARTESIAN_POINT('Ctrl Pts',(-44.2358141697137,44.9557921216003,-456.189595586012));
#34276=CARTESIAN_POINT('Ctrl Pts',(-44.4721203184572,45.1003006586869,-455.910458214757));
#34277=CARTESIAN_POINT('Ctrl Pts',(-44.7070275434294,45.2465058687078,-455.631041156453));
#34278=CARTESIAN_POINT('Ctrl Pts',(-44.9403037377182,45.3946741562122,-455.351299568589));
#34279=CARTESIAN_POINT('Ctrl Pts',(-45.240700079509,45.5854746434694,-454.991068427573));
#34280=CARTESIAN_POINT('Ctrl Pts',(-45.5381389695975,45.7798299821193,-454.630250129497));
#34281=CARTESIAN_POINT('Ctrl Pts',(-45.8336313302898,45.9765136570778,-454.269041480137));
#34282=CARTESIAN_POINT('Ctrl Pts',(-46.5193665414722,46.4329482026873,-453.430801571433));
#34283=CARTESIAN_POINT('Ctrl Pts',(-47.1964439938651,46.8997279795032,-452.59080707252));
#34284=CARTESIAN_POINT('Ctrl Pts',(-47.879046287083,47.3598643087836,-451.751944466043));
#34285=CARTESIAN_POINT('Ctrl Pts',(-48.2897059737973,47.6366864681957,-451.247277167684));
#34286=CARTESIAN_POINT('Ctrl Pts',(-48.7024673284649,47.910980788196,-450.743045916156));
#34287=CARTESIAN_POINT('Ctrl Pts',(-49.1164444213912,48.1838184566469,-450.239075976318));
#34288=CARTESIAN_POINT('Ctrl Pts',(-49.6846286879767,48.5582886222539,-449.547376373752));
#34289=CARTESIAN_POINT('Ctrl Pts',(-50.254528115132,48.9307093367966,-448.856042300473));
#34290=CARTESIAN_POINT('Ctrl Pts',(-50.8246359664257,49.3028643087629,-448.164779253762));
#34291=CARTESIAN_POINT('Ctrl Pts',(-50.825185828888,49.3032232479509,-448.164112538508));
#34292=CARTESIAN_POINT('Ctrl Pts',(-50.8257356894882,49.3035821893701,-448.163445822851));
#34293=CARTESIAN_POINT('Ctrl Pts',(-50.8262855481909,49.3039411330631,-448.162779106782));
#34294=CARTESIAN_POINT('Ctrl Pts',(-50.8478649914022,49.3180280339392,-448.13661354557));
#34295=CARTESIAN_POINT('Ctrl Pts',(-50.8694413893419,49.332118585145,-448.110447322959));
#34296=CARTESIAN_POINT('Ctrl Pts',(-50.8910131109905,49.3462147596686,-448.084280059973));
#34297=CARTESIAN_POINT('Ctrl Pts',(-50.9178408197646,49.3637454913882,-448.051737098301));
#34298=CARTESIAN_POINT('Ctrl Pts',(-50.9446603430864,49.3812860730376,-448.019192307034));
#34299=CARTESIAN_POINT('Ctrl Pts',(-50.971478129671,49.3988287152465,-447.986647158958));
#34300=CARTESIAN_POINT('Ctrl Pts',(-51.9014817827599,50.0071832223397,-446.858026550983));
#34301=CARTESIAN_POINT('Ctrl Pts',(-52.830781565206,50.6163348829018,-445.72929845917));
#34302=CARTESIAN_POINT('Ctrl Pts',(-53.7602372678272,51.2252767470049,-444.600618965139));
#34303=CARTESIAN_POINT('Ctrl Pts',(-53.7649288881994,51.2283505073219,-444.594921721373));
#34304=CARTESIAN_POINT('Ctrl Pts',(-53.7696205154581,51.2314242588856,-444.589224479561));
#34305=CARTESIAN_POINT('Ctrl Pts',(-53.7743121497644,51.2344980015086,-444.583527239736));
#34306=CARTESIAN_POINT('Ctrl Pts',(-53.7749926814309,51.2349438545,-444.582700842822));
#34307=CARTESIAN_POINT('Ctrl Pts',(-53.7756732132458,51.2353897073031,-444.581874445952));
#34308=CARTESIAN_POINT('Ctrl Pts',(-53.7766035309538,51.2359992078201,-444.580744724428));
#34309=CARTESIAN_POINT('Ctrl Pts',(-53.7768533167191,51.2361628556965,-444.580441399742));
#34310=CARTESIAN_POINT('Ctrl Pts',(-54.7572059250983,51.8784435905557,-443.38996075712));
#34311=CARTESIAN_POINT('Ctrl Pts',(-55.7376166746149,52.5201719518042,-442.199871278583));
#34312=CARTESIAN_POINT('Ctrl Pts',(-56.7204946137808,53.1638621099781,-441.006502807678));
#34313=CARTESIAN_POINT('Ctrl Pts',(-56.7231781091608,53.1656195429638,-441.003244619903));
#34314=CARTESIAN_POINT('Ctrl Pts',(-56.7850035851904,53.206109380605,-440.928178664855));
#34315=CARTESIAN_POINT('Ctrl Pts',(-56.8441455674789,53.2448417837246,-440.856370897749));
#34316=CARTESIAN_POINT('Ctrl Pts',(-56.9032875497673,53.2835741868442,-440.784563130644));
#34317=CARTESIAN_POINT('Ctrl Pts',(-38.7453917572008,41.8263434012394,-462.499999999991));
#34318=CARTESIAN_POINT('Ctrl Pts',(-39.7788308189521,42.4190348163309,-461.308907091454));
#34319=CARTESIAN_POINT('Ctrl Pts',(-40.8137298218099,43.0125653951676,-460.119519192124));
#34320=CARTESIAN_POINT('Ctrl Pts',(-41.8477747406438,43.6056914173716,-458.928850923932));
#34321=CARTESIAN_POINT('Ctrl Pts',(-41.8912898696879,43.6306516051987,-458.878744702824));
#34322=CARTESIAN_POINT('Ctrl Pts',(-41.9348035168151,43.6556110942547,-458.828636230518));
#34323=CARTESIAN_POINT('Ctrl Pts',(-41.9783151993904,43.6805696127678,-458.778525120191));
#34324=CARTESIAN_POINT('Ctrl Pts',(-42.4790680707299,43.96780396157,-458.201822935923));
#34325=CARTESIAN_POINT('Ctrl Pts',(-42.9795514885468,44.2549044214201,-457.624766450826));
#34326=CARTESIAN_POINT('Ctrl Pts',(-43.4789894486357,44.5414334488357,-457.046744684544));
#34327=CARTESIAN_POINT('Ctrl Pts',(-43.7256582648306,44.6829480745672,-456.761263891698));
#34328=CARTESIAN_POINT('Ctrl Pts',(-43.9678169353505,44.8314293212802,-456.47548097038));
#34329=CARTESIAN_POINT('Ctrl Pts',(-44.2096704208597,44.9797817325908,-456.189434721086));
#34330=CARTESIAN_POINT('Ctrl Pts',(-44.4456870170472,45.1245538084617,-455.910291908782));
#34331=CARTESIAN_POINT('Ctrl Pts',(-44.680306259769,45.2710191268505,-455.630869972474));
#34332=CARTESIAN_POINT('Ctrl Pts',(-44.913296233648,45.4194436160569,-455.351124206549));
#34333=CARTESIAN_POINT('Ctrl Pts',(-45.2133240013361,45.6105740214795,-454.990887685325));
#34334=CARTESIAN_POINT('Ctrl Pts',(-45.5103972388836,45.8052528000895,-454.630065167715));
#34335=CARTESIAN_POINT('Ctrl Pts',(-45.8055272775946,46.0022524198349,-454.268853751822));
#34336=CARTESIAN_POINT('Ctrl Pts',(-46.4904216652111,46.4594201636385,-453.430607422953));
#34337=CARTESIAN_POINT('Ctrl Pts',(-47.1666762305336,46.9268927739179,-452.5906143289));
#34338=CARTESIAN_POINT('Ctrl Pts',(-47.8484786847142,47.3876688621575,-451.751764605686));
#34339=CARTESIAN_POINT('Ctrl Pts',(-48.2586571810607,47.6648759063206,-451.247105058015));
#34340=CARTESIAN_POINT('Ctrl Pts',(-48.6709293769293,47.9395596801869,-450.742882074723));
#34341=CARTESIAN_POINT('Ctrl Pts',(-49.0844109446666,48.2127905597223,-450.238920749702));
#34342=CARTESIAN_POINT('Ctrl Pts',(-49.6519151020844,48.587800408214,-449.547232970989));
#34343=CARTESIAN_POINT('Ctrl Pts',(-50.2211224273152,48.9607678833433,-448.855911374438));
#34344=CARTESIAN_POINT('Ctrl Pts',(-50.7905303259489,49.3334745944688,-448.164661015305));
#34345=CARTESIAN_POINT('Ctrl Pts',(-50.7910795133149,49.3338340658028,-448.163994312287));
#34346=CARTESIAN_POINT('Ctrl Pts',(-50.7916286988116,49.3341935393728,-448.163327608868));
#34347=CARTESIAN_POINT('Ctrl Pts',(-50.7921778824033,49.3345530152211,-448.162660905037));
#34348=CARTESIAN_POINT('Ctrl Pts',(-50.8137308305952,49.348660800764,-448.136495824087));
#34349=CARTESIAN_POINT('Ctrl Pts',(-50.8352807222728,49.3627722437666,-448.11033008204));
#34350=CARTESIAN_POINT('Ctrl Pts',(-50.8568259266415,49.3768893171035,-448.084163299895));
#34351=CARTESIAN_POINT('Ctrl Pts',(-50.8836206571549,49.3944460396681,-448.051620936223));
#34352=CARTESIAN_POINT('Ctrl Pts',(-50.910407185175,49.4120126230145,-448.019076743385));
#34353=CARTESIAN_POINT('Ctrl Pts',(-50.937191959849,49.4295812775534,-447.986532194121));
#34354=CARTESIAN_POINT('Ctrl Pts',(-51.8660508056535,50.0388378561823,-446.857932352111));
#34355=CARTESIAN_POINT('Ctrl Pts',(-52.7941858068855,50.6489043755752,-445.729225486989));
#34356=CARTESIAN_POINT('Ctrl Pts',(-53.7224747742633,51.2587647535248,-444.600565757327));
#34357=CARTESIAN_POINT('Ctrl Pts',(-53.7271605052976,51.261843150231,-444.594868613325));
#34358=CARTESIAN_POINT('Ctrl Pts',(-53.7318462431683,51.2649215382768,-444.589171471241));
#34359=CARTESIAN_POINT('Ctrl Pts',(-53.7365319880393,51.267999917474,-444.583474331106));
#34360=CARTESIAN_POINT('Ctrl Pts',(-53.7372116654306,51.2684464430104,-444.582647948653));
#34361=CARTESIAN_POINT('Ctrl Pts',(-53.7378913429692,51.2688929683606,-444.581821566241));
#34362=CARTESIAN_POINT('Ctrl Pts',(-53.7388204928419,51.2695033882821,-444.580691864483));
#34363=CARTESIAN_POINT('Ctrl Pts',(-53.7390699650489,51.2696672830144,-444.580388545105));
#34364=CARTESIAN_POINT('Ctrl Pts',(-54.7181919280243,51.9129168722811,-443.389928730339));
#34365=CARTESIAN_POINT('Ctrl Pts',(-55.6973702941219,52.5556178438312,-442.199858435399));
#34366=CARTESIAN_POINT('Ctrl Pts',(-56.679031605489,53.2002765515568,-441.006505296162));
#34367=CARTESIAN_POINT('Ctrl Pts',(-56.6817117793207,53.2020366288693,-441.003247150217));
#34368=CARTESIAN_POINT('Ctrl Pts',(-56.7434607329299,53.2425873884486,-440.928182158226));
#34369=CARTESIAN_POINT('Ctrl Pts',(-56.8025295142029,53.28137806923,-440.856375312376));
#34370=CARTESIAN_POINT('Ctrl Pts',(-56.8615982954759,53.3201687500114,-440.784568466526));
#34371=CARTESIAN_POINT('Ctrl Pts',(-38.7260050947043,41.8439701681072,-462.499999999991));
#34372=CARTESIAN_POINT('Ctrl Pts',(-39.7581488632683,42.4378961980291,-461.30888084498));
#34373=CARTESIAN_POINT('Ctrl Pts',(-40.7917548038261,43.0326645465224,-460.119458028552));
#34374=CARTESIAN_POINT('Ctrl Pts',(-41.8245239512239,43.626994046764,-458.928756936488));
#34375=CARTESIAN_POINT('Ctrl Pts',(-41.8679853926983,43.6520048798785,-458.878649334071));
#34376=CARTESIAN_POINT('Ctrl Pts',(-41.9114453828767,43.6770149534938,-458.828539484164));
#34377=CARTESIAN_POINT('Ctrl Pts',(-41.9549034402465,43.7020239930474,-458.778427000744));
#34378=CARTESIAN_POINT('Ctrl Pts',(-42.4550391675447,43.9898397617028,-458.201709014284));
#34379=CARTESIAN_POINT('Ctrl Pts',(-42.9549096455548,44.2775132286661,-457.624637324207));
#34380=CARTESIAN_POINT('Ctrl Pts',(-43.4537405807944,44.5646025967642,-457.046602172866));
#34381=CARTESIAN_POINT('Ctrl Pts',(-43.7001095917822,44.7063939707285,-456.761114769235));
#34382=CARTESIAN_POINT('Ctrl Pts',(-43.9419698999314,44.8551488759503,-456.475325681066));
#34383=CARTESIAN_POINT('Ctrl Pts',(-44.1835266720058,45.0037713435814,-456.18927385616));
#34384=CARTESIAN_POINT('Ctrl Pts',(-44.4192537156373,45.1488069582364,-455.910125602806));
#34385=CARTESIAN_POINT('Ctrl Pts',(-44.6535849761086,45.2955323849931,-455.630698788494));
#34386=CARTESIAN_POINT('Ctrl Pts',(-44.886288729578,45.4442130759016,-455.350948844508));
#34387=CARTESIAN_POINT('Ctrl Pts',(-45.1859479231632,45.6356733994895,-454.990706943076));
#34388=CARTESIAN_POINT('Ctrl Pts',(-45.4826555081698,45.8306756180597,-454.629880205933));
#34389=CARTESIAN_POINT('Ctrl Pts',(-45.7774232248994,46.0279911825921,-454.268666023506));
#34390=CARTESIAN_POINT('Ctrl Pts',(-46.46147678895,46.4858921245897,-453.430413274473));
#34391=CARTESIAN_POINT('Ctrl Pts',(-47.1369084672023,46.9540575683327,-452.590421585279));
#34392=CARTESIAN_POINT('Ctrl Pts',(-47.8179110823453,47.4154734155314,-451.75158474533));
#34393=CARTESIAN_POINT('Ctrl Pts',(-48.227608388324,47.6930653444455,-451.246932948346));
#34394=CARTESIAN_POINT('Ctrl Pts',(-48.6393914253937,47.9681385721777,-450.74271823329));
#34395=CARTESIAN_POINT('Ctrl Pts',(-49.052377467942,48.2417626627977,-450.238765523087));
#34396=CARTESIAN_POINT('Ctrl Pts',(-49.6192015161921,48.6173121941742,-449.547089568225));
#34397=CARTESIAN_POINT('Ctrl Pts',(-50.1877167394984,48.9908264298899,-448.855780448404));
#34398=CARTESIAN_POINT('Ctrl Pts',(-50.7564246854722,49.3640848801747,-448.164542776848));
#34399=CARTESIAN_POINT('Ctrl Pts',(-50.7569731977418,49.3644448836548,-448.163876086068));
#34400=CARTESIAN_POINT('Ctrl Pts',(-50.7575217081349,49.3648048893754,-448.163209394885));
#34401=CARTESIAN_POINT('Ctrl Pts',(-50.7580702166158,49.3651648973791,-448.162542703291));
#34402=CARTESIAN_POINT('Ctrl Pts',(-50.7795966697881,49.3792935675887,-448.136378102604));
#34403=CARTESIAN_POINT('Ctrl Pts',(-50.8011200552037,49.3934259023882,-448.110212841121));
#34404=CARTESIAN_POINT('Ctrl Pts',(-50.8226387422926,49.4075638745383,-448.084046539819));
#34405=CARTESIAN_POINT('Ctrl Pts',(-50.8494004945451,49.425146587948,-448.051504774145));
#34406=CARTESIAN_POINT('Ctrl Pts',(-50.8761540272635,49.4427391729914,-448.018961179735));
#34407=CARTESIAN_POINT('Ctrl Pts',(-50.902905790027,49.4603338398603,-447.986417229284));
#34408=CARTESIAN_POINT('Ctrl Pts',(-51.8306198285471,50.0704924900249,-446.857838153238));
#34409=CARTESIAN_POINT('Ctrl Pts',(-52.757590048565,50.6814738682486,-445.729152514807));
#34410=CARTESIAN_POINT('Ctrl Pts',(-53.6847122806995,51.2922527600448,-444.600512549515));
#34411=CARTESIAN_POINT('Ctrl Pts',(-53.6893921223957,51.29533579314,-444.594815505278));
#34412=CARTESIAN_POINT('Ctrl Pts',(-53.6940719708786,51.2984188176681,-444.589118462921));
#34413=CARTESIAN_POINT('Ctrl Pts',(-53.6987518263143,51.3015018334394,-444.583421422477));
#34414=CARTESIAN_POINT('Ctrl Pts',(-53.6994306494303,51.3019490315209,-444.582595054483));
#34415=CARTESIAN_POINT('Ctrl Pts',(-53.7001094726926,51.3023962294181,-444.581768686531));
#34416=CARTESIAN_POINT('Ctrl Pts',(-53.70103745473,51.3030075687442,-444.580639004539));
#34417=CARTESIAN_POINT('Ctrl Pts',(-53.7012866133788,51.3031717103323,-444.580335690467));
#34418=CARTESIAN_POINT('Ctrl Pts',(-54.6791779309502,51.9473901540065,-443.389896703558));
#34419=CARTESIAN_POINT('Ctrl Pts',(-55.6571239136289,52.5910637358582,-442.199845592215));
#34420=CARTESIAN_POINT('Ctrl Pts',(-56.6375685971972,53.2366909931355,-441.006507784646));
#34421=CARTESIAN_POINT('Ctrl Pts',(-56.6402454494806,53.2384537147748,-441.003249680531));
#34422=CARTESIAN_POINT('Ctrl Pts',(-56.7019178806694,53.2790653962921,-440.928185651597));
#34423=CARTESIAN_POINT('Ctrl Pts',(-56.7609134609269,53.3179143547354,-440.856379727003));
#34424=CARTESIAN_POINT('Ctrl Pts',(-56.8199090411844,53.3567633131786,-440.78457380241));
#34425=CARTESIAN_POINT('Ctrl Pts',(-38.7066184322078,41.8615969349749,-462.499999999991));
#34426=CARTESIAN_POINT('Ctrl Pts',(-39.7374669075845,42.4567575797274,-461.308854598505));
#34427=CARTESIAN_POINT('Ctrl Pts',(-40.7697797858423,43.0527636978772,-460.11939686498));
#34428=CARTESIAN_POINT('Ctrl Pts',(-41.8012731618041,43.6482966761564,-458.928662949044));
#34429=CARTESIAN_POINT('Ctrl Pts',(-41.8446809157088,43.6733581545582,-458.878553965319));
#34430=CARTESIAN_POINT('Ctrl Pts',(-41.8880872489384,43.6984188127329,-458.82844273781));
#34431=CARTESIAN_POINT('Ctrl Pts',(-41.9314916811027,43.723478373327,-458.778328881298));
#34432=CARTESIAN_POINT('Ctrl Pts',(-42.4310102643594,44.0118755618356,-458.201595092646));
#34433=CARTESIAN_POINT('Ctrl Pts',(-42.9302678025629,44.300122035912,-457.624508197589));
#34434=CARTESIAN_POINT('Ctrl Pts',(-43.428491712953,44.5877717446927,-457.046459661188));
#34435=CARTESIAN_POINT('Ctrl Pts',(-43.6745609187339,44.7298398668897,-456.760965646773));
#34436=CARTESIAN_POINT('Ctrl Pts',(-43.9161228645122,44.8788684306205,-456.475170391752));
#34437=CARTESIAN_POINT('Ctrl Pts',(-44.1573829231518,45.027760954572,-456.189112991235));
#34438=CARTESIAN_POINT('Ctrl Pts',(-44.3928204142273,45.1730601080112,-455.909959296831));
#34439=CARTESIAN_POINT('Ctrl Pts',(-44.6268636924482,45.3200456431357,-455.630527604515));
#34440=CARTESIAN_POINT('Ctrl Pts',(-44.8592812255079,45.4689825357462,-455.350773482467));
#34441=CARTESIAN_POINT('Ctrl Pts',(-45.1585718449904,45.6607727774995,-454.990526200827));
#34442=CARTESIAN_POINT('Ctrl Pts',(-45.454913777456,45.8560984360299,-454.629695244152));
#34443=CARTESIAN_POINT('Ctrl Pts',(-45.7493191722042,46.0537299453492,-454.268478295191));
#34444=CARTESIAN_POINT('Ctrl Pts',(-46.432531912689,46.5123640855408,-453.430219125993));
#34445=CARTESIAN_POINT('Ctrl Pts',(-47.1071407038709,46.9812223627475,-452.590228841659));
#34446=CARTESIAN_POINT('Ctrl Pts',(-47.7873434799765,47.4432779689052,-451.751404884973));
#34447=CARTESIAN_POINT('Ctrl Pts',(-48.1965595955874,47.7212547825704,-451.246760838677));
#34448=CARTESIAN_POINT('Ctrl Pts',(-48.6078534738581,47.9967174641686,-450.742554391857));
#34449=CARTESIAN_POINT('Ctrl Pts',(-49.0203439912174,48.2707347658732,-450.238610296471));
#34450=CARTESIAN_POINT('Ctrl Pts',(-49.5864879302998,48.6468239801343,-449.546946165461));
#34451=CARTESIAN_POINT('Ctrl Pts',(-50.1543110516816,49.0208849764366,-448.855649522369));
#34452=CARTESIAN_POINT('Ctrl Pts',(-50.7223190449954,49.3946951658807,-448.16442453839));
#34453=CARTESIAN_POINT('Ctrl Pts',(-50.7228668821688,49.3950557015069,-448.163757859847));
#34454=CARTESIAN_POINT('Ctrl Pts',(-50.7234147174583,49.3954162393782,-448.163091180901));
#34455=CARTESIAN_POINT('Ctrl Pts',(-50.7239625508283,49.3957767795372,-448.162424501545));
#34456=CARTESIAN_POINT('Ctrl Pts',(-50.745462508981,49.4099263344135,-448.136260381121));
#34457=CARTESIAN_POINT('Ctrl Pts',(-50.7669593881346,49.4240795610099,-448.110095600202));
#34458=CARTESIAN_POINT('Ctrl Pts',(-50.7884515579436,49.4382384319732,-448.083929779741));
#34459=CARTESIAN_POINT('Ctrl Pts',(-50.8151803319354,49.4558471362279,-448.051388612068));
#34460=CARTESIAN_POINT('Ctrl Pts',(-50.8419008693521,49.4734657229684,-448.018845616087));
#34461=CARTESIAN_POINT('Ctrl Pts',(-50.868619620205,49.4910864021673,-447.986302264447));
#34462=CARTESIAN_POINT('Ctrl Pts',(-51.7951888514407,50.1021471238675,-446.857743954364));
#34463=CARTESIAN_POINT('Ctrl Pts',(-52.7209942902445,50.714043360922,-445.729079542625));
#34464=CARTESIAN_POINT('Ctrl Pts',(-53.6469497871357,51.3257407665647,-444.600459341703));
#34465=CARTESIAN_POINT('Ctrl Pts',(-53.6516237394938,51.328828436049,-444.594762397231));
#34466=CARTESIAN_POINT('Ctrl Pts',(-53.6562976985889,51.3319160970593,-444.589065454601));
#34467=CARTESIAN_POINT('Ctrl Pts',(-53.6609716645893,51.3350037494048,-444.583368513846));
#34468=CARTESIAN_POINT('Ctrl Pts',(-53.66164963343,51.3354516200314,-444.582542160313));
#34469=CARTESIAN_POINT('Ctrl Pts',(-53.662327602416,51.3358994904756,-444.581715806821));
#34470=CARTESIAN_POINT('Ctrl Pts',(-53.663254416618,51.3365117492062,-444.580586144595));
#34471=CARTESIAN_POINT('Ctrl Pts',(-53.6635032617087,51.3366761376502,-444.58028283583));
#34472=CARTESIAN_POINT('Ctrl Pts',(-54.6401639338761,51.9818634357318,-443.389864676778));
#34473=CARTESIAN_POINT('Ctrl Pts',(-55.6168775331359,52.6265096278852,-442.199832749031));
#34474=CARTESIAN_POINT('Ctrl Pts',(-56.5961055889053,53.2731054347143,-441.00651027313));
#34475=CARTESIAN_POINT('Ctrl Pts',(-56.5987791196405,53.2748708006803,-441.003252210846));
#34476=CARTESIAN_POINT('Ctrl Pts',(-56.660375028409,53.3155434041358,-440.928189144968));
#34477=CARTESIAN_POINT('Ctrl Pts',(-56.7192974076509,53.3544506402408,-440.85638414163));
#34478=CARTESIAN_POINT('Ctrl Pts',(-56.7782197868929,53.3933578763459,-440.784579138293));
#34479=CARTESIAN_POINT('Ctrl Pts',(-38.3840553815676,42.1548781377002,-462.499999999991));
#34480=CARTESIAN_POINT('Ctrl Pts',(-39.3933522504188,42.7705807981887,-461.308417899162));
#34481=CARTESIAN_POINT('Ctrl Pts',(-40.4041506405478,43.3871814233334,-460.118379200986));
#34482=CARTESIAN_POINT('Ctrl Pts',(-41.4144172206949,44.0027383509268,-458.927099148328));
#34483=CARTESIAN_POINT('Ctrl Pts',(-41.4569316993248,44.0286424858926,-458.876967181839));
#34484=CARTESIAN_POINT('Ctrl Pts',(-41.4994452667629,44.0545447902129,-458.826833033245));
#34485=CARTESIAN_POINT('Ctrl Pts',(-41.5419574612932,44.0804449401011,-458.776696330672));
#34486=CARTESIAN_POINT('Ctrl Pts',(-42.031207754961,44.378516024855,-458.199699618824));
#34487=CARTESIAN_POINT('Ctrl Pts',(-42.5202669553144,44.6762964206426,-457.622359737223));
#34488=CARTESIAN_POINT('Ctrl Pts',(-43.0083909432826,44.9732693019898,-457.044088494844));
#34489=CARTESIAN_POINT('Ctrl Pts',(-43.2494718700247,45.1199420720588,-456.758484487548));
#34490=CARTESIAN_POINT('Ctrl Pts',(-43.48606954325,45.2735238756008,-456.472586625987));
#34491=CARTESIAN_POINT('Ctrl Pts',(-43.7223927649944,45.4269097047084,-456.186436456212));
#34492=CARTESIAN_POINT('Ctrl Pts',(-43.9530125647411,45.5765937219271,-455.907192231443));
#34493=CARTESIAN_POINT('Ctrl Pts',(-44.1822642790075,45.7279070441918,-455.627679376945));
#34494=CARTESIAN_POINT('Ctrl Pts',(-44.4099195623238,45.8811067232721,-455.347855738637));
#34495=CARTESIAN_POINT('Ctrl Pts',(-44.7030776983524,46.0783862755194,-454.987518938944));
#34496=CARTESIAN_POINT('Ctrl Pts',(-44.9933357574793,46.2790934575717,-454.626617775994));
#34497=CARTESIAN_POINT('Ctrl Pts',(-45.2817126940726,46.4819817827217,-454.265354796337));
#34498=CARTESIAN_POINT('Ctrl Pts',(-45.9509354755063,46.9528151679476,-453.426988805868));
#34499=CARTESIAN_POINT('Ctrl Pts',(-46.6118527422302,47.4332010856463,-452.58702189615));
#34500=CARTESIAN_POINT('Ctrl Pts',(-47.2787474762744,47.9059012574457,-451.748412296366));
#34501=CARTESIAN_POINT('Ctrl Pts',(-47.6799573539367,48.1902819376597,-451.243897209111));
#34502=CARTESIAN_POINT('Ctrl Pts',(-48.0831124123112,48.4722245085679,-450.739828332511));
#34503=CARTESIAN_POINT('Ctrl Pts',(-48.4873581832285,48.7527842136913,-450.236027573909));
#34504=CARTESIAN_POINT('Ctrl Pts',(-49.0421861937476,49.1378528878107,-449.54456017288));
#34505=CARTESIAN_POINT('Ctrl Pts',(-49.598493846277,49.521011105607,-448.853471122598));
#34506=CARTESIAN_POINT('Ctrl Pts',(-50.15485574706,49.9040013520307,-448.162457239611));
#34507=CARTESIAN_POINT('Ctrl Pts',(-50.1553923517111,49.9043707417163,-448.161790764672));
#34508=CARTESIAN_POINT('Ctrl Pts',(-50.1559289543568,49.9047401337239,-448.161124289334));
#34509=CARTESIAN_POINT('Ctrl Pts',(-50.1564655549617,49.9051095280963,-448.160457813588));
#34510=CARTESIAN_POINT('Ctrl Pts',(-50.1775246783738,49.9196065704169,-448.134301683965));
#34511=CARTESIAN_POINT('Ctrl Pts',(-50.19858053573,49.9341074030923,-448.108144898866));
#34512=CARTESIAN_POINT('Ctrl Pts',(-50.2196315004226,49.9486139968755,-448.08198707884));
#34513=CARTESIAN_POINT('Ctrl Pts',(-50.2458115689115,49.9666551472137,-448.049455860921));
#34514=CARTESIAN_POINT('Ctrl Pts',(-50.2719831172911,49.9847063605971,-448.016922821836));
#34515=CARTESIAN_POINT('Ctrl Pts',(-50.2981526027619,50.0027598433546,-447.984389433468));
#34516=CARTESIAN_POINT('Ctrl Pts',(-51.2056740721611,50.6288295923436,-446.856176635811));
#34517=CARTESIAN_POINT('Ctrl Pts',(-52.1120994148901,51.2559476168219,-445.72786540226));
#34518=CARTESIAN_POINT('Ctrl Pts',(-53.0186423037857,51.8829276235022,-444.599574048826));
#34519=CARTESIAN_POINT('Ctrl Pts',(-53.0232182669799,51.8860924350838,-444.593878764279));
#34520=CARTESIAN_POINT('Ctrl Pts',(-53.0277942360827,51.8892572397411,-444.588183480956));
#34521=CARTESIAN_POINT('Ctrl Pts',(-53.0323702113011,51.8924220372635,-444.582488198884));
#34522=CARTESIAN_POINT('Ctrl Pts',(-53.0330339663677,51.8928810979642,-444.581662085947));
#34523=CARTESIAN_POINT('Ctrl Pts',(-53.0336977215629,51.8933401585148,-444.580835973034));
#34524=CARTESIAN_POINT('Ctrl Pts',(-53.0346051048533,51.8939677146664,-444.579706639678));
#34525=CARTESIAN_POINT('Ctrl Pts',(-53.034848732837,51.8941362103973,-444.579403419211));
#34526=CARTESIAN_POINT('Ctrl Pts',(-53.9910334341756,52.55544369592,-443.389331802383));
#34527=CARTESIAN_POINT('Ctrl Pts',(-54.9472421448168,53.2162725675843,-442.199619058995));
#34528=CARTESIAN_POINT('Ctrl Pts',(-55.9062274602824,53.8789834895428,-441.006551677525));
#34529=CARTESIAN_POINT('Ctrl Pts',(-55.9088457257679,53.8807928528758,-441.003294311226));
#34530=CARTESIAN_POINT('Ctrl Pts',(-55.9691684238764,53.9224790999222,-440.928247269069));
#34531=CARTESIAN_POINT('Ctrl Pts',(-56.0268728553218,53.962355983091,-440.856457593954));
#34532=CARTESIAN_POINT('Ctrl Pts',(-56.0845772867672,54.0022328662598,-440.784667918839));
#34533=CARTESIAN_POINT('Ctrl Pts',(-38.0485358858946,42.4342626183073,-462.49999999999));
#34534=CARTESIAN_POINT('Ctrl Pts',(-39.0356229365182,43.0696980016412,-461.308013965751));
#34535=CARTESIAN_POINT('Ctrl Pts',(-40.024611351385,43.7058204031952,-460.117292961907));
#34536=CARTESIAN_POINT('Ctrl Pts',(-41.0122388620067,44.3416392648618,-458.925224977469));
#34537=CARTESIAN_POINT('Ctrl Pts',(-41.0538006334439,44.3683960713702,-458.875059852891));
#34538=CARTESIAN_POINT('Ctrl Pts',(-41.0953600222231,44.3951523559108,-458.824892357397));
#34539=CARTESIAN_POINT('Ctrl Pts',(-41.1369165959835,44.4219078194676,-458.774722170664));
#34540=CARTESIAN_POINT('Ctrl Pts',(-41.6151691571787,44.729822255478,-458.197340107383));
#34541=CARTESIAN_POINT('Ctrl Pts',(-42.0930406432342,45.0376232051348,-457.619597236635));
#34542=CARTESIAN_POINT('Ctrl Pts',(-42.5698361712411,45.3448341513233,-457.040986313764));
#34543=CARTESIAN_POINT('Ctrl Pts',(-42.8053220530903,45.4965634279782,-456.755214540715));
#34544=CARTESIAN_POINT('Ctrl Pts',(-43.0367606506595,45.6544693989459,-456.469171724908));
#34545=CARTESIAN_POINT('Ctrl Pts',(-43.2678916148795,45.8122303117749,-456.182896741484));
#34546=CARTESIAN_POINT('Ctrl Pts',(-43.4934444669871,45.9661838244933,-455.903530715316));
#34547=CARTESIAN_POINT('Ctrl Pts',(-43.7177199550653,46.1216144233747,-455.623918373332));
#34548=CARTESIAN_POINT('Ctrl Pts',(-43.9405112854632,46.2787488604059,-455.344024006501));
#34549=CARTESIAN_POINT('Ctrl Pts',(-44.2274059719884,46.481095311562,-454.983596127692));
#34550=CARTESIAN_POINT('Ctrl Pts',(-44.5116147019647,46.6865336179401,-454.622656992109));
#34551=CARTESIAN_POINT('Ctrl Pts',(-44.7940809283859,46.8939195056093,-454.261399114584));
#34552=CARTESIAN_POINT('Ctrl Pts',(-45.4495870029688,47.3751901724509,-453.423044964395));
#34553=CARTESIAN_POINT('Ctrl Pts',(-46.0973324307058,47.8649979689372,-452.583283464107));
#34554=CARTESIAN_POINT('Ctrl Pts',(-46.750484847807,48.3475659606927,-451.744900168167));
#34555=CARTESIAN_POINT('Ctrl Pts',(-47.1434272238412,48.637883210256,-451.240521227343));
#34556=CARTESIAN_POINT('Ctrl Pts',(-47.5380826456442,48.9259784554183,-450.73658927729));
#34557=CARTESIAN_POINT('Ctrl Pts',(-47.9336785752366,49.2128162688131,-450.232930506939));
#34558=CARTESIAN_POINT('Ctrl Pts',(-48.4766346637746,49.60650165725,-449.541657985025));
#34559=CARTESIAN_POINT('Ctrl Pts',(-49.0208509935435,49.9984361157421,-448.850787354041));
#34560=CARTESIAN_POINT('Ctrl Pts',(-49.5650274806359,50.3902365781675,-448.160009139721));
#34561=CARTESIAN_POINT('Ctrl Pts',(-49.5655523325958,50.3906144652049,-448.159342892082));
#34562=CARTESIAN_POINT('Ctrl Pts',(-49.5660771826899,50.3909923543223,-448.158676644111));
#34563=CARTESIAN_POINT('Ctrl Pts',(-49.5666020308868,50.3913702455573,-448.158010395802));
#34564=CARTESIAN_POINT('Ctrl Pts',(-49.5871999259553,50.4062007509343,-448.13186319202));
#34565=CARTESIAN_POINT('Ctrl Pts',(-49.6077947898249,50.4210346498013,-448.105715441795));
#34566=CARTESIAN_POINT('Ctrl Pts',(-49.628385178826,50.4358736949496,-448.079566806258));
#34567=CARTESIAN_POINT('Ctrl Pts',(-49.6539924515631,50.4543282990007,-448.047047010645));
#34568=CARTESIAN_POINT('Ctrl Pts',(-49.6795919556881,50.4727918877815,-448.014525649639));
#34569=CARTESIAN_POINT('Ctrl Pts',(-49.7051894407867,50.4912575287471,-447.982004029836));
#34570=CARTESIAN_POINT('Ctrl Pts',(-50.5928747304147,51.1316203528912,-446.854199349668));
#34571=CARTESIAN_POINT('Ctrl Pts',(-51.4793636318734,51.7729560277259,-445.726369506217));
#34572=CARTESIAN_POINT('Ctrl Pts',(-52.3659887730324,52.4141980326467,-444.598510963065));
#34573=CARTESIAN_POINT('Ctrl Pts',(-52.3704641972652,52.4174348346216,-444.592817863218));
#34574=CARTESIAN_POINT('Ctrl Pts',(-52.3749396275605,52.4206716311789,-444.587124763277));
#34575=CARTESIAN_POINT('Ctrl Pts',(-52.379415064135,52.42390842213,-444.581431663254));
#34576=CARTESIAN_POINT('Ctrl Pts',(-52.3800642358547,52.4243779256327,-444.580605866827));
#34577=CARTESIAN_POINT('Ctrl Pts',(-52.3807134077064,52.4248474290174,-444.579780070399));
#34578=CARTESIAN_POINT('Ctrl Pts',(-52.3816008549171,52.4254892610355,-444.57865116965));
#34579=CARTESIAN_POINT('Ctrl Pts',(-52.3818391301617,52.4256615897709,-444.578348065331));
#34580=CARTESIAN_POINT('Ctrl Pts',(-53.3170155448827,53.1020127665171,-443.388732293172));
#34581=CARTESIAN_POINT('Ctrl Pts',(-54.2522286275839,53.777948100645,-442.199416824245));
#34582=CARTESIAN_POINT('Ctrl Pts',(-55.190351532113,54.4559698826095,-441.006592867525));
#34583=CARTESIAN_POINT('Ctrl Pts',(-55.1929128395437,54.4578210495521,-441.003336164678));
#34584=CARTESIAN_POINT('Ctrl Pts',(-55.2519233041263,54.5004704453264,-440.928304381204));
#34585=CARTESIAN_POINT('Ctrl Pts',(-55.3083724586708,54.5412686723922,-440.856529302479));
#34586=CARTESIAN_POINT('Ctrl Pts',(-55.3648216132152,54.5820668994579,-440.784754223754));
#34587=CARTESIAN_POINT('Ctrl Pts',(-37.7015139289768,42.6984598857191,-462.499999999992));
#34588=CARTESIAN_POINT('Ctrl Pts',(-38.6656677555457,43.3526547647935,-461.307627240141));
#34589=CARTESIAN_POINT('Ctrl Pts',(-39.6321479825285,44.0070708483155,-460.116339751994));
#34590=CARTESIAN_POINT('Ctrl Pts',(-40.5960403389216,44.6623261314753,-458.923599022175));
#34591=CARTESIAN_POINT('Ctrl Pts',(-40.6366032772516,44.6899008699457,-458.873405586832));
#34592=CARTESIAN_POINT('Ctrl Pts',(-40.6771616557822,44.7174771073708,-458.823209590049));
#34593=CARTESIAN_POINT('Ctrl Pts',(-40.7177150805053,44.7450546030494,-458.773010768619));
#34594=CARTESIAN_POINT('Ctrl Pts',(-41.184422931611,45.0624293706537,-458.195299163805));
#34595=CARTESIAN_POINT('Ctrl Pts',(-41.6504677956014,45.3799668296249,-457.617209805434));
#34596=CARTESIAN_POINT('Ctrl Pts',(-42.1152192455461,45.697282757234,-457.038325670186));
#34597=CARTESIAN_POINT('Ctrl Pts',(-42.3447566438694,45.8540028115309,-456.75241895951));
#34598=CARTESIAN_POINT('Ctrl Pts',(-42.5708216095122,46.015940864641,-456.466268917899));
#34599=CARTESIAN_POINT('Ctrl Pts',(-42.7965272793444,46.177825518152,-456.179908704162));
#34600=CARTESIAN_POINT('Ctrl Pts',(-43.0167857710584,46.335803249241,-455.900459504629));
#34601=CARTESIAN_POINT('Ctrl Pts',(-43.2358810096817,46.495077391614,-455.620789119718));
#34602=CARTESIAN_POINT('Ctrl Pts',(-43.4536348320486,46.6558385524204,-455.340868446679));
#34603=CARTESIAN_POINT('Ctrl Pts',(-43.7340425772515,46.8628552381805,-454.980406692624));
#34604=CARTESIAN_POINT('Ctrl Pts',(-44.0120383736682,47.072560028791,-454.619493541349));
#34605=CARTESIAN_POINT('Ctrl Pts',(-44.2884645672501,47.2839543133247,-454.25830384698));
#34606=CARTESIAN_POINT('Ctrl Pts',(-44.9299538219574,47.7745270780749,-453.420107926229));
#34607=CARTESIAN_POINT('Ctrl Pts',(-45.5643443466039,48.2725707246637,-452.580680637434));
#34608=CARTESIAN_POINT('Ctrl Pts',(-46.203310866777,48.7643743207005,-451.742523665027));
#34609=CARTESIAN_POINT('Ctrl Pts',(-46.5877188794695,49.0602477929697,-451.238280882478));
#34610=CARTESIAN_POINT('Ctrl Pts',(-46.9736034978234,49.3541840440922,-450.734458758233));
#34611=CARTESIAN_POINT('Ctrl Pts',(-47.3602852066659,49.6470247257858,-450.230896972499));
#34612=CARTESIAN_POINT('Ctrl Pts',(-47.8910065120105,50.0489490612078,-449.539757562139));
#34613=CARTESIAN_POINT('Ctrl Pts',(-48.4228027385423,50.4493248931892,-448.849014551141));
#34614=CARTESIAN_POINT('Ctrl Pts',(-48.954498800334,50.8495967064915,-448.158370168331));
#34615=CARTESIAN_POINT('Ctrl Pts',(-48.9550116150673,50.8499827640495,-448.157704049771));
#34616=CARTESIAN_POINT('Ctrl Pts',(-48.9555244281821,50.8503688233494,-448.157037930955));
#34617=CARTESIAN_POINT('Ctrl Pts',(-48.9560372396523,50.8507548844229,-448.156371811876));
#34618=CARTESIAN_POINT('Ctrl Pts',(-48.9761627481588,50.865906018653,-448.13022967979));
#34619=CARTESIAN_POINT('Ctrl Pts',(-48.9962856325201,50.8810599944751,-448.104087122759));
#34620=CARTESIAN_POINT('Ctrl Pts',(-49.0164046910113,50.8962182734208,-448.077943857189));
#34621=CARTESIAN_POINT('Ctrl Pts',(-49.0414257927484,50.9150698931336,-448.045430739947));
#34622=CARTESIAN_POINT('Ctrl Pts',(-49.066440270253,50.9339290234222,-448.012916363251));
#34623=CARTESIAN_POINT('Ctrl Pts',(-49.0914529239671,50.9527898809208,-447.980401815122));
#34624=CARTESIAN_POINT('Ctrl Pts',(-49.9588570721109,51.6068582664193,-446.852842370824));
#34625=CARTESIAN_POINT('Ctrl Pts',(-50.8250953085433,52.2617567039541,-445.725315370698));
#34626=CARTESIAN_POINT('Ctrl Pts',(-51.6914750408701,52.9165575812234,-444.597742047636));
#34627=CARTESIAN_POINT('Ctrl Pts',(-51.6958482722041,52.9198628244178,-444.592050387496));
#34628=CARTESIAN_POINT('Ctrl Pts',(-51.7002215093043,52.9231680625987,-444.586358726709));
#34629=CARTESIAN_POINT('Ctrl Pts',(-51.7045947523765,52.9264732956039,-444.580667065271));
#34630=CARTESIAN_POINT('Ctrl Pts',(-51.7052291007084,52.926952726774,-444.579841477514));
#34631=CARTESIAN_POINT('Ctrl Pts',(-51.7058634491659,52.9274321578352,-444.579015889744));
#34632=CARTESIAN_POINT('Ctrl Pts',(-51.7067306321233,52.9280875614446,-444.577887274224));
#34633=CARTESIAN_POINT('Ctrl Pts',(-51.7069634665143,52.928263534087,-444.577584246486));
#34634=CARTESIAN_POINT('Ctrl Pts',(-52.6207857604491,53.6189162247599,-443.388269030704));
#34635=CARTESIAN_POINT('Ctrl Pts',(-53.5346367726972,54.3091680481,-442.199229111192));
#34636=CARTESIAN_POINT('Ctrl Pts',(-54.4513541348557,55.0016680018326,-441.00663068191));
#34637=CARTESIAN_POINT('Ctrl Pts',(-54.453857000037,55.0035586986396,-441.00337459443));
#34638=CARTESIAN_POINT('Ctrl Pts',(-54.5115210061605,55.0471188509615,-440.928356979771));
#34639=CARTESIAN_POINT('Ctrl Pts',(-54.5666821443815,55.0887883037915,-440.856595454873));
#34640=CARTESIAN_POINT('Ctrl Pts',(-54.6218432826024,55.1304577566214,-440.784833929974));
#34641=CARTESIAN_POINT('Ctrl Pts',(-37.6313113290433,42.751907037111,-462.499999999992));
#34642=CARTESIAN_POINT('Ctrl Pts',(-38.5908257605495,43.4098969653116,-461.307549005485));
#34643=CARTESIAN_POINT('Ctrl Pts',(-39.5527525773585,44.068013863756,-460.116146917469));
#34644=CARTESIAN_POINT('Ctrl Pts',(-40.5118433080807,44.727201138235,-458.923270091147));
#34645=CARTESIAN_POINT('Ctrl Pts',(-40.5522041823061,44.7549413444782,-458.873070928532));
#34646=CARTESIAN_POINT('Ctrl Pts',(-40.5925600562959,44.782683458509,-458.822869165933));
#34647=CARTESIAN_POINT('Ctrl Pts',(-40.6329105438009,44.8104272514234,-458.772664551699));
#34648=CARTESIAN_POINT('Ctrl Pts',(-41.0972828981243,45.1297158456914,-458.194886280578));
#34649=CARTESIAN_POINT('Ctrl Pts',(-41.5609352344926,45.4492230021257,-457.616726827702));
#34650=CARTESIAN_POINT('Ctrl Pts',(-42.0232501654307,45.7685831691666,-457.037787421545));
#34651=CARTESIAN_POINT('Ctrl Pts',(-42.2515841845416,45.9263128586153,-456.751853412964));
#34652=CARTESIAN_POINT('Ctrl Pts',(-42.4765620635468,46.0890666026172,-456.465681679556));
#34653=CARTESIAN_POINT('Ctrl Pts',(-42.7011701954168,46.2517854895581,-456.179304223712));
#34654=CARTESIAN_POINT('Ctrl Pts',(-42.9203576371376,46.4105773206966,-455.899838198193));
#34655=CARTESIAN_POINT('Ctrl Pts',(-43.1384049104296,46.5706290125608,-455.620156071188));
#34656=CARTESIAN_POINT('Ctrl Pts',(-43.3551396440792,46.7321238601938,-455.340230076399));
#34657=CARTESIAN_POINT('Ctrl Pts',(-43.6342350799674,46.9400853351954,-454.979761469377));
#34658=CARTESIAN_POINT('Ctrl Pts',(-43.9109739988857,47.1506532362798,-454.618853574731));
#34659=CARTESIAN_POINT('Ctrl Pts',(-44.1861782928139,47.3628584201697,-454.257677673826));
#34660=CARTESIAN_POINT('Ctrl Pts',(-44.8248319425155,47.8553130008829,-453.419513762917));
#34661=CARTESIAN_POINT('Ctrl Pts',(-45.456520768033,48.3550227613251,-452.580154085162));
#34662=CARTESIAN_POINT('Ctrl Pts',(-46.0926174788846,48.8486947216528,-451.742042898044));
#34663=CARTESIAN_POINT('Ctrl Pts',(-46.4752989884454,49.145692218705,-451.237827660337));
#34664=CARTESIAN_POINT('Ctrl Pts',(-46.8594092717944,49.4408101063103,-450.734027753871));
#34665=CARTESIAN_POINT('Ctrl Pts',(-47.244287632288,49.7348651692648,-450.230485588141));
#34666=CARTESIAN_POINT('Ctrl Pts',(-47.7725338389458,50.1384562450403,-449.539373106272));
#34667=CARTESIAN_POINT('Ctrl Pts',(-48.3018174765153,50.5405397682904,-448.848655912817));
#34668=CARTESIAN_POINT('Ctrl Pts',(-48.830988746181,50.9425253372923,-448.158038604143));
#34669=CARTESIAN_POINT('Ctrl Pts',(-48.8314991257813,50.9429130477479,-448.157372511697));
#34670=CARTESIAN_POINT('Ctrl Pts',(-48.8320095038132,50.9433007598771,-448.156706419009));
#34671=CARTESIAN_POINT('Ctrl Pts',(-48.8325198802515,50.9436884737103,-448.156040326072));
#34672=CARTESIAN_POINT('Ctrl Pts',(-48.8525498248776,50.958904471211,-448.129899219992));
#34673=CARTESIAN_POINT('Ctrl Pts',(-48.8725772277053,50.9741231986547,-448.103757713546));
#34674=CARTESIAN_POINT('Ctrl Pts',(-48.8926009359556,50.989346058651,-448.077615534322));
#34675=CARTESIAN_POINT('Ctrl Pts',(-48.9175034552013,51.0082779946986,-448.045103768114));
#34676=CARTESIAN_POINT('Ctrl Pts',(-48.9423995817228,51.0272171431003,-448.012590804346));
#34677=CARTESIAN_POINT('Ctrl Pts',(-48.96729392395,51.0461579529697,-447.980077686819));
#34678=CARTESIAN_POINT('Ctrl Pts',(-49.8305951937789,51.7029989758228,-446.852567853776));
#34679=CARTESIAN_POINT('Ctrl Pts',(-50.6927367172891,52.3606411625206,-445.725102118905));
#34680=CARTESIAN_POINT('Ctrl Pts',(-51.5550208000225,53.0181850019341,-444.597586495915));
#34681=CARTESIAN_POINT('Ctrl Pts',(-51.559373357716,53.0215040907987,-444.591895127029));
#34682=CARTESIAN_POINT('Ctrl Pts',(-51.5637259211157,53.0248231747315,-444.586203757383));
#34683=CARTESIAN_POINT('Ctrl Pts',(-51.5680784904252,53.0281422535756,-444.580512386972));
#34684=CARTESIAN_POINT('Ctrl Pts',(-51.5687098399833,53.0286236931145,-444.579686841428));
#34685=CARTESIAN_POINT('Ctrl Pts',(-51.5693411896657,53.0291051325464,-444.57886129587));
#34686=CARTESIAN_POINT('Ctrl Pts',(-51.5702042731612,53.029763281691,-444.577732738052));
#34687=CARTESIAN_POINT('Ctrl Pts',(-51.5704360068666,53.0299399914963,-444.577429725806));
#34688=CARTESIAN_POINT('Ctrl Pts',(-52.4799383585943,53.7234858808289,-443.388175312629));
#34689=CARTESIAN_POINT('Ctrl Pts',(-53.3894678204164,54.4166339323314,-442.19919113681));
#34690=CARTESIAN_POINT('Ctrl Pts',(-54.3018548377726,55.1120628226348,-441.006638331766));
#34691=CARTESIAN_POINT('Ctrl Pts',(-54.3043458800771,55.1139615163399,-441.003382368775));
#34692=CARTESIAN_POINT('Ctrl Pts',(-54.361737497429,55.1577059148643,-440.928367620467));
#34693=CARTESIAN_POINT('Ctrl Pts',(-54.4166380697321,55.1995516168126,-440.856608837506));
#34694=CARTESIAN_POINT('Ctrl Pts',(-54.4715386420352,55.241397318761,-440.784850054546));
#34695=CARTESIAN_POINT('Ctrl Pts',(-37.5606381983877,42.8047320086185,-462.499999999992));
#34696=CARTESIAN_POINT('Ctrl Pts',(-38.5154836291893,43.4664771562781,-461.307471475064));
#34697=CARTESIAN_POINT('Ctrl Pts',(-39.4728284330313,44.1282446737561,-460.11595952772));
#34698=CARTESIAN_POINT('Ctrl Pts',(-40.4270726428532,44.7913302408702,-458.92295131962));
#34699=CARTESIAN_POINT('Ctrl Pts',(-40.4672295636733,44.8192344967634,-458.87274662814));
#34700=CARTESIAN_POINT('Ctrl Pts',(-40.5073810149251,44.847141098464,-458.822539298062));
#34701=CARTESIAN_POINT('Ctrl Pts',(-40.5475266184879,44.8750498302346,-458.77232908952));
#34702=CARTESIAN_POINT('Ctrl Pts',(-41.0095410722123,45.1962366182965,-458.194486436468));
#34703=CARTESIAN_POINT('Ctrl Pts',(-41.4707747128536,45.5177018945107,-457.616259201806));
#34704=CARTESIAN_POINT('Ctrl Pts',(-41.9306238174049,45.8391009011587,-457.037267245341));
#34705=CARTESIAN_POINT('Ctrl Pts',(-42.1577399825993,45.9978375588247,-456.751307282541));
#34706=CARTESIAN_POINT('Ctrl Pts',(-42.3816219841029,46.1613950630015,-456.465115401567));
#34707=CARTESIAN_POINT('Ctrl Pts',(-42.6051230311094,46.3249379193904,-456.178722323756));
#34708=CARTESIAN_POINT('Ctrl Pts',(-42.8232301063401,46.4845338343074,-455.89924105329));
#34709=CARTESIAN_POINT('Ctrl Pts',(-43.040221055301,46.6453518941958,-455.619548880493));
#34710=CARTESIAN_POINT('Ctrl Pts',(-43.2559295886666,46.8075678422351,-455.339619382112));
#34711=CARTESIAN_POINT('Ctrl Pts',(-43.533703557475,47.0164578985896,-454.979146263414));
#34712=CARTESIAN_POINT('Ctrl Pts',(-43.8091788928938,47.2278699183855,-454.618246243049));
#34713=CARTESIAN_POINT('Ctrl Pts',(-44.0831559855213,47.4408660030456,-454.257086717384));
#34714=CARTESIAN_POINT('Ctrl Pts',(-44.7189617269349,47.9351559899446,-453.418960807727));
#34715=CARTESIAN_POINT('Ctrl Pts',(-45.3479413476419,48.4364833568867,-452.579674012533));
#34716=CARTESIAN_POINT('Ctrl Pts',(-45.9811500955024,48.9319978078526,-451.741608611509));
#34717=CARTESIAN_POINT('Ctrl Pts',(-46.3620941805204,49.2301037638653,-451.237420919129));
#34718=CARTESIAN_POINT('Ctrl Pts',(-46.7444190537688,49.526390552976,-450.733642121788));
#34719=CARTESIAN_POINT('Ctrl Pts',(-47.1274832847747,49.8216487675473,-450.230117735052));
#34720=CARTESIAN_POINT('Ctrl Pts',(-47.6532395956147,50.2268911709703,-449.539029654883));
#34721=CARTESIAN_POINT('Ctrl Pts',(-48.1799972723325,50.6306687557846,-448.848334564663));
#34722=CARTESIAN_POINT('Ctrl Pts',(-48.7066317741023,51.0343542998095,-448.157740164373));
#34723=CARTESIAN_POINT('Ctrl Pts',(-48.7071397070192,51.0347436498714,-448.157074094021));
#34724=CARTESIAN_POINT('Ctrl Pts',(-48.7076476384221,51.0351330015347,-448.156408023443));
#34725=CARTESIAN_POINT('Ctrl Pts',(-48.708155568287,51.0355223548284,-448.155741952633));
#34726=CARTESIAN_POINT('Ctrl Pts',(-48.7280894960771,51.0508026936685,-448.129601714899));
#34727=CARTESIAN_POINT('Ctrl Pts',(-48.7480209714833,51.0660856444756,-448.103461101891));
#34728=CARTESIAN_POINT('Ctrl Pts',(-48.7679488930859,51.0813725479371,-448.077319852977));
#34729=CARTESIAN_POINT('Ctrl Pts',(-48.7927322871024,51.1003841317505,-448.04480924375));
#34730=CARTESIAN_POINT('Ctrl Pts',(-48.8175095360115,51.1194026135235,-448.012297500911));
#34731=CARTESIAN_POINT('Ctrl Pts',(-48.8422850463451,51.1384226866356,-447.979785621856));
#34732=CARTESIAN_POINT('Ctrl Pts',(-49.7014653908732,51.7980124488417,-446.852318737373));
#34733=CARTESIAN_POINT('Ctrl Pts',(-50.559497538848,52.4583717597448,-445.724906964639));
#34734=CARTESIAN_POINT('Ctrl Pts',(-51.4176727221505,53.1186299287702,-444.59744300476));
#34735=CARTESIAN_POINT('Ctrl Pts',(-51.4220045393222,53.1219627187762,-444.591751896654));
#34736=CARTESIAN_POINT('Ctrl Pts',(-51.4263363621208,53.1252955038863,-444.586060787705));
#34737=CARTESIAN_POINT('Ctrl Pts',(-51.4306681907468,53.128628283949,-444.580369677911));
#34738=CARTESIAN_POINT('Ctrl Pts',(-51.431296531824,53.1291117108792,-444.57954417017));
#34739=CARTESIAN_POINT('Ctrl Pts',(-51.4319248730238,53.1295951377032,-444.578718662414));
#34740=CARTESIAN_POINT('Ctrl Pts',(-51.4327838437864,53.1302560037031,-444.577590156269));
#34741=CARTESIAN_POINT('Ctrl Pts',(-51.433014473243,53.1304334429709,-444.577287157896));
#34742=CARTESIAN_POINT('Ctrl Pts',(-52.3381828974584,53.8268423076476,-443.388087195484));
#34743=CARTESIAN_POINT('Ctrl Pts',(-53.2433759381523,54.5228543703159,-442.199153784258));
#34744=CARTESIAN_POINT('Ctrl Pts',(-54.1514103835472,55.2211781197432,-441.006645871012));
#34745=CARTESIAN_POINT('Ctrl Pts',(-54.1538895422346,55.2230847172935,-441.003390030542));
#34746=CARTESIAN_POINT('Ctrl Pts',(-54.211007370146,55.2670112178498,-440.928378103979));
#34747=CARTESIAN_POINT('Ctrl Pts',(-54.2656460366574,55.3090311178125,-440.856622020288));
#34748=CARTESIAN_POINT('Ctrl Pts',(-54.3202847031689,55.351051017775,-440.784865936597));
#34749=CARTESIAN_POINT('Ctrl Pts',(-37.4895054223497,42.8569273733703,-462.499999999992));
#34750=CARTESIAN_POINT('Ctrl Pts',(-38.4396517070487,43.5223865535762,-461.30739452007));
#34751=CARTESIAN_POINT('Ctrl Pts',(-39.3923845302881,44.1877558922935,-460.115776989513));
#34752=CARTESIAN_POINT('Ctrl Pts',(-40.3417425663939,44.854700825913,-458.922642054846));
#34753=CARTESIAN_POINT('Ctrl Pts',(-40.3816938651216,44.8827674933499,-458.872432030404));
#34754=CARTESIAN_POINT('Ctrl Pts',(-40.4216392077703,44.9108369620788,-458.822219329407));
#34755=CARTESIAN_POINT('Ctrl Pts',(-40.4615782246053,44.9389090304533,-458.772003723843));
#34756=CARTESIAN_POINT('Ctrl Pts',(-40.9212151812771,45.2619755728383,-458.194098959325));
#34757=CARTESIAN_POINT('Ctrl Pts',(-41.3800082970933,45.5853829698017,-457.615806314063));
#34758=CARTESIAN_POINT('Ctrl Pts',(-41.8373679432734,45.9088086873809,-457.03676440528));
#34759=CARTESIAN_POINT('Ctrl Pts',(-42.063254582884,46.0685463229984,-456.750779771391));
#34760=CARTESIAN_POINT('Ctrl Pts',(-42.2860324560788,46.2328960939693,-456.464569141792));
#34761=CARTESIAN_POINT('Ctrl Pts',(-42.5084177401601,46.3972524853508,-456.178161869978));
#34762=CARTESIAN_POINT('Ctrl Pts',(-42.7254359802761,46.5576423014161,-455.898666748067));
#34763=CARTESIAN_POINT('Ctrl Pts',(-42.941362733517,46.7192159075507,-455.618965976344));
#34764=CARTESIAN_POINT('Ctrl Pts',(-43.1560379722264,46.8821413693933,-455.339034467228));
#34765=CARTESIAN_POINT('Ctrl Pts',(-43.4324813383313,47.091945086705,-454.97855875925));
#34766=CARTESIAN_POINT('Ctrl Pts',(-43.7066854724977,47.3041847647207,-454.617668656292));
#34767=CARTESIAN_POINT('Ctrl Pts',(-43.9794286502786,47.5179548513687,-454.256527458661));
#34768=CARTESIAN_POINT('Ctrl Pts',(-44.6123709035941,48.0140410282453,-453.418444082009));
#34769=CARTESIAN_POINT('Ctrl Pts',(-45.2386289538674,48.5169464151524,-452.579233899357));
#34770=CARTESIAN_POINT('Ctrl Pts',(-45.8689315080284,49.0142786796981,-451.741214186485));
#34771=CARTESIAN_POINT('Ctrl Pts',(-46.2481272007452,49.3134782487302,-451.237053980509));
#34772=CARTESIAN_POINT('Ctrl Pts',(-46.6286559997937,49.6109208470317,-450.733295367014));
#34773=CARTESIAN_POINT('Ctrl Pts',(-47.0098959158467,49.9073700575108,-450.229787248531));
#34774=CARTESIAN_POINT('Ctrl Pts',(-47.5331483513002,50.3142471048499,-449.538721496565));
#34775=CARTESIAN_POINT('Ctrl Pts',(-48.0573675108946,50.7197032017148,-448.848045448175));
#34776=CARTESIAN_POINT('Ctrl Pts',(-48.5814538539718,51.1250730868311,-448.157470490684));
#34777=CARTESIAN_POINT('Ctrl Pts',(-48.5819593292189,51.1254640614206,-448.156804439085));
#34778=CARTESIAN_POINT('Ctrl Pts',(-48.5824648030095,51.1258550375369,-448.156138387274));
#34779=CARTESIAN_POINT('Ctrl Pts',(-48.5829702753206,51.1262460152077,-448.155472335249));
#34780=CARTESIAN_POINT('Ctrl Pts',(-48.6028077553457,51.1415901034307,-448.129332834687));
#34781=CARTESIAN_POINT('Ctrl Pts',(-48.6226428771039,51.1569366818667,-448.103192984056));
#34782=CARTESIAN_POINT('Ctrl Pts',(-48.6424745919669,51.1722870274805,-448.077052534873));
#34783=CARTESIAN_POINT('Ctrl Pts',(-48.6671383383061,51.1913775112361,-448.044542920233));
#34784=CARTESIAN_POINT('Ctrl Pts',(-48.6917961975074,51.2104745688835,-448.012032236872));
#34785=CARTESIAN_POINT('Ctrl Pts',(-48.7164523682614,51.229573145118,-447.979521434495));
#34786=CARTESIAN_POINT('Ctrl Pts',(-49.5714941816486,51.8918852867524,-446.852091887728));
#34787=CARTESIAN_POINT('Ctrl Pts',(-50.4254033950816,52.5549337315204,-445.724727758715));
#34788=CARTESIAN_POINT('Ctrl Pts',(-51.2794555464531,53.2178767746817,-444.597310199858));
#34789=CARTESIAN_POINT('Ctrl Pts',(-51.2837665517663,53.2212231171466,-444.59161932597));
#34790=CARTESIAN_POINT('Ctrl Pts',(-51.2880775626097,53.2245694547171,-444.585928451187));
#34791=CARTESIAN_POINT('Ctrl Pts',(-51.2923885791803,53.2279157872473,-444.580237575499));
#34792=CARTESIAN_POINT('Ctrl Pts',(-51.293013901424,53.2284011799921,-444.579412101718));
#34793=CARTESIAN_POINT('Ctrl Pts',(-51.2936392237882,53.2288865726309,-444.578586627916));
#34794=CARTESIAN_POINT('Ctrl Pts',(-51.2944940676643,53.229550125988,-444.577458168189));
#34795=CARTESIAN_POINT('Ctrl Pts',(-51.2947235890718,53.229728286798,-444.577155182282));
#34796=CARTESIAN_POINT('Ctrl Pts',(-52.1955431706003,53.9289690413498,-443.388004133628));
#34797=CARTESIAN_POINT('Ctrl Pts',(-53.096384092799,54.6278125449327,-442.199117108152));
#34798=CARTESIAN_POINT('Ctrl Pts',(-54.0000443626148,55.3289968257504,-441.006653315026));
#34799=CARTESIAN_POINT('Ctrl Pts',(-54.0025115786581,55.3309112334103,-441.003397594997));
#34800=CARTESIAN_POINT('Ctrl Pts',(-54.0593542561864,55.3750176761223,-440.928388442925));
#34801=CARTESIAN_POINT('Ctrl Pts',(-54.1137297150346,55.4172097079706,-440.8566350133));
#34802=CARTESIAN_POINT('Ctrl Pts',(-54.1681051738827,55.459401739819,-440.784881583676));
#34803=CARTESIAN_POINT('Ctrl Pts',(-37.2083128059277,43.0632591376727,-462.499999999992));
#34804=CARTESIAN_POINT('Ctrl Pts',(-38.1398830521092,43.7434001366877,-461.307090311834));
#34805=CARTESIAN_POINT('Ctrl Pts',(-39.0743844078769,44.42300771542,-460.115055403785));
#34806=CARTESIAN_POINT('Ctrl Pts',(-40.0044270728122,45.1052089826993,-458.921419510532));
#34807=CARTESIAN_POINT('Ctrl Pts',(-40.0435655336703,45.13391767382,-458.871188404532));
#34808=CARTESIAN_POINT('Ctrl Pts',(-40.0826961152396,45.1626309667934,-458.820954471935));
#34809=CARTESIAN_POINT('Ctrl Pts',(-40.121818480937,45.1913487156767,-458.770717531581));
#34810=CARTESIAN_POINT('Ctrl Pts',(-40.5720570329071,45.5218460524969,-458.19256723629));
#34811=CARTESIAN_POINT('Ctrl Pts',(-41.0212025910257,45.8529307825446,-457.614016018555));
#34812=CARTESIAN_POINT('Ctrl Pts',(-41.4687212419307,46.1843682238502,-457.034776644924));
#34813=CARTESIAN_POINT('Ctrl Pts',(-41.6897474847581,46.3480627921904,-456.748694484566));
#34814=CARTESIAN_POINT('Ctrl Pts',(-41.9081606649748,46.5155444467336,-456.462409740401));
#34815=CARTESIAN_POINT('Ctrl Pts',(-42.1261352636642,46.6831167962974,-456.175946358746));
#34816=CARTESIAN_POINT('Ctrl Pts',(-42.3388492658203,46.846644956646,-455.896396481149));
#34817=CARTESIAN_POINT('Ctrl Pts',(-42.550569182276,47.0112052875742,-455.616661717296));
#34818=CARTESIAN_POINT('Ctrl Pts',(-42.7611597381693,47.1769355048875,-455.33672225961));
#34819=CARTESIAN_POINT('Ctrl Pts',(-43.0323431428835,47.3903509850093,-454.976236316035));
#34820=CARTESIAN_POINT('Ctrl Pts',(-43.3015221335637,47.6058624512679,-454.615385417249));
#34821=CARTESIAN_POINT('Ctrl Pts',(-43.5693875635118,47.8226922194896,-454.254316671561));
#34822=CARTESIAN_POINT('Ctrl Pts',(-44.1910102570514,48.3258788553598,-453.41640143072));
#34823=CARTESIAN_POINT('Ctrl Pts',(-44.8065097575579,48.8350222606245,-452.577494102567));
#34824=CARTESIAN_POINT('Ctrl Pts',(-45.425323933847,49.3395404637074,-451.739654998012));
#34825=CARTESIAN_POINT('Ctrl Pts',(-45.7976081149786,49.643063158076,-451.235603447626));
#34826=CARTESIAN_POINT('Ctrl Pts',(-46.1710369127103,49.9450747473344,-450.731924622224));
#34827=CARTESIAN_POINT('Ctrl Pts',(-46.5450651898624,50.2462320442134,-450.228480813228));
#34828=CARTESIAN_POINT('Ctrl Pts',(-47.058419638616,50.6595709481716,-449.537503326142));
#34829=CARTESIAN_POINT('Ctrl Pts',(-47.5726038704107,51.0716623153226,-448.846902551382));
#34830=CARTESIAN_POINT('Ctrl Pts',(-48.0866171719202,51.4836905133122,-448.156404452575));
#34831=CARTESIAN_POINT('Ctrl Pts',(-48.0871129318347,51.4840879097679,-448.155738475105));
#34832=CARTESIAN_POINT('Ctrl Pts',(-48.0876086905194,51.4844853074556,-448.155072497485));
#34833=CARTESIAN_POINT('Ctrl Pts',(-48.0881044479561,51.4848827063976,-448.154406519712));
#34834=CARTESIAN_POINT('Ctrl Pts',(-48.1075606635219,51.5004788001911,-448.128269933244));
#34835=CARTESIAN_POINT('Ctrl Pts',(-48.1270148928715,51.5160769028946,-448.10213309634));
#34836=CARTESIAN_POINT('Ctrl Pts',(-48.1464662960652,51.5316780395761,-448.075995808548));
#34837=CARTESIAN_POINT('Ctrl Pts',(-48.1706570671417,51.5510804200746,-448.043490125577));
#34838=CARTESIAN_POINT('Ctrl Pts',(-48.1948429708511,51.5704880934038,-448.010983630402));
#34839=CARTESIAN_POINT('Ctrl Pts',(-48.2190273842736,51.5898969977258,-447.978477084207));
#34840=CARTESIAN_POINT('Ctrl Pts',(-49.0577093075446,52.2629708871368,-446.85119513592));
#34841=CARTESIAN_POINT('Ctrl Pts',(-49.8953202852591,52.9366496577472,-445.724019345728));
#34842=CARTESIAN_POINT('Ctrl Pts',(-50.7330738159265,53.610206187758,-444.596785213209));
#34843=CARTESIAN_POINT('Ctrl Pts',(-50.7373025505724,53.6136061039984,-444.591095265205));
#34844=CARTESIAN_POINT('Ctrl Pts',(-50.7415312903665,53.6170060153503,-444.585405316087));
#34845=CARTESIAN_POINT('Ctrl Pts',(-50.7457600354915,53.6204059216904,-444.579715365841));
#34846=CARTESIAN_POINT('Ctrl Pts',(-50.7463734240847,53.6208990854317,-444.578890026296));
#34847=CARTESIAN_POINT('Ctrl Pts',(-50.7469868127902,53.6213922490676,-444.578064686727));
#34848=CARTESIAN_POINT('Ctrl Pts',(-50.7478253428082,53.6220664257269,-444.576936410497));
#34849=CARTESIAN_POINT('Ctrl Pts',(-50.7480504840236,53.6222474388418,-444.576633473854));
#34850=CARTESIAN_POINT('Ctrl Pts',(-51.6316787998422,54.3326828432827,-443.387675784562));
#34851=CARTESIAN_POINT('Ctrl Pts',(-52.5153155068425,55.0427192219841,-442.198972125054));
#34852=CARTESIAN_POINT('Ctrl Pts',(-53.401684368333,55.7552113745149,-441.006682741713));
#34853=CARTESIAN_POINT('Ctrl Pts',(-53.4041043743063,55.7571566560599,-441.003427497796));
#34854=CARTESIAN_POINT('Ctrl Pts',(-53.4598593639825,55.8019744221367,-440.928429313338));
#34855=CARTESIAN_POINT('Ctrl Pts',(-53.5131943453476,55.8448469028314,-440.856686375285));
#34856=CARTESIAN_POINT('Ctrl Pts',(-53.5665293267126,55.8877193835262,-440.784943437231));
#34857=CARTESIAN_POINT('Ctrl Pts',(-36.9199317767795,43.2597666774808,-462.499999999992));
#34858=CARTESIAN_POINT('Ctrl Pts',(-37.8324549102319,43.9539458782433,-461.306795095633));
#34859=CARTESIAN_POINT('Ctrl Pts',(-38.7482571578729,44.647027599901,-460.114409634641));
#34860=CARTESIAN_POINT('Ctrl Pts',(-39.658365681366,45.3438748510546,-458.920345532314));
#34861=CARTESIAN_POINT('Ctrl Pts',(-39.6966652649939,45.3731998808534,-458.870096406233));
#34862=CARTESIAN_POINT('Ctrl Pts',(-39.7349547780735,45.4025315850734,-458.81984431378));
#34863=CARTESIAN_POINT('Ctrl Pts',(-39.7732339211675,45.4318698879971,-458.769589121741));
#34864=CARTESIAN_POINT('Ctrl Pts',(-40.2137682715346,45.7695088520574,-458.191228777496));
#34865=CARTESIAN_POINT('Ctrl Pts',(-40.6529256329602,46.108019773596,-457.612456043251));
#34866=CARTESIAN_POINT('Ctrl Pts',(-41.0902344735065,46.44727828479,-457.033059804923));
#34867=CARTESIAN_POINT('Ctrl Pts',(-41.3062181644335,46.6148356232938,-456.74690017022));
#34868=CARTESIAN_POINT('Ctrl Pts',(-41.5201379527339,46.7852690047599,-456.460563173376));
#34869=CARTESIAN_POINT('Ctrl Pts',(-41.7335664838255,46.9558937191734,-456.174065997285));
#34870=CARTESIAN_POINT('Ctrl Pts',(-41.9418441331284,47.1224005786326,-455.894483140846));
#34871=CARTESIAN_POINT('Ctrl Pts',(-42.1492344243933,47.2897780164087,-455.614736995588));
#34872=CARTESIAN_POINT('Ctrl Pts',(-42.355629639368,47.4581314476689,-455.334812918698));
#34873=CARTESIAN_POINT('Ctrl Pts',(-42.6214105851287,47.6749249144548,-454.974346781408));
#34874=CARTESIAN_POINT('Ctrl Pts',(-42.8854456343389,47.8934503728073,-454.613567015252));
#34875=CARTESIAN_POINT('Ctrl Pts',(-43.1483286166096,48.1130752521023,-454.252601238184));
#34876=CARTESIAN_POINT('Ctrl Pts',(-43.7583887783723,48.6227483706607,-453.414924951775));
#34877=CARTESIAN_POINT('Ctrl Pts',(-44.3629368138195,49.1375104332791,-452.576378766951));
#34878=CARTESIAN_POINT('Ctrl Pts',(-44.9699777257463,49.6488289529857,-451.738718740192));
#34879=CARTESIAN_POINT('Ctrl Pts',(-45.3351790050144,49.9564427790748,-451.234774924621));
#34880=CARTESIAN_POINT('Ctrl Pts',(-45.70134058345,50.2628191175988,-450.731161428449));
#34881=CARTESIAN_POINT('Ctrl Pts',(-46.067997071373,50.5684951457719,-450.227758321355));
#34882=CARTESIAN_POINT('Ctrl Pts',(-46.5712337268281,50.9880360161434,-449.5368366977));
#34883=CARTESIAN_POINT('Ctrl Pts',(-47.0751846899181,51.4065209593756,-448.846263357661));
#34884=CARTESIAN_POINT('Ctrl Pts',(-47.5789444621768,51.8249646754256,-448.155787962735));
#34885=CARTESIAN_POINT('Ctrl Pts',(-47.5794303326803,51.8253682595746,-448.155122007162));
#34886=CARTESIAN_POINT('Ctrl Pts',(-47.5799162022267,51.8257718446248,-448.154456051502));
#34887=CARTESIAN_POINT('Ctrl Pts',(-47.5804020708026,51.8261754305922,-448.153790095752));
#34888=CARTESIAN_POINT('Ctrl Pts',(-47.5994701937419,51.8420143368808,-448.127654373588));
#34889=CARTESIAN_POINT('Ctrl Pts',(-47.6185367754878,51.8578547120417,-448.101518502401));
#34890=CARTESIAN_POINT('Ctrl Pts',(-47.6376012071881,51.8736973011133,-448.075382335517));
#34891=CARTESIAN_POINT('Ctrl Pts',(-47.6613107205006,51.8933999642927,-448.042878046564));
#34892=CARTESIAN_POINT('Ctrl Pts',(-47.6850165472328,51.9131064885463,-448.01037321669));
#34893=CARTESIAN_POINT('Ctrl Pts',(-47.70872115003,51.9328139156338,-447.977868398389));
#34894=CARTESIAN_POINT('Ctrl Pts',(-48.5307639061233,52.6162401606172,-446.850646371043));
#34895=CARTESIAN_POINT('Ctrl Pts',(-49.351859747534,53.3001149112981,-445.723560185446));
#34896=CARTESIAN_POINT('Ctrl Pts',(-50.1730897445005,53.9838271096126,-444.596427251579));
#34897=CARTESIAN_POINT('Ctrl Pts',(-50.177235073184,53.9872782886944,-444.590737814395));
#34898=CARTESIAN_POINT('Ctrl Pts',(-50.1813804063884,53.9907294623442,-444.585048376292));
#34899=CARTESIAN_POINT('Ctrl Pts',(-50.185525744272,53.9941806304614,-444.579358937251));
#34900=CARTESIAN_POINT('Ctrl Pts',(-50.1861270344651,53.994681229834,-444.578533671858));
#34901=CARTESIAN_POINT('Ctrl Pts',(-50.1867283247567,53.9951818290902,-444.577708406444));
#34902=CARTESIAN_POINT('Ctrl Pts',(-50.1875503156819,53.9958661705609,-444.576580231593));
#34903=CARTESIAN_POINT('Ctrl Pts',(-50.18777101623,53.9960499128762,-444.576277322171));
#34904=CARTESIAN_POINT('Ctrl Pts',(-51.0539707121218,54.7171968052672,-443.387426468621));
#34905=CARTESIAN_POINT('Ctrl Pts',(-51.9201546955739,55.4379190446405,-442.198837749311));
#34906=CARTESIAN_POINT('Ctrl Pts',(-52.7888945371382,56.1611826490833,-441.006710716959));
#34907=CARTESIAN_POINT('Ctrl Pts',(-52.7912664106188,56.163157339747,-441.003455916653));
#34908=CARTESIAN_POINT('Ctrl Pts',(-52.8459124453165,56.2086526773579,-440.928467960805));
#34909=CARTESIAN_POINT('Ctrl Pts',(-52.8981866051577,56.2521733200442,-440.856734807396));
#34910=CARTESIAN_POINT('Ctrl Pts',(-52.9504607649989,56.2956939627305,-440.785001653987));
#34911=CARTESIAN_POINT('Ctrl Pts',(-36.6250350054762,43.44599737661,-462.499999999992));
#34912=CARTESIAN_POINT('Ctrl Pts',(-37.5180066093736,44.15348732022,-461.306500914477));
#34913=CARTESIAN_POINT('Ctrl Pts',(-38.4145575367227,44.8593642524127,-460.113803019785));
#34914=CARTESIAN_POINT('Ctrl Pts',(-39.3044366439474,45.5699226199423,-458.919379760096));
#34915=CARTESIAN_POINT('Ctrl Pts',(-39.3418849244615,45.5998246469174,-458.869115519798));
#34916=CARTESIAN_POINT('Ctrl Pts',(-39.3793213988626,45.6297349680817,-458.818848228504));
#34917=CARTESIAN_POINT('Ctrl Pts',(-39.4167458019573,45.659653565018,-458.768577792298));
#34918=CARTESIAN_POINT('Ctrl Pts',(-39.847443403123,46.0039708250165,-458.190042011011));
#34919=CARTESIAN_POINT('Ctrl Pts',(-40.2765397746495,46.3493827979472,-457.611088416315));
#34920=CARTESIAN_POINT('Ctrl Pts',(-40.7036203901279,46.6958551892692,-457.03156832762));
#34921=CARTESIAN_POINT('Ctrl Pts',(-40.9145524342622,46.8669754112811,-456.74534752411));
#34922=CARTESIAN_POINT('Ctrl Pts',(-41.1238833998925,47.0402069499242,-456.458971155554));
#34923=CARTESIAN_POINT('Ctrl Pts',(-41.3326840621497,47.2137094884313,-456.17245062354));
#34924=CARTESIAN_POINT('Ctrl Pts',(-41.536445531553,47.3830247186094,-455.892844974849));
#34925=CARTESIAN_POINT('Ctrl Pts',(-41.7394134450216,47.5530714696157,-455.613094645132));
#34926=CARTESIAN_POINT('Ctrl Pts',(-41.9415036422248,47.723927962429,-455.33318917845));
#34927=CARTESIAN_POINT('Ctrl Pts',(-42.2017408950516,47.9439446922492,-454.972747006051));
#34928=CARTESIAN_POINT('Ctrl Pts',(-42.4604567863254,48.1653822678638,-454.612034804759));
#34929=CARTESIAN_POINT('Ctrl Pts',(-42.7181653193154,48.3877287873109,-454.251163653175));
#34930=CARTESIAN_POINT('Ctrl Pts',(-43.3162173802191,48.9037178880493,-453.413706959669));
#34931=CARTESIAN_POINT('Ctrl Pts',(-43.9093206928263,49.4240297334006,-452.575484973039));
#34932=CARTESIAN_POINT('Ctrl Pts',(-44.5042986949365,49.9418368656499,-451.737996393529));
#34933=CARTESIAN_POINT('Ctrl Pts',(-44.8622428190275,50.2533542994772,-451.234155722167));
#34934=CARTESIAN_POINT('Ctrl Pts',(-45.2209889388158,50.5638744191451,-450.730604440263));
#34935=CARTESIAN_POINT('Ctrl Pts',(-45.5801392660453,50.8738318088303,-450.22723885709));
#34936=CARTESIAN_POINT('Ctrl Pts',(-46.0730737031377,51.2992488551844,-449.536368735082));
#34937=CARTESIAN_POINT('Ctrl Pts',(-46.5666196378205,51.723786943774,-448.845815383258));
#34938=CARTESIAN_POINT('Ctrl Pts',(-47.0599537059709,52.1483121119869,-448.155351859473));
#34939=CARTESIAN_POINT('Ctrl Pts',(-47.0604295210027,52.1487215616265,-448.154685915349));
#34940=CARTESIAN_POINT('Ctrl Pts',(-47.0609053353016,52.1491310119003,-448.154019971187));
#34941=CARTESIAN_POINT('Ctrl Pts',(-47.0613811488582,52.1495404628192,-448.153354026984));
#34942=CARTESIAN_POINT('Ctrl Pts',(-47.0800546582078,52.1656095416749,-448.12721875797));
#34943=CARTESIAN_POINT('Ctrl Pts',(-47.0987269925228,52.181679652834,-448.101083418635));
#34944=CARTESIAN_POINT('Ctrl Pts',(-47.1173977360254,52.1977513071622,-448.074947907397));
#34945=CARTESIAN_POINT('Ctrl Pts',(-47.1406176383329,52.2177388477424,-448.042444433842));
#34946=CARTESIAN_POINT('Ctrl Pts',(-47.1638348317754,52.2377290755748,-448.009940636929));
#34947=CARTESIAN_POINT('Ctrl Pts',(-47.1870510158254,52.257719953065,-447.9774368953));
#34948=CARTESIAN_POINT('Ctrl Pts',(-47.9921560870102,52.950975864979,-446.850252205454));
#34949=CARTESIAN_POINT('Ctrl Pts',(-48.7964083779301,53.6445747397623,-445.723217860489));
#34950=CARTESIAN_POINT('Ctrl Pts',(-49.6007898856695,54.3379719240151,-444.596151878923));
#34951=CARTESIAN_POINT('Ctrl Pts',(-49.6048501681102,54.3414719900715,-444.590462779695));
#34952=CARTESIAN_POINT('Ctrl Pts',(-49.6089104546008,54.3449720501023,-444.584773679848));
#34953=CARTESIAN_POINT('Ctrl Pts',(-49.6129707452809,54.3484721040223,-444.579084579361));
#34954=CARTESIAN_POINT('Ctrl Pts',(-49.6135596991939,54.348979794386,-444.578259363076));
#34955=CARTESIAN_POINT('Ctrl Pts',(-49.6141486531951,54.3494874846209,-444.577434146777));
#34956=CARTESIAN_POINT('Ctrl Pts',(-49.614953779844,54.3501815197612,-444.576306039075));
#34957=CARTESIAN_POINT('Ctrl Pts',(-49.6151699524152,54.3503678647776,-444.576003147684));
#34958=CARTESIAN_POINT('Ctrl Pts',(-50.4635983594652,55.0817297627234,-443.38722306242));
#34959=CARTESIAN_POINT('Ctrl Pts',(-51.3119941322142,55.8126389863823,-442.198718028092));
#34960=CARTESIAN_POINT('Ctrl Pts',(-52.1628056643231,56.5461223255794,-441.006738864584));
#34961=CARTESIAN_POINT('Ctrl Pts',(-52.1651285884545,56.5481249186544,-441.003484468476));
#34962=CARTESIAN_POINT('Ctrl Pts',(-52.2186468548831,56.594263105605,-440.92850583605));
#34963=CARTESIAN_POINT('Ctrl Pts',(-52.2698421964883,56.6383986951822,-440.856781601387));
#34964=CARTESIAN_POINT('Ctrl Pts',(-52.3210375380934,56.6825342847595,-440.785057366722));
#34965=CARTESIAN_POINT('Ctrl Pts',(-36.4766084300011,43.5397304642866,-462.499999999992));
#34966=CARTESIAN_POINT('Ctrl Pts',(-37.3597394155548,44.2539199318322,-461.306352848082));
#34967=CARTESIAN_POINT('Ctrl Pts',(-38.2466008250035,44.9662369117535,-460.11349770018));
#34968=CARTESIAN_POINT('Ctrl Pts',(-39.126298121938,45.6836963180454,-458.918893670464));
#34969=CARTESIAN_POINT('Ctrl Pts',(-39.163317927073,45.713888757542,-458.868621822924));
#34970=CARTESIAN_POINT('Ctrl Pts',(-39.2003250525556,45.7440903064847,-458.818346881794));
#34971=CARTESIAN_POINT('Ctrl Pts',(-39.2373192504284,45.7743009752964,-458.768068772937));
#34972=CARTESIAN_POINT('Ctrl Pts',(-39.6630658479214,46.1219795355618,-458.189444691194));
#34973=CARTESIAN_POINT('Ctrl Pts',(-40.0870983516069,46.4708649253793,-457.610400066349));
#34974=CARTESIAN_POINT('Ctrl Pts',(-40.5090309269309,46.8209681856273,-457.030817641651));
#34975=CARTESIAN_POINT('Ctrl Pts',(-40.7174203910613,46.9938816676861,-456.744566050838));
#34976=CARTESIAN_POINT('Ctrl Pts',(-40.9244417239637,47.1685215665686,-456.458169865827));
#34977=CARTESIAN_POINT('Ctrl Pts',(-41.1309131008923,47.3434725630331,-456.171637578378));
#34978=CARTESIAN_POINT('Ctrl Pts',(-41.3324014999132,47.5142012941004,-455.892020457959));
#34979=CARTESIAN_POINT('Ctrl Pts',(-41.5331435551981,47.6855915559898,-455.612268022131));
#34980=CARTESIAN_POINT('Ctrl Pts',(-41.7330669635199,47.8577078823811,-455.332371922285));
#34981=CARTESIAN_POINT('Ctrl Pts',(-41.9905139811264,48.0793469354703,-454.971941811825));
#34982=CARTESIAN_POINT('Ctrl Pts',(-42.2465526494743,48.3022502293791,-454.611263617082));
#34983=CARTESIAN_POINT('Ctrl Pts',(-42.5016567938734,48.5259665967417,-454.250440092116));
#34984=CARTESIAN_POINT('Ctrl Pts',(-43.0936649727752,49.045134639052,-453.413093923464));
#34985=CARTESIAN_POINT('Ctrl Pts',(-43.6810079611479,49.5682397847237,-452.575035111317));
#34986=CARTESIAN_POINT('Ctrl Pts',(-44.269914494973,50.0893127463512,-451.737632824132));
#34987=CARTESIAN_POINT('Ctrl Pts',(-44.6242059690676,50.4027949325426,-451.233844067009));
#34988=CARTESIAN_POINT('Ctrl Pts',(-44.9792197620226,50.7154006879465,-450.730324098608));
#34989=CARTESIAN_POINT('Ctrl Pts',(-45.3345921105317,51.0275129599142,-450.226977401865));
#34990=CARTESIAN_POINT('Ctrl Pts',(-45.8223412653823,51.4558875858787,-449.536133201512));
#34991=CARTESIAN_POINT('Ctrl Pts',(-46.3106501717744,51.8834723257838,-448.8455899101));
#34992=CARTESIAN_POINT('Ctrl Pts',(-46.7987368052008,52.3110583926103,-448.155132361262));
#34993=CARTESIAN_POINT('Ctrl Pts',(-46.7992075591422,52.3114707944515,-448.1544664229));
#34994=CARTESIAN_POINT('Ctrl Pts',(-46.7996783124634,52.3118831967924,-448.153800484525));
#34995=CARTESIAN_POINT('Ctrl Pts',(-46.8001490651575,52.3122955996415,-448.153134546134));
#34996=CARTESIAN_POINT('Ctrl Pts',(-46.8186239587558,52.3284805282765,-448.126999505198));
#34997=CARTESIAN_POINT('Ctrl Pts',(-46.8370978616136,52.3446662694824,-448.100864433553));
#34998=CARTESIAN_POINT('Ctrl Pts',(-46.8555704551306,52.3608532162617,-448.074729252314));
#34999=CARTESIAN_POINT('Ctrl Pts',(-46.8785439278674,52.3809841404973,-448.042226189162));
#35000=CARTESIAN_POINT('Ctrl Pts',(-46.9015151838398,52.4011171611805,-448.009722912155));
#35001=CARTESIAN_POINT('Ctrl Pts',(-46.9244855384026,52.4212507040935,-447.977219712434));
#35002=CARTESIAN_POINT('Ctrl Pts',(-47.7210655838424,53.1194540550525,-446.85005381519));
#35003=CARTESIAN_POINT('Ctrl Pts',(-48.5168402284758,53.817947247375,-445.723045562498));
#35004=CARTESIAN_POINT('Ctrl Pts',(-49.3127416041782,54.5162190502612,-444.596013279167));
#35005=CARTESIAN_POINT('Ctrl Pts',(-49.3167590813941,54.5197437219659,-444.590324350038));
#35006=CARTESIAN_POINT('Ctrl Pts',(-49.320776562423,54.5232683873462,-444.584635420441));
#35007=CARTESIAN_POINT('Ctrl Pts',(-49.3247940473947,54.5267930463247,-444.578946490355));
#35008=CARTESIAN_POINT('Ctrl Pts',(-49.3253767922476,54.5273043057051,-444.578121298786));
#35009=CARTESIAN_POINT('Ctrl Pts',(-49.3259595371832,54.5278155649508,-444.577296107207));
#35010=CARTESIAN_POINT('Ctrl Pts',(-49.3267561757542,54.5285144790801,-444.576168033304));
#35011=CARTESIAN_POINT('Ctrl Pts',(-49.3269700693174,54.5287021340803,-444.575865150988));
#35012=CARTESIAN_POINT('Ctrl Pts',(-50.166453883543,55.2652054185741,-443.387120684609));
#35013=CARTESIAN_POINT('Ctrl Pts',(-51.005896546406,56.0012419251978,-442.19865777036));
#35014=CARTESIAN_POINT('Ctrl Pts',(-51.847684454537,56.7398690312296,-441.006753031764));
#35015=CARTESIAN_POINT('Ctrl Pts',(-51.8499827416259,56.7418856680639,-441.003498839095));
#35016=CARTESIAN_POINT('Ctrl Pts',(-51.9029333830493,56.7883474120568,-440.928524899335));
#35017=CARTESIAN_POINT('Ctrl Pts',(-51.9535857370357,56.8327925148976,-440.856805153656));
#35018=CARTESIAN_POINT('Ctrl Pts',(-52.0042380910221,56.8772376177383,-440.785085407977));
#35019=CARTESIAN_POINT('Ctrl Pts',(-36.3265298420472,43.6308599885747,-462.499999999992));
#35020=CARTESIAN_POINT('Ctrl Pts',(-37.1996924263205,44.3515646943029,-461.306205043894));
#35021=CARTESIAN_POINT('Ctrl Pts',(-38.0767245769759,45.0701497336524,-460.113202298343));
#35022=CARTESIAN_POINT('Ctrl Pts',(-38.9461654620509,45.7942733563001,-458.918434989852));
#35023=CARTESIAN_POINT('Ctrl Pts',(-38.9827536523909,45.8247462422545,-458.868156271143));
#35024=CARTESIAN_POINT('Ctrl Pts',(-39.0193284050684,45.8552289382071,-458.817874430222));
#35025=CARTESIAN_POINT('Ctrl Pts',(-39.055889488618,45.8857214801469,-458.767589410541));
#35026=CARTESIAN_POINT('Ctrl Pts',(-39.4766516031382,46.2366439687069,-458.188885795776));
#35027=CARTESIAN_POINT('Ctrl Pts',(-39.8956019078602,46.588869745845,-457.60976043929));
#35028=CARTESIAN_POINT('Ctrl Pts',(-40.3123818868539,46.9424500599523,-457.030124041237));
#35029=CARTESIAN_POINT('Ctrl Pts',(-40.5182265207175,47.117080833903,-456.743845793373));
#35030=CARTESIAN_POINT('Ctrl Pts',(-40.7229140991737,47.2930901910441,-456.45743305462));
#35031=CARTESIAN_POINT('Ctrl Pts',(-40.9270355202662,47.4694454308959,-456.170891655718));
#35032=CARTESIAN_POINT('Ctrl Pts',(-41.1262306772588,47.6415445153561,-455.891265643742));
#35033=CARTESIAN_POINT('Ctrl Pts',(-41.3247234268514,47.814240849281,-455.611512924627));
#35034=CARTESIAN_POINT('Ctrl Pts',(-41.5224523086685,47.9875865726217,-455.331627009372));
#35035=CARTESIAN_POINT('Ctrl Pts',(-41.7770733725339,48.210808754874,-454.971210013896));
#35036=CARTESIAN_POINT('Ctrl Pts',(-42.0303904861937,48.4351519609238,-454.610564921474));
#35037=CARTESIAN_POINT('Ctrl Pts',(-42.2828416508517,48.6602195653475,-454.249786909219));
#35038=CARTESIAN_POINT('Ctrl Pts',(-42.8686931845577,49.1825233598961,-453.412546359771));
#35039=CARTESIAN_POINT('Ctrl Pts',(-43.4501509656181,49.7084043601187,-452.574641362324));
#35040=CARTESIAN_POINT('Ctrl Pts',(-44.0329126558366,50.2326641877339,-451.737323434432));
#35041=CARTESIAN_POINT('Ctrl Pts',(-44.3835073366807,50.5480636212026,-451.23358542862));
#35042=CARTESIAN_POINT('Ctrl Pts',(-44.7347523585696,50.8626983517476,-450.730095988748));
#35043=CARTESIAN_POINT('Ctrl Pts',(-45.0863145944221,51.1769041993063,-450.226767380469));
#35044=CARTESIAN_POINT('Ctrl Pts',(-45.5688343631488,51.6081522613428,-449.535948006564));
#35045=CARTESIAN_POINT('Ctrl Pts',(-46.051866847541,52.0386948751203,-448.8454129045));
#35046=CARTESIAN_POINT('Ctrl Pts',(-46.5346672429426,52.4692542469965,-448.154958604317));
#35047=CARTESIAN_POINT('Ctrl Pts',(-46.5351328983683,52.4696695165561,-448.154292669089));
#35048=CARTESIAN_POINT('Ctrl Pts',(-46.5355985532749,52.4700847864969,-448.153626733868));
#35049=CARTESIAN_POINT('Ctrl Pts',(-46.5360642076574,52.4705000568251,-448.15296079865));
#35050=CARTESIAN_POINT('Ctrl Pts',(-46.5543390158089,52.486797520918,-448.126825882315));
#35051=CARTESIAN_POINT('Ctrl Pts',(-46.5726129985307,52.5030956034475,-448.100690969133));
#35052=CARTESIAN_POINT('Ctrl Pts',(-46.590885924727,52.5193945911968,-448.074556000714));
#35053=CARTESIAN_POINT('Ctrl Pts',(-46.6136110808565,52.5396648553776,-448.04205320224));
#35054=CARTESIAN_POINT('Ctrl Pts',(-46.6363344623507,52.5599366896367,-448.009550285811));
#35055=CARTESIAN_POINT('Ctrl Pts',(-46.6590570386816,52.5802089368378,-447.97704746389));
#35056=CARTESIAN_POINT('Ctrl Pts',(-47.4470444786043,53.2832223601798,-446.849894668207));
#35057=CARTESIAN_POINT('Ctrl Pts',(-48.2342679927543,53.9864843524237,-445.722902977322));
#35058=CARTESIAN_POINT('Ctrl Pts',(-49.0216147906279,54.6895066857866,-444.595895746019));
#35059=CARTESIAN_POINT('Ctrl Pts',(-49.0255890868387,54.6930553367788,-444.590206943346));
#35060=CARTESIAN_POINT('Ctrl Pts',(-49.0295633866179,54.6966039811641,-444.584518140382));
#35061=CARTESIAN_POINT('Ctrl Pts',(-49.0335376900874,54.700152618871,-444.578829337106));
#35062=CARTESIAN_POINT('Ctrl Pts',(-49.0341141713702,54.7006673564177,-444.578004163932));
#35063=CARTESIAN_POINT('Ctrl Pts',(-49.0346906527306,54.7011820938238,-444.577178990751));
#35064=CARTESIAN_POINT('Ctrl Pts',(-49.035478728706,54.7018857627464,-444.576050942003));
#35065=CARTESIAN_POINT('Ctrl Pts',(-49.0356903232536,54.7020746943845,-444.575748066442));
#35066=CARTESIAN_POINT('Ctrl Pts',(-49.8661510191605,55.4435884902993,-443.387030112924));
#35067=CARTESIAN_POINT('Ctrl Pts',(-50.6965617967901,56.1846220730185,-442.19860142409));
#35068=CARTESIAN_POINT('Ctrl Pts',(-51.5292502964639,56.928253159528,-441.006767441799));
#35069=CARTESIAN_POINT('Ctrl Pts',(-51.5315237396241,56.9302834584019,-441.003513442585));
#35070=CARTESIAN_POINT('Ctrl Pts',(-51.5839019901038,56.9770599633293,-440.928543966134));
#35071=CARTESIAN_POINT('Ctrl Pts',(-51.6340067973954,57.0218061651152,-440.856828490035));
#35072=CARTESIAN_POINT('Ctrl Pts',(-51.6841116046869,57.0665523669012,-440.785113013937));
#35073=CARTESIAN_POINT('Ctrl Pts',(-36.1748926818072,43.719331120904,-462.499999999992));
#35074=CARTESIAN_POINT('Ctrl Pts',(-37.0379548305357,44.4463560888641,-461.30605648736));
#35075=CARTESIAN_POINT('Ctrl Pts',(-37.9050017202358,45.1710409795027,-460.112919510267));
#35076=CARTESIAN_POINT('Ctrl Pts',(-38.7641455383955,45.9015411849164,-458.918015765539));
#35077=CARTESIAN_POINT('Ctrl Pts',(-38.8003004030767,45.9322824130066,-458.86773130526));
#35078=CARTESIAN_POINT('Ctrl Pts',(-38.836441276667,45.9630339403556,-458.817443718184));
#35079=CARTESIAN_POINT('Ctrl Pts',(-38.8725679428437,45.9937958220965,-458.767152961549));
#35080=CARTESIAN_POINT('Ctrl Pts',(-39.288330578282,46.3478179995397,-458.188383323229));
#35081=CARTESIAN_POINT('Ctrl Pts',(-39.7022105061783,46.703211031918,-457.609193372195));
#35082=CARTESIAN_POINT('Ctrl Pts',(-40.1138740358445,47.0600563389859,-457.029515743679));
#35083=CARTESIAN_POINT('Ctrl Pts',(-40.3171916921862,47.2362996694757,-456.743217132386));
#35084=CARTESIAN_POINT('Ctrl Pts',(-40.5195236792124,47.4136404438748,-456.456792590743));
#35085=CARTESIAN_POINT('Ctrl Pts',(-40.7212794045083,47.5913518598966,-456.170245768125));
#35086=CARTESIAN_POINT('Ctrl Pts',(-40.9181659593801,47.7647743905864,-455.890614463328));
#35087=CARTESIAN_POINT('Ctrl Pts',(-41.1143879832752,47.9387398116063,-455.610863743241));
#35088=CARTESIAN_POINT('Ctrl Pts',(-41.3098930235588,48.1132901226562,-455.330988558208));
#35089=CARTESIAN_POINT('Ctrl Pts',(-41.5616503838927,48.3380634865121,-454.970585380343));
#35090=CARTESIAN_POINT('Ctrl Pts',(-41.8121923904017,48.5638380597795,-454.60997068752));
#35091=CARTESIAN_POINT('Ctrl Pts',(-42.0619290902754,48.7902603788824,-454.249233490737));
#35092=CARTESIAN_POINT('Ctrl Pts',(-42.6414812933395,49.3157079960141,-453.412087659836));
#35093=CARTESIAN_POINT('Ctrl Pts',(-43.2168880235552,49.8444141500828,-452.574318560928));
#35094=CARTESIAN_POINT('Ctrl Pts',(-43.7934308880573,50.3717913051393,-451.737082281518));
#35095=CARTESIAN_POINT('Ctrl Pts',(-44.1402842673473,50.6890661508696,-451.233393396167));
#35096=CARTESIAN_POINT('Ctrl Pts',(-44.4877284502663,51.005671883583,-450.729933812533));
#35097=CARTESIAN_POINT('Ctrl Pts',(-44.835455089325,51.3219052879597,-450.226622807157));
#35098=CARTESIAN_POINT('Ctrl Pts',(-45.3127104949056,51.7559361751894,-449.535827593268));
#35099=CARTESIAN_POINT('Ctrl Pts',(-45.7904378177086,52.1893383421085,-448.845299007264));
#35100=CARTESIAN_POINT('Ctrl Pts',(-46.2679227237807,52.622775348591,-448.154844964195));
#35101=CARTESIAN_POINT('Ctrl Pts',(-46.2683832524782,52.6231933935963,-448.154179029215));
#35102=CARTESIAN_POINT('Ctrl Pts',(-46.2688437807351,52.623611438893,-448.153513094256));
#35103=CARTESIAN_POINT('Ctrl Pts',(-46.2693043085481,52.6240294844856,-448.152847159317));
#35104=CARTESIAN_POINT('Ctrl Pts',(-46.2873779222567,52.640435865038,-448.126712253849));
#35105=CARTESIAN_POINT('Ctrl Pts',(-46.3054508392597,52.656842716909,-448.100577375332));
#35106=CARTESIAN_POINT('Ctrl Pts',(-46.3235228985128,52.673250241708,-448.074442481881));
#35107=CARTESIAN_POINT('Ctrl Pts',(-46.3459982461223,52.6936554881774,-448.041939776636));
#35108=CARTESIAN_POINT('Ctrl Pts',(-46.3684721674282,52.7140618959818,-448.009437025237));
#35109=CARTESIAN_POINT('Ctrl Pts',(-46.3909453552282,52.7344686413403,-447.976934377398));
#35110=CARTESIAN_POINT('Ctrl Pts',(-47.1702843467058,53.4421462742838,-446.849787618707));
#35111=CARTESIAN_POINT('Ctrl Pts',(-47.9488861626814,54.1500539505149,-445.722799052326));
#35112=CARTESIAN_POINT('Ctrl Pts',(-48.7276050737667,54.857706910967,-444.595804874112));
#35113=CARTESIAN_POINT('Ctrl Pts',(-48.7315358189299,54.8612789360096,-444.590116137326));
#35114=CARTESIAN_POINT('Ctrl Pts',(-48.7354665673788,54.8648509542079,-444.584427400473));
#35115=CARTESIAN_POINT('Ctrl Pts',(-48.7393973192287,54.8684229654936,-444.578738663531));
#35116=CARTESIAN_POINT('Ctrl Pts',(-48.7399674832552,54.8689410934282,-444.577913499979));
#35117=CARTESIAN_POINT('Ctrl Pts',(-48.7405376473532,54.8694592212174,-444.577088336424));
#35118=CARTESIAN_POINT('Ctrl Pts',(-48.7413170873395,54.8701675249388,-444.575960300843));
#35119=CARTESIAN_POINT('Ctrl Pts',(-48.7415263631654,54.8703577009971,-444.575657428817));
#35120=CARTESIAN_POINT('Ctrl Pts',(-49.5628865989681,55.6167555612587,-443.386953354745));
#35121=CARTESIAN_POINT('Ctrl Pts',(-50.3841865870562,56.3626616466884,-442.198548263877));
#35122=CARTESIAN_POINT('Ctrl Pts',(-51.207704839932,57.1111550019579,-441.006781019456));
#35123=CARTESIAN_POINT('Ctrl Pts',(-51.2099532458194,57.1131985758379,-441.003527202775));
#35124=CARTESIAN_POINT('Ctrl Pts',(-51.261754652298,57.1602809218721,-440.928561939201));
#35125=CARTESIAN_POINT('Ctrl Pts',(-51.3113076531195,57.2053196899347,-440.856850493122));
#35126=CARTESIAN_POINT('Ctrl Pts',(-51.360860653941,57.2503584579972,-440.785139047043));
#35127=CARTESIAN_POINT('Ctrl Pts',(-35.9475629882934,43.8519642786695,-462.499999999992));
#35128=CARTESIAN_POINT('Ctrl Pts',(-36.7954828795889,44.5884643863239,-461.305833776046));
#35129=CARTESIAN_POINT('Ctrl Pts',(-37.6475601780025,45.322293983457,-460.112495563219));
#35130=CARTESIAN_POINT('Ctrl Pts',(-38.4912669551212,46.0623537625501,-458.917387277545));
#35131=CARTESIAN_POINT('Ctrl Pts',(-38.5267721915119,46.0934972807872,-458.867094209685));
#35132=CARTESIAN_POINT('Ctrl Pts',(-38.5622626071291,46.1246518317674,-458.816798008153));
#35133=CARTESIAN_POINT('Ctrl Pts',(-38.5977380083514,46.155817499324,-458.766498650856));
#35134=CARTESIAN_POINT('Ctrl Pts',(-39.0060055809331,46.5144866335072,-458.187630032083));
#35135=CARTESIAN_POINT('Ctrl Pts',(-39.4122841582898,46.8746279159974,-457.608343242923));
#35136=CARTESIAN_POINT('Ctrl Pts',(-39.8162772669613,47.2363679985138,-457.028603802983));
#35137=CARTESIAN_POINT('Ctrl Pts',(-40.0158065575446,47.4150288233912,-456.742274663472));
#35138=CARTESIAN_POINT('Ctrl Pts',(-40.214607115487,47.5943656169502,-456.455832427307));
#35139=CARTESIAN_POINT('Ctrl Pts',(-40.4128162635484,47.7741101699194,-456.169277473623));
#35140=CARTESIAN_POINT('Ctrl Pts',(-40.6062418342412,47.9495167698522,-455.889638233994));
#35141=CARTESIAN_POINT('Ctrl Pts',(-40.7990596571074,48.1253847665991,-455.609890510788));
#35142=CARTESIAN_POINT('Ctrl Pts',(-40.9912307836365,48.3017409579112,-455.330031412169));
#35143=CARTESIAN_POINT('Ctrl Pts',(-41.2386949690977,48.5288398047689,-454.969648949234));
#35144=CARTESIAN_POINT('Ctrl Pts',(-41.4850766216601,48.7567602390532,-454.609079830539));
#35145=CARTESIAN_POINT('Ctrl Pts',(-41.7307438807284,48.9852135040821,-454.248403823038));
#35146=CARTESIAN_POINT('Ctrl Pts',(-42.3008523240842,49.5153742418177,-453.411399991223));
#35147=CARTESIAN_POINT('Ctrl Pts',(-42.8671875079075,50.0483157782754,-452.573834627159));
#35148=CARTESIAN_POINT('Ctrl Pts',(-43.4344073031703,50.5803663332472,-451.736720752602));
#35149=CARTESIAN_POINT('Ctrl Pts',(-43.775651840048,50.9004527384523,-451.233105507114));
#35150=CARTESIAN_POINT('Ctrl Pts',(-44.1173979239211,51.2200133360429,-450.729690683017));
#35151=CARTESIAN_POINT('Ctrl Pts',(-44.4593743560895,51.5392863902607,-450.226406067365));
#35152=CARTESIAN_POINT('Ctrl Pts',(-44.9287375928996,51.977489202085,-449.535647073417));
#35153=CARTESIAN_POINT('Ctrl Pts',(-45.3985115831802,52.4151783217421,-448.845128256085));
#35154=CARTESIAN_POINT('Ctrl Pts',(-45.8680276737047,52.8529293881298,-448.154674598474));
#35155=CARTESIAN_POINT('Ctrl Pts',(-45.8684805165712,52.8533515939961,-448.154008663867));
#35156=CARTESIAN_POINT('Ctrl Pts',(-45.8689333591152,52.8537738000197,-448.153342729301));
#35157=CARTESIAN_POINT('Ctrl Pts',(-45.8693862013353,52.8541960062022,-448.152676794776));
#35158=CARTESIAN_POINT('Ctrl Pts',(-45.8871581906202,52.8707656709084,-448.126541905606));
#35159=CARTESIAN_POINT('Ctrl Pts',(-45.9049296761791,52.8873355863782,-448.100407079054));
#35160=CARTESIAN_POINT('Ctrl Pts',(-45.9227006019857,52.9039058265311,-448.07427229799));
#35161=CARTESIAN_POINT('Ctrl Pts',(-45.9448014444662,52.9245134342308,-448.041769732515));
#35162=CARTESIAN_POINT('Ctrl Pts',(-45.9669013828508,52.9451215904905,-448.00926722852));
#35163=CARTESIAN_POINT('Ctrl Pts',(-45.9890006951563,52.9657299712847,-447.976764841665));
#35164=CARTESIAN_POINT('Ctrl Pts',(-46.7553742029008,53.6804000415537,-446.84962713344));
#35165=CARTESIAN_POINT('Ctrl Pts',(-47.5210506383138,54.395272382088,-445.72264325122));
#35166=CARTESIAN_POINT('Ctrl Pts',(-48.2868348910593,55.1098674340124,-444.595668641787));
#35167=CARTESIAN_POINT('Ctrl Pts',(-48.2907003458527,55.1134745007011,-444.589980003779));
#35168=CARTESIAN_POINT('Ctrl Pts',(-48.2945658035078,55.1170815601898,-444.584291366036));
#35169=CARTESIAN_POINT('Ctrl Pts',(-48.2984312641301,55.1206886124145,-444.57860272854));
#35170=CARTESIAN_POINT('Ctrl Pts',(-48.2989919575233,55.1212118231128,-444.577777579412));
#35171=CARTESIAN_POINT('Ctrl Pts',(-48.299552650979,55.1217350336583,-444.57695243029));
#35172=CARTESIAN_POINT('Ctrl Pts',(-48.30031914416,55.1224502857254,-444.575824414447));
#35173=CARTESIAN_POINT('Ctrl Pts',(-48.300524943831,55.1226423273794,-444.575521547722));
#35174=CARTESIAN_POINT('Ctrl Pts',(-49.1082420541422,55.8763622243326,-443.386838281281));
#35175=CARTESIAN_POINT('Ctrl Pts',(-49.9158834311692,56.6295730136096,-442.198468567746));
#35176=CARTESIAN_POINT('Ctrl Pts',(-50.7256539365221,57.3853557303075,-441.006801374657));
#35177=CARTESIAN_POINT('Ctrl Pts',(-50.7278648073123,57.3874192056623,-441.003547831624));
#35178=CARTESIAN_POINT('Ctrl Pts',(-50.7788014272818,57.434960059129,-440.928588883822));
#35179=CARTESIAN_POINT('Ctrl Pts',(-50.8275271770784,57.4804374334134,-440.856883479385));
#35180=CARTESIAN_POINT('Ctrl Pts',(-50.876252926875,57.5259148076979,-440.785178074948));
#35181=CARTESIAN_POINT('Ctrl Pts',(-35.7167344653798,43.9786237267065,-462.499999999992));
#35182=CARTESIAN_POINT('Ctrl Pts',(-36.5492153513124,44.7241607642468,-461.305609373832));
#35183=CARTESIAN_POINT('Ctrl Pts',(-37.385971991095,45.4667569183785,-460.112099964991));
#35184=CARTESIAN_POINT('Ctrl Pts',(-38.2141497530743,46.2157296786755,-458.916847466227));
#35185=CARTESIAN_POINT('Ctrl Pts',(-38.2490014906803,46.247248276873,-458.86654832953));
#35186=CARTESIAN_POINT('Ctrl Pts',(-38.2838380373636,46.2787781663597,-458.816246106305));
#35187=CARTESIAN_POINT('Ctrl Pts',(-38.3186592191928,46.3103194452406,-458.765940786591));
#35188=CARTESIAN_POINT('Ctrl Pts',(-38.7193977278485,46.6733112908902,-458.187003549521));
#35189=CARTESIAN_POINT('Ctrl Pts',(-39.118101195542,47.0378116345601,-457.607656189956));
#35190=CARTESIAN_POINT('Ctrl Pts',(-39.5145047963644,47.4039698112403,-457.02788357782));
#35191=CARTESIAN_POINT('Ctrl Pts',(-39.7102856836097,47.5848127010472,-456.7415380548));
#35192=CARTESIAN_POINT('Ctrl Pts',(-39.9055055724271,47.7660599804359,-456.455088801439));
#35193=CARTESIAN_POINT('Ctrl Pts',(-40.1001326109166,47.9477296040555,-456.168534004658));
#35194=CARTESIAN_POINT('Ctrl Pts',(-40.2900625226301,48.1250148150051,-455.888894918146));
#35195=CARTESIAN_POINT('Ctrl Pts',(-40.4794278543523,48.302702230494,-455.609155321109));
#35196=CARTESIAN_POINT('Ctrl Pts',(-40.6681990411052,48.480808511884,-455.329313535));
#35197=CARTESIAN_POINT('Ctrl Pts',(-40.9112850281215,48.7101609991476,-454.968953365873));
#35198=CARTESIAN_POINT('Ctrl Pts',(-41.1533858001681,48.9402080524733,-454.608423746657));
#35199=CARTESIAN_POINT('Ctrl Pts',(-41.3948452851314,49.1707000470535,-454.24779837114));
#35200=CARTESIAN_POINT('Ctrl Pts',(-41.9551889452019,49.7055919684858,-453.410912038584));
#35201=CARTESIAN_POINT('Ctrl Pts',(-42.5120796284979,50.2428796389268,-452.573510142326));
#35202=CARTESIAN_POINT('Ctrl Pts',(-43.0698100792138,50.7794473054458,-451.736512580054));
#35203=CARTESIAN_POINT('Ctrl Pts',(-43.4053457409566,51.1022512456362,-451.232967309084));
#35204=CARTESIAN_POINT('Ctrl Pts',(-43.7413162638231,51.4246393226488,-450.729595690695));
#35205=CARTESIAN_POINT('Ctrl Pts',(-44.0774759502298,51.7468086495426,-450.226336299815));
#35206=CARTESIAN_POINT('Ctrl Pts',(-44.5388556935541,52.1889866005578,-449.535611926908));
#35207=CARTESIAN_POINT('Ctrl Pts',(-45.0005917476346,52.6307524990785,-448.845098958398));
#35208=CARTESIAN_POINT('Ctrl Pts',(-45.4620498885854,53.0726152328005,-448.154638776746));
#35209=CARTESIAN_POINT('Ctrl Pts',(-45.4624949596523,53.0730414043226,-448.153972835846));
#35210=CARTESIAN_POINT('Ctrl Pts',(-45.4629400304607,53.0734675759348,-448.153306894995));
#35211=CARTESIAN_POINT('Ctrl Pts',(-45.4633851010109,53.0738937476368,-448.152640954193));
#35212=CARTESIAN_POINT('Ctrl Pts',(-45.4808520877385,53.0906190408758,-448.126505818669));
#35213=CARTESIAN_POINT('Ctrl Pts',(-45.4983186766536,53.1073444726047,-448.100370758764));
#35214=CARTESIAN_POINT('Ctrl Pts',(-45.515784877734,53.1240700362378,-448.074235773136));
#35215=CARTESIAN_POINT('Ctrl Pts',(-45.5375067487839,53.1448708122511,-448.041732953258));
#35216=CARTESIAN_POINT('Ctrl Pts',(-45.5592280199817,53.1656717922767,-448.009230248262));
#35217=CARTESIAN_POINT('Ctrl Pts',(-45.5809487105189,53.1864729636486,-447.976727655573));
#35218=CARTESIAN_POINT('Ctrl Pts',(-46.3341921403375,53.9078287438245,-446.849582809351));
#35219=CARTESIAN_POINT('Ctrl Pts',(-47.086737395337,54.6294145238461,-445.722573035568));
#35220=CARTESIAN_POINT('Ctrl Pts',(-47.8393839597814,55.3507028414842,-444.595590722938));
#35221=CARTESIAN_POINT('Ctrl Pts',(-47.8431830993691,55.3543436938193,-444.589902046046));
#35222=CARTESIAN_POINT('Ctrl Pts',(-47.8469822415353,55.3579845385777,-444.584213369854));
#35223=CARTESIAN_POINT('Ctrl Pts',(-47.8507813863828,55.3616253756915,-444.578524694348));
#35224=CARTESIAN_POINT('Ctrl Pts',(-47.85133246053,55.3621534869608,-444.577699539707));
#35225=CARTESIAN_POINT('Ctrl Pts',(-47.8518835347336,55.3626815980692,-444.57687438508));
#35226=CARTESIAN_POINT('Ctrl Pts',(-47.8526368779575,55.3634035494146,-444.575746361725));
#35227=CARTESIAN_POINT('Ctrl Pts',(-47.8528391469287,55.363597389791,-444.575443492985));
#35228=CARTESIAN_POINT('Ctrl Pts',(-48.6466990572118,56.1243768599733,-443.386752320462));
#35229=CARTESIAN_POINT('Ctrl Pts',(-49.4404742924094,56.884628672487,-442.198393858917));
#35230=CARTESIAN_POINT('Ctrl Pts',(-50.2363376755567,57.6473823416216,-441.00681768439));
#35231=CARTESIAN_POINT('Ctrl Pts',(-50.2385105764817,57.6494648487129,-441.003564390457));
#35232=CARTESIAN_POINT('Ctrl Pts',(-50.2885724016608,57.6974441622301,-440.928611195469));
#35233=CARTESIAN_POINT('Ctrl Pts',(-50.336461326554,57.7433409654976,-440.856911294148));
#35234=CARTESIAN_POINT('Ctrl Pts',(-50.3843502514473,57.7892377687651,-440.785211392827));
#35235=CARTESIAN_POINT('Ctrl Pts',(-35.4827207341128,44.0991249603451,-462.499999999992));
#35236=CARTESIAN_POINT('Ctrl Pts',(-36.2994515423613,44.8532246984928,-461.305379862298));
#35237=CARTESIAN_POINT('Ctrl Pts',(-37.1204817421049,45.6042217030189,-460.111741809773));
#35238=CARTESIAN_POINT('Ctrl Pts',(-37.9331529959546,46.3612892574823,-458.916436947675));
#35239=CARTESIAN_POINT('Ctrl Pts',(-37.9673521819257,46.3931485043366,-458.866135607401));
#35240=CARTESIAN_POINT('Ctrl Pts',(-38.0015365664587,46.4250185004757,-458.815831315687));
#35241=CARTESIAN_POINT('Ctrl Pts',(-38.0357059902503,46.4568993332573,-458.765524060738));
#35242=CARTESIAN_POINT('Ctrl Pts',(-38.4289437614191,46.8237989246134,-458.186564552082));
#35243=CARTESIAN_POINT('Ctrl Pts',(-38.8202000143432,47.1921338048814,-457.607212569856));
#35244=CARTESIAN_POINT('Ctrl Pts',(-39.2092322209606,47.5620369281162,-457.027450190993));
#35245=CARTESIAN_POINT('Ctrl Pts',(-39.4013724296281,47.7447294200904,-456.741109722113));
#35246=CARTESIAN_POINT('Ctrl Pts',(-39.5929701347858,47.9278044479374,-456.454669146702));
#35247=CARTESIAN_POINT('Ctrl Pts',(-39.7839961708745,48.1112779928082,-456.168126315193));
#35248=CARTESIAN_POINT('Ctrl Pts',(-39.9704119867388,48.2903235891937,-455.888498905184));
#35249=CARTESIAN_POINT('Ctrl Pts',(-40.1562833938311,48.4697486991241,-455.608774115215));
#35250=CARTESIAN_POINT('Ctrl Pts',(-40.3415833236734,48.6495681499273,-455.328949954032));
#35251=CARTESIAN_POINT('Ctrl Pts',(-40.5801992751574,48.8811267338146,-454.968612481019));
#35252=CARTESIAN_POINT('Ctrl Pts',(-40.8178676002812,49.1133392152827,-454.608110230613));
#35253=CARTESIAN_POINT('Ctrl Pts',(-41.0549375578775,49.3459520531875,-454.247516228856));
#35254=CARTESIAN_POINT('Ctrl Pts',(-41.605094648424,49.8857657158846,-453.410702703908));
#35255=CARTESIAN_POINT('Ctrl Pts',(-42.1520299024585,50.4277350191744,-452.573395183637));
#35256=CARTESIAN_POINT('Ctrl Pts',(-42.700102688811,50.9686952648692,-451.736505220437));
#35257=CARTESIAN_POINT('Ctrl Pts',(-43.0298282127016,51.2941418202487,-451.233024682037));
#35258=CARTESIAN_POINT('Ctrl Pts',(-43.3599651617063,51.6192234296391,-450.729695153505));
#35259=CARTESIAN_POINT('Ctrl Pts',(-43.6902720539313,51.9441260974159,-450.226460975302));
#35260=CARTESIAN_POINT('Ctrl Pts',(-44.1436188272522,52.3900555634583,-449.535771206835));
#35261=CARTESIAN_POINT('Ctrl Pts',(-44.5972857048412,52.835647966713,-448.845261050184));
#35262=CARTESIAN_POINT('Ctrl Pts',(-45.0506493623309,53.2813834737626,-448.154786794391));
#35263=CARTESIAN_POINT('Ctrl Pts',(-45.0510866263617,53.2818133805301,-448.154120839917));
#35264=CARTESIAN_POINT('Ctrl Pts',(-45.0515238901104,53.2822432874305,-448.153454885476));
#35265=CARTESIAN_POINT('Ctrl Pts',(-45.0519611535773,53.2826731944639,-448.152788931068));
#35266=CARTESIAN_POINT('Ctrl Pts',(-45.0691217479385,53.2995450824021,-448.126653261581));
#35267=CARTESIAN_POINT('Ctrl Pts',(-45.0862819082435,53.3164171750821,-448.100517643539));
#35268=CARTESIAN_POINT('Ctrl Pts',(-45.1034416450612,53.3332894643605,-448.07438207641));
#35269=CARTESIAN_POINT('Ctrl Pts',(-45.1247823813031,53.3542727159754,-448.041878533347));
#35270=CARTESIAN_POINT('Ctrl Pts',(-45.1461224625502,53.3752562716634,-448.00937506903));
#35271=CARTESIAN_POINT('Ctrl Pts',(-45.1674619091309,53.3962401157622,-447.976871682436));
#35272=CARTESIAN_POINT('Ctrl Pts',(-45.9074843271741,54.1239307328129,-446.849699304724));
#35273=CARTESIAN_POINT('Ctrl Pts',(-46.6467436227848,54.8519680802525,-445.722620410717));
#35274=CARTESIAN_POINT('Ctrl Pts',(-47.3860866986765,55.5796997443964,-444.595592240322));
#35275=CARTESIAN_POINT('Ctrl Pts',(-47.3898186861473,55.583373120859,-444.589903331954));
#35276=CARTESIAN_POINT('Ctrl Pts',(-47.3935506757501,55.5870464895352,-444.584214424878));
#35277=CARTESIAN_POINT('Ctrl Pts',(-47.3972826675936,55.5907198503415,-444.578525519089));
#35278=CARTESIAN_POINT('Ctrl Pts',(-47.3978240010529,55.5912526792425,-444.577700331045));
#35279=CARTESIAN_POINT('Ctrl Pts',(-47.3983653345593,55.591785507978,-444.576875143028));
#35280=CARTESIAN_POINT('Ctrl Pts',(-47.3991053618007,55.5925139085243,-444.575747074044));
#35281=CARTESIAN_POINT('Ctrl Pts',(-47.3993040554946,55.5927094804788,-444.575444193054));
#35282=CARTESIAN_POINT('Ctrl Pts',(-48.1791318076515,56.3602850002595,-443.386704951096));
#35283=CARTESIAN_POINT('Ctrl Pts',(-48.9588592874826,57.127321149212,-442.198324735079));
#35284=CARTESIAN_POINT('Ctrl Pts',(-49.7406729832468,57.8967208089775,-441.006829369427));
#35285=CARTESIAN_POINT('Ctrl Pts',(-49.7428075253643,57.8988214600748,-441.003576296889));
#35286=CARTESIAN_POINT('Ctrl Pts',(-49.7919856016638,57.9472187693854,-440.928628220373));
#35287=CARTESIAN_POINT('Ctrl Pts',(-49.8390291362108,57.9935154256164,-440.856933215362));
#35288=CARTESIAN_POINT('Ctrl Pts',(-49.8860726707578,58.0398120818473,-440.785238210351));
#35289=CARTESIAN_POINT('Ctrl Pts',(-35.0926443215359,44.2999879125929,-462.499999999992));
#35290=CARTESIAN_POINT('Ctrl Pts',(-35.8831213977166,45.0683607770092,-461.304997290577));
#35291=CARTESIAN_POINT('Ctrl Pts',(-36.6779372668746,45.8333611204278,-460.111144802486));
#35292=CARTESIAN_POINT('Ctrl Pts',(-37.4647607936271,46.6039218500648,-458.915752656189));
#35293=CARTESIAN_POINT('Ctrl Pts',(-37.4978722442788,46.6363489225989,-458.865447642783));
#35294=CARTESIAN_POINT('Ctrl Pts',(-37.5309695427217,46.6687858409527,-458.815139903113));
#35295=CARTESIAN_POINT('Ctrl Pts',(-37.5640525540381,46.7012326745701,-458.764829422331));
#35296=CARTESIAN_POINT('Ctrl Pts',(-37.9447873803808,47.0746460692748,-458.185832789269));
#35297=CARTESIAN_POINT('Ctrl Pts',(-38.3236299052502,47.4493727209661,-457.606473101551));
#35298=CARTESIAN_POINT('Ctrl Pts',(-38.7003747687633,47.8255182783924,-457.026727780484));
#35299=CARTESIAN_POINT('Ctrl Pts',(-38.8864463470506,48.0112938637139,-456.740395736327));
#35300=CARTESIAN_POINT('Ctrl Pts',(-39.0720062509222,48.1974155570617,-456.45396962615));
#35301=CARTESIAN_POINT('Ctrl Pts',(-39.2570297926673,48.3838960499711,-456.167446739499));
#35302=CARTESIAN_POINT('Ctrl Pts',(-39.4375879783198,48.5658760247446,-455.887838792999));
#35303=CARTESIAN_POINT('Ctrl Pts',(-39.6176353785126,48.7481976895492,-455.608138684863));
#35304=CARTESIAN_POINT('Ctrl Pts',(-39.7971490861727,48.9308728145696,-455.328343902587));
#35305=CARTESIAN_POINT('Ctrl Pts',(-40.0283139559821,49.1661087307745,-454.968044261623));
#35306=CARTESIAN_POINT('Ctrl Pts',(-40.2585938557126,49.4019307544559,-454.607587632161));
#35307=CARTESIAN_POINT('Ctrl Pts',(-40.4883469303252,49.6380788163462,-454.24704592718));
#35308=CARTESIAN_POINT('Ctrl Pts',(-41.0215240749735,50.1860965069258,-453.410353764899));
#35309=CARTESIAN_POINT('Ctrl Pts',(-41.5518646697502,50.7358696024833,-452.573203559526));
#35310=CARTESIAN_POINT('Ctrl Pts',(-42.0838391397846,51.2841518182078,-451.736492952724));
#35311=CARTESIAN_POINT('Ctrl Pts',(-42.4038797716061,51.6140033366944,-451.233120316749));
#35312=CARTESIAN_POINT('Ctrl Pts',(-42.7242927631654,51.9435747828198,-450.729860947609));
#35313=CARTESIAN_POINT('Ctrl Pts',(-43.0448436596819,52.2730336439458,-450.226668796296));
#35314=CARTESIAN_POINT('Ctrl Pts',(-43.4848003122421,52.725216493136,-449.53603670981));
#35315=CARTESIAN_POINT('Ctrl Pts',(-43.9250167166423,53.1771872795364,-448.845531240238));
#35316=CARTESIAN_POINT('Ctrl Pts',(-44.3648877168719,53.6293782946376,-448.155033524324));
#35317=CARTESIAN_POINT('Ctrl Pts',(-44.3653119673901,53.6298144276682,-448.154367547222));
#35318=CARTESIAN_POINT('Ctrl Pts',(-44.3657362175869,53.6302505609037,-448.153701570128));
#35319=CARTESIAN_POINT('Ctrl Pts',(-44.3661604674627,53.6306866943438,-448.153035593041));
#35320=CARTESIAN_POINT('Ctrl Pts',(-44.3828103377971,53.6478029403118,-448.126899033492));
#35321=CARTESIAN_POINT('Ctrl Pts',(-44.3994597136609,53.6649195014566,-448.100762485096));
#35322=CARTESIAN_POINT('Ctrl Pts',(-44.4161086066083,53.6820363670388,-448.074625948665));
#35323=CARTESIAN_POINT('Ctrl Pts',(-44.4368140309913,53.7033237863947,-448.042121200129));
#35324=CARTESIAN_POINT('Ctrl Pts',(-44.4575187084622,53.7246116766146,-448.009616470102));
#35325=CARTESIAN_POINT('Ctrl Pts',(-44.478222661245,53.7459000170419,-447.977111760154));
#35326=CARTESIAN_POINT('Ctrl Pts',(-45.1962070355543,54.4841501445497,-446.849893490325));
#35327=CARTESIAN_POINT('Ctrl Pts',(-45.913320026553,55.2229415800519,-445.722699380136));
#35328=CARTESIAN_POINT('Ctrl Pts',(-46.6304875785502,55.9614136288578,-444.595594769643));
#35329=CARTESIAN_POINT('Ctrl Pts',(-46.6341076304664,55.9651412196388,-444.589905475428));
#35330=CARTESIAN_POINT('Ctrl Pts',(-46.6377276837699,55.9688688022845,-444.584216183493));
#35331=CARTESIAN_POINT('Ctrl Pts',(-46.6413477385799,55.9725963766842,-444.578526893846));
#35332=CARTESIAN_POINT('Ctrl Pts',(-46.6418728353313,55.9731370693837,-444.577701650123));
#35333=CARTESIAN_POINT('Ctrl Pts',(-46.6423979321143,55.9736777619098,-444.576876406447));
#35334=CARTESIAN_POINT('Ctrl Pts',(-46.6431157630056,55.9744169125997,-444.575748261405));
#35335=CARTESIAN_POINT('Ctrl Pts',(-46.6433084970863,55.974615370914,-444.575445359997));
#35336=CARTESIAN_POINT('Ctrl Pts',(-47.3997461093869,56.7535191945194,-443.386625991318));
#35337=CARTESIAN_POINT('Ctrl Pts',(-48.1560574503936,57.5318641226853,-442.19820951287));
#35338=CARTESIAN_POINT('Ctrl Pts',(-48.9144517868643,58.312341953673,-441.006848847162));
#35339=CARTESIAN_POINT('Ctrl Pts',(-48.916522388862,58.3144728489302,-441.003596143665));
#35340=CARTESIAN_POINT('Ctrl Pts',(-48.9642273482186,58.3635669135128,-440.928656599108));
#35341=CARTESIAN_POINT('Ctrl Pts',(-49.0098617054858,58.4105300828157,-440.856969755731));
#35342=CARTESIAN_POINT('Ctrl Pts',(-49.0554960627529,58.4574932521186,-440.785282912355));
#35343=CARTESIAN_POINT('Ctrl Pts',(-34.6937162549713,44.4837348679316,-462.499999999992));
#35344=CARTESIAN_POINT('Ctrl Pts',(-35.4568775601461,45.2647808331932,-461.305006320268));
#35345=CARTESIAN_POINT('Ctrl Pts',(-36.2238622232575,46.0429432083199,-460.110949296857));
#35346=CARTESIAN_POINT('Ctrl Pts',(-36.9837888169173,46.8260011505549,-458.91546450044));
#35347=CARTESIAN_POINT('Ctrl Pts',(-37.0157683791055,46.8589541362374,-458.865155588091));
#35348=CARTESIAN_POINT('Ctrl Pts',(-37.0477354434537,46.8919157905208,-458.814844147584));
#35349=CARTESIAN_POINT('Ctrl Pts',(-37.0796898950869,46.9248861637916,-458.76453016749));
#35350=CARTESIAN_POINT('Ctrl Pts',(-37.4474367267489,47.3043246986239,-458.185493262703));
#35351=CARTESIAN_POINT('Ctrl Pts',(-37.8135129358142,47.6849180817468,-457.60611997644));
#35352=CARTESIAN_POINT('Ctrl Pts',(-38.1777442157752,48.066742731875,-457.026393048804));
#35353=CARTESIAN_POINT('Ctrl Pts',(-38.3576354251521,48.2553231802341,-456.74007008903));
#35354=CARTESIAN_POINT('Ctrl Pts',(-38.5370766294755,48.4442039585018,-456.453660871109));
#35355=CARTESIAN_POINT('Ctrl Pts',(-38.7160468882022,48.633394236783,-456.167163326133));
#35356=CARTESIAN_POINT('Ctrl Pts',(-38.8906978807008,48.8180185989985,-455.887580109712));
#35357=CARTESIAN_POINT('Ctrl Pts',(-39.064900390378,49.0029377005569,-455.607912779175));
#35358=CARTESIAN_POINT('Ctrl Pts',(-39.2386348864512,49.1881600800444,-455.328159397521));
#35359=CARTESIAN_POINT('Ctrl Pts',(-39.4623577023278,49.4266761677469,-454.967913069305));
#35360=CARTESIAN_POINT('Ctrl Pts',(-39.6853044481674,49.6656951536519,-454.607524049405));
#35361=CARTESIAN_POINT('Ctrl Pts',(-39.9077944947688,49.9049821886886,-454.247056749965));
#35362=CARTESIAN_POINT('Ctrl Pts',(-40.4241166722174,50.4602843464826,-453.410537257122));
#35363=CARTESIAN_POINT('Ctrl Pts',(-40.9379795370076,51.0170297897597,-452.573596243841));
#35364=CARTESIAN_POINT('Ctrl Pts',(-41.4533752294989,51.5722849505129,-451.737038725624));
#35365=CARTESIAN_POINT('Ctrl Pts',(-41.7634419194518,51.9063314555231,-451.233758189122));
#35366=CARTESIAN_POINT('Ctrl Pts',(-42.0738280092103,52.240150054641,-450.730566128798));
#35367=CARTESIAN_POINT('Ctrl Pts',(-42.3843277118328,52.573887105166,-450.227421760993));
#35368=CARTESIAN_POINT('Ctrl Pts',(-42.8104890836191,53.031941776608,-449.536855257452));
#35369=CARTESIAN_POINT('Ctrl Pts',(-43.2368704944582,53.4898406553964,-448.846379690617));
#35370=CARTESIAN_POINT('Ctrl Pts',(-43.662949213368,53.9479584646017,-448.155891290016));
#35371=CARTESIAN_POINT('Ctrl Pts',(-43.6633601613895,53.9484003139571,-448.155225321899));
#35372=CARTESIAN_POINT('Ctrl Pts',(-43.6637711091287,53.9488421635163,-448.15455935377));
#35373=CARTESIAN_POINT('Ctrl Pts',(-43.664182056586,53.9492840132792,-448.153893385629));
#35374=CARTESIAN_POINT('Ctrl Pts',(-43.6803098677362,53.9666245988145,-448.127757177169));
#35375=CARTESIAN_POINT('Ctrl Pts',(-43.6964372445572,53.9839654980612,-448.101620950182));
#35376=CARTESIAN_POINT('Ctrl Pts',(-43.7125641962304,54.0013067017012,-448.07548470511));
#35377=CARTESIAN_POINT('Ctrl Pts',(-43.7326205074486,54.0228731194691,-448.04298031892));
#35378=CARTESIAN_POINT('Ctrl Pts',(-43.7526761611034,54.0444400080328,-448.010475904759));
#35379=CARTESIAN_POINT('Ctrl Pts',(-43.7727311748529,54.0660073494699,-447.977971463475));
#35380=CARTESIAN_POINT('Ctrl Pts',(-44.4682112433112,54.8139328451354,-446.85076251054));
#35381=CARTESIAN_POINT('Ctrl Pts',(-45.1629219292152,55.5624028563398,-445.723520968408));
#35382=CARTESIAN_POINT('Ctrl Pts',(-45.857598497673,56.3106707131351,-444.596282029048));
#35383=CARTESIAN_POINT('Ctrl Pts',(-45.8611050216865,56.314447750288,-444.59059205678));
#35384=CARTESIAN_POINT('Ctrl Pts',(-45.8646115448271,56.3182247822925,-444.584902084578));
#35385=CARTESIAN_POINT('Ctrl Pts',(-45.8681180671893,56.3220018090526,-444.579212112446));
#35386=CARTESIAN_POINT('Ctrl Pts',(-45.8686266958145,56.3225496749236,-444.578386769726));
#35387=CARTESIAN_POINT('Ctrl Pts',(-45.8691353244232,56.3230975406842,-444.577561427008));
#35388=CARTESIAN_POINT('Ctrl Pts',(-45.8698306425161,56.3238464975938,-444.576433146507));
#35389=CARTESIAN_POINT('Ctrl Pts',(-45.8700173320142,56.3240475888386,-444.576130208722));
#35390=CARTESIAN_POINT('Ctrl Pts',(-46.6027313019823,57.1132851013013,-443.387168045725));
#35391=CARTESIAN_POINT('Ctrl Pts',(-47.3352250969972,57.9020921615662,-442.198511933312));
#35392=CARTESIAN_POINT('Ctrl Pts',(-48.0699634411771,58.6930115612169,-441.006849591051));
#35393=CARTESIAN_POINT('Ctrl Pts',(-48.0719694582289,58.695170964141,-441.003596063446));
#35394=CARTESIAN_POINT('Ctrl Pts',(-48.1181864730666,58.7449218132285,-440.928637521526));
#35395=CARTESIAN_POINT('Ctrl Pts',(-48.1623974690588,58.792513259741,-440.856932505353));
#35396=CARTESIAN_POINT('Ctrl Pts',(-48.2066084650511,58.8401047062535,-440.785227489179));
#35397=CARTESIAN_POINT('Ctrl Pts',(-34.2872595209354,44.6497527723323,-462.499999999992));
#35398=CARTESIAN_POINT('Ctrl Pts',(-35.0224304000914,45.4421310218592,-461.305151339373));
#35399=CARTESIAN_POINT('Ctrl Pts',(-35.7607385756046,46.2323164757708,-460.110931894838));
#35400=CARTESIAN_POINT('Ctrl Pts',(-36.4931193505426,47.0266864032259,-458.915400919906));
#35401=CARTESIAN_POINT('Ctrl Pts',(-36.5239397175793,47.0601154248016,-458.865090064252));
#35402=CARTESIAN_POINT('Ctrl Pts',(-36.5547495888943,47.0935518558537,-458.814776886249));
#35403=CARTESIAN_POINT('Ctrl Pts',(-36.5855488679042,47.1269957313529,-458.764461378322));
#35404=CARTESIAN_POINT('Ctrl Pts',(-36.9400014306773,47.5118835521334,-458.185406890509));
#35405=CARTESIAN_POINT('Ctrl Pts',(-37.2930508462519,47.8977574574093,-457.606043765974));
#35406=CARTESIAN_POINT('Ctrl Pts',(-37.6445513595258,48.2846701266294,-457.026360754561));
#35407=CARTESIAN_POINT('Ctrl Pts',(-37.8181549348041,48.4757635110216,-456.740059484693));
#35408=CARTESIAN_POINT('Ctrl Pts',(-37.9913807419683,48.6671102582059,-456.45368019583));
#35409=CARTESIAN_POINT('Ctrl Pts',(-38.1642112882018,48.8587166783817,-456.1672215441));
#35410=CARTESIAN_POINT('Ctrl Pts',(-38.3328707439603,49.0456988713503,-455.887676282276));
#35411=CARTESIAN_POINT('Ctrl Pts',(-38.5011537998596,49.2329283499863,-455.608055444416));
#35412=CARTESIAN_POINT('Ctrl Pts',(-38.6690439880478,49.4204110496045,-455.328357739766));
#35413=CARTESIAN_POINT('Ctrl Pts',(-38.8852409236505,49.6618378153579,-454.968183108402));
#35414=CARTESIAN_POINT('Ctrl Pts',(-39.1007863839428,49.9036844796046,-454.607881012199));
#35415=CARTESIAN_POINT('Ctrl Pts',(-39.3159450882721,50.1457533784629,-454.247505626363));
#35416=CARTESIAN_POINT('Ctrl Pts',(-39.8152537648325,50.7075112766714,-453.411199433092));
#35417=CARTESIAN_POINT('Ctrl Pts',(-40.3124792433739,51.2704659645045,-452.574498490218));
#35418=CARTESIAN_POINT('Ctrl Pts',(-40.8109390344613,51.8321453062596,-451.738081361453));
#35419=CARTESIAN_POINT('Ctrl Pts',(-41.1108169336148,52.1700566564129,-451.234885284506));
#35420=CARTESIAN_POINT('Ctrl Pts',(-41.410962076571,52.5077819260265,-450.731753539923));
#35421=CARTESIAN_POINT('Ctrl Pts',(-41.711203404823,52.8454452232713,-450.228650126377));
#35422=CARTESIAN_POINT('Ctrl Pts',(-42.1232851402775,53.3088886750373,-449.538139832627));
#35423=CARTESIAN_POINT('Ctrl Pts',(-42.5355621332702,53.7722102900826,-448.84768546806));
#35424=CARTESIAN_POINT('Ctrl Pts',(-42.9476124941153,54.2357233582771,-448.157197595481));
#35425=CARTESIAN_POINT('Ctrl Pts',(-42.9480099119469,54.2361704112977,-448.156531627873));
#35426=CARTESIAN_POINT('Ctrl Pts',(-42.948407329566,54.2366174644969,-448.155865660234));
#35427=CARTESIAN_POINT('Ctrl Pts',(-42.9488047469729,54.2370645178746,-448.155199692564));
#35428=CARTESIAN_POINT('Ctrl Pts',(-42.9644015654331,54.2546093215285,-448.129063502567));
#35429=CARTESIAN_POINT('Ctrl Pts',(-42.9799980571234,54.2721544000718,-448.102927264174));
#35430=CARTESIAN_POINT('Ctrl Pts',(-42.9955942275873,54.2896997469008,-448.076790977015));
#35431=CARTESIAN_POINT('Ctrl Pts',(-43.0149904318407,54.3115200476971,-448.044286538483));
#35432=CARTESIAN_POINT('Ctrl Pts',(-43.0343861392631,54.3333407634428,-448.011782024527));
#35433=CARTESIAN_POINT('Ctrl Pts',(-43.0537813605145,54.3551618814368,-447.979277434437));
#35434=CARTESIAN_POINT('Ctrl Pts',(-43.7263807400131,55.1118879962072,-446.852063321111));
#35435=CARTESIAN_POINT('Ctrl Pts',(-44.3983956724348,55.8690977462486,-445.724757698917));
#35436=CARTESIAN_POINT('Ctrl Pts',(-45.0702692045423,56.6262622154341,-444.597330620593));
#35437=CARTESIAN_POINT('Ctrl Pts',(-45.0736606255018,56.6300841600827,-444.591639698654));
#35438=CARTESIAN_POINT('Ctrl Pts',(-45.0770520428539,56.6339061035798,-444.58594877362));
#35439=CARTESIAN_POINT('Ctrl Pts',(-45.0804434566555,56.6377280458573,-444.580257845486));
#35440=CARTESIAN_POINT('Ctrl Pts',(-45.0809353885358,56.638282426821,-444.579432364097));
#35441=CARTESIAN_POINT('Ctrl Pts',(-45.0814273203415,56.6388368077588,-444.578606882642));
#35442=CARTESIAN_POINT('Ctrl Pts',(-45.0820998130759,56.6395946713239,-444.57747841239));
#35443=CARTESIAN_POINT('Ctrl Pts',(-45.0822803740693,56.6397981539734,-444.577175423649));
#35444=CARTESIAN_POINT('Ctrl Pts',(-45.7909413206515,57.4384214330053,-443.388013234218));
#35445=CARTESIAN_POINT('Ctrl Pts',(-46.4992668825881,58.2367877057615,-442.199018696807));
#35446=CARTESIAN_POINT('Ctrl Pts',(-47.2100390429521,59.0373060430022,-441.006896336889));
#35447=CARTESIAN_POINT('Ctrl Pts',(-47.2119796284694,59.0394916534735,-441.003641552419));
#35448=CARTESIAN_POINT('Ctrl Pts',(-47.2566892012544,59.0898463050323,-440.928654032679));
#35449=CARTESIAN_POINT('Ctrl Pts',(-47.2994581847153,59.1380153463707,-440.856921296449));
#35450=CARTESIAN_POINT('Ctrl Pts',(-47.3422271681762,59.1861843877091,-440.785188560218));
#35451=CARTESIAN_POINT('Ctrl Pts',(-34.2870189837742,44.6498510128264,-462.499999999991));
#35452=CARTESIAN_POINT('Ctrl Pts',(-35.022173298412,45.4422359681457,-461.30515142524));
#35453=CARTESIAN_POINT('Ctrl Pts',(-35.7604645033475,46.2324285367216,-460.110931884602));
#35454=CARTESIAN_POINT('Ctrl Pts',(-36.4928289768881,47.0268051580112,-458.915400882359));
#35455=CARTESIAN_POINT('Ctrl Pts',(-36.5236486579223,47.0602344612798,-458.865090025556));
#35456=CARTESIAN_POINT('Ctrl Pts',(-36.5544578444197,47.0936711732796,-458.814776846525));
#35457=CARTESIAN_POINT('Ctrl Pts',(-36.5852564398078,47.1271153289722,-458.764461337694));
#35458=CARTESIAN_POINT('Ctrl Pts',(-36.9397011351403,47.5120063743502,-458.185406839484));
#35459=CARTESIAN_POINT('Ctrl Pts',(-37.2927428415779,47.8978834043482,-457.606043720971));
#35460=CARTESIAN_POINT('Ctrl Pts',(-37.6442358209138,48.2847990843685,-457.026360735556));
#35461=CARTESIAN_POINT('Ctrl Pts',(-37.8178356752343,48.4758939557733,-456.740059478528));
#35462=CARTESIAN_POINT('Ctrl Pts',(-37.9910578041932,48.6672421621754,-456.453680207381));
#35463=CARTESIAN_POINT('Ctrl Pts',(-38.1638847170138,48.858850012082,-456.167221578672));
#35464=CARTESIAN_POINT('Ctrl Pts',(-38.3325406270483,49.0458336002762,-455.887676339314));
#35465=CARTESIAN_POINT('Ctrl Pts',(-38.5008201798844,49.2330644460553,-455.608055528972));
#35466=CARTESIAN_POINT('Ctrl Pts',(-38.6687069094829,49.4205484831939,-455.328357857276));
#35467=CARTESIAN_POINT('Ctrl Pts',(-38.884899391362,49.66197697131,-454.968183268347));
#35468=CARTESIAN_POINT('Ctrl Pts',(-39.1004404716694,49.9038253088016,-454.607881223591));
#35469=CARTESIAN_POINT('Ctrl Pts',(-39.3155948374051,50.1458958537967,-454.247505892154));
#35470=CARTESIAN_POINT('Ctrl Pts',(-39.8148934455952,50.7076575721175,-453.411199825125));
#35471=CARTESIAN_POINT('Ctrl Pts',(-40.3121090783446,51.2706159342137,-452.574499024332));
#35472=CARTESIAN_POINT('Ctrl Pts',(-40.8105588469142,51.8322990775026,-451.738081978642));
#35473=CARTESIAN_POINT('Ctrl Pts',(-41.1104307164308,52.170212714693,-451.234885951675));
#35474=CARTESIAN_POINT('Ctrl Pts',(-41.4105697988818,52.5079402960933,-450.731754242783));
#35475=CARTESIAN_POINT('Ctrl Pts',(-41.7108050563151,52.8456059167068,-450.22865085347));
#35476=CARTESIAN_POINT('Ctrl Pts',(-42.1228784595606,53.3090525573004,-449.538140592981));
#35477=CARTESIAN_POINT('Ctrl Pts',(-42.5351471056795,53.7723773812622,-448.847686240956));
#35478=CARTESIAN_POINT('Ctrl Pts',(-42.9471891646714,54.2358936421045,-448.157198368687));
#35479=CARTESIAN_POINT('Ctrl Pts',(-42.9475865744959,54.2363406982042,-448.15653240108));
#35480=CARTESIAN_POINT('Ctrl Pts',(-42.947983984108,54.2367877544828,-448.155866433441));
#35481=CARTESIAN_POINT('Ctrl Pts',(-42.948381393508,54.2372348109397,-448.155200465771));
#35482=CARTESIAN_POINT('Ctrl Pts',(-42.9639778977315,54.2547797354398,-448.129064275785));
#35483=CARTESIAN_POINT('Ctrl Pts',(-42.9795740752489,54.2723249348063,-448.102928037385));
#35484=CARTESIAN_POINT('Ctrl Pts',(-42.9951699316014,54.2898704024371,-448.076791750201));
#35485=CARTESIAN_POINT('Ctrl Pts',(-43.0145657452096,54.3116908534688,-448.044287311638));
#35486=CARTESIAN_POINT('Ctrl Pts',(-43.033961062082,54.3335117194169,-448.011782797623));
#35487=CARTESIAN_POINT('Ctrl Pts',(-43.0533558928743,54.3553329875833,-447.979278207444));
#35488=CARTESIAN_POINT('Ctrl Pts',(-43.725941731794,55.1120643101229,-446.852064091059));
#35489=CARTESIAN_POINT('Ctrl Pts',(-44.3979432331023,55.8692792318855,-445.724758430936));
#35490=CARTESIAN_POINT('Ctrl Pts',(-45.0698032706076,56.6264489656385,-444.597331241255));
#35491=CARTESIAN_POINT('Ctrl Pts',(-45.0731946234504,56.6302709368613,-444.591640318754));
#35492=CARTESIAN_POINT('Ctrl Pts',(-45.076585972684,56.6340929069347,-444.585949393156));
#35493=CARTESIAN_POINT('Ctrl Pts',(-45.0799773183656,56.6379148757911,-444.580258464457));
#35494=CARTESIAN_POINT('Ctrl Pts',(-45.0804692403649,56.63846926061,-444.579432982985));
#35495=CARTESIAN_POINT('Ctrl Pts',(-45.0809611622896,56.6390236454031,-444.578607501448));
#35496=CARTESIAN_POINT('Ctrl Pts',(-45.0816336415163,56.6397815142388,-444.577479031083));
#35497=CARTESIAN_POINT('Ctrl Pts',(-45.0818141988828,56.6399849983033,-444.577176042312));
#35498=CARTESIAN_POINT('Ctrl Pts',(-45.7904609111333,57.43861383136,-443.388013734489));
#35499=CARTESIAN_POINT('Ctrl Pts',(-46.498772170558,58.2369857607961,-442.199018996768));
#35500=CARTESIAN_POINT('Ctrl Pts',(-47.2095301480132,59.0375097782374,-441.006896364563));
#35501=CARTESIAN_POINT('Ctrl Pts',(-47.2114706948088,59.0396954042171,-441.003641579351));
#35502=CARTESIAN_POINT('Ctrl Pts',(-47.2561793755078,59.0900504130787,-440.928654042424));
#35503=CARTESIAN_POINT('Ctrl Pts',(-47.2989475056031,59.1382197962114,-440.856921289753));
#35504=CARTESIAN_POINT('Ctrl Pts',(-47.3417156356984,59.1863891793441,-440.785188537082));
#35505=CARTESIAN_POINT('Ctrl Pts',(-33.882499227078,44.8150532196688,-462.499999999992));
#35506=CARTESIAN_POINT('Ctrl Pts',(-34.5897963205529,45.6187146263589,-461.305295910369));
#35507=CARTESIAN_POINT('Ctrl Pts',(-35.2995473263181,46.4208713719593,-460.11091477585));
#35508=CARTESIAN_POINT('Ctrl Pts',(-36.004497088199,47.2265044265567,-458.915337870982));
#35509=CARTESIAN_POINT('Ctrl Pts',(-36.0341630913862,47.2604074279587,-458.865025082485));
#35510=CARTESIAN_POINT('Ctrl Pts',(-36.06382059298,47.2943165848991,-458.814710176593));
#35511=CARTESIAN_POINT('Ctrl Pts',(-36.0934695146101,47.3282319170015,-458.764393149568));
#35512=CARTESIAN_POINT('Ctrl Pts',(-36.4346832245758,47.7185454817157,-458.185321179272));
#35513=CARTESIAN_POINT('Ctrl Pts',(-36.7747601945371,48.109677063011,-457.605968201868));
#35514=CARTESIAN_POINT('Ctrl Pts',(-37.1135830980392,48.5016557071232,-457.026328952538));
#35515=CARTESIAN_POINT('Ctrl Pts',(-37.2809252930373,48.6952511400767,-456.740049296448));
#35516=CARTESIAN_POINT('Ctrl Pts',(-37.4479616662434,48.8890531643603,-456.453699826454));
#35517=CARTESIAN_POINT('Ctrl Pts',(-37.6146781577475,49.0830652430437,-456.167279920779));
#35518=CARTESIAN_POINT('Ctrl Pts',(-37.7773711153053,49.2723950363843,-455.887772469913));
#35519=CARTESIAN_POINT('Ctrl Pts',(-37.9397594650648,49.4619248602184,-455.608197945846));
#35520=CARTESIAN_POINT('Ctrl Pts',(-38.1018297888824,49.6516580582508,-455.328555701444));
#35521=CARTESIAN_POINT('Ctrl Pts',(-38.3105323208151,49.8959828543535,-454.968452487807));
#35522=CARTESIAN_POINT('Ctrl Pts',(-38.5187074679136,50.140644897714,-454.608236973389));
#35523=CARTESIAN_POINT('Ctrl Pts',(-38.7265655086456,50.3854835677273,-454.247953136177));
#35524=CARTESIAN_POINT('Ctrl Pts',(-39.2089318788736,50.9536691434688,-453.411859395487));
#35525=CARTESIAN_POINT('Ctrl Pts',(-39.6895895863211,51.5228061244817,-452.575397552201));
#35526=CARTESIAN_POINT('Ctrl Pts',(-40.1711841106882,52.0908820466578,-451.739120208895));
#35527=CARTESIAN_POINT('Ctrl Pts',(-40.4609157135043,52.4326416371961,-451.23600822814));
#35528=CARTESIAN_POINT('Ctrl Pts',(-40.7508626122354,52.7742567903562,-450.732936537627));
#35529=CARTESIAN_POINT('Ctrl Pts',(-41.0408883415266,53.1158294556676,-450.229873897835));
#35530=CARTESIAN_POINT('Ctrl Pts',(-41.4389491499721,53.5846385217771,-449.539419566132));
#35531=CARTESIAN_POINT('Ctrl Pts',(-41.8371805402333,54.0533595457502,-448.848986303267));
#35532=CARTESIAN_POINT('Ctrl Pts',(-42.2352610710188,54.5222446334621,-448.158498944552));
#35533=CARTESIAN_POINT('Ctrl Pts',(-42.23564501511,54.5226968677337,-448.15783297744));
#35534=CARTESIAN_POINT('Ctrl Pts',(-42.2360289590583,54.5231491021588,-448.157167010277));
#35535=CARTESIAN_POINT('Ctrl Pts',(-42.236412902864,54.5236013367372,-448.156501043064));
#35536=CARTESIAN_POINT('Ctrl Pts',(-42.251480944002,54.541349478861,-448.130364871002));
#35537=CARTESIAN_POINT('Ctrl Pts',(-42.2665487655235,54.5590978571757,-448.104228620798));
#35538=CARTESIAN_POINT('Ctrl Pts',(-42.2816163693486,54.5768464677822,-448.078092291274));
#35539=CARTESIAN_POINT('Ctrl Pts',(-42.3003552207916,54.5989195579256,-448.045587800056));
#35540=CARTESIAN_POINT('Ctrl Pts',(-42.3190937355299,54.6209930073476,-448.013083186158));
#35541=CARTESIAN_POINT('Ctrl Pts',(-42.3378319172539,54.6430668085493,-447.980578447317));
#35542=CARTESIAN_POINT('Ctrl Pts',(-42.9876460769867,55.40855562659,-446.853359175542));
#35543=CARTESIAN_POINT('Ctrl Pts',(-43.6370600294435,56.1744673877555,-445.72598971932));
#35544=CARTESIAN_POINT('Ctrl Pts',(-44.2862257462271,56.9404901210901,-444.598375225355));
#35545=CARTESIAN_POINT('Ctrl Pts',(-44.2895025447805,56.9443567796637,-444.592683357397));
#35546=CARTESIAN_POINT('Ctrl Pts',(-44.2927793370035,56.9482234410669,-444.586991483194));
#35547=CARTESIAN_POINT('Ctrl Pts',(-44.2960561229152,56.9520901052595,-444.581299602734));
#35548=CARTESIAN_POINT('Ctrl Pts',(-44.2965314277732,56.9526509732333,-444.580473983208));
#35549=CARTESIAN_POINT('Ctrl Pts',(-44.2970067324983,56.9532118412657,-444.579648363549));
#35550=CARTESIAN_POINT('Ctrl Pts',(-44.2976564951886,56.9539785730952,-444.578519704276));
#35551=CARTESIAN_POINT('Ctrl Pts',(-44.2978309532686,56.9541844368416,-444.578216664775));
#35552=CARTESIAN_POINT('Ctrl Pts',(-44.9825393171837,57.7621530264513,-443.388855217941));
#35553=CARTESIAN_POINT('Ctrl Pts',(-45.6667975667759,58.5700373708246,-442.199523556902));
#35554=CARTESIAN_POINT('Ctrl Pts',(-46.3537037290544,59.3801133786364,-441.006942922665));
#35555=CARTESIAN_POINT('Ctrl Pts',(-46.3555791565611,59.3823250839859,-441.003686886098));
#35556=CARTESIAN_POINT('Ctrl Pts',(-46.3987875888851,59.4332809422084,-440.928670498321));
#35557=CARTESIAN_POINT('Ctrl Pts',(-46.4401205878902,59.4820250952344,-440.856910147053));
#35558=CARTESIAN_POINT('Ctrl Pts',(-46.4814535868953,59.5307692482604,-440.785149795784));
#35559=CARTESIAN_POINT('Ctrl Pts',(-33.4710017122312,44.9624982997247,-462.499999999992));
#35560=CARTESIAN_POINT('Ctrl Pts',(-34.1498065842261,45.7760949547167,-461.305574764512));
#35561=CARTESIAN_POINT('Ctrl Pts',(-34.8302145362503,46.5890736375712,-460.111073961072));
#35562=CARTESIAN_POINT('Ctrl Pts',(-35.5071397368667,47.4047760112341,-458.915497269838));
#35563=CARTESIAN_POINT('Ctrl Pts',(-35.5356263982502,47.4391027541106,-458.865184490332));
#35564=CARTESIAN_POINT('Ctrl Pts',(-35.5641068927283,47.4734343199053,-458.814869805673));
#35565=CARTESIAN_POINT('Ctrl Pts',(-35.5925811583742,47.5077707165236,-458.764553216379));
#35566=CARTESIAN_POINT('Ctrl Pts',(-35.9202763757838,47.9029300893719,-458.185486283692));
#35567=CARTESIAN_POINT('Ctrl Pts',(-36.2471461026656,48.2987294808301,-457.606166988185));
#35568=CARTESIAN_POINT('Ctrl Pts',(-36.5730989065517,48.6951797757475,-457.026596718414));
#35569=CARTESIAN_POINT('Ctrl Pts',(-36.7340846519198,48.8909837248705,-456.740351130832));
#35570=CARTESIAN_POINT('Ctrl Pts',(-36.8948468485331,49.0869464039666,-456.454044346223));
#35571=CARTESIAN_POINT('Ctrl Pts',(-37.0553745659741,49.2830690882183,-456.167676545631));
#35572=CARTESIAN_POINT('Ctrl Pts',(-37.2120281092728,49.4744585497958,-455.888219942345));
#35573=CARTESIAN_POINT('Ctrl Pts',(-37.3684583839647,49.6660003759221,-455.608705238052));
#35574=CARTESIAN_POINT('Ctrl Pts',(-37.5246547051888,49.857695944655,-455.329132497536));
#35575=CARTESIAN_POINT('Ctrl Pts',(-37.7257931181328,50.1045477409151,-454.969118786015));
#35576=CARTESIAN_POINT('Ctrl Pts',(-37.9265435396957,50.3516544917298,-454.609008828603));
#35577=CARTESIAN_POINT('Ctrl Pts',(-38.1270461953369,50.5989043899216,-454.248833716317));
#35578=CARTESIAN_POINT('Ctrl Pts',(-38.5923432696388,51.1726855893882,-453.412992288444));
#35579=CARTESIAN_POINT('Ctrl Pts',(-39.0563044147987,51.7472381853159,-452.57679969215));
#35580=CARTESIAN_POINT('Ctrl Pts',(-39.5207100112726,52.3211556802638,-451.740649315997));
#35581=CARTESIAN_POINT('Ctrl Pts',(-39.8001006002745,52.6664296135875,-451.237613719826));
#35582=CARTESIAN_POINT('Ctrl Pts',(-40.0796597373392,53.0115890944338,-450.734595265531));
#35583=CARTESIAN_POINT('Ctrl Pts',(-40.3592902725819,53.356713226554,-450.231566929635));
#35584=CARTESIAN_POINT('Ctrl Pts',(-40.7430836594543,53.8303966869201,-449.541159680087));
#35585=CARTESIAN_POINT('Ctrl Pts',(-41.1270436081776,54.3040019309654,-448.85073965213));
#35586=CARTESIAN_POINT('Ctrl Pts',(-41.5109640329818,54.7777171498825,-448.16024502308));
#35587=CARTESIAN_POINT('Ctrl Pts',(-41.5113343198136,54.7781740427599,-448.159579048956));
#35588=CARTESIAN_POINT('Ctrl Pts',(-41.5117046066051,54.7786309357411,-448.158913074762));
#35589=CARTESIAN_POINT('Ctrl Pts',(-41.5120748933564,54.7790878288258,-448.158247100498));
#35590=CARTESIAN_POINT('Ctrl Pts',(-41.5266069574702,54.7970187960456,-448.132110651728));
#35591=CARTESIAN_POINT('Ctrl Pts',(-41.5411389597152,54.8149499226548,-448.10597409512));
#35592=CARTESIAN_POINT('Ctrl Pts',(-41.5556708969731,54.8328812087858,-448.079837428255));
#35593=CARTESIAN_POINT('Ctrl Pts',(-41.5737435657675,54.8551814836599,-448.0473325175));
#35594=CARTESIAN_POINT('Ctrl Pts',(-41.5918161340486,54.8774820052618,-448.014827436212));
#35595=CARTESIAN_POINT('Ctrl Pts',(-41.609888595815,54.8997827738486,-447.982322179732));
#35596=CARTESIAN_POINT('Ctrl Pts',(-42.2366165105127,55.6731425060908,-446.85508495696));
#35597=CARTESIAN_POINT('Ctrl Pts',(-42.8632166744256,56.446799156781,-445.727637147225));
#35598=CARTESIAN_POINT('Ctrl Pts',(-43.4894364238166,57.2207642094785,-444.599783822231));
#35599=CARTESIAN_POINT('Ctrl Pts',(-43.492597397842,57.2246709585559,-444.594090748724));
#35600=CARTESIAN_POINT('Ctrl Pts',(-43.4957583621677,57.228577715493,-444.588397664883));
#35601=CARTESIAN_POINT('Ctrl Pts',(-43.4989193167611,57.2324844802916,-444.582704570682));
#35602=CARTESIAN_POINT('Ctrl Pts',(-43.4993778200367,57.2330511649446,-444.5818787751));
#35603=CARTESIAN_POINT('Ctrl Pts',(-43.4998363231075,57.233617849763,-444.581052979299));
#35604=CARTESIAN_POINT('Ctrl Pts',(-43.5004631170844,57.2343925335459,-444.579924079114));
#35605=CARTESIAN_POINT('Ctrl Pts',(-43.5006314081677,57.2346005323672,-444.579620974917));
#35606=CARTESIAN_POINT('Ctrl Pts',(-44.1611356691744,58.0509488636593,-443.390005567788));
#35607=CARTESIAN_POINT('Ctrl Pts',(-44.821046186353,58.8674324443465,-442.200240815627));
#35608=CARTESIAN_POINT('Ctrl Pts',(-45.4838216333574,59.686214391916,-441.007046063224));
#35609=CARTESIAN_POINT('Ctrl Pts',(-45.4856311802341,59.6884498672306,-441.00378834862));
#35610=CARTESIAN_POINT('Ctrl Pts',(-45.5273218264009,59.7399533800503,-440.928733269294));
#35611=CARTESIAN_POINT('Ctrl Pts',(-45.5672029177492,59.7892214170893,-440.856935905857));
#35612=CARTESIAN_POINT('Ctrl Pts',(-45.6070840090976,59.8384894541283,-440.78513854242));
#35613=CARTESIAN_POINT('Ctrl Pts',(-33.0533836161765,45.091854154172,-462.499999999992));
#35614=CARTESIAN_POINT('Ctrl Pts',(-33.7034151132609,45.9143089978342,-461.305736187933));
#35615=CARTESIAN_POINT('Ctrl Pts',(-34.3544003661019,46.7366884856134,-460.111197234966));
#35616=CARTESIAN_POINT('Ctrl Pts',(-35.0030466122211,47.5611021033272,-458.915728574456));
#35617=CARTESIAN_POINT('Ctrl Pts',(-35.0303432263138,47.5957954365733,-458.865420341145));
#35618=CARTESIAN_POINT('Ctrl Pts',(-35.0576356987778,47.6304923717441,-458.81511046151));
#35619=CARTESIAN_POINT('Ctrl Pts',(-35.0849239853749,47.6651929130949,-458.764798934386));
#35620=CARTESIAN_POINT('Ctrl Pts',(-35.3989703990889,48.0645430344869,-458.185790259525));
#35621=CARTESIAN_POINT('Ctrl Pts',(-35.7124617861774,48.464371018814,-457.606563255973));
#35622=CARTESIAN_POINT('Ctrl Pts',(-36.0253343395421,48.8646819472439,-457.027116886978));
#35623=CARTESIAN_POINT('Ctrl Pts',(-36.1798598432595,49.0623926354905,-456.740932493099));
#35624=CARTESIAN_POINT('Ctrl Pts',(-36.3342345379915,49.26022107364,-456.454694617896));
#35625=CARTESIAN_POINT('Ctrl Pts',(-36.4884508294031,49.4581678377631,-456.168403151226));
#35626=CARTESIAN_POINT('Ctrl Pts',(-36.638945266558,49.6513373568889,-455.88902103962));
#35627=CARTESIAN_POINT('Ctrl Pts',(-36.7892888905276,49.8446195462205,-455.609587898822));
#35628=CARTESIAN_POINT('Ctrl Pts',(-36.9394739770257,50.0380151880987,-455.330103495726));
#35629=CARTESIAN_POINT('Ctrl Pts',(-37.1328715532901,50.2870562165485,-454.970203538794));
#35630=CARTESIAN_POINT('Ctrl Pts',(-37.3260061809514,50.5362853956562,-454.610218565813));
#35631=CARTESIAN_POINT('Ctrl Pts',(-37.5189638217216,50.785631966803,-454.250167529876));
#35632=CARTESIAN_POINT('Ctrl Pts',(-37.9667515351936,51.3642788164959,-453.414614040146));
#35633=CARTESIAN_POINT('Ctrl Pts',(-38.4135839406132,51.943558591785,-452.57870439064));
#35634=CARTESIAN_POINT('Ctrl Pts',(-38.8605715509455,52.5225745434955,-451.742681745474));
#35635=CARTESIAN_POINT('Ctrl Pts',(-39.1294833226286,52.8709157543212,-451.239722993414));
#35636=CARTESIAN_POINT('Ctrl Pts',(-39.3985305366766,53.2191901195012,-450.736738959138));
#35637=CARTESIAN_POINT('Ctrl Pts',(-39.6676464559522,53.5674526320097,-450.233712353502));
#35638=CARTESIAN_POINT('Ctrl Pts',(-40.0370085144638,54.0454435248148,-449.54330747874));
#35639=CARTESIAN_POINT('Ctrl Pts',(-40.4065400300739,54.5233975701954,-448.852829696241));
#35640=CARTESIAN_POINT('Ctrl Pts',(-40.7761244907476,55.0014367516422,-448.162244300311));
#35641=CARTESIAN_POINT('Ctrl Pts',(-40.7764809507071,55.0018978149318,-448.161578238643));
#35642=CARTESIAN_POINT('Ctrl Pts',(-40.7768374107112,55.0023588783023,-448.160912176875));
#35643=CARTESIAN_POINT('Ctrl Pts',(-40.7771938707602,55.0028199417536,-448.160246115005));
#35644=CARTESIAN_POINT('Ctrl Pts',(-40.7911832999486,55.020914576818,-448.134106228125));
#35645=CARTESIAN_POINT('Ctrl Pts',(-40.8051727983377,55.0390093362169,-448.10796618588));
#35646=CARTESIAN_POINT('Ctrl Pts',(-40.8191623586508,55.057104222479,-448.081825985748));
#35647=CARTESIAN_POINT('Ctrl Pts',(-40.8365604994238,55.0796079589375,-448.049316680841));
#35648=CARTESIAN_POINT('Ctrl Pts',(-40.8539587359728,55.1021118916113,-448.016807131734));
#35649=CARTESIAN_POINT('Ctrl Pts',(-40.8713570542966,55.1246160253655,-447.984297333575));
#35650=CARTESIAN_POINT('Ctrl Pts',(-41.4747066091777,55.9050281796226,-446.856902611653));
#35651=CARTESIAN_POINT('Ctrl Pts',(-42.0781549044513,56.6856820489916,-445.729208498906));
#35652=CARTESIAN_POINT('Ctrl Pts',(-42.681115280234,57.4667812939235,-444.601011806645));
#35653=CARTESIAN_POINT('Ctrl Pts',(-42.6841588477485,57.4707240543153,-444.59531699992));
#35654=CARTESIAN_POINT('Ctrl Pts',(-42.6872024028231,57.4746668260569,-444.589622180388));
#35655=CARTESIAN_POINT('Ctrl Pts',(-42.6902459453823,57.4786096091744,-444.583927348021));
#35656=CARTESIAN_POINT('Ctrl Pts',(-42.6906874177893,57.4791815183622,-444.583101300314));
#35657=CARTESIAN_POINT('Ctrl Pts',(-42.6911288899329,57.4797534277893,-444.582275252337));
#35658=CARTESIAN_POINT('Ctrl Pts',(-42.6917324017885,57.4805352539479,-444.581146007343));
#35659=CARTESIAN_POINT('Ctrl Pts',(-42.6918944417284,57.480745170472,-444.580842810561));
#35660=CARTESIAN_POINT('Ctrl Pts',(-43.3278643503816,58.3046200899417,-443.390863995632));
#35661=CARTESIAN_POINT('Ctrl Pts',(-43.9631249009979,59.1287818793436,-442.200627878454));
#35662=CARTESIAN_POINT('Ctrl Pts',(-44.6013941965172,59.9552283282957,-441.006936223393));
#35663=CARTESIAN_POINT('Ctrl Pts',(-44.6031368371902,59.957484729313,-441.003677151942));
#35664=CARTESIAN_POINT('Ctrl Pts',(-44.6432860563195,60.0094703469446,-440.928590807858));
#35665=CARTESIAN_POINT('Ctrl Pts',(-44.6816926252475,60.0591995633562,-440.85676353669));
#35666=CARTESIAN_POINT('Ctrl Pts',(-44.7200991941757,60.1089287797678,-440.784936265522));
#35667=CARTESIAN_POINT('Ctrl Pts',(-33.0529806979711,45.0919789381448,-462.499999999992));
#35668=CARTESIAN_POINT('Ctrl Pts',(-33.7029844346161,45.9144423270676,-461.305736343562));
#35669=CARTESIAN_POINT('Ctrl Pts',(-34.3539413007462,46.7368308832956,-460.111197353865));
#35670=CARTESIAN_POINT('Ctrl Pts',(-35.0025602634613,47.5612529042377,-458.915728797683));
#35671=CARTESIAN_POINT('Ctrl Pts',(-35.029855729402,47.5959465911122,-458.865420568762));
#35672=CARTESIAN_POINT('Ctrl Pts',(-35.0571470556675,47.6306438787335,-458.815110693767));
#35673=CARTESIAN_POINT('Ctrl Pts',(-35.0844341980371,47.6653447713533,-458.764799171531));
#35674=CARTESIAN_POINT('Ctrl Pts',(-35.3984674434415,48.0646989353141,-458.185790552926));
#35675=CARTESIAN_POINT('Ctrl Pts',(-35.7119459231226,48.4645308057789,-457.606563638471));
#35676=CARTESIAN_POINT('Ctrl Pts',(-36.0248058566361,48.864845458328,-457.027117389066));
#35677=CARTESIAN_POINT('Ctrl Pts',(-36.1793251274998,49.0625579858903,-456.740933054251));
#35678=CARTESIAN_POINT('Ctrl Pts',(-36.3336936595474,49.2603882238248,-456.454695245554));
#35679=CARTESIAN_POINT('Ctrl Pts',(-36.4879038616631,49.4583367475293,-456.168403852554));
#35680=CARTESIAN_POINT('Ctrl Pts',(-36.638392356481,49.6515079837707,-455.889021812838));
#35681=CARTESIAN_POINT('Ctrl Pts',(-36.7887301080094,49.8447918519287,-455.609588750752));
#35682=CARTESIAN_POINT('Ctrl Pts',(-36.9389093948188,50.0381891337709,-455.3301044329));
#35683=CARTESIAN_POINT('Ctrl Pts',(-37.1322995026599,50.2872322740483,-454.970204585739));
#35684=CARTESIAN_POINT('Ctrl Pts',(-37.3254267825243,50.5364635005466,-454.61021973336));
#35685=CARTESIAN_POINT('Ctrl Pts',(-37.5183771437858,50.7858120942428,-454.250168817144));
#35686=CARTESIAN_POINT('Ctrl Pts',(-37.966147964044,51.364463637571,-453.414615605247));
#35687=CARTESIAN_POINT('Ctrl Pts',(-38.4129638434758,51.9437479729391,-452.578706228737));
#35688=CARTESIAN_POINT('Ctrl Pts',(-38.8599346489484,52.5227688428812,-451.742683706805));
#35689=CARTESIAN_POINT('Ctrl Pts',(-39.1288363106765,52.8711130125594,-451.239725028884));
#35690=CARTESIAN_POINT('Ctrl Pts',(-39.3978733828416,53.2193903825393,-450.736741027798));
#35691=CARTESIAN_POINT('Ctrl Pts',(-39.66697915764,53.5676559225319,-450.233714423801));
#35692=CARTESIAN_POINT('Ctrl Pts',(-40.0363272928394,54.0456509705641,-449.543309551288));
#35693=CARTESIAN_POINT('Ctrl Pts',(-40.4058448879359,54.5236092111141,-448.852831713002));
#35694=CARTESIAN_POINT('Ctrl Pts',(-40.7754155172909,55.0016525637938,-448.162246229423));
#35695=CARTESIAN_POINT('Ctrl Pts',(-40.7757719639103,55.0021136311065,-448.161580167671));
#35696=CARTESIAN_POINT('Ctrl Pts',(-40.7761284105743,55.0025746985001,-448.160914105818));
#35697=CARTESIAN_POINT('Ctrl Pts',(-40.7764848572834,55.0030357659744,-448.160248043864));
#35698=CARTESIAN_POINT('Ctrl Pts',(-40.7904737629383,55.0211305589256,-448.134108153664));
#35699=CARTESIAN_POINT('Ctrl Pts',(-40.8044627379204,55.0392254761776,-448.107968108053));
#35700=CARTESIAN_POINT('Ctrl Pts',(-40.8184517749489,55.0573205202613,-448.081827904509));
#35701=CARTESIAN_POINT('Ctrl Pts',(-40.8358492649381,55.0798244529948,-448.049318595359));
#35702=CARTESIAN_POINT('Ctrl Pts',(-40.8532468508926,55.102328581895,-448.016809041938));
#35703=CARTESIAN_POINT('Ctrl Pts',(-40.8706445188036,55.1248329118314,-447.984299239393));
#35704=CARTESIAN_POINT('Ctrl Pts',(-41.4739715182697,55.9052518694137,-446.856904365388));
#35705=CARTESIAN_POINT('Ctrl Pts',(-42.0773974766002,56.6859124889152,-445.729210014854));
#35706=CARTESIAN_POINT('Ctrl Pts',(-42.6803354117444,57.4670186160727,-444.601012991219));
#35707=CARTESIAN_POINT('Ctrl Pts',(-42.6833788659852,57.4709614112041,-444.595318182822));
#35708=CARTESIAN_POINT('Ctrl Pts',(-42.6864223077834,57.4749042176885,-444.589623361614));
#35709=CARTESIAN_POINT('Ctrl Pts',(-42.6894657370635,57.4788470355523,-444.58392852757));
#35710=CARTESIAN_POINT('Ctrl Pts',(-42.6899071930391,57.4794189497801,-444.58310247962));
#35711=CARTESIAN_POINT('Ctrl Pts',(-42.6903486487513,57.4799908642473,-444.582276431399));
#35712=CARTESIAN_POINT('Ctrl Pts',(-42.6909521381443,57.4807726972959,-444.581147186073));
#35713=CARTESIAN_POINT('Ctrl Pts',(-42.6911141720531,57.48098261567,-444.5808439892));
#35714=CARTESIAN_POINT('Ctrl Pts',(-43.3270604099691,58.304864795902,-443.390864823559));
#35715=CARTESIAN_POINT('Ctrl Pts',(-43.9622971783327,59.1290339922837,-442.200628251578));
#35716=CARTESIAN_POINT('Ctrl Pts',(-44.6005428302862,59.9554878348756,-441.006936117221));
#35717=CARTESIAN_POINT('Ctrl Pts',(-44.602285406408,59.957744256079,-441.003677044461));
#35718=CARTESIAN_POINT('Ctrl Pts',(-44.6424331383656,60.0097303387795,-440.92859067022));
#35719=CARTESIAN_POINT('Ctrl Pts',(-44.6808382846717,60.059460000074,-440.856763370203));
#35720=CARTESIAN_POINT('Ctrl Pts',(-44.7192434309778,60.1091896613684,-440.784936070187));
#35721=CARTESIAN_POINT('Ctrl Pts',(-32.6383541991618,45.2203697961812,-462.499999999991));
#35722=CARTESIAN_POINT('Ctrl Pts',(-33.2597909482979,46.0516256021186,-461.305896380459));
#35723=CARTESIAN_POINT('Ctrl Pts',(-33.8815365596243,46.8833446286893,-460.11131967209));
#35724=CARTESIAN_POINT('Ctrl Pts',(-34.5020794511689,47.7164126393723,-458.915958576709));
#35725=CARTESIAN_POINT('Ctrl Pts',(-34.5281934076432,47.751470170556,-458.865654870001));
#35726=CARTESIAN_POINT('Ctrl Pts',(-34.55430523456,47.7865300904887,-458.815349774274));
#35727=CARTESIAN_POINT('Ctrl Pts',(-34.5804149052619,47.8215923998134,-458.76504328668));
#35728=CARTESIAN_POINT('Ctrl Pts',(-34.8808972539054,48.2251059168955,-458.18609260911));
#35729=CARTESIAN_POINT('Ctrl Pts',(-35.1810932773081,48.6289361814173,-457.606957435406));
#35730=CARTESIAN_POINT('Ctrl Pts',(-35.4809666250378,49.0330825307212,-457.02763430117));
#35731=CARTESIAN_POINT('Ctrl Pts',(-35.6290719145911,49.2326875057504,-456.741510772053));
#35732=CARTESIAN_POINT('Ctrl Pts',(-35.7770986636649,49.4323695190089,-456.455341427537));
#35733=CARTESIAN_POINT('Ctrl Pts',(-35.9250425936302,49.6321284546669,-456.169125866008));
#35734=CARTESIAN_POINT('Ctrl Pts',(-36.0694160464399,49.8270664103998,-455.889817827648));
#35735=CARTESIAN_POINT('Ctrl Pts',(-36.2137106732404,50.0220776044787,-455.610465784224));
#35736=CARTESIAN_POINT('Ctrl Pts',(-36.3579216923215,50.2171622298651,-455.331069204655));
#35737=CARTESIAN_POINT('Ctrl Pts',(-36.5436262932987,50.4683782100658,-454.971282340559));
#35738=CARTESIAN_POINT('Ctrl Pts',(-36.7291921822414,50.7197159827528,-454.61142161106));
#35739=CARTESIAN_POINT('Ctrl Pts',(-36.9146514253514,50.9711455673303,-454.251493908347));
#35740=CARTESIAN_POINT('Ctrl Pts',(-37.3450379603595,51.5546263682339,-453.416226632226));
#35741=CARTESIAN_POINT('Ctrl Pts',(-37.7748474534568,52.1386025657758,-452.580598193939));
#35742=CARTESIAN_POINT('Ctrl Pts',(-38.2045250964898,52.7226837998791,-451.744702485881));
#35743=CARTESIAN_POINT('Ctrl Pts',(-38.4630230359624,53.0740723302074,-451.241820100329));
#35744=CARTESIAN_POINT('Ctrl Pts',(-38.7216235428773,53.4254413601958,-450.738870235561));
#35745=CARTESIAN_POINT('Ctrl Pts',(-38.980290086803,53.7768219194506,-450.235845286766));
#35746=CARTESIAN_POINT('Ctrl Pts',(-39.3353103598129,54.2590923367369,-449.545442686022));
#35747=CARTESIAN_POINT('Ctrl Pts',(-39.6905029782764,54.7413670799393,-448.85490737208));
#35748=CARTESIAN_POINT('Ctrl Pts',(-40.0458403977317,55.2237023319474,-448.164231613875));
#35749=CARTESIAN_POINT('Ctrl Pts',(-40.0461831165839,55.2241675387477,-448.163565465054));
#35750=CARTESIAN_POINT('Ctrl Pts',(-40.0465258355652,55.2246327456062,-448.162899316101));
#35751=CARTESIAN_POINT('Ctrl Pts',(-40.0468685546759,55.2250979525229,-448.162233167017));
#35752=CARTESIAN_POINT('Ctrl Pts',(-40.0603187147842,55.2433551996868,-448.136089857356));
#35753=CARTESIAN_POINT('Ctrl Pts',(-40.0737690742939,55.2616125364301,-448.109946345064));
#35754=CARTESIAN_POINT('Ctrl Pts',(-40.0872196217972,55.2798699676587,-448.08380262752));
#35755=CARTESIAN_POINT('Ctrl Pts',(-40.1039474183612,55.3025758534449,-448.051288948177));
#35756=CARTESIAN_POINT('Ctrl Pts',(-40.1206755056895,55.3252818853689,-448.018774951378));
#35757=CARTESIAN_POINT('Ctrl Pts',(-40.1374038618344,55.347988072869,-447.98626063208));
#35758=CARTESIAN_POINT('Ctrl Pts',(-40.7175200573205,56.135407170867,-446.858709123344));
#35759=CARTESIAN_POINT('Ctrl Pts',(-41.2979599832958,56.9230132620828,-445.730769918261));
#35760=CARTESIAN_POINT('Ctrl Pts',(-41.8778052042609,57.7112007315841,-444.602231795743));
#35761=CARTESIAN_POINT('Ctrl Pts',(-41.8807320932388,57.715179271259,-444.596535265579));
#35762=CARTESIAN_POINT('Ctrl Pts',(-41.883658967055,57.719157825749,-444.590838720151));
#35763=CARTESIAN_POINT('Ctrl Pts',(-41.8865858255911,57.7231363951044,-444.585142159434));
#35764=CARTESIAN_POINT('Ctrl Pts',(-41.8870103727291,57.7237134951632,-444.584315861025));
#35765=CARTESIAN_POINT('Ctrl Pts',(-41.8874349195456,57.7242905955347,-444.583489562295));
#35766=CARTESIAN_POINT('Ctrl Pts',(-41.8880152936402,57.7250795180474,-444.582359974441));
#35767=CARTESIAN_POINT('Ctrl Pts',(-41.8881711211969,57.7252913399177,-444.582056685595));
#35768=CARTESIAN_POINT('Ctrl Pts',(-42.4997588024213,58.5566443504447,-443.391716515218));
#35769=CARTESIAN_POINT('Ctrl Pts',(-43.110522288096,59.3884347749287,-442.201011894464));
#35770=CARTESIAN_POINT('Ctrl Pts',(-43.7244373063526,60.2224959997518,-441.006826656209));
#35771=CARTESIAN_POINT('Ctrl Pts',(-43.726113455465,60.2247731907088,-441.003566236976));
#35772=CARTESIAN_POINT('Ctrl Pts',(-43.7647308003352,60.2772377852853,-440.928448837104));
#35773=CARTESIAN_POINT('Ctrl Pts',(-43.8016719849895,60.3274251889655,-440.856591858102));
#35774=CARTESIAN_POINT('Ctrl Pts',(-43.8386131696438,60.3776125926457,-440.784734879101));
#35775=CARTESIAN_POINT('Ctrl Pts',(-32.2184964333868,45.3306825375905,-462.499999999992));
#35776=CARTESIAN_POINT('Ctrl Pts',(-32.8111445755329,46.1696524166233,-461.305940121841));
#35777=CARTESIAN_POINT('Ctrl Pts',(-33.4036575962112,47.0092828772597,-460.111406153985));
#35778=CARTESIAN_POINT('Ctrl Pts',(-33.9959283196953,47.8496414198625,-458.916258639274));
#35779=CARTESIAN_POINT('Ctrl Pts',(-34.0208525144688,47.8850057543887,-458.86596392056));
#35780=CARTESIAN_POINT('Ctrl Pts',(-34.0457762803665,47.9203713782159,-458.815668115338));
#35781=CARTESIAN_POINT('Ctrl Pts',(-34.0706996094887,47.9557382963416,-458.76537121323));
#35782=CARTESIAN_POINT('Ctrl Pts',(-34.3575289822595,48.3627573945163,-458.18653084992));
#35783=CARTESIAN_POINT('Ctrl Pts',(-34.644299674474,48.7699482318228,-457.607545041494));
#35784=CARTESIAN_POINT('Ctrl Pts',(-34.9310044180742,49.1773166053379,-457.028398945302));
#35785=CARTESIAN_POINT('Ctrl Pts',(-35.0726058287653,49.3785129149502,-456.742362854001));
#35786=CARTESIAN_POINT('Ctrl Pts',(-35.214191342309,49.5797524594164,-456.456287701493));
#35787=CARTESIAN_POINT('Ctrl Pts',(-35.355760189644,49.7810359012113,-456.170171716108));
#35788=CARTESIAN_POINT('Ctrl Pts',(-35.4939124159966,49.9774615706671,-455.890960850722));
#35789=CARTESIAN_POINT('Ctrl Pts',(-35.632048820103,50.1739290262489,-455.611711108655));
#35790=CARTESIAN_POINT('Ctrl Pts',(-35.7701677782543,50.3704392242245,-455.332420665377));
#35791=CARTESIAN_POINT('Ctrl Pts',(-35.9480274603671,50.6234909544982,-454.97277047598));
#35792=CARTESIAN_POINT('Ctrl Pts',(-36.1258581314242,50.8766135926294,-454.613052778229));
#35793=CARTESIAN_POINT('Ctrl Pts',(-36.3036537099415,51.1298101455982,-454.253263180005));
#35794=CARTESIAN_POINT('Ctrl Pts',(-36.7162555392955,51.717391466868,-453.418316396471));
#35795=CARTESIAN_POINT('Ctrl Pts',(-37.1286652611844,52.3053719738747,-452.58298184057));
#35796=CARTESIAN_POINT('Ctrl Pts',(-37.54085746243,52.8937711567081,-451.747213467217));
#35797=CARTESIAN_POINT('Ctrl Pts',(-37.7888360026596,53.2477574038771,-451.244407687371));
#35798=CARTESIAN_POINT('Ctrl Pts',(-38.0368974401792,53.6017882593027,-450.741473324899));
#35799=CARTESIAN_POINT('Ctrl Pts',(-38.2850266726511,53.9558697509131,-450.238417879064));
#35800=CARTESIAN_POINT('Ctrl Pts',(-38.6255844677064,54.441847202467,-449.547973421078));
#35801=CARTESIAN_POINT('Ctrl Pts',(-38.9663238237679,54.927900505144,-448.85731067279));
#35802=CARTESIAN_POINT('Ctrl Pts',(-39.3072807059536,55.4140183332813,-448.166462398451));
#35803=CARTESIAN_POINT('Ctrl Pts',(-39.3076095549431,55.4144871883328,-448.16579608324));
#35804=CARTESIAN_POINT('Ctrl Pts',(-39.3079384041286,55.4149560434464,-448.165129767856));
#35805=CARTESIAN_POINT('Ctrl Pts',(-39.3082672535106,55.4154248986222,-448.164463452298));
#35806=CARTESIAN_POINT('Ctrl Pts',(-39.3211730900984,55.4338253232971,-448.138313609296));
#35807=CARTESIAN_POINT('Ctrl Pts',(-39.3340792292319,55.4522258436757,-448.11216349893));
#35808=CARTESIAN_POINT('Ctrl Pts',(-39.3469856562669,55.4706264654386,-448.086013119611));
#35809=CARTESIAN_POINT('Ctrl Pts',(-39.3630367564735,55.4935104303793,-448.053491155341));
#35810=CARTESIAN_POINT('Ctrl Pts',(-39.3790883019688,55.5163945521283,-448.020968775089));
#35811=CARTESIAN_POINT('Ctrl Pts',(-39.3951402645792,55.5392788416133,-447.988445975798));
#35812=CARTESIAN_POINT('Ctrl Pts',(-39.9518000701818,56.33287426949,-446.860600392663));
#35813=CARTESIAN_POINT('Ctrl Pts',(-40.5089619902815,57.1266713155322,-445.732251028844));
#35814=CARTESIAN_POINT('Ctrl Pts',(-41.0654476693404,57.9211264847329,-444.603269305596));
#35815=CARTESIAN_POINT('Ctrl Pts',(-41.068256646187,57.9251366619217,-444.597570536264));
#35816=CARTESIAN_POINT('Ctrl Pts',(-41.0710656057938,57.9291468558807,-444.591871750819));
#35817=CARTESIAN_POINT('Ctrl Pts',(-41.073874548009,57.9331570666687,-444.586172949239));
#35818=CARTESIAN_POINT('Ctrl Pts',(-41.0742819911305,57.9337387563854,-444.58534632579));
#35819=CARTESIAN_POINT('Ctrl Pts',(-41.074689433886,57.9343204464562,-444.584519702));
#35820=CARTESIAN_POINT('Ctrl Pts',(-41.0752464259017,57.9351156433501,-444.58338966975));
#35821=CARTESIAN_POINT('Ctrl Pts',(-41.0753959754787,57.9353291498666,-444.583086261584));
#35822=CARTESIAN_POINT('Ctrl Pts',(-41.6623439855686,58.7732940367474,-443.392277776917));
#35823=CARTESIAN_POINT('Ctrl Pts',(-42.2483816075473,59.6117803613952,-442.201068283792));
#35824=CARTESIAN_POINT('Ctrl Pts',(-42.8376428218466,60.4524075711013,-441.006506688383));
#35825=CARTESIAN_POINT('Ctrl Pts',(-42.8392516610929,60.4547026876939,-441.003245242575));
#35826=CARTESIAN_POINT('Ctrl Pts',(-42.876318266513,60.5075802484488,-440.928104213679));
#35827=CARTESIAN_POINT('Ctrl Pts',(-42.9117760205334,60.5581626937845,-440.856224631257));
#35828=CARTESIAN_POINT('Ctrl Pts',(-42.9472337745537,60.6087451391203,-440.784345048834));
#35829=CARTESIAN_POINT('Ctrl Pts',(-31.7948796623065,45.4225605594505,-462.499999999992));
#35830=CARTESIAN_POINT('Ctrl Pts',(-32.3588794542992,46.2684182687363,-461.305621084361));
#35831=CARTESIAN_POINT('Ctrl Pts',(-32.9228912587844,47.1142703716486,-460.111245917452));
#35832=CARTESIAN_POINT('Ctrl Pts',(-33.487095575851,47.960402219425,-458.916474195592));
#35833=CARTESIAN_POINT('Ctrl Pts',(-33.5108386678746,47.9960095086962,-458.866195291157));
#35834=CARTESIAN_POINT('Ctrl Pts',(-33.5345821010408,48.0316172932942,-458.815915684491));
#35835=CARTESIAN_POINT('Ctrl Pts',(-33.5583258888889,48.0672255944519,-458.765635345777));
#35836=CARTESIAN_POINT('Ctrl Pts',(-33.8315805468946,48.4770226418846,-458.186985601788));
#35837=CARTESIAN_POINT('Ctrl Pts',(-34.1048813488116,48.8868884209216,-457.608238733626));
#35838=CARTESIAN_POINT('Ctrl Pts',(-34.3782537048229,49.2968534751884,-457.029350268047));
#35839=CARTESIAN_POINT('Ctrl Pts',(-34.5132703451794,49.4993322667469,-456.743441418651));
#35840=CARTESIAN_POINT('Ctrl Pts',(-34.6483046294387,49.7018352029504,-456.457498067189));
#35841=CARTESIAN_POINT('Ctrl Pts',(-34.7833597254613,49.9043659276222,-456.171514872232));
#35842=CARTESIAN_POINT('Ctrl Pts',(-34.9151554033029,50.102008778044,-455.892433592512));
#35843=CARTESIAN_POINT('Ctrl Pts',(-35.0469709497132,50.2996780738909,-455.613314378314));
#35844=CARTESIAN_POINT('Ctrl Pts',(-35.1788083996885,50.4973775420912,-455.334152087623));
#35845=CARTESIAN_POINT('Ctrl Pts',(-35.3485792063683,50.7519607292116,-454.974666923932));
#35846=CARTESIAN_POINT('Ctrl Pts',(-35.5183862530979,51.0065939799953,-454.615110313089));
#35847=CARTESIAN_POINT('Ctrl Pts',(-35.6882312710722,51.2612862178016,-454.255470778925));
#35848=CARTESIAN_POINT('Ctrl Pts',(-36.0823826088463,51.8523385044639,-453.420872241992));
#35849=CARTESIAN_POINT('Ctrl Pts',(-36.4767353190538,52.4437095841588,-452.585826569913));
#35850=CARTESIAN_POINT('Ctrl Pts',(-36.87136162915,53.0354928881843,-451.750199183157));
#35851=CARTESIAN_POINT('Ctrl Pts',(-37.1087723710762,53.3915150531381,-451.247478222116));
#35852=CARTESIAN_POINT('Ctrl Pts',(-37.3462763440645,53.7476890875467,-450.744544962216));
#35853=CARTESIAN_POINT('Ctrl Pts',(-37.5838553593534,54.1039950517834,-450.241428853719));
#35854=CARTESIAN_POINT('Ctrl Pts',(-37.9099329633186,54.5930255958134,-449.550901136127));
#35855=CARTESIAN_POINT('Ctrl Pts',(-38.2362057805615,55.082285128756,-448.860038777299));
#35856=CARTESIAN_POINT('Ctrl Pts',(-38.5627017963575,55.5716951867403,-448.168931295036));
#35857=CARTESIAN_POINT('Ctrl Pts',(-38.5630166980077,55.5721672171096,-448.168264729822));
#35858=CARTESIAN_POINT('Ctrl Pts',(-38.5633315998594,55.5726392476211,-448.167598164379));
#35859=CARTESIAN_POINT('Ctrl Pts',(-38.5636465019127,55.5731112782746,-448.166931598707));
#35860=CARTESIAN_POINT('Ctrl Pts',(-38.5760049695387,55.5916363259503,-448.140771939877));
#35861=CARTESIAN_POINT('Ctrl Pts',(-38.5883637478265,55.6101615924535,-448.114611928373));
#35862=CARTESIAN_POINT('Ctrl Pts',(-38.6007228216992,55.6286870798237,-448.088451565684));
#35863=CARTESIAN_POINT('Ctrl Pts',(-38.616093205203,55.651726334092,-448.055917185578));
#35864=CARTESIAN_POINT('Ctrl Pts',(-38.6314640458791,55.6747659299684,-448.023382262304));
#35865=CARTESIAN_POINT('Ctrl Pts',(-38.6468353147218,55.6978058713774,-447.990846798726));
#35866=CARTESIAN_POINT('Ctrl Pts',(-39.1798896043096,56.4967990921528,-446.862562035657));
#35867=CARTESIAN_POINT('Ctrl Pts',(-39.7134592987254,57.2962077502379,-445.733627656976));
#35868=CARTESIAN_POINT('Ctrl Pts',(-40.2463313260584,58.0961962652654,-444.604161990745));
#35869=CARTESIAN_POINT('Ctrl Pts',(-40.2490211081019,58.1002343731646,-444.59846077861));
#35870=CARTESIAN_POINT('Ctrl Pts',(-40.2517108723597,58.1042724958398,-444.592759552937));
#35871=CARTESIAN_POINT('Ctrl Pts',(-40.2544006186752,58.1083106333122,-444.587058313738));
#35872=CARTESIAN_POINT('Ctrl Pts',(-40.2547907721747,58.1088963738547,-444.586231336706));
#35873=CARTESIAN_POINT('Ctrl Pts',(-40.2551809252966,58.1094821147085,-444.58540435939));
#35874=CARTESIAN_POINT('Ctrl Pts',(-40.2557142815918,58.1102828491458,-444.584273843927));
#35875=CARTESIAN_POINT('Ctrl Pts',(-40.2558574850924,58.1104978424598,-444.583970306028));
#35876=CARTESIAN_POINT('Ctrl Pts',(-40.817898576209,58.9542980499274,-443.392652678696));
#35877=CARTESIAN_POINT('Ctrl Pts',(-41.3790115672474,59.7985292162566,-442.201048219499));
#35878=CARTESIAN_POINT('Ctrl Pts',(-41.9432149726083,60.6444843430236,-441.006495234176));
#35879=CARTESIAN_POINT('Ctrl Pts',(-41.9447553974262,60.6467940028981,-441.003233814901));
#35880=CARTESIAN_POINT('Ctrl Pts',(-41.980245779804,60.7000065541704,-440.928093467114));
#35881=CARTESIAN_POINT('Ctrl Pts',(-42.0141957256967,60.7509094499825,-440.856214536236));
#35882=CARTESIAN_POINT('Ctrl Pts',(-42.0481456715894,60.8018123457946,-440.784335605358));
#35883=CARTESIAN_POINT('',(-56.601452649167,53.2766361680307,-440.999994148306));
#35884=CARTESIAN_POINT('Ctrl Pts',(-56.601452649167,53.2766361680307,-440.999994148306));
#35885=CARTESIAN_POINT('Ctrl Pts',(-54.7738391120521,52.0698384740113,-443.227191994004));
#35886=CARTESIAN_POINT('Ctrl Pts',(-53.3158598386457,51.107187317318,-445.003882932941));
#35887=CARTESIAN_POINT('Ctrl Pts',(-51.6833143334207,50.029459956972,-446.993158893569));
#35888=CARTESIAN_POINT('Ctrl Pts',(-51.0056480219981,49.582157997243,-447.818856763786));
#35889=CARTESIAN_POINT('Ctrl Pts',(-50.4575987060053,49.2205386069633,-448.486525753376));
#35890=CARTESIAN_POINT('Ctrl Pts',(-50.2442148715028,49.0797866305474,-448.746448951586));
#35891=CARTESIAN_POINT('Ctrl Pts',(-50.1400159078363,49.0110713760401,-448.873361284946));
#35892=CARTESIAN_POINT('Ctrl Pts',(-50.0938062106593,48.9806040828583,-448.929638990356));
#35893=CARTESIAN_POINT('Ctrl Pts',(-50.0719407184908,48.966189323167,-448.956267112864));
#35894=CARTESIAN_POINT('Ctrl Pts',(-50.0725610927088,48.9665983008579,-448.955511613539));
#35895=CARTESIAN_POINT('Ctrl Pts',(-49.7377894632215,48.7459020199295,-449.363200799079));
#35896=CARTESIAN_POINT('Ctrl Pts',(-49.4352278905934,48.5459054812786,-449.732078168407));
#35897=CARTESIAN_POINT('Ctrl Pts',(-49.0277940186024,48.275622186605,-450.229556155105));
#35898=CARTESIAN_POINT('Ctrl Pts',(-48.8356784662846,48.1479084645981,-450.464336151231));
#35899=CARTESIAN_POINT('Ctrl Pts',(-48.631853759036,48.0119009321817,-450.713817161894));
#35900=CARTESIAN_POINT('Ctrl Pts',(-48.5281028279955,47.9425189717714,-450.840924242818));
#35901=CARTESIAN_POINT('Ctrl Pts',(-48.4811669407684,47.9110877548734,-450.898459603619));
#35902=CARTESIAN_POINT('Ctrl Pts',(-48.4547091942354,47.89335897057,-450.930900721537));
#35903=CARTESIAN_POINT('Ctrl Pts',(-48.4493956713363,47.8897979200664,-450.93741632498));
#35904=CARTESIAN_POINT('Ctrl Pts',(-48.1911818927057,47.7167009016883,-451.254080950314));
#35905=CARTESIAN_POINT('Ctrl Pts',(-47.923909337161,47.5360147897983,-451.583018814021));
#35906=CARTESIAN_POINT('Ctrl Pts',(-47.6043364692148,47.3181959778586,-451.977676579559));
#35907=CARTESIAN_POINT('Ctrl Pts',(-47.5685660211511,47.2937918188525,-452.02186914582));
#35908=CARTESIAN_POINT('Ctrl Pts',(-47.4965008239971,47.2445789396727,-452.11093768424));
#35909=CARTESIAN_POINT('Ctrl Pts',(-47.4642724250937,47.2225555768963,-452.150781383843));
#35910=CARTESIAN_POINT('Ctrl Pts',(-47.3634872668974,47.1536731292441,-452.275388990803));
#35911=CARTESIAN_POINT('Ctrl Pts',(-47.1661706984304,47.0187276878275,-452.519410718903));
#35912=CARTESIAN_POINT('Ctrl Pts',(-46.969015806605,46.8836314119994,-452.763428011278));
#35913=CARTESIAN_POINT('Ctrl Pts',(-46.8348570128172,46.7915814454118,-452.929565431352));
#35914=CARTESIAN_POINT('Ctrl Pts',(-46.8316879630588,46.7894070127498,-452.933489914907));
#35915=CARTESIAN_POINT('Ctrl Pts',(-46.4926707116515,46.5567784766192,-453.353331356604));
#35916=CARTESIAN_POINT('Ctrl Pts',(-46.1908192095058,46.3511215126281,-453.726005587852));
#35917=CARTESIAN_POINT('Ctrl Pts',(-45.7857235243058,46.0779816977538,-454.223955146678));
#35918=CARTESIAN_POINT('Ctrl Pts',(-45.5950973931695,45.9502467837759,-454.457664487715));
#35919=CARTESIAN_POINT('Ctrl Pts',(-45.3935239240952,45.8167251802618,-454.703611002445));
#35920=CARTESIAN_POINT('Ctrl Pts',(-45.297939241582,45.7538440372232,-454.819905681308));
#35921=CARTESIAN_POINT('Ctrl Pts',(-45.2481260815286,45.7211974134129,-454.880417499361));
#35922=CARTESIAN_POINT('Ctrl Pts',(-45.2252590617721,45.7062454173416,-454.908169368993));
#35923=CARTESIAN_POINT('Ctrl Pts',(-45.2122850284238,45.6977707604777,-454.923908320153));
#35924=CARTESIAN_POINT('Ctrl Pts',(-45.2098033528762,45.696150112695,-454.926918574951));
#35925=CARTESIAN_POINT('Ctrl Pts',(-44.6961082429141,45.3608345902825,-455.549911919046));
#35926=CARTESIAN_POINT('Ctrl Pts',(-44.1419304533118,45.0135796250764,-456.210946793152));
#35927=CARTESIAN_POINT('Ctrl Pts',(-43.5419127712896,44.6532698807934,-456.914899800777));
#35928=CARTESIAN_POINT('Ctrl Pts',(-41.9462958339113,60.6491036583583,-440.999972397991));
#35929=CARTESIAN_POINT('Ctrl Pts',(-42.4536076986967,60.5401595182708,-440.999978861914));
#35930=CARTESIAN_POINT('Ctrl Pts',(-42.9582396954925,60.4191084556018,-441.000072725249));
#35931=CARTESIAN_POINT('Ctrl Pts',(-43.9613151855463,60.1529933426888,-441.000299642132));
#35932=CARTESIAN_POINT('Ctrl Pts',(-44.4596200480986,60.0079647356423,-441.000418945381));
#35933=CARTESIAN_POINT('Ctrl Pts',(-45.9432689217911,59.5374326211282,-441.000516453555));
#35934=CARTESIAN_POINT('Ctrl Pts',(-46.9167473739368,59.1766923215432,-441.000393081996));
#35935=CARTESIAN_POINT('Ctrl Pts',(-48.5073188404937,58.4992293403753,-441.000331534641));
#35936=CARTESIAN_POINT('Ctrl Pts',(-49.134498395159,58.2081810247175,-441.000338333599));
#35937=CARTESIAN_POINT('Ctrl Pts',(-50.986111138267,57.2761989420374,-441.000292512001));
#35938=CARTESIAN_POINT('Ctrl Pts',(-52.1794941815985,56.5771072599769,-441.000229810147));
#35939=CARTESIAN_POINT('Ctrl Pts',(-53.8971333256094,55.4182676375983,-441.000147690528));
#35940=CARTESIAN_POINT('Ctrl Pts',(-54.4569722800717,55.0140887402452,-441.000120670842));
#35941=CARTESIAN_POINT('Ctrl Pts',(-55.2767819376056,54.3816364844746,-441.000066623273));
#35942=CARTESIAN_POINT('Ctrl Pts',(-55.5466526868058,54.1665147681349,-441.000049725274));
#35943=CARTESIAN_POINT('Ctrl Pts',(-55.9462310386895,53.8374804277519,-441.000028586167));
#35944=CARTESIAN_POINT('Ctrl Pts',(-56.0785341359438,53.7267594825738,-441.000022093514));
#35945=CARTESIAN_POINT('Ctrl Pts',(-56.2756523821078,53.5591158372563,-441.000012193514));
#35946=CARTESIAN_POINT('Ctrl Pts',(-56.3411311310312,53.5029782684191,-441.000008857992));
#35947=CARTESIAN_POINT('Ctrl Pts',(-56.4390115504381,53.418384631197,-441.000003597922));
#35948=CARTESIAN_POINT('Ctrl Pts',(-56.4715809264883,53.39012321023,-441.000001801287));
#35949=CARTESIAN_POINT('Ctrl Pts',(-56.5437212175141,53.3272733766563,-440.999997673909));
#35950=CARTESIAN_POINT('Ctrl Pts',(-56.5769261061491,53.2981760183113,-440.999995669541));
#35951=CARTESIAN_POINT('Ctrl Pts',(-56.601452649167,53.2766361680308,-440.999994148306));
#35952=CARTESIAN_POINT('Ctrl Pts',(-64.2658958771365,45.6374763139969,-440.999637204112));
#35953=CARTESIAN_POINT('Ctrl Pts',(-55.774321890447,32.4272154387425,-456.914897282309));
#35954=CARTESIAN_POINT('Ctrl Pts',(-61.8717342174773,48.3453380510754,-440.999999999991));
#35955=CARTESIAN_POINT('Ctrl Pts',(-51.8201097042196,36.6236615680269,-456.919527670999));
#35956=CARTESIAN_POINT('Ctrl Pts',(-59.3135877730462,50.8952105744119,-440.999999999991));
#35957=CARTESIAN_POINT('Ctrl Pts',(-47.7405554577368,40.7010682615931,-456.919527671));
#35958=CARTESIAN_POINT('Ctrl Pts',(-56.601452649167,53.2766361680307,-440.999994148306));
#35959=CARTESIAN_POINT('Ctrl Pts',(-43.5418850322421,44.6532394081086,-456.91486065554));
#35960=CARTESIAN_POINT('Ctrl Pts',(-56.6012177920432,53.2768423873892,-440.999994147799));
#35961=CARTESIAN_POINT('Ctrl Pts',(-43.5415211446437,44.6535819322701,-456.914860251062));
#35962=CARTESIAN_POINT('Ctrl Pts',(-56.6009829349194,53.2770486067477,-440.999994147292));
#35963=CARTESIAN_POINT('Ctrl Pts',(-43.5411572570453,44.6539244564316,-456.914859846584));
#35964=CARTESIAN_POINT('Ctrl Pts',(-56.6007480777956,53.2772548261063,-440.999994146786));
#35965=CARTESIAN_POINT('Ctrl Pts',(-43.5407933694469,44.6542669805931,-456.914859442107));
#35966=CARTESIAN_POINT('',(-64.2657028580431,45.6371756443949,-440.999998037155));
#35967=CARTESIAN_POINT('',(-64.2657034184046,45.63717615959,-440.999998440138));
#35968=CARTESIAN_POINT('Ctrl Pts',(-56.601452649167,53.2766361680308,-440.999994148306));
#35969=CARTESIAN_POINT('Ctrl Pts',(-57.7028809440721,52.3093280492766,-441.000142795397));
#35970=CARTESIAN_POINT('Ctrl Pts',(-58.7792997824101,51.3139675750334,-441.000170909128));
#35971=CARTESIAN_POINT('Ctrl Pts',(-59.8294787290137,50.2917255855174,-441.00015198801));
#35972=CARTESIAN_POINT('Ctrl Pts',(-60.8795257991174,49.2696119643105,-441.000133069268));
#35973=CARTESIAN_POINT('Ctrl Pts',(-61.9033396129511,48.220623538411,-441.000067127489));
#35974=CARTESIAN_POINT('Ctrl Pts',(-62.8997269250625,47.1459676259387,-441.000027633498));
#35975=CARTESIAN_POINT('Ctrl Pts',(-63.3609673081903,46.6484957103752,-441.000009351227));
#35976=CARTESIAN_POINT('Ctrl Pts',(-63.8163310265106,46.1455240769036,-440.999996736404));
#35977=CARTESIAN_POINT('Ctrl Pts',(-64.2657023428471,45.6371752088159,-440.999997077097));
#35978=CARTESIAN_POINT('Ctrl Pts',(-69.7776904941909,32.0305578312519,-441.000027286454));
#35979=CARTESIAN_POINT('Ctrl Pts',(-56.5915605594688,20.6258796622837,-462.499999999988));
#35980=CARTESIAN_POINT('Ctrl Pts',(-69.5425906598027,37.113747189771,-440.99999999999));
#35981=CARTESIAN_POINT('Ctrl Pts',(-56.0041009291263,23.3343857139598,-462.499999999988));
#35982=CARTESIAN_POINT('Ctrl Pts',(-67.6327997693356,41.8281639590277,-440.99999999999));
#35983=CARTESIAN_POINT('Ctrl Pts',(-54.7064708585609,25.7833181444718,-462.499999999989));
#35984=CARTESIAN_POINT('Ctrl Pts',(-64.2658958771893,45.637476314079,-440.999637204013));
#35985=CARTESIAN_POINT('Ctrl Pts',(-52.7943871585138,27.7913593228122,-462.500014523132));
#35986=CARTESIAN_POINT('',(-69.7776893278308,32.0305568224675,-441.000029188202));
#35987=CARTESIAN_POINT('Origin',(-47.7274224530678,31.0176628730264,-440.980660458913));
#35988=CARTESIAN_POINT('Origin',(-54.2736315587492,-11.1690000000156,-438.999999999984));
#35989=CARTESIAN_POINT('',(-70.5084762417148,-34.7635952579923,-438.99999999998));
#35990=CARTESIAN_POINT('',(-70.4554509568028,-36.792411599386,-438.99999999998));
#35991=CARTESIAN_POINT('Origin',(871.003976208289,-11.171261467625,-438.999999999992));
#35992=CARTESIAN_POINT('Ctrl Pts',(-70.508476241715,-34.7635952579923,-438.999999999982));
#35993=CARTESIAN_POINT('Ctrl Pts',(-70.4767675684555,-35.1005664161786,
-438.999999999982));
#35994=CARTESIAN_POINT('Ctrl Pts',(-70.456475079011,-35.4385125585903,-438.999999999979));
#35995=CARTESIAN_POINT('Ctrl Pts',(-70.4387772188577,-36.1153666437888,
-438.999999999979));
#35996=CARTESIAN_POINT('Ctrl Pts',(-70.4413882261958,-36.45407804119,-438.999999999981));
#35997=CARTESIAN_POINT('Ctrl Pts',(-70.4554509568029,-36.7924115993857,
-438.999999999981));
#35998=CARTESIAN_POINT('Ctrl Pts',(-69.7814241414421,-54.3757509201429,
-440.993983453141));
#35999=CARTESIAN_POINT('Ctrl Pts',(-69.7777140088065,-54.3725409130246,
-441.000032808645));
#36000=CARTESIAN_POINT('Ctrl Pts',(-56.5915605594633,-42.9638796623204,
-462.499999999981));
#36001=CARTESIAN_POINT('Ctrl Pts',(-56.5783744060139,-42.9524710010697,
-462.521499967173));
#36002=CARTESIAN_POINT('Ctrl Pts',(-69.9806527515224,-49.9927595127392,
-440.993963941929));
#36003=CARTESIAN_POINT('Ctrl Pts',(-69.9770872889478,-49.9898995318794,
-440.99999999998));
#36004=CARTESIAN_POINT('Ctrl Pts',(-57.277168782509,-39.8028556101424,-462.499999999981));
#36005=CARTESIAN_POINT('Ctrl Pts',(-57.2644408666255,-39.792646108556,-462.52154739742));
#36006=CARTESIAN_POINT('Ctrl Pts',(-70.1511013536826,-45.6102732255524,
-440.993975224971));
#36007=CARTESIAN_POINT('Ctrl Pts',(-70.1476583281878,-45.6077541556496,
-440.99999999998));
#36008=CARTESIAN_POINT('Ctrl Pts',(-57.8608844602732,-36.6182063587309,
-462.499999999982));
#36009=CARTESIAN_POINT('Ctrl Pts',(-57.8485475387398,-36.6091801206816,
-462.521587750828));
#36010=CARTESIAN_POINT('Ctrl Pts',(-70.2928114147138,-41.2265701727283,
-440.994016766951));
#36011=CARTESIAN_POINT('Ctrl Pts',(-70.2894684716153,-41.2243846605893,
-441.000032274629));
#36012=CARTESIAN_POINT('Ctrl Pts',(-58.341487923045,-33.4131668933052,-462.499999999982));
#36013=CARTESIAN_POINT('Ctrl Pts',(-58.3294727137636,-33.4053117234853,
-462.521620943431));
#36014=CARTESIAN_POINT('',(-70.2893406259791,-41.2283906269187,-441.000029101383));
#36015=CARTESIAN_POINT('Ctrl Pts',(-70.2893406186478,-41.228390626661,-441.000029070991));
#36016=CARTESIAN_POINT('Ctrl Pts',(-70.1494588909743,-45.6109060280408,
-440.996616656315));
#36017=CARTESIAN_POINT('Ctrl Pts',(-69.9789058201507,-49.992411625971,-440.996967909007));
#36018=CARTESIAN_POINT('Ctrl Pts',(-69.7777140088065,-54.3725409130246,
-441.000032808645));
#36019=CARTESIAN_POINT('Ctrl Pts',(-70.2893406401635,-41.2283906506288,
-441.000029112448));
#36020=CARTESIAN_POINT('Ctrl Pts',(-69.123590435456,-40.9599833732949,-443.069542538055));
#36021=CARTESIAN_POINT('Ctrl Pts',(-67.9450458275156,-40.6639886984268,
-445.141170812192));
#36022=CARTESIAN_POINT('Ctrl Pts',(-65.551152303873,-40.004777240294,-449.304140893811));
#36023=CARTESIAN_POINT('Ctrl Pts',(-64.3222984007391,-39.6362874672872,
-451.417506435825));
#36024=CARTESIAN_POINT('Ctrl Pts',(-61.3238515421179,-38.6439304718567,
-456.517206904405));
#36025=CARTESIAN_POINT('Ctrl Pts',(-59.5048995836444,-37.9635263279722,
-459.558563915027));
#36026=CARTESIAN_POINT('Ctrl Pts',(-57.7295804999056,-37.1684431733089,
-462.499999999981));
#36027=CARTESIAN_POINT('Ctrl Pts',(-70.292529859086,18.8884758131824,-440.994261297969));
#36028=CARTESIAN_POINT('Ctrl Pts',(-70.2893242457657,18.886380058914,-441.000029755883));
#36029=CARTESIAN_POINT('Ctrl Pts',(-58.3414879230488,11.0751668932692,-462.499999999987));
#36030=CARTESIAN_POINT('Ctrl Pts',(-58.3294728588049,11.0673117280768,-462.521620945969));
#36031=CARTESIAN_POINT('Ctrl Pts',(-70.15095995233,23.2721697700229,-440.994222656018));
#36032=CARTESIAN_POINT('Ctrl Pts',(-70.1476583281939,23.2697541556153,-440.999999999988));
#36033=CARTESIAN_POINT('Ctrl Pts',(-57.8608844602774,14.2802063586947,-462.499999999988));
#36034=CARTESIAN_POINT('Ctrl Pts',(-57.8485475387442,14.2711801206454,-462.521587750834));
#36035=CARTESIAN_POINT('Ctrl Pts',(-69.9805063218111,27.6546420563625,-440.994211836358));
#36036=CARTESIAN_POINT('Ctrl Pts',(-69.9770872889547,27.6518995318446,-440.999999999989));
#36037=CARTESIAN_POINT('Ctrl Pts',(-57.277168782514,17.4648556101059,-462.499999999988));
#36038=CARTESIAN_POINT('Ctrl Pts',(-57.2644408666304,17.4546461085195,-462.521547397427));
#36039=CARTESIAN_POINT('Ctrl Pts',(-69.7812482493198,32.0336349321488,-440.994226369993));
#36040=CARTESIAN_POINT('Ctrl Pts',(-69.7776904941909,32.0305578312519,-441.000027286454));
#36041=CARTESIAN_POINT('Ctrl Pts',(-56.5915605594688,20.6258796622837,-462.499999999988));
#36042=CARTESIAN_POINT('Ctrl Pts',(-56.5783744295341,20.6144749841147,-462.521499972702));
#36043=CARTESIAN_POINT('',(-70.289206435783,18.8900706285948,-441.000027137208));
#36044=CARTESIAN_POINT('Ctrl Pts',(-57.7295804999102,14.8304431732719,-462.499999999987));
#36045=CARTESIAN_POINT('Ctrl Pts',(-59.5045045244752,15.6253388507935,-459.559205212572));
#36046=CARTESIAN_POINT('Ctrl Pts',(-61.3230116147034,16.3055894393686,-456.518594345998));
#36047=CARTESIAN_POINT('Ctrl Pts',(-64.3212741457954,17.2978938106733,-451.419209339214));
#36048=CARTESIAN_POINT('Ctrl Pts',(-65.550328672081,17.6664301595495,-449.305489097914));
#36049=CARTESIAN_POINT('Ctrl Pts',(-67.9445832191676,18.3256861822974,-445.141842101897));
#36050=CARTESIAN_POINT('Ctrl Pts',(-69.1233006778753,18.6216836058714,-443.069871435287));
#36051=CARTESIAN_POINT('Ctrl Pts',(-70.2892064356818,18.8900706273276,-441.000027136986));
#36052=CARTESIAN_POINT('Ctrl Pts',(-69.7776893278306,32.0305568224675,-441.000029188203));
#36053=CARTESIAN_POINT('Ctrl Pts',(-69.8782554180672,29.8411055079886,-440.998663142711));
#36054=CARTESIAN_POINT('Ctrl Pts',(-69.9711674064275,27.6513214514411,-440.997879764828));
#36055=CARTESIAN_POINT('Ctrl Pts',(-70.1416774153024,23.2710915157206,-440.997783805102));
#36056=CARTESIAN_POINT('Ctrl Pts',(-70.2192715819682,21.0807504505387,-440.99847273527));
#36057=CARTESIAN_POINT('Ctrl Pts',(-70.289206435962,18.8900706286,-441.00002713642));
#36058=CARTESIAN_POINT('Origin',(-54.2736315587492,-11.1690000000156,-438.999999999984));
#36059=CARTESIAN_POINT('',(-70.4553279483522,14.4544082600061,-438.999999999986));
#36060=CARTESIAN_POINT('',(-70.508362966475,12.4255924277826,-438.999999999986));
#36061=CARTESIAN_POINT('Origin',(871.003976208289,-11.171261467625,-438.999999999992));
#36062=CARTESIAN_POINT('Origin',(-85.4463381859629,13.8311852560246,-439.000015674809));
#36063=CARTESIAN_POINT('Ctrl Pts',(-58.3152526335012,7.11256737780218,-462.499999999986));
#36064=CARTESIAN_POINT('Ctrl Pts',(-70.9880999661371,9.82056904889893,-439.000749857024));
#36065=CARTESIAN_POINT('Ctrl Pts',(-57.2363227355981,9.63550019499528,-462.499999999987));
#36066=CARTESIAN_POINT('Ctrl Pts',(-70.1268305119616,12.9271295702052,-438.999052441603));
#36067=CARTESIAN_POINT('Ctrl Pts',(-57.0028527815747,12.4931127438228,-462.499999999987));
#36068=CARTESIAN_POINT('Ctrl Pts',(-70.2442207404255,16.2699753471456,-439.000717531333));
#36069=CARTESIAN_POINT('Ctrl Pts',(-57.8729593028357,15.3392709969105,-462.499999999987));
#36070=CARTESIAN_POINT('Ctrl Pts',(-71.5424551395504,19.4736999487602,-438.999999999988));
#36071=CARTESIAN_POINT('Ctrl Pts',(-70.2892064359492,18.8900706285019,-441.00002713733));
#36072=CARTESIAN_POINT('Ctrl Pts',(-70.3185646663934,18.2566939697067,-440.477202905431));
#36073=CARTESIAN_POINT('Ctrl Pts',(-70.347804124619,17.5655437203867,-440.030299535459));
#36074=CARTESIAN_POINT('Ctrl Pts',(-70.4043926371724,16.0677660576806,-439.340085108649));
#36075=CARTESIAN_POINT('Ctrl Pts',(-70.4311133436359,15.2759782175062,-439.106074007436));
#36076=CARTESIAN_POINT('Ctrl Pts',(-70.4553279483522,14.454408260006,-438.999999999988));
#36077=CARTESIAN_POINT('',(-70.5581573682015,9.72869661935509,-439.797992054518));
#36078=CARTESIAN_POINT('',(-58.3152526335012,7.11256737780218,-462.499999999987));
#36079=CARTESIAN_POINT('Ctrl Pts',(-70.5083629664747,12.4255924277829,-438.999999999988));
#36080=CARTESIAN_POINT('Ctrl Pts',(-70.5190417311927,11.9581189779784,-439.059413282611));
#36081=CARTESIAN_POINT('Ctrl Pts',(-70.528502917745,11.4975517735212,-439.158641883047));
#36082=CARTESIAN_POINT('Ctrl Pts',(-70.5450909658798,10.5948954496699,-439.428499909191));
#36083=CARTESIAN_POINT('Ctrl Pts',(-70.5521753927515,10.1552367203658,-439.59832946049));
#36084=CARTESIAN_POINT('Ctrl Pts',(-70.5581573682015,9.72869661935604,-439.797992054519));
#36085=CARTESIAN_POINT('Ctrl Pts',(-59.0902650976014,-0.703506953312267,
-462.499999999985));
#36086=CARTESIAN_POINT('Ctrl Pts',(-70.7677853055098,1.15015641282444,-439.798680793982));
#36087=CARTESIAN_POINT('Ctrl Pts',(-59.6440060900478,1.94053476148597,-462.499999999986));
#36088=CARTESIAN_POINT('Ctrl Pts',(-71.4248025866691,3.99812226801711,-439.789824991756));
#36089=CARTESIAN_POINT('Ctrl Pts',(-59.3774521833115,4.62875623508382,-462.499999999986));
#36090=CARTESIAN_POINT('Ctrl Pts',(-71.3533291948978,6.91847187716548,-439.789824991757));
#36091=CARTESIAN_POINT('Ctrl Pts',(-58.3152526335012,7.11256737780218,-462.499999999986));
#36092=CARTESIAN_POINT('Ctrl Pts',(-70.5581573682015,9.72869661935526,-439.797992054521));
#36093=CARTESIAN_POINT('',(-70.707553625092,1.14059537096935,-439.915772315053));
#36094=CARTESIAN_POINT('',(-59.0902650976014,-0.703506953312267,-462.499999999986));
#36095=CARTESIAN_POINT('Ctrl Pts',(-70.5581573682015,9.7286966193551,-439.797992054521));
#36096=CARTESIAN_POINT('Ctrl Pts',(-70.5678046345493,9.04133438885232,-440.119320391241));
#36097=CARTESIAN_POINT('Ctrl Pts',(-70.5782199854561,8.32772296577743,-440.386730380512));
#36098=CARTESIAN_POINT('Ctrl Pts',(-70.6003622288596,6.88955219928298,-440.760094435853));
#36099=CARTESIAN_POINT('Ctrl Pts',(-70.6119275337347,6.17248248578738,-440.870819207139));
#36100=CARTESIAN_POINT('Ctrl Pts',(-70.637063876889,4.7026944634276,-440.916714503241));
#36101=CARTESIAN_POINT('Ctrl Pts',(-70.6503587134966,3.96810546432371,-440.847278158492));
#36102=CARTESIAN_POINT('Ctrl Pts',(-70.6784620794615,2.5112022870367,-440.514928775699));
#36103=CARTESIAN_POINT('Ctrl Pts',(-70.6928736353993,1.81053750859871,-440.254969959199));
#36104=CARTESIAN_POINT('Ctrl Pts',(-70.707553625092,1.14059537097008,-439.915772315053));
#36105=CARTESIAN_POINT('Origin',(-54.2736315587492,-11.1690000000156,-438.999999999984));
#36106=CARTESIAN_POINT('',(-70.7571158415876,-1.77222784066373,-438.999999999984));
#36107=CARTESIAN_POINT('',(-70.776418222841,-3.96119924583428,-438.999999999984));
#36108=CARTESIAN_POINT('Origin',(871.003976208289,-11.171261467625,-438.999999999992));
#36109=CARTESIAN_POINT('Ctrl Pts',(-70.7571158415876,-1.77222784066382,
-438.999999999986));
#36110=CARTESIAN_POINT('Ctrl Pts',(-70.7374577456278,-2.13718693330326,
-438.999999999986));
#36111=CARTESIAN_POINT('Ctrl Pts',(-70.7292454393531,-2.50266922432743,
-438.999999999985));
#36112=CARTESIAN_POINT('Ctrl Pts',(-70.7357313681723,-3.23286508272366,
-438.999999999985));
#36113=CARTESIAN_POINT('Ctrl Pts',(-70.7503808772078,-3.59739324964435,
-438.999999999986));
#36114=CARTESIAN_POINT('Ctrl Pts',(-70.7764182228409,-3.96119924583425,
-438.999999999986));
#36115=CARTESIAN_POINT('Ctrl Pts',(-59.4064050032667,-7.27543664707476,
-462.499999999985));
#36116=CARTESIAN_POINT('Ctrl Pts',(-71.2501735645804,-6.94091182239155,
-439.000746326908));
#36117=CARTESIAN_POINT('Ctrl Pts',(-58.7385280596105,-5.1359471967354,-462.499999999985));
#36118=CARTESIAN_POINT('Ctrl Pts',(-70.5811457040036,-4.25282607367328,
-438.999669295073));
#36119=CARTESIAN_POINT('Ctrl Pts',(-58.6308352736725,-2.89722502017172,
-462.499999999985));
#36120=CARTESIAN_POINT('Ctrl Pts',(-70.5567348878677,-1.48408888094075,
-438.999671718532));
#36121=CARTESIAN_POINT('Ctrl Pts',(-59.0902650976014,-0.703506953312267,
-462.499999999985));
#36122=CARTESIAN_POINT('Ctrl Pts',(-71.1782425626859,1.21531147720845,-439.000744155921));
#36123=CARTESIAN_POINT('',(-70.7782178075338,-6.95424211600733,-439.93715503818));
#36124=CARTESIAN_POINT('',(-59.4064050032667,-7.27543664707476,-462.499999999985));
#36125=CARTESIAN_POINT('Ctrl Pts',(-70.7764182228408,-3.96119924583428,
-438.999999999986));
#36126=CARTESIAN_POINT('Ctrl Pts',(-70.7792259582827,-4.48285116764463,
-439.067939102373));
#36127=CARTESIAN_POINT('Ctrl Pts',(-70.7807027348374,-4.99571525392328,
-439.183374598125));
#36128=CARTESIAN_POINT('Ctrl Pts',(-70.7812087649267,-5.99846114666605,
-439.500477515119));
#36129=CARTESIAN_POINT('Ctrl Pts',(-70.7802394325318,-6.48469492714696,
-439.700886889843));
#36130=CARTESIAN_POINT('Ctrl Pts',(-70.7782178073704,-6.95424211587693,
-439.937155038438));
#36131=CARTESIAN_POINT('Ctrl Pts',(-70.707553625092,1.14059537096959,-439.915772315052));
#36132=CARTESIAN_POINT('Ctrl Pts',(-70.7175664400768,0.684205669526496,
-439.683996098304));
#36133=CARTESIAN_POINT('Ctrl Pts',(-70.7268359140479,0.21125137401857,-439.488172163492));
#36134=CARTESIAN_POINT('Ctrl Pts',(-70.7435314502,-0.76501779240385,-439.178742173232));
#36135=CARTESIAN_POINT('Ctrl Pts',(-70.7508854143187,-1.26427873052628,
-439.066507814377));
#36136=CARTESIAN_POINT('Ctrl Pts',(-70.7571158415874,-1.77222784066387,
-438.999999999986));
#36137=CARTESIAN_POINT('Ctrl Pts',(-59.4064050032661,-15.0625633529625,
-462.499999999984));
#36138=CARTESIAN_POINT('Ctrl Pts',(-70.7782380423279,-15.3837579656666,
-439.937155391899));
#36139=CARTESIAN_POINT('Ctrl Pts',(-60.204044757482,-12.5073892965367,-462.499999999984));
#36140=CARTESIAN_POINT('Ctrl Pts',(-71.4803706009381,-12.6028580262609,
-439.927462314947));
#36141=CARTESIAN_POINT('Ctrl Pts',(-60.2040447574823,-9.83061070350056,
-462.499999999985));
#36142=CARTESIAN_POINT('Ctrl Pts',(-71.4803706009383,-9.73514197377313,
-439.927462314947));
#36143=CARTESIAN_POINT('Ctrl Pts',(-59.4064050032667,-7.27543664707476,
-462.499999999985));
#36144=CARTESIAN_POINT('Ctrl Pts',(-70.7782178073682,-6.95424211638727,
-439.937155038694));
#36145=CARTESIAN_POINT('',(-70.7782380423279,-15.3837579656666,-439.9371553919));
#36146=CARTESIAN_POINT('',(-59.4064050032661,-15.0625633529624,-462.499999999984));
#36147=CARTESIAN_POINT('Ctrl Pts',(-70.7782178073682,-6.95424211638724,
-439.937155038694));
#36148=CARTESIAN_POINT('Ctrl Pts',(-70.7753632379763,-7.61931765885983,
-440.271299916673));
#36149=CARTESIAN_POINT('Ctrl Pts',(-70.773068988079,-8.31344450348613,-440.540438931827));
#36150=CARTESIAN_POINT('Ctrl Pts',(-70.7699981011486,-9.73451302894079,
-440.901051397528));
#36151=CARTESIAN_POINT('Ctrl Pts',(-70.7692082793061,-10.4455629420233,
-440.994026431782));
#36152=CARTESIAN_POINT('Ctrl Pts',(-70.7692093849802,-11.88970116692,-440.99430585424));
#36153=CARTESIAN_POINT('Ctrl Pts',(-70.7700014883587,-12.6013038302797,
-440.901465936896));
#36154=CARTESIAN_POINT('Ctrl Pts',(-70.7730793305623,-14.0235098939738,
-440.540838886405));
#36155=CARTESIAN_POINT('Ctrl Pts',(-70.7753781859942,-14.7181790435964,
-440.271549168403));
#36156=CARTESIAN_POINT('Ctrl Pts',(-70.7782380423279,-15.3837579656657,
-439.9371553919));
#36157=CARTESIAN_POINT('Origin',(-54.2736315587492,-11.1690000000156,-438.999999999984));
#36158=CARTESIAN_POINT('',(-70.7764528366089,-18.3768010105731,-438.999999999982));
#36159=CARTESIAN_POINT('',(-70.7571609664515,-20.5657726010771,-438.999999999982));
#36160=CARTESIAN_POINT('Origin',(871.003976208289,-11.171261467625,-438.999999999992));
#36161=CARTESIAN_POINT('Ctrl Pts',(-70.7764528366089,-18.3768010105731,
-438.999999999984));
#36162=CARTESIAN_POINT('Ctrl Pts',(-70.7503902427032,-18.7409820044107,
-438.999999999984));
#36163=CARTESIAN_POINT('Ctrl Pts',(-70.7357390480042,-19.1058864417604,
-438.999999999983));
#36164=CARTESIAN_POINT('Ctrl Pts',(-70.729303684327,-19.8360828380082,-438.999999999983));
#36165=CARTESIAN_POINT('Ctrl Pts',(-70.7375211543362,-20.2011888207014,
-438.999999999984));
#36166=CARTESIAN_POINT('Ctrl Pts',(-70.7571609664516,-20.5657726010769,
-438.999999999984));
#36167=CARTESIAN_POINT('Ctrl Pts',(-59.0902650975996,-21.634493046725,-462.499999999983));
#36168=CARTESIAN_POINT('Ctrl Pts',(-71.1782916618887,-23.5533103055587,
-439.000769312961));
#36169=CARTESIAN_POINT('Ctrl Pts',(-58.6308352736711,-19.4407749798654,
-462.499999999984));
#36170=CARTESIAN_POINT('Ctrl Pts',(-70.5567881485483,-20.8539012598249,
-438.999654953635));
#36171=CARTESIAN_POINT('Ctrl Pts',(-58.7385280596094,-17.2020528033017,
-462.499999999984));
#36172=CARTESIAN_POINT('Ctrl Pts',(-70.5811778706299,-18.0851841799639,
-438.999671159419));
#36173=CARTESIAN_POINT('Ctrl Pts',(-59.4064050032661,-15.0625633529625,
-462.499999999984));
#36174=CARTESIAN_POINT('Ctrl Pts',(-71.2501905188668,-15.3970881466845,
-439.000754870191));
#36175=CARTESIAN_POINT('',(-70.7076127187097,-23.4785961349091,-439.915773346617));
#36176=CARTESIAN_POINT('',(-59.0902650975996,-21.6344930467249,-462.499999999983));
#36177=CARTESIAN_POINT('Ctrl Pts',(-70.7571609664513,-20.5657726010769,
-438.999999999984));
#36178=CARTESIAN_POINT('Ctrl Pts',(-70.7509329724109,-21.0737218053046,
-439.066508123017));
#36179=CARTESIAN_POINT('Ctrl Pts',(-70.7435813995415,-21.5729826180562,
-439.178742939681));
#36180=CARTESIAN_POINT('Ctrl Pts',(-70.7268905415287,-22.5492518033819,
-439.488173552908));
#36181=CARTESIAN_POINT('Ctrl Pts',(-70.7176233372533,-23.0222061235976,
-439.68399760213));
#36182=CARTESIAN_POINT('Ctrl Pts',(-70.7076127187097,-23.4785961349081,
-439.915773346618));
#36183=CARTESIAN_POINT('Ctrl Pts',(-70.7782380423279,-15.3837579656662,
-439.937155391899));
#36184=CARTESIAN_POINT('Ctrl Pts',(-70.7802619096142,-15.8533053674025,
-439.700887922278));
#36185=CARTESIAN_POINT('Ctrl Pts',(-70.781233575539,-16.3395391453776,-439.500478619951));
#36186=CARTESIAN_POINT('Ctrl Pts',(-70.7807323681793,-17.3422849482419,
-439.18337532313));
#36187=CARTESIAN_POINT('Ctrl Pts',(-70.7792580624525,-17.8551489817955,
-439.067939400421));
#36188=CARTESIAN_POINT('Ctrl Pts',(-70.7764528366087,-18.3768010105732,
-438.999999999984));
#36189=CARTESIAN_POINT('Ctrl Pts',(-58.315252633498,-29.4505673778391,-462.499999999982));
#36190=CARTESIAN_POINT('Ctrl Pts',(-70.5582576736305,-32.0666988371032,
-439.797993805781));
#36191=CARTESIAN_POINT('Ctrl Pts',(-59.3774521833087,-26.966756235121,-462.499999999982));
#36192=CARTESIAN_POINT('Ctrl Pts',(-71.3533291948944,-29.2564718771995,
-439.789824991752));
#36193=CARTESIAN_POINT('Ctrl Pts',(-59.6440060900456,-24.2785347615233,
-462.499999999982));
#36194=CARTESIAN_POINT('Ctrl Pts',(-71.4248025866663,-26.3361222680511,
-439.789824991753));
#36195=CARTESIAN_POINT('Ctrl Pts',(-59.0902650975996,-21.634493046725,-462.499999999983));
#36196=CARTESIAN_POINT('Ctrl Pts',(-70.7678327375085,-23.4881552809602,
-439.798705096793));
#36197=CARTESIAN_POINT('',(-70.5582576736306,-32.0666988371032,-439.79799380578));
#36198=CARTESIAN_POINT('',(-58.315252633498,-29.4505673778391,-462.499999999982));
#36199=CARTESIAN_POINT('Ctrl Pts',(-70.7076127187096,-23.4785961349083,
-439.915773346619));
#36200=CARTESIAN_POINT('Ctrl Pts',(-70.692931806569,-24.1487583902344,-440.255043384189));
#36201=CARTESIAN_POINT('Ctrl Pts',(-70.6785197101522,-24.8496535886884,
-440.515026634784));
#36202=CARTESIAN_POINT('Ctrl Pts',(-70.6504156840113,-26.3070483489971,
-440.847322448924));
#36203=CARTESIAN_POINT('Ctrl Pts',(-70.6371209616,-27.0418804194973,-440.916677181194));
#36204=CARTESIAN_POINT('Ctrl Pts',(-70.6119935199245,-28.5116679207172,
-440.870550005376));
#36205=CARTESIAN_POINT('Ctrl Pts',(-70.6004358519606,-29.2285024225826,
-440.759792257379));
#36206=CARTESIAN_POINT('Ctrl Pts',(-70.5783080855848,-30.6661840163611,
-440.386490214465));
#36207=CARTESIAN_POINT('Ctrl Pts',(-70.5678992612722,-31.379554830566,-440.119180932133));
#36208=CARTESIAN_POINT('Ctrl Pts',(-70.5582576736304,-32.0666988371033,
-439.797993805781));
#36209=CARTESIAN_POINT('Ctrl Pts',(-57.8729592854352,-37.6772709400444,
-462.499999999981));
#36210=CARTESIAN_POINT('Ctrl Pts',(-71.5424551136841,-41.8116998850977,
-438.999999999981));
#36211=CARTESIAN_POINT('Ctrl Pts',(-57.002852784825,-34.8311127040267,-462.499999999982));
#36212=CARTESIAN_POINT('Ctrl Pts',(-70.2444010733898,-38.6079211063178,
-439.000759209165));
#36213=CARTESIAN_POINT('Ctrl Pts',(-57.2363227433805,-31.9735001768253,
-462.499999999982));
#36214=CARTESIAN_POINT('Ctrl Pts',(-70.1269516413443,-35.2651683193791,
-438.998997400818));
#36215=CARTESIAN_POINT('Ctrl Pts',(-58.315252633498,-29.4505673778391,-462.499999999982));
#36216=CARTESIAN_POINT('Ctrl Pts',(-70.9881812819792,-32.1585665340612,
-439.000793413576));
#36217=CARTESIAN_POINT('Ctrl Pts',(-70.4554509568026,-36.7924115993857,
-438.999999999982));
#36218=CARTESIAN_POINT('Ctrl Pts',(-70.4314005258243,-37.6085426071128,
-439.105374792254));
#36219=CARTESIAN_POINT('Ctrl Pts',(-70.404873950049,-38.395408212837,-439.336981328181));
#36220=CARTESIAN_POINT('Ctrl Pts',(-70.3483212379187,-39.8946310210821,
-440.024425265895));
#36221=CARTESIAN_POINT('Ctrl Pts',(-70.3188922841445,-40.590758615142,-440.473747059951));
#36222=CARTESIAN_POINT('Ctrl Pts',(-70.2893406183184,-41.2283906081489,
-441.000029123694));
#36223=CARTESIAN_POINT('Ctrl Pts',(-70.5582576736304,-32.0666988371036,
-439.797993805781));
#36224=CARTESIAN_POINT('Ctrl Pts',(-70.5522778094327,-32.4932382706619,
-439.598328470635));
#36225=CARTESIAN_POINT('Ctrl Pts',(-70.5451955315253,-32.9328963563196,
-439.428497688943));
#36226=CARTESIAN_POINT('Ctrl Pts',(-70.5286110764291,-33.8355932537874,
-439.1586274275));
#36227=CARTESIAN_POINT('Ctrl Pts',(-70.519152260206,-34.2961448342265,-439.059408910764));
#36228=CARTESIAN_POINT('Ctrl Pts',(-70.5084762417147,-34.7635952579922,
-438.999999999982));
#36229=CARTESIAN_POINT('Origin',(-1.50000000000897,104.331,-355.5));
#36230=CARTESIAN_POINT('',(-51.000000000009,104.330999999988,-407.5));
#36231=CARTESIAN_POINT('',(47.999999999991,104.330999999997,-407.5));
#36232=CARTESIAN_POINT('',(-1.500000000009,104.330999999993,-407.5));
#36233=CARTESIAN_POINT('',(-55.000000000009,104.330999999989,-403.5));
#36234=CARTESIAN_POINT('Origin',(-51.000000000009,104.330999999989,-403.5));
#36235=CARTESIAN_POINT('',(-55.000000000009,104.331,-307.5));
#36236=CARTESIAN_POINT('',(-55.000000000009,104.330999999994,-355.5));
#36237=CARTESIAN_POINT('',(-51.000000000009,104.331,-303.5));
#36238=CARTESIAN_POINT('Origin',(-51.000000000009,104.331,-307.5));
#36239=CARTESIAN_POINT('',(47.999999999991,104.331000000009,-303.5));
#36240=CARTESIAN_POINT('',(-25.500000000009,104.331000000003,-303.5));
#36241=CARTESIAN_POINT('',(51.999999999991,104.331000000009,-307.5));
#36242=CARTESIAN_POINT('Origin',(47.999999999991,104.331000000009,-307.5));
#36243=CARTESIAN_POINT('',(51.999999999991,104.330999999998,-403.5));
#36244=CARTESIAN_POINT('',(51.999999999991,104.331000000003,-355.5));
#36245=CARTESIAN_POINT('Origin',(47.999999999991,104.330999999998,-403.5));
#36246=CARTESIAN_POINT('Origin',(-47.7278656583192,-53.3599981836911,-427.99999999998));
#36247=CARTESIAN_POINT('',(-70.0043915535533,-54.382950086646,-427.999999999977));
#36248=CARTESIAN_POINT('',(-64.4357425873311,-68.1294560302671,-427.999999999978));
#36249=CARTESIAN_POINT('Origin',(-47.7278656583192,-53.3599981836911,-427.99999999998));
#36250=CARTESIAN_POINT('',(-70.004392491464,-54.3829501297155,-427.999946210488));
#36251=CARTESIAN_POINT('',(-64.4357419744368,-68.1294554884797,-428.000046864887));
#36252=CARTESIAN_POINT('Origin',(-0.00177950443039366,-11.1710102813481,
-427.999999999985));
#36253=CARTESIAN_POINT('',(-56.9487785810004,-75.6150902024262,-427.999999999977));
#36254=CARTESIAN_POINT('Origin',(-0.00177950443039366,-11.1710102813481,
-427.999999999985));
#36255=CARTESIAN_POINT('',(-56.9487778856762,-75.6150894155625,-428.000060157994));
#36256=CARTESIAN_POINT('Origin',(-42.1822887306986,-58.9045897810235,-427.99999999998));
#36257=CARTESIAN_POINT('',(-43.2050881469284,-81.1811229086658,-427.999999999976));
#36258=CARTESIAN_POINT('Origin',(-42.1822887306986,-58.9045897810235,-427.99999999998));
#36259=CARTESIAN_POINT('',(-43.2050880985635,-81.1811218552779,-428.0000604121));
#36260=CARTESIAN_POINT('Origin',(0.000158749880824205,859.827542634463,
-428.000000000085));
#36261=CARTESIAN_POINT('',(43.2079320035479,-81.1810069107222,-427.999999999977));
#36262=CARTESIAN_POINT('',(43.207931941457,-81.1810055584643,-428.000077552408));
#36263=CARTESIAN_POINT('Origin',(0.000158749880824205,859.827542634463,
-428.000000000083));
#36264=CARTESIAN_POINT('Origin',(42.1850727668518,-58.9044762258028,-427.999999999981));
#36265=CARTESIAN_POINT('',(56.9519860533863,-75.6146028669214,-427.999999999979));
#36266=CARTESIAN_POINT('Origin',(42.1850727668518,-58.9044762258028,-427.999999999981));
#36267=CARTESIAN_POINT('',(56.9519851501412,-75.614601844816,-428.000078144642));
#36268=CARTESIAN_POINT('Origin',(0.00335440791734976,-11.1719648985687,
-427.999999999985));
#36269=CARTESIAN_POINT('',(64.4405276263421,-68.1267798155728,-427.99999999998));
#36270=CARTESIAN_POINT('Origin',(0.00335440791734976,-11.1719648985687,
-427.999999999984));
#36271=CARTESIAN_POINT('',(64.4405263142287,-68.1267786558203,-428.000100325606));
#36272=CARTESIAN_POINT('Origin',(47.7318177098118,-53.3582629290221,-427.999999999981));
#36273=CARTESIAN_POINT('Origin',(47.7318177098118,-53.3582629290221,-427.999999999981));
#36274=CARTESIAN_POINT('Origin',(47.7318177098045,31.0202629290117,-427.999999999991));
#36275=CARTESIAN_POINT('',(64.4405276263324,45.7887798155652,-427.999999999993));
#36276=CARTESIAN_POINT('Origin',(47.7318177098045,31.0202629290117,-427.999999999991));
#36277=CARTESIAN_POINT('',(64.4405266043137,45.788778912222,-428.000078144656));
#36278=CARTESIAN_POINT('Origin',(0.00335440791743302,-11.16603510145,-427.999999999987));
#36279=CARTESIAN_POINT('',(56.7520934677589,53.4526994089804,-427.999999999993));
#36280=CARTESIAN_POINT('Origin',(0.00335440791743302,-11.16603510145,-427.999999999986));
#36281=CARTESIAN_POINT('',(56.7520925748523,53.4526983922443,-428.00007752232));
#36282=CARTESIAN_POINT('Origin',(35.1083877883366,28.8074139931111,-427.99999999999));
#36283=CARTESIAN_POINT('',(41.9923368054846,60.8737188148991,-427.999999331678));
#36284=CARTESIAN_POINT('Origin',(35.1083877883366,28.8074139931111,-427.99999999999));
#36285=CARTESIAN_POINT('Ctrl Pts',(41.9923369765522,60.8737187517663,-427.999999331209));
#36286=CARTESIAN_POINT('Ctrl Pts',(41.9758064463718,60.7967417673027,-432.332897601345));
#36287=CARTESIAN_POINT('Ctrl Pts',(41.9599261581031,60.7227955022272,-436.665849967173));
#36288=CARTESIAN_POINT('Ctrl Pts',(41.9454903641296,60.6521460670534,-440.99653250072));
#36289=CARTESIAN_POINT('Origin',(-0.0017653923509997,-134.670997806537,
-427.999999999971));
#36290=CARTESIAN_POINT('',(-41.9939391803561,60.8709610296021,-427.999999999994));
#36291=CARTESIAN_POINT('',(-41.9939390098067,60.870960235417,-428.000046536129));
#36292=CARTESIAN_POINT('Origin',(-0.0017653923509997,-134.670997806537,
-427.999999999972));
#36293=CARTESIAN_POINT('Origin',(-35.107222536544,28.8020791165365,-427.999999999989));
#36294=CARTESIAN_POINT('',(-56.7511891313755,53.4471346719238,-427.999999999992));
#36295=CARTESIAN_POINT('Origin',(-35.107222536544,28.8020791165365,-427.999999999989));
#36296=CARTESIAN_POINT('',(-56.7511885953632,53.4471340615896,-428.000046536128));
#36297=CARTESIAN_POINT('Origin',(-0.00176539236174112,-11.1709978065374,
-427.999999999985));
#36298=CARTESIAN_POINT('',(-64.435714908143,45.7874632814507,-427.999999999991));
#36299=CARTESIAN_POINT('Origin',(-0.00176539236174112,-11.1709978065374,
-427.999999999985));
#36300=CARTESIAN_POINT('',(-64.435714908143,45.7874632814507,-427.999999999991));
#36301=CARTESIAN_POINT('Origin',(-47.7278415015221,31.0180014613125,-427.99999999999));
#36302=CARTESIAN_POINT('',(-70.004366803487,32.0409661230246,-427.999999999987));
#36303=CARTESIAN_POINT('Origin',(-47.7278415015221,31.0180014613125,-427.99999999999));
#36304=CARTESIAN_POINT('',(-70.0043677413975,32.0409661660946,-427.999946210498));
#36305=CARTESIAN_POINT('Origin',(871.003976208289,-11.1712614676237,-427.99999999999));
#36306=CARTESIAN_POINT('Origin',(871.003976208289,-11.1712614676237,-427.99999999999));
#36307=CARTESIAN_POINT('Origin',(-25.500000000006,70.3310000000027,-303.499999999994));
#36308=CARTESIAN_POINT('',(47.9999999999939,71.3310000000091,-303.499999999995));
#36309=CARTESIAN_POINT('',(47.999999999994,70.3310000000091,-303.499999999994));
#36310=CARTESIAN_POINT('',(-51.0000000000061,71.331,-303.499999999995));
#36311=CARTESIAN_POINT('',(-51.000000000006,70.331,-303.499999999994));
#36312=CARTESIAN_POINT('',(-55.0000000000061,71.331,-303.499999999995));
#36313=CARTESIAN_POINT('Origin',(51.999999999994,70.3310000000035,-355.499999999994));
#36314=CARTESIAN_POINT('',(51.9999999999939,71.330999999998,-403.499999999995));
#36315=CARTESIAN_POINT('',(51.999999999994,70.330999999998,-403.499999999995));
#36316=CARTESIAN_POINT('',(51.9999999999939,71.331000000009,-307.499999999995));
#36317=CARTESIAN_POINT('',(51.999999999994,70.331000000009,-307.499999999994));
#36318=CARTESIAN_POINT('',(51.9999999999939,71.3309999999976,-407.499999999995));
#36319=CARTESIAN_POINT('Origin',(47.999999999994,70.3310000000087,-307.499999999994));
#36320=CARTESIAN_POINT('',(50.6457513110586,70.3310000000093,-304.499999999994));
#36321=CARTESIAN_POINT('Ctrl Pts',(50.6457513110591,70.3310000000092,-304.499999999995));
#36322=CARTESIAN_POINT('Ctrl Pts',(50.3169215545075,70.3310000000094,-304.20999941349));
#36323=CARTESIAN_POINT('Ctrl Pts',(49.8828383607448,70.4697262929124,-303.947060144719));
#36324=CARTESIAN_POINT('Ctrl Pts',(49.0403497074305,70.8111780179431,-303.605608419688));
#36325=CARTESIAN_POINT('Ctrl Pts',(48.4763938626813,71.0928030686654,-303.499999999995));
#36326=CARTESIAN_POINT('Ctrl Pts',(47.9999999999939,71.3310000000091,-303.499999999995));
#36327=CARTESIAN_POINT('',(50.9999999999939,70.3310000000092,-304.85424868893));
#36328=CARTESIAN_POINT('Origin',(47.999999999994,70.3310000000087,-307.499999999994));
#36329=CARTESIAN_POINT('Ctrl Pts',(51.9999999999939,71.331000000009,-307.499999999995));
#36330=CARTESIAN_POINT('Ctrl Pts',(51.9999999999939,71.0928030686655,-307.023606137307));
#36331=CARTESIAN_POINT('Ctrl Pts',(51.8943915803007,70.8111780179428,-306.459650292559));
#36332=CARTESIAN_POINT('Ctrl Pts',(51.5529398552703,70.4697262929124,-305.617161639245));
#36333=CARTESIAN_POINT('Ctrl Pts',(51.2900005864986,70.3310000000092,-305.183078445482));
#36334=CARTESIAN_POINT('Ctrl Pts',(50.999999999994,70.3310000000092,-304.85424868893));
#36335=CARTESIAN_POINT('Origin',(-1.50000000000603,70.3309999999929,-407.499999999995));
#36336=CARTESIAN_POINT('',(-51.0000000000061,71.3309999999886,-407.499999999995));
#36337=CARTESIAN_POINT('',(-51.000000000006,70.3309999999886,-407.499999999995));
#36338=CARTESIAN_POINT('',(47.9999999999939,71.3309999999972,-407.499999999995));
#36339=CARTESIAN_POINT('',(47.999999999994,70.3309999999972,-407.499999999995));
#36340=CARTESIAN_POINT('',(-55.0000000000061,71.3309999999882,-407.499999999995));
#36341=CARTESIAN_POINT('Origin',(47.999999999994,70.3309999999976,-403.499999999995));
#36342=CARTESIAN_POINT('',(50.9999999999939,70.3309999999976,-406.145751311059));
#36343=CARTESIAN_POINT('Ctrl Pts',(50.999999999994,70.3309999999976,-406.145751311059));
#36344=CARTESIAN_POINT('Ctrl Pts',(51.2900005864986,70.3309999999975,-405.816921554508));
#36345=CARTESIAN_POINT('Ctrl Pts',(51.5529398552703,70.4697262929009,-405.382838360744));
#36346=CARTESIAN_POINT('Ctrl Pts',(51.8943915803007,70.8111780179315,-404.54034970743));
#36347=CARTESIAN_POINT('Ctrl Pts',(51.9999999999939,71.0928030686541,-403.976393862682));
#36348=CARTESIAN_POINT('Ctrl Pts',(51.9999999999939,71.3309999999978,-403.499999999995));
#36349=CARTESIAN_POINT('',(50.6457513110586,70.3309999999976,-406.499999999995));
#36350=CARTESIAN_POINT('Origin',(47.999999999994,70.3309999999976,-403.499999999995));
#36351=CARTESIAN_POINT('Ctrl Pts',(47.9999999999939,71.3309999999972,-407.499999999995));
#36352=CARTESIAN_POINT('Ctrl Pts',(48.4763938626809,71.0928030686538,-407.499999999995));
#36353=CARTESIAN_POINT('Ctrl Pts',(49.0403497074289,70.8111780179308,-407.394391580302));
#36354=CARTESIAN_POINT('Ctrl Pts',(49.8828383607432,70.4697262929006,-407.052939855271));
#36355=CARTESIAN_POINT('Ctrl Pts',(50.3169215545064,70.3309999999975,-406.790000586499));
#36356=CARTESIAN_POINT('Ctrl Pts',(50.6457513110582,70.3309999999975,-406.499999999995));
#36357=CARTESIAN_POINT('Origin',(-51.000000000006,70.330999999989,-403.499999999995));
#36358=CARTESIAN_POINT('',(-53.6457513110706,70.3309999999884,-406.499999999995));
#36359=CARTESIAN_POINT('Ctrl Pts',(-53.6457513110702,70.3309999999884,-406.499999999995));
#36360=CARTESIAN_POINT('Ctrl Pts',(-53.271654714955,70.3309999999883,-406.82992218654));
#36361=CARTESIAN_POINT('Ctrl Pts',(-52.8397473959416,70.480582189106,-407.085008016199));
#36362=CARTESIAN_POINT('Ctrl Pts',(-51.9262909192953,70.8660628162156,-407.421591216636));
#36363=CARTESIAN_POINT('Ctrl Pts',(-51.4461362235074,71.1079318882378,-407.499999999995));
#36364=CARTESIAN_POINT('Ctrl Pts',(-51.0000000000061,71.3309999999885,-407.499999999995));
#36365=CARTESIAN_POINT('',(-54.0000000000059,70.3309999999884,-406.145751311059));
#36366=CARTESIAN_POINT('Origin',(-51.000000000006,70.330999999989,-403.499999999995));
#36367=CARTESIAN_POINT('',(-55.0000000000061,71.3309999999887,-403.499999999995));
#36368=CARTESIAN_POINT('Ctrl Pts',(-55.0000000000061,71.3309999999885,-403.499999999995));
#36369=CARTESIAN_POINT('Ctrl Pts',(-55.000000000006,71.092803068645,-403.976393862682));
#36370=CARTESIAN_POINT('Ctrl Pts',(-54.8943915803128,70.8111780179222,-404.54034970743));
#36371=CARTESIAN_POINT('Ctrl Pts',(-54.5529398552823,70.4697262928917,-405.382838360744));
#36372=CARTESIAN_POINT('Ctrl Pts',(-54.2900005865106,70.3309999999885,-405.816921554507));
#36373=CARTESIAN_POINT('Ctrl Pts',(-54.000000000006,70.3309999999885,-406.145751311059));
#36374=CARTESIAN_POINT('',(-55.000000000006,70.3309999999887,-403.499999999995));
#36375=CARTESIAN_POINT('Origin',(-51.000000000006,70.331,-307.499999999994));
#36376=CARTESIAN_POINT('',(-55.0000000000061,71.331,-307.499999999995));
#36377=CARTESIAN_POINT('',(-55.000000000006,70.331,-307.499999999994));
#36378=CARTESIAN_POINT('',(-54.0000000000059,70.331,-304.85424868893));
#36379=CARTESIAN_POINT('Ctrl Pts',(-54.000000000006,70.3310000000001,-304.85424868893));
#36380=CARTESIAN_POINT('Ctrl Pts',(-54.2900005865106,70.3310000000001,-305.183078445482));
#36381=CARTESIAN_POINT('Ctrl Pts',(-54.5529398552823,70.4697262929032,-305.617161639245));
#36382=CARTESIAN_POINT('Ctrl Pts',(-54.8943915803128,70.8111780179335,-306.459650292559));
#36383=CARTESIAN_POINT('Ctrl Pts',(-55.0000000000061,71.0928030686562,-307.023606137307));
#36384=CARTESIAN_POINT('Ctrl Pts',(-55.0000000000061,71.3309999999997,-307.499999999995));
#36385=CARTESIAN_POINT('',(-53.6457513110706,70.331,-304.499999999994));
#36386=CARTESIAN_POINT('Origin',(-51.000000000006,70.331,-307.499999999994));
#36387=CARTESIAN_POINT('Ctrl Pts',(-51.0000000000063,71.3310000000004,-303.499999999995));
#36388=CARTESIAN_POINT('Ctrl Pts',(-51.4461362235077,71.1079318882496,-303.499999999995));
#36389=CARTESIAN_POINT('Ctrl Pts',(-51.9262909192962,70.8660628162283,-303.578408783354));
#36390=CARTESIAN_POINT('Ctrl Pts',(-52.8397473959424,70.480582189118,-303.91499198379));
#36391=CARTESIAN_POINT('Ctrl Pts',(-53.2716547149558,70.3310000000002,-304.170077813449));
#36392=CARTESIAN_POINT('Ctrl Pts',(-53.6457513110711,70.3310000000001,-304.499999999995));
#36393=CARTESIAN_POINT('Origin',(-55.000000000006,70.3309999999942,-355.499999999994));
#36394=CARTESIAN_POINT('',(-55.0000000000061,71.3309999999882,-407.499999999995));
#36395=CARTESIAN_POINT('Ctrl Pts',(-71.7242220719942,-61.2914501133864,
-419.974938351021));
#36396=CARTESIAN_POINT('Ctrl Pts',(-71.723675161943,-61.2913712681343,-419.984638846289));
#36397=CARTESIAN_POINT('Ctrl Pts',(-71.2717722995097,-61.2262227212994,
-427.999999999979));
#36398=CARTESIAN_POINT('Ctrl Pts',(-71.2712259684214,-61.2261439595135,
-428.009690226232));
#36399=CARTESIAN_POINT('Ctrl Pts',(-71.7242858769396,-61.2947293352783,
-419.974938351021));
#36400=CARTESIAN_POINT('Ctrl Pts',(-71.7237373707235,-61.2946510609304,
-419.984638846289));
#36401=CARTESIAN_POINT('Ctrl Pts',(-71.2705156232134,-61.2299742429629,
-427.999999999979));
#36402=CARTESIAN_POINT('Ctrl Pts',(-71.26996769765,-61.2298960514769,-428.009690226232));
#36403=CARTESIAN_POINT('Ctrl Pts',(-71.724349681885,-61.2980085571703,-419.974938351021));
#36404=CARTESIAN_POINT('Ctrl Pts',(-71.723799579504,-61.2979308537266,-419.984638846289));
#36405=CARTESIAN_POINT('Ctrl Pts',(-71.2692589469172,-61.2337257646263,
-427.999999999979));
#36406=CARTESIAN_POINT('Ctrl Pts',(-71.2687094268786,-61.2336481434402,
-428.009690226232));
#36407=CARTESIAN_POINT('Ctrl Pts',(-71.7244134868304,-61.3012877790621,
-419.974938351021));
#36408=CARTESIAN_POINT('Ctrl Pts',(-71.7238617882844,-61.3012106465228,
-419.984638846289));
#36409=CARTESIAN_POINT('Ctrl Pts',(-71.2680022706209,-61.2374772862898,
-427.999999999979));
#36410=CARTESIAN_POINT('Ctrl Pts',(-71.267451156107,-61.2374002354035,-428.009690226232));
#36411=CARTESIAN_POINT('Ctrl Pts',(-71.7523909953645,-62.7391772385893,
-419.974938351021));
#36412=CARTESIAN_POINT('Ctrl Pts',(-71.7511394025092,-62.739350438968,-419.984638846289));
#36413=CARTESIAN_POINT('Ctrl Pts',(-70.7169686230121,-62.8824630892737,
-427.999999999979));
#36414=CARTESIAN_POINT('Ctrl Pts',(-70.715718355102,-62.8826361063013,-428.009690226232));
#36415=CARTESIAN_POINT('Ctrl Pts',(-71.7706749200703,-64.1748827234151,
-419.97493835102));
#36416=CARTESIAN_POINT('Ctrl Pts',(-71.7685254439165,-64.175261649583,-419.984638846288));
#36417=CARTESIAN_POINT('Ctrl Pts',(-69.9924483273783,-64.4883621667485,
-427.999999999978));
#36418=CARTESIAN_POINT('Ctrl Pts',(-69.9903011266753,-64.4887406917823,
-428.009690226232));
#36419=CARTESIAN_POINT('Ctrl Pts',(-71.7897768306913,-67.0361903512381,
-419.97493835102));
#36420=CARTESIAN_POINT('Ctrl Pts',(-71.7854748505741,-67.0367743707917,
-419.984638846288));
#36421=CARTESIAN_POINT('Ctrl Pts',(-68.2308187876847,-67.5193402102946,
-427.999999999978));
#36422=CARTESIAN_POINT('Ctrl Pts',(-68.2265213616744,-67.5199236116008,
-428.009690226232));
#36423=CARTESIAN_POINT('Ctrl Pts',(-71.7906156729946,-68.4617566097018,
-419.974938351019));
#36424=CARTESIAN_POINT('Ctrl Pts',(-71.7850594981988,-68.4623392639196,
-419.984638846288));
#36425=CARTESIAN_POINT('Ctrl Pts',(-67.1940828116454,-68.9437769487302,
-427.999999999977));
#36426=CARTESIAN_POINT('Ctrl Pts',(-67.188532518656,-68.9443589861462,-428.009690226231));
#36427=CARTESIAN_POINT('Ctrl Pts',(-71.7847586494582,-69.8799811589918,
-419.974938351019));
#36428=CARTESIAN_POINT('Ctrl Pts',(-71.7778115186237,-69.8804124953274,
-419.984638846288));
#36429=CARTESIAN_POINT('Ctrl Pts',(-66.0375105252458,-70.2368186801329,
-427.999999999977));
#36430=CARTESIAN_POINT('Ctrl Pts',(-66.0305707486938,-70.2372495598528,
-428.009690226231));
#36431=CARTESIAN_POINT('Ctrl Pts',(-71.7847466560944,-69.8828852420776,
-419.974938351019));
#36432=CARTESIAN_POINT('Ctrl Pts',(-71.7777966770143,-69.8833162685612,
-419.984638846288));
#36433=CARTESIAN_POINT('Ctrl Pts',(-66.0351422246716,-70.239466427715,-427.999999999977));
#36434=CARTESIAN_POINT('Ctrl Pts',(-66.0281996028891,-70.239896997911,-428.009690226231));
#36435=CARTESIAN_POINT('Ctrl Pts',(-71.7847346627306,-69.8857893251633,
-419.974938351019));
#36436=CARTESIAN_POINT('Ctrl Pts',(-71.7777818354048,-69.8862200417949,
-419.984638846288));
#36437=CARTESIAN_POINT('Ctrl Pts',(-66.0327739240975,-70.2421141752972,
-427.999999999977));
#36438=CARTESIAN_POINT('Ctrl Pts',(-66.0258284570844,-70.2425444359691,
-428.009690226231));
#36439=CARTESIAN_POINT('Ctrl Pts',(-71.7847226693668,-69.8886934082491,
-419.974938351019));
#36440=CARTESIAN_POINT('Ctrl Pts',(-71.7777669937953,-69.8891238150288,
-419.984638846288));
#36441=CARTESIAN_POINT('Ctrl Pts',(-66.0304056235233,-70.2447619228793,
-427.999999999977));
#36442=CARTESIAN_POINT('Ctrl Pts',(-66.0234573112798,-70.2451918740273,
-428.009690226231));
#36443=CARTESIAN_POINT('',(-66.0375105251866,-70.2368186801118,-427.999999999978));
#36444=CARTESIAN_POINT('',(-71.2680022706209,-61.2374772862897,-427.999999999979));
#36445=CARTESIAN_POINT('Ctrl Pts',(-66.0375105251866,-70.2368186801118,
-427.999999999978));
#36446=CARTESIAN_POINT('Ctrl Pts',(-67.1940828116442,-68.9437769487396,
-427.999999999967));
#36447=CARTESIAN_POINT('Ctrl Pts',(-68.2308187876832,-67.5193402103046,
-427.999999999967));
#36448=CARTESIAN_POINT('Ctrl Pts',(-69.9924483273808,-64.4883621667479,
-427.999999999967));
#36449=CARTESIAN_POINT('Ctrl Pts',(-70.7169686230136,-62.8824630892733,
-427.999999999968));
#36450=CARTESIAN_POINT('Ctrl Pts',(-71.2680022706209,-61.2374772862897,
-427.999999999979));
#36451=CARTESIAN_POINT('',(-71.6057458572746,-69.8910957793807,-420.224899491137));
#36452=CARTESIAN_POINT('',(-68.8215314165109,-70.063963238333,-424.112584875117));
#36453=CARTESIAN_POINT('',(-71.7785821060117,-69.7241904101603,-419.984638846415));
#36454=CARTESIAN_POINT('Origin',(-64.4008420418883,-77.3577815801559,-409.614647544567));
#36455=CARTESIAN_POINT('Ctrl Pts',(-71.268002270621,-61.2374772862896,-427.999999999978));
#36456=CARTESIAN_POINT('Ctrl Pts',(-71.2899303949503,-61.3466114274369,
-427.017655373544));
#36457=CARTESIAN_POINT('Ctrl Pts',(-71.3115444253862,-61.4774240219384,
-426.107461484164));
#36458=CARTESIAN_POINT('Ctrl Pts',(-71.3561812057394,-61.8206184542583,
-424.410282741723));
#36459=CARTESIAN_POINT('Ctrl Pts',(-71.3784339270585,-62.0406036470746,
-423.68637123802));
#36460=CARTESIAN_POINT('Ctrl Pts',(-71.4224149843577,-62.5795974842737,
-422.516016605151));
#36461=CARTESIAN_POINT('Ctrl Pts',(-71.4446474358491,-62.9048724301656,
-422.056379398897));
#36462=CARTESIAN_POINT('Ctrl Pts',(-71.4929560658814,-63.7151444243507,
-421.316245633231));
#36463=CARTESIAN_POINT('Ctrl Pts',(-71.5196071135653,-64.2098545996343,
-421.027118835742));
#36464=CARTESIAN_POINT('Ctrl Pts',(-71.605083940526,-65.9138105320977,-420.392921361503));
#36465=CARTESIAN_POINT('Ctrl Pts',(-71.6736227710617,-67.391175606321,-420.161937548972));
#36466=CARTESIAN_POINT('Ctrl Pts',(-71.7697681700019,-69.5279869464756,
-419.998805056281));
#36467=CARTESIAN_POINT('Ctrl Pts',(-71.774178781962,-69.6261206245261,-419.991593225368));
#36468=CARTESIAN_POINT('Ctrl Pts',(-71.7785821060559,-69.7241904101554,
-419.984638846373));
#36469=CARTESIAN_POINT('Ctrl Pts',(-71.6135253144154,-69.8855065275808,
-420.221597501086));
#36470=CARTESIAN_POINT('Ctrl Pts',(-71.6111594298038,-69.8856543483064,
-420.224899490927));
#36471=CARTESIAN_POINT('Ctrl Pts',(-66.0402789827285,-70.2337235592324,
-427.999999999977));
#36472=CARTESIAN_POINT('Ctrl Pts',(-66.0377194565801,-70.2338834787021,
-428.003572249148));
#36473=CARTESIAN_POINT('Ctrl Pts',(-71.6117204158214,-69.887320670077,-420.221597501086));
#36474=CARTESIAN_POINT('Ctrl Pts',(-71.6093549056591,-69.887468158653,-420.224899490927));
#36475=CARTESIAN_POINT('Ctrl Pts',(-66.0393561635675,-70.2347552661992,
-427.999999999977));
#36476=CARTESIAN_POINT('Ctrl Pts',(-66.0367970425162,-70.2349148263336,
-428.003572249148));
#36477=CARTESIAN_POINT('Ctrl Pts',(-71.6099155172274,-69.8891348125733,
-420.221597501086));
#36478=CARTESIAN_POINT('Ctrl Pts',(-71.6075503815144,-69.8892819689994,
-420.224899490927));
#36479=CARTESIAN_POINT('Ctrl Pts',(-66.0384333444067,-70.235786973166,-427.999999999977));
#36480=CARTESIAN_POINT('Ctrl Pts',(-66.0358746284523,-70.2359461739651,
-428.003572249148));
#36481=CARTESIAN_POINT('Ctrl Pts',(-71.6081106186334,-69.8909489550694,
-420.221597501086));
#36482=CARTESIAN_POINT('Ctrl Pts',(-71.6057458573697,-69.8910957793458,
-420.224899490927));
#36483=CARTESIAN_POINT('Ctrl Pts',(-66.0375105252458,-70.2368186801329,
-427.999999999977));
#36484=CARTESIAN_POINT('Ctrl Pts',(-66.0349522143885,-70.2369775215966,
-428.003572249148));
#36485=CARTESIAN_POINT('Ctrl Pts',(-69.4660550218801,-72.0439752249162,
-420.221597501086));
#36486=CARTESIAN_POINT('Ctrl Pts',(-69.4641346574427,-72.0437278535533,
-420.224899490927));
#36487=CARTESIAN_POINT('Ctrl Pts',(-64.9423077504781,-71.4612496203996,
-427.999999999977));
#36488=CARTESIAN_POINT('Ctrl Pts',(-64.940230209178,-71.4609820023305,-428.003572249148));
#36489=CARTESIAN_POINT('Ctrl Pts',(-67.3210277409069,-74.1944878424358,
-420.221597501085));
#36490=CARTESIAN_POINT('Ctrl Pts',(-67.3195381750349,-74.1938347731011,
-420.224899490927));
#36491=CARTESIAN_POINT('Ctrl Pts',(-63.8121002593275,-72.6560711942995,
-427.999999999977));
#36492=CARTESIAN_POINT('Ctrl Pts',(-63.8104887763412,-72.6553646729287,
-428.003572249148));
#36493=CARTESIAN_POINT('Ctrl Pts',(-63.0254878424137,-78.4900277409281,
-420.221597501084));
#36494=CARTESIAN_POINT('Ctrl Pts',(-63.0248347730789,-78.4885381750561,
-420.224899490927));
#36495=CARTESIAN_POINT('Ctrl Pts',(-61.4870711942769,-74.9811002593497,
-427.999999999977));
#36496=CARTESIAN_POINT('Ctrl Pts',(-61.4863646729061,-74.9794887763634,
-428.003572249148));
#36497=CARTESIAN_POINT('Ctrl Pts',(-60.8749752248937,-80.6350550219009,
-420.221597501084));
#36498=CARTESIAN_POINT('Ctrl Pts',(-60.8747278535309,-80.6331346574634,
-420.224899490927));
#36499=CARTESIAN_POINT('Ctrl Pts',(-60.2922496203767,-76.1113077505,-427.999999999977));
#36500=CARTESIAN_POINT('Ctrl Pts',(-60.2919820023077,-76.1092302091999,
-428.003572249148));
#36501=CARTESIAN_POINT('Ctrl Pts',(-58.7219489550468,-82.7771106186537,
-420.221597501084));
#36502=CARTESIAN_POINT('Ctrl Pts',(-58.7220957793232,-82.7747458573899,
-420.224899490926));
#36503=CARTESIAN_POINT('Ctrl Pts',(-59.0678186801098,-77.2065105252675,
-427.999999999977));
#36504=CARTESIAN_POINT('Ctrl Pts',(-59.0679775215736,-77.2039522144101,
-428.003572249148));
#36505=CARTESIAN_POINT('Ctrl Pts',(-58.7201348125564,-82.7789155172418,
-420.221597501084));
#36506=CARTESIAN_POINT('Ctrl Pts',(-58.7202819689826,-82.7765503815288,
-420.224899490926));
#36507=CARTESIAN_POINT('Ctrl Pts',(-59.0667869731464,-77.2074333444253,
-427.999999999977));
#36508=CARTESIAN_POINT('Ctrl Pts',(-59.0669461739455,-77.2048746284709,
-428.003572249148));
#36509=CARTESIAN_POINT('Ctrl Pts',(-58.7183206700661,-82.78072041583,-420.221597501084));
#36510=CARTESIAN_POINT('Ctrl Pts',(-58.718468158642,-82.7783549056677,-420.224899490926));
#36511=CARTESIAN_POINT('Ctrl Pts',(-59.0657552661828,-77.2083561635832,
-427.999999999977));
#36512=CARTESIAN_POINT('Ctrl Pts',(-59.0659148263172,-77.2057970425319,
-428.003572249148));
#36513=CARTESIAN_POINT('Ctrl Pts',(-58.7165065275757,-82.7825253144182,
-420.221597501084));
#36514=CARTESIAN_POINT('Ctrl Pts',(-58.7166543483013,-82.7801594298066,
-420.224899490926));
#36515=CARTESIAN_POINT('Ctrl Pts',(-59.0647235592194,-77.2092789827411,
-427.999999999977));
#36516=CARTESIAN_POINT('Ctrl Pts',(-59.0648834786889,-77.2067194565927,
-428.003572249148));
#36517=CARTESIAN_POINT('',(-59.0678186801297,-77.2065105251389,-427.999999999977));
#36518=CARTESIAN_POINT('Origin',(-31.3096336212146,-42.4786335233977,-427.999999993621));
#36519=CARTESIAN_POINT('',(-58.722095779334,-82.7747458573179,-420.224899491172));
#36520=CARTESIAN_POINT('',(-58.8896152555255,-80.0766663721036,-423.992311952553));
#36521=CARTESIAN_POINT('Ctrl Pts',(-71.6057458572757,-69.8910957793828,
-420.224899491013));
#36522=CARTESIAN_POINT('Ctrl Pts',(-71.5787972094958,-69.918039166144,-420.225112615511));
#36523=CARTESIAN_POINT('Ctrl Pts',(-71.3433559394484,-70.1534350994587,
-420.226949212009));
#36524=CARTESIAN_POINT('Ctrl Pts',(-71.0675267617563,-70.4292133340037,
-420.229012925027));
#36525=CARTESIAN_POINT('Ctrl Pts',(-70.9330282538967,-70.5636877197912,
-420.229990113068));
#36526=CARTESIAN_POINT('Ctrl Pts',(-70.5296622518239,-70.9669835947287,
-420.232830971758));
#36527=CARTESIAN_POINT('Ctrl Pts',(-70.2608984858126,-71.2357035867425,
-420.23460426166));
#36528=CARTESIAN_POINT('Ctrl Pts',(-69.4547425198419,-72.0417375568549,
-420.239546328562));
#36529=CARTESIAN_POINT('Ctrl Pts',(-68.9182881782136,-72.5781231052261,
-420.242333151682));
#36530=CARTESIAN_POINT('Ctrl Pts',(-67.305913743286,-74.1903309310481,-420.249082506593));
#36531=CARTESIAN_POINT('Ctrl Pts',(-66.238637509614,-75.2575503716149,-420.25138320211));
#36532=CARTESIAN_POINT('Ctrl Pts',(-64.088541529322,-77.4076463522807,-420.251383186951));
#36533=CARTESIAN_POINT('Ctrl Pts',(-63.021323830494,-78.4749208443966,-420.249082484014));
#36534=CARTESIAN_POINT('Ctrl Pts',(-61.4091186736197,-80.0872926103647,
-420.242333129556));
#36535=CARTESIAN_POINT('Ctrl Pts',(-60.8727340074292,-80.6237460697621,
-420.239546308457));
#36536=CARTESIAN_POINT('Ctrl Pts',(-60.0667013675136,-81.429900705396,-420.234604247222));
#36537=CARTESIAN_POINT('Ctrl Pts',(-59.7979818185861,-81.6986640282635,
-420.232830959641));
#36538=CARTESIAN_POINT('Ctrl Pts',(-59.3946866091394,-82.1020293647443,
-420.229990105046));
#36539=CARTESIAN_POINT('Ctrl Pts',(-59.2602124452137,-82.2365276507058,
-420.229012918471));
#36540=CARTESIAN_POINT('Ctrl Pts',(-58.9844213336794,-82.5123697077706,
-420.226949108894));
#36541=CARTESIAN_POINT('Ctrl Pts',(-58.7490049828989,-82.7478313994131,
-420.225112345118));
#36542=CARTESIAN_POINT('Ctrl Pts',(-58.7220957793367,-82.7747458573193,
-420.224899491011));
#36543=CARTESIAN_POINT('Ctrl Pts',(-58.7197046369747,-82.9535412049402,
-419.975191424209));
#36544=CARTESIAN_POINT('Ctrl Pts',(-58.7201238150062,-82.9467669938159,
-419.984638846285));
#36545=CARTESIAN_POINT('Ctrl Pts',(-59.0757619228566,-77.1994056235447,
-427.999999999977));
#36546=CARTESIAN_POINT('Ctrl Pts',(-59.0761804379555,-77.1926421258772,
-428.009432480898));
#36547=CARTESIAN_POINT('Ctrl Pts',(-58.7168005619725,-82.953553272611,-419.975191424209));
#36548=CARTESIAN_POINT('Ctrl Pts',(-58.7172200417724,-82.9467818354254,
-419.984638846285));
#36549=CARTESIAN_POINT('Ctrl Pts',(-59.0731141752743,-77.201773924119,-427.999999999977));
#36550=CARTESIAN_POINT('Ctrl Pts',(-59.0735329916644,-77.1950131960031,
-428.009432480898));
#36551=CARTESIAN_POINT('Ctrl Pts',(-58.7138964869703,-82.9535653402818,
-419.975191424209));
#36552=CARTESIAN_POINT('Ctrl Pts',(-58.7143162685385,-82.9467966770348,
-419.984638846285));
#36553=CARTESIAN_POINT('Ctrl Pts',(-59.070466427692,-77.2041422246933,-427.999999999977));
#36554=CARTESIAN_POINT('Ctrl Pts',(-59.0708855453734,-77.197384266129,-428.009432480898));
#36555=CARTESIAN_POINT('Ctrl Pts',(-58.710992411968,-82.9535774079526,-419.975191424209));
#36556=CARTESIAN_POINT('Ctrl Pts',(-58.7114124953047,-82.9468115186443,
-419.984638846285));
#36557=CARTESIAN_POINT('Ctrl Pts',(-59.0678186801098,-77.2065105252675,
-427.999999999977));
#36558=CARTESIAN_POINT('Ctrl Pts',(-59.0682380990822,-77.199755336255,-428.009432480898));
#36559=CARTESIAN_POINT('Ctrl Pts',(-57.2927718103627,-82.9594707197063,
-419.975191424209));
#36560=CARTESIAN_POINT('Ctrl Pts',(-57.2933392638967,-82.9540594982192,
-419.984638846285));
#36561=CARTESIAN_POINT('Ctrl Pts',(-57.7747769487071,-78.3630828116667,
-427.999999999977));
#36562=CARTESIAN_POINT('Ctrl Pts',(-57.7753435048097,-78.3576801480598,
-428.009432480898));
#36563=CARTESIAN_POINT('Ctrl Pts',(-55.8672055875188,-82.958664597696,-419.975191424209));
#36564=CARTESIAN_POINT('Ctrl Pts',(-55.8677743707687,-82.9544748505942,
-419.984638846285));
#36565=CARTESIAN_POINT('Ctrl Pts',(-56.3503402102711,-79.3998187877058,
-427.999999999977));
#36566=CARTESIAN_POINT('Ctrl Pts',(-56.3509080939867,-79.395635666715,-428.009432480898));
#36567=CARTESIAN_POINT('Ctrl Pts',(-53.0058926090782,-82.9396188430779,
-419.975191424209));
#36568=CARTESIAN_POINT('Ctrl Pts',(-53.0062616495595,-82.937525443936,-419.984638846285));
#36569=CARTESIAN_POINT('Ctrl Pts',(-53.3193621667245,-81.1614483273987,
-427.999999999976));
#36570=CARTESIAN_POINT('Ctrl Pts',(-53.3197306235661,-81.1593582389807,
-428.009432480897));
#36571=CARTESIAN_POINT('Ctrl Pts',(-51.5701817571364,-82.9213583429688,
-419.975191424209));
#36572=CARTESIAN_POINT('Ctrl Pts',(-51.5703504389445,-82.9201394025285,
-419.984638846286));
#36573=CARTESIAN_POINT('Ctrl Pts',(-51.7134630892495,-81.8859686230323,
-427.999999999976));
#36574=CARTESIAN_POINT('Ctrl Pts',(-51.7136315042863,-81.8847516103539,
-428.009432480897));
#36575=CARTESIAN_POINT('Ctrl Pts',(-50.1322857667517,-82.8933990937584,
-419.975191424209));
#36576=CARTESIAN_POINT('Ctrl Pts',(-50.1322106464991,-82.8928617883035,
-419.984638846286));
#36577=CARTESIAN_POINT('Ctrl Pts',(-50.0684772862654,-82.4370022706408,
-427.999999999976));
#36578=CARTESIAN_POINT('Ctrl Pts',(-50.068402284816,-82.4364658149378,-428.009432480897));
#36579=CARTESIAN_POINT('Ctrl Pts',(-50.1290939798984,-82.89333703088,-419.975191424209));
#36580=CARTESIAN_POINT('Ctrl Pts',(-50.1290183184633,-82.8928012384925,
-419.984638846286));
#36581=CARTESIAN_POINT('Ctrl Pts',(-50.0648258093193,-82.4382254341825,
-427.999999999976));
#36582=CARTESIAN_POINT('Ctrl Pts',(-50.0647502675432,-82.4376904891539,
-428.009432480897));
#36583=CARTESIAN_POINT('Ctrl Pts',(-50.1259021930451,-82.8932749680016,
-419.975191424209));
#36584=CARTESIAN_POINT('Ctrl Pts',(-50.1258259904275,-82.8927406886815,
-419.984638846286));
#36585=CARTESIAN_POINT('Ctrl Pts',(-50.0611743323731,-82.4394485977242,
-427.999999999976));
#36586=CARTESIAN_POINT('Ctrl Pts',(-50.0610982502703,-82.4389151633701,
-428.009432480897));
#36587=CARTESIAN_POINT('Ctrl Pts',(-50.1227104061918,-82.8932129051231,
-419.975191424209));
#36588=CARTESIAN_POINT('Ctrl Pts',(-50.1226336623915,-82.8926801388705,
-419.984638846286));
#36589=CARTESIAN_POINT('Ctrl Pts',(-50.057522855427,-82.4406717612658,-427.999999999976));
#36590=CARTESIAN_POINT('Ctrl Pts',(-50.0574462329975,-82.4401398375863,
-428.009432480897));
#36591=CARTESIAN_POINT('',(-50.0684772862639,-82.4370022706413,-427.999999999976));
#36592=CARTESIAN_POINT('Ctrl Pts',(-50.0684772862639,-82.4370022706413,
-427.999999999976));
#36593=CARTESIAN_POINT('Ctrl Pts',(-51.7134630892489,-81.8859686230341,
-427.999999999963));
#36594=CARTESIAN_POINT('Ctrl Pts',(-53.3193621667236,-81.1614483274017,
-427.999999999963));
#36595=CARTESIAN_POINT('Ctrl Pts',(-56.3503402102723,-79.3998187877103,
-427.999999999964));
#36596=CARTESIAN_POINT('Ctrl Pts',(-57.7747769487082,-78.3630828116726,
-427.999999999964));
#36597=CARTESIAN_POINT('Ctrl Pts',(-59.0678186801297,-77.2065105251389,
-427.999999999977));
#36598=CARTESIAN_POINT('',(-58.5551904101346,-82.9475821060765,-419.98463884637));
#36599=CARTESIAN_POINT('Ctrl Pts',(-58.5551904101346,-82.9475821060766,
-419.98463884637));
#36600=CARTESIAN_POINT('Ctrl Pts',(-58.4188729154943,-82.9414614634676,
-419.994305468106));
#36601=CARTESIAN_POINT('Ctrl Pts',(-58.2823655888712,-82.9353237594846,
-420.004474223787));
#36602=CARTESIAN_POINT('Ctrl Pts',(-56.066191044342,-82.8355192518713,-420.178712470519));
#36603=CARTESIAN_POINT('Ctrl Pts',(-54.6525784405451,-82.769565172487,-420.421071349311));
#36604=CARTESIAN_POINT('Ctrl Pts',(-53.0155721288554,-82.6872714498112,
-421.040386425013));
#36605=CARTESIAN_POINT('Ctrl Pts',(-52.5265838564269,-82.6608599495699,
-421.330101387063));
#36606=CARTESIAN_POINT('Ctrl Pts',(-51.7205137979776,-82.6126582331124,
-422.074616347874));
#36607=CARTESIAN_POINT('Ctrl Pts',(-51.3955527915526,-82.5903403336599,
-422.539928724141));
#36608=CARTESIAN_POINT('Ctrl Pts',(-50.8567852682764,-82.5460626358379,
-423.727827254023));
#36609=CARTESIAN_POINT('Ctrl Pts',(-50.6369357056377,-82.5235929056932,
-424.464498286675));
#36610=CARTESIAN_POINT('Ctrl Pts',(-50.2838325468242,-82.4770364056074,
-426.246791579634));
#36611=CARTESIAN_POINT('Ctrl Pts',(-50.1582077546299,-82.4550316503171,
-427.192312850031));
#36612=CARTESIAN_POINT('Ctrl Pts',(-50.0684772862656,-82.4370022706407,
-427.999999999976));
#36613=CARTESIAN_POINT('Origin',(-66.1887815785501,-75.5698420254738,-409.614647535942));
#36614=CARTESIAN_POINT('Ctrl Pts',(58.7197056437309,-82.9535249352716,-419.975214114133));
#36615=CARTESIAN_POINT('Ctrl Pts',(58.7201238150205,-82.9467669938057,-419.984638846287));
#36616=CARTESIAN_POINT('Ctrl Pts',(59.0757619228695,-77.1994056235345,-427.999999999979));
#36617=CARTESIAN_POINT('Ctrl Pts',(59.0761795998615,-77.1926556702662,-428.009413591666));
#36618=CARTESIAN_POINT('Ctrl Pts',(58.7168015694534,-82.9535370096046,-419.975214114133));
#36619=CARTESIAN_POINT('Ctrl Pts',(58.7172200417867,-82.9467818354151,-419.984638846287));
#36620=CARTESIAN_POINT('Ctrl Pts',(59.0731141752874,-77.2017739241088,-427.999999999979));
#36621=CARTESIAN_POINT('Ctrl Pts',(59.073532152967,-77.1950267348458,-428.009413591666));
#36622=CARTESIAN_POINT('Ctrl Pts',(58.7138974951761,-82.9535490839376,-419.975214114133));
#36623=CARTESIAN_POINT('Ctrl Pts',(58.7143162685529,-82.9467966770246,-419.984638846287));
#36624=CARTESIAN_POINT('Ctrl Pts',(59.0704664277052,-77.204142224683,-427.999999999979));
#36625=CARTESIAN_POINT('Ctrl Pts',(59.0708847060726,-77.1973977994254,-428.009413591666));
#36626=CARTESIAN_POINT('Ctrl Pts',(58.7109934208987,-82.9535611582706,-419.975214114133));
#36627=CARTESIAN_POINT('Ctrl Pts',(58.7114124953191,-82.9468115186341,-419.984638846287));
#36628=CARTESIAN_POINT('Ctrl Pts',(59.067818680123,-77.2065105252572,-427.999999999979));
#36629=CARTESIAN_POINT('Ctrl Pts',(59.0682372591782,-77.1997688640051,-428.009413591664));
#36630=CARTESIAN_POINT('Ctrl Pts',(57.2927731732331,-82.9594577235373,-419.975214114133));
#36631=CARTESIAN_POINT('Ctrl Pts',(57.293339263911,-82.9540594982091,-419.984638846287));
#36632=CARTESIAN_POINT('Ctrl Pts',(57.7747769487204,-78.3630828116567,-427.999999999979));
#36633=CARTESIAN_POINT('Ctrl Pts',(57.775342370253,-78.3576909672791,-428.009413591664));
#36634=CARTESIAN_POINT('Ctrl Pts',(55.8672069535827,-82.9586545351486,-419.975214114133));
#36635=CARTESIAN_POINT('Ctrl Pts',(55.867774370783,-82.9544748505844,-419.984638846287));
#36636=CARTESIAN_POINT('Ctrl Pts',(56.3503402102845,-79.399818787696,-427.999999999979));
#36637=CARTESIAN_POINT('Ctrl Pts',(56.3509069567715,-79.3956440437112,-428.009413591664));
#36638=CARTESIAN_POINT('Ctrl Pts',(53.0058934954191,-82.939613815341,-419.975214114133));
#36639=CARTESIAN_POINT('Ctrl Pts',(53.0062616495739,-82.9375254439268,-419.984638846287));
#36640=CARTESIAN_POINT('Ctrl Pts',(53.3193621667384,-81.1614483273895,-427.999999999979));
#36641=CARTESIAN_POINT('Ctrl Pts',(53.3197298857181,-81.1593624245264,-428.009413591664));
#36642=CARTESIAN_POINT('Ctrl Pts',(51.5701821622747,-82.9213554154241,-419.975214114133));
#36643=CARTESIAN_POINT('Ctrl Pts',(51.5703504389588,-82.9201394025195,-419.984638846287));
#36644=CARTESIAN_POINT('Ctrl Pts',(51.7134630892636,-81.8859686230233,-427.999999999978));
#36645=CARTESIAN_POINT('Ctrl Pts',(51.7136311670369,-81.8847540475019,-428.009413591664));
#36646=CARTESIAN_POINT('Ctrl Pts',(50.1322855863494,-82.8933978033003,-419.975214114133));
#36647=CARTESIAN_POINT('Ctrl Pts',(50.1322106465135,-82.8928617882947,-419.984638846287));
#36648=CARTESIAN_POINT('Ctrl Pts',(50.0684772862794,-82.437002270632,-427.999999999978));
#36649=CARTESIAN_POINT('Ctrl Pts',(50.0684024350259,-82.4364668892208,-428.009413591664));
#36650=CARTESIAN_POINT('Ctrl Pts',(50.1290999320919,-82.8933358633196,-419.975214114133));
#36651=CARTESIAN_POINT('Ctrl Pts',(50.1290244534106,-82.8928013548467,-419.984638846287));
#36652=CARTESIAN_POINT('Ctrl Pts',(50.0648328266468,-82.4382230835297,-427.999999999978));
#36653=CARTESIAN_POINT('Ctrl Pts',(50.0647574371849,-82.4376892068704,-428.009413591664));
#36654=CARTESIAN_POINT('Ctrl Pts',(50.1259142778343,-82.893273923339,-419.975214114133));
#36655=CARTESIAN_POINT('Ctrl Pts',(50.1258382603078,-82.8927409213988,-419.984638846287));
#36656=CARTESIAN_POINT('Ctrl Pts',(50.0611883670142,-82.4394438964275,-427.999999999978));
#36657=CARTESIAN_POINT('Ctrl Pts',(50.061112439344,-82.4389115245201,-428.009413591664));
#36658=CARTESIAN_POINT('Ctrl Pts',(50.1227286235768,-82.8932119833583,-419.975214114133));
#36659=CARTESIAN_POINT('Ctrl Pts',(50.1226520672052,-82.8926804879508,-419.984638846287));
#36660=CARTESIAN_POINT('Ctrl Pts',(50.0575439073816,-82.4406647093253,-427.999999999978));
#36661=CARTESIAN_POINT('Ctrl Pts',(50.0574674415031,-82.4401338421698,-428.009413591664));
#36662=CARTESIAN_POINT('',(58.7220957793721,-82.7747458572873,-420.224899491043));
#36663=CARTESIAN_POINT('',(59.0678186800936,-77.2065105252676,-427.999999999979));
#36664=CARTESIAN_POINT('',(58.8949632383239,-79.9905314165215,-424.112584875118));
#36665=CARTESIAN_POINT('',(58.5551904101516,-82.947582106022,-419.984638846415));
#36666=CARTESIAN_POINT('Origin',(66.1887816381845,-75.569842237361,-409.61464764338));
#36667=CARTESIAN_POINT('',(50.0684772862795,-82.4370022706321,-427.999999999977));
#36668=CARTESIAN_POINT('Ctrl Pts',(50.0684772862793,-82.437002270632,-427.999999999977));
#36669=CARTESIAN_POINT('Ctrl Pts',(50.1776098648765,-82.4589300810008,-427.017669438463));
#36670=CARTESIAN_POINT('Ctrl Pts',(50.3084199515129,-82.4805437409056,-426.10749048955));
#36671=CARTESIAN_POINT('Ctrl Pts',(50.6516098353792,-82.5251802709515,-424.410314707175));
#36672=CARTESIAN_POINT('Ctrl Pts',(50.8715944931139,-82.5474330763281,-423.686397055261));
#36673=CARTESIAN_POINT('Ctrl Pts',(51.410590597809,-82.5914145260594,-422.516025627724));
#36674=CARTESIAN_POINT('Ctrl Pts',(51.7358697925533,-82.6136472976727,-422.056380716835));
#36675=CARTESIAN_POINT('Ctrl Pts',(52.5461423541371,-82.6619559233828,-421.316248616454));
#36676=CARTESIAN_POINT('Ctrl Pts',(53.0408434762955,-82.688606506298,-421.027125796862));
#36677=CARTESIAN_POINT('Ctrl Pts',(54.7447370654671,-82.7740803411882,-420.392943782119));
#36678=CARTESIAN_POINT('Ctrl Pts',(56.2220249700593,-82.8426158585167,-420.161956759134));
#36679=CARTESIAN_POINT('Ctrl Pts',(58.3588571103766,-82.9387623345377,-419.998814597882));
#36680=CARTESIAN_POINT('Ctrl Pts',(58.4570557771101,-82.9431758703299,-419.991597823863));
#36681=CARTESIAN_POINT('Ctrl Pts',(58.5551904101466,-82.9475821060663,-419.984638846372));
#36682=CARTESIAN_POINT('Ctrl Pts',(59.0678186800936,-77.2065105252676,-427.999999999979));
#36683=CARTESIAN_POINT('Ctrl Pts',(57.7747769487207,-78.3630828116585,-427.999999999975));
#36684=CARTESIAN_POINT('Ctrl Pts',(56.3503402102848,-79.3998187876973,-427.999999999975));
#36685=CARTESIAN_POINT('Ctrl Pts',(53.3193621667383,-81.1614483273903,-427.999999999975));
#36686=CARTESIAN_POINT('Ctrl Pts',(51.7134630892636,-81.8859686230238,-427.999999999974));
#36687=CARTESIAN_POINT('Ctrl Pts',(50.0684772862795,-82.4370022706321,-427.999999999977));
#36688=CARTESIAN_POINT('Ctrl Pts',(71.6135253144103,-69.8855065275854,-420.221597501088));
#36689=CARTESIAN_POINT('Ctrl Pts',(71.6111594297988,-69.885654348311,-420.224899490929));
#36690=CARTESIAN_POINT('Ctrl Pts',(66.0402789827317,-70.2337235592304,-427.99999999998));
#36691=CARTESIAN_POINT('Ctrl Pts',(66.0377194565832,-70.2338834787001,-428.00357224915));
#36692=CARTESIAN_POINT('Ctrl Pts',(71.611720415822,-69.8873206700759,-420.221597501088));
#36693=CARTESIAN_POINT('Ctrl Pts',(71.6093549056598,-69.8874681586518,-420.224899490929));
#36694=CARTESIAN_POINT('Ctrl Pts',(66.0393561635738,-70.2347552661941,-427.99999999998));
#36695=CARTESIAN_POINT('Ctrl Pts',(66.0367970425222,-70.2349148263284,-428.00357224915));
#36696=CARTESIAN_POINT('Ctrl Pts',(71.6099155172337,-69.8891348125665,-420.221597501088));
#36697=CARTESIAN_POINT('Ctrl Pts',(71.6075503815208,-69.8892819689926,-420.224899490929));
#36698=CARTESIAN_POINT('Ctrl Pts',(66.0384333444158,-70.2357869731577,-427.99999999998));
#36699=CARTESIAN_POINT('Ctrl Pts',(66.0358746284611,-70.2359461739567,-428.00357224915));
#36700=CARTESIAN_POINT('Ctrl Pts',(71.6081106186453,-69.8909489550569,-420.221597501088));
#36701=CARTESIAN_POINT('Ctrl Pts',(71.6057458573818,-69.8910957793334,-420.224899490929));
#36702=CARTESIAN_POINT('Ctrl Pts',(66.0375105252578,-70.2368186801213,-427.99999999998));
#36703=CARTESIAN_POINT('Ctrl Pts',(66.0349522144002,-70.236977521585,-428.00357224915));
#36704=CARTESIAN_POINT('Ctrl Pts',(69.4660550218924,-72.0439752249039,-420.221597501088));
#36705=CARTESIAN_POINT('Ctrl Pts',(69.4641346574551,-72.0437278535411,-420.224899490929));
#36706=CARTESIAN_POINT('Ctrl Pts',(64.9423077504902,-71.4612496203883,-427.99999999998));
#36707=CARTESIAN_POINT('Ctrl Pts',(64.94023020919,-71.460982002319,-428.00357224915));
#36708=CARTESIAN_POINT('Ctrl Pts',(67.3210277409196,-74.194487842424,-420.221597501087));
#36709=CARTESIAN_POINT('Ctrl Pts',(67.3195381750477,-74.1938347730893,-420.224899490929));
#36710=CARTESIAN_POINT('Ctrl Pts',(63.8121002593399,-72.6560711942883,-427.999999999979));
#36711=CARTESIAN_POINT('Ctrl Pts',(63.8104887763535,-72.6553646729174,-428.00357224915));
#36712=CARTESIAN_POINT('Ctrl Pts',(63.0254878424273,-78.4900277409171,-420.221597501087));
#36713=CARTESIAN_POINT('Ctrl Pts',(63.0248347730926,-78.4885381750452,-420.224899490929));
#36714=CARTESIAN_POINT('Ctrl Pts',(61.4870711942897,-74.9811002593389,-427.999999999979));
#36715=CARTESIAN_POINT('Ctrl Pts',(61.4863646729188,-74.9794887763524,-428.00357224915));
#36716=CARTESIAN_POINT('Ctrl Pts',(60.8749752249077,-80.6350550218902,-420.221597501087));
#36717=CARTESIAN_POINT('Ctrl Pts',(60.8747278535448,-80.6331346574529,-420.224899490929));
#36718=CARTESIAN_POINT('Ctrl Pts',(60.2922496203898,-76.1113077504894,-427.999999999979));
#36719=CARTESIAN_POINT('Ctrl Pts',(60.2919820023206,-76.1092302091891,-428.00357224915));
#36720=CARTESIAN_POINT('Ctrl Pts',(58.721948955061,-82.7771106186434,-420.221597501086));
#36721=CARTESIAN_POINT('Ctrl Pts',(58.7220957793374,-82.7747458573798,-420.224899490928));
#36722=CARTESIAN_POINT('Ctrl Pts',(59.067818680123,-77.2065105252572,-427.999999999979));
#36723=CARTESIAN_POINT('Ctrl Pts',(59.0679775215867,-77.2039522143996,-428.00357224915));
#36724=CARTESIAN_POINT('Ctrl Pts',(58.7201348125646,-82.7789155172375,-420.221597501086));
#36725=CARTESIAN_POINT('Ctrl Pts',(58.7202819689909,-82.7765503815246,-420.224899490928));
#36726=CARTESIAN_POINT('Ctrl Pts',(59.0667869731561,-77.2074333444181,-427.999999999979));
#36727=CARTESIAN_POINT('Ctrl Pts',(59.0669461739552,-77.2048746284635,-428.00357224915));
#36728=CARTESIAN_POINT('Ctrl Pts',(58.7183206700682,-82.7807204158317,-420.221597501086));
#36729=CARTESIAN_POINT('Ctrl Pts',(58.7184681586442,-82.7783549056695,-420.224899490928));
#36730=CARTESIAN_POINT('Ctrl Pts',(59.0657552661892,-77.2083561635791,-427.999999999979));
#36731=CARTESIAN_POINT('Ctrl Pts',(59.0659148263236,-77.2057970425275,-428.00357224915));
#36732=CARTESIAN_POINT('Ctrl Pts',(58.716506527572,-82.7825253144258,-420.221597501086));
#36733=CARTESIAN_POINT('Ctrl Pts',(58.7166543482976,-82.7801594298143,-420.224899490928));
#36734=CARTESIAN_POINT('Ctrl Pts',(59.0647235592222,-77.20927898274,-427.999999999977));
#36735=CARTESIAN_POINT('Ctrl Pts',(59.0648834786919,-77.2067194565913,-428.00357224915));
#36736=CARTESIAN_POINT('',(71.605745857323,-69.891095779332,-420.224899491139));
#36737=CARTESIAN_POINT('',(66.0375105251256,-70.2368186801723,-427.99999999998));
#36738=CARTESIAN_POINT('',(68.9076646990879,-70.0586153594102,-423.992314288627));
#36739=CARTESIAN_POINT('Ctrl Pts',(58.7220957793725,-82.7747458572875,-420.224899491013));
#36740=CARTESIAN_POINT('Ctrl Pts',(58.7490050273729,-82.7478313549345,-420.225112345472));
#36741=CARTESIAN_POINT('Ctrl Pts',(58.9844242521529,-82.5123667887596,-420.226949130836));
#36742=CARTESIAN_POINT('Ctrl Pts',(59.2602133340799,-82.2365267616816,-420.229012925029));
#36743=CARTESIAN_POINT('Ctrl Pts',(59.3946877198224,-82.1020282538672,-420.229990113069));
#36744=CARTESIAN_POINT('Ctrl Pts',(59.7979835946476,-81.6986622519067,-420.232830971759));
#36745=CARTESIAN_POINT('Ctrl Pts',(60.066703586697,-81.4298984858598,-420.234604261661));
#36746=CARTESIAN_POINT('Ctrl Pts',(60.8727375567166,-80.6237425199819,-420.239546328562));
#36747=CARTESIAN_POINT('Ctrl Pts',(61.4091231051532,-80.0872881782882,-420.242333151683));
#36748=CARTESIAN_POINT('Ctrl Pts',(63.0213309310981,-78.4749137432377,-420.249082506595));
#36749=CARTESIAN_POINT('Ctrl Pts',(64.0885503716301,-77.4076375096007,-420.251383202111));
#36750=CARTESIAN_POINT('Ctrl Pts',(66.2386463522281,-75.2575415293765,-420.251383186953));
#36751=CARTESIAN_POINT('Ctrl Pts',(67.3059208443083,-74.1903238305842,-420.249082484017));
#36752=CARTESIAN_POINT('Ctrl Pts',(68.918292610394,-72.5781186735924,-420.242333129559));
#36753=CARTESIAN_POINT('Ctrl Pts',(69.4547460698333,-72.0417340073601,-420.239546308459));
#36754=CARTESIAN_POINT('Ctrl Pts',(70.2609007054355,-71.2357013674762,-420.234604247225));
#36755=CARTESIAN_POINT('Ctrl Pts',(70.529664028348,-70.9669818185037,-420.232830959644));
#36756=CARTESIAN_POINT('Ctrl Pts',(70.9330293646617,-70.563686609224,-420.229990105049));
#36757=CARTESIAN_POINT('Ctrl Pts',(71.0675276505347,-70.4292124453869,-420.229012918476));
#36758=CARTESIAN_POINT('Ctrl Pts',(71.3433567842835,-70.1534342547818,-420.226949205589));
#36759=CARTESIAN_POINT('Ctrl Pts',(71.578797254063,-69.9180391215851,-420.225112615161));
#36760=CARTESIAN_POINT('Ctrl Pts',(71.605745857324,-69.891095779334,-420.224899491015));
#36761=CARTESIAN_POINT('Origin',(31.3096308343611,-42.4786310540604,-427.999999997311));
#36762=CARTESIAN_POINT('Ctrl Pts',(71.7242220720048,-61.2914501133736,-419.974938351023));
#36763=CARTESIAN_POINT('Ctrl Pts',(71.7236751619536,-61.2913712681216,-419.98463884629));
#36764=CARTESIAN_POINT('Ctrl Pts',(71.2717722995202,-61.2262227212868,-427.999999999981));
#36765=CARTESIAN_POINT('Ctrl Pts',(71.2712259684319,-61.2261439595009,-428.009690226235));
#36766=CARTESIAN_POINT('Ctrl Pts',(71.7242858769502,-61.2947293352656,-419.974938351023));
#36767=CARTESIAN_POINT('Ctrl Pts',(71.7237373707341,-61.2946510609178,-419.98463884629));
#36768=CARTESIAN_POINT('Ctrl Pts',(71.2705156232239,-61.2299742429503,-427.999999999981));
#36769=CARTESIAN_POINT('Ctrl Pts',(71.2699676976604,-61.2298960514643,-428.009690226235));
#36770=CARTESIAN_POINT('Ctrl Pts',(71.7243496818956,-61.2980085571576,-419.974938351023));
#36771=CARTESIAN_POINT('Ctrl Pts',(71.7237995795144,-61.2979308537141,-419.98463884629));
#36772=CARTESIAN_POINT('Ctrl Pts',(71.2692589469276,-61.2337257646139,-427.999999999981));
#36773=CARTESIAN_POINT('Ctrl Pts',(71.2687094268889,-61.2336481434277,-428.009690226235));
#36774=CARTESIAN_POINT('Ctrl Pts',(71.724413486841,-61.3012877790496,-419.974938351023));
#36775=CARTESIAN_POINT('Ctrl Pts',(71.723861788295,-61.3012106465104,-419.98463884629));
#36776=CARTESIAN_POINT('Ctrl Pts',(71.2680022706313,-61.2374772862774,-427.999999999981));
#36777=CARTESIAN_POINT('Ctrl Pts',(71.2674511561174,-61.2374002353911,-428.009690226235));
#36778=CARTESIAN_POINT('Ctrl Pts',(71.7523909953753,-62.7391772385768,-419.974938351023));
#36779=CARTESIAN_POINT('Ctrl Pts',(71.75113940252,-62.7393504389554,-419.98463884629));
#36780=CARTESIAN_POINT('Ctrl Pts',(70.7169686230227,-62.8824630892614,-427.999999999981));
#36781=CARTESIAN_POINT('Ctrl Pts',(70.7157183551126,-62.882636106289,-428.009690226235));
#36782=CARTESIAN_POINT('Ctrl Pts',(71.7706749200814,-64.1748827234026,-419.974938351022));
#36783=CARTESIAN_POINT('Ctrl Pts',(71.7685254439275,-64.1752616495704,-419.98463884629));
#36784=CARTESIAN_POINT('Ctrl Pts',(69.9924483273891,-64.4883621667363,-427.99999999998));
#36785=CARTESIAN_POINT('Ctrl Pts',(69.9903011266861,-64.4887406917701,-428.009690226234));
#36786=CARTESIAN_POINT('Ctrl Pts',(71.789776830703,-67.0361903512256,-419.974938351022));
#36787=CARTESIAN_POINT('Ctrl Pts',(71.7854748505856,-67.0367743707791,-419.984638846289));
#36788=CARTESIAN_POINT('Ctrl Pts',(68.2308187876961,-67.5193402102826,-427.99999999998));
#36789=CARTESIAN_POINT('Ctrl Pts',(68.2265213616857,-67.5199236115889,-428.009690226233));
#36790=CARTESIAN_POINT('Ctrl Pts',(71.7906156730065,-68.4617566096892,-419.974938351022));
#36791=CARTESIAN_POINT('Ctrl Pts',(71.7850594982106,-68.462339263907,-419.984638846289));
#36792=CARTESIAN_POINT('Ctrl Pts',(67.194082811657,-68.9437769487185,-427.99999999998));
#36793=CARTESIAN_POINT('Ctrl Pts',(67.1885325186674,-68.9443589861345,-428.009690226233));
#36794=CARTESIAN_POINT('Ctrl Pts',(71.7847586494703,-69.8799811589792,-419.974938351022));
#36795=CARTESIAN_POINT('Ctrl Pts',(71.7778115186357,-69.8804124953149,-419.984638846289));
#36796=CARTESIAN_POINT('Ctrl Pts',(66.0375105252578,-70.2368186801213,-427.99999999998));
#36797=CARTESIAN_POINT('Ctrl Pts',(66.0305707487055,-70.2372495598412,-428.009690226233));
#36798=CARTESIAN_POINT('Ctrl Pts',(71.7847466561065,-69.8828852420651,-419.974938351022));
#36799=CARTESIAN_POINT('Ctrl Pts',(71.7777966770263,-69.8833162685488,-419.984638846289));
#36800=CARTESIAN_POINT('Ctrl Pts',(66.0351422246835,-70.2394664277036,-427.99999999998));
#36801=CARTESIAN_POINT('Ctrl Pts',(66.0281996029007,-70.2398969978995,-428.009690226233));
#36802=CARTESIAN_POINT('Ctrl Pts',(71.7847346627427,-69.885789325151,-419.974938351022));
#36803=CARTESIAN_POINT('Ctrl Pts',(71.7777818354168,-69.8862200417827,-419.984638846289));
#36804=CARTESIAN_POINT('Ctrl Pts',(66.0327739241091,-70.2421141752859,-427.99999999998));
#36805=CARTESIAN_POINT('Ctrl Pts',(66.0258284570958,-70.2425444359578,-428.009690226233));
#36806=CARTESIAN_POINT('Ctrl Pts',(71.7847226693789,-69.8886934082369,-419.974938351022));
#36807=CARTESIAN_POINT('Ctrl Pts',(71.7777669938073,-69.8891238150166,-419.984638846289));
#36808=CARTESIAN_POINT('Ctrl Pts',(66.030405623535,-70.2447619228682,-427.99999999998));
#36809=CARTESIAN_POINT('Ctrl Pts',(66.0234573112912,-70.2451918740163,-428.009690226233));
#36810=CARTESIAN_POINT('',(71.2680022706319,-61.2374772862763,-427.999999999981));
#36811=CARTESIAN_POINT('Ctrl Pts',(71.2680022706319,-61.2374772862763,-427.999999999981));
#36812=CARTESIAN_POINT('Ctrl Pts',(70.7169686230221,-62.8824630892616,-427.999999999984));
#36813=CARTESIAN_POINT('Ctrl Pts',(69.9924483273882,-64.4883621667366,-427.999999999984));
#36814=CARTESIAN_POINT('Ctrl Pts',(68.2308187876944,-67.5193402102828,-427.999999999984));
#36815=CARTESIAN_POINT('Ctrl Pts',(67.1940828116548,-68.9437769487187,-427.999999999983));
#36816=CARTESIAN_POINT('Ctrl Pts',(66.0375105251256,-70.2368186801723,-427.99999999998));
#36817=CARTESIAN_POINT('',(71.7785821060487,-69.7241904101463,-419.984638846392));
#36818=CARTESIAN_POINT('Ctrl Pts',(71.778582106068,-69.7241904101441,-419.984638846374));
#36819=CARTESIAN_POINT('Ctrl Pts',(71.7724644689808,-69.5879398537705,-419.994300721347));
#36820=CARTESIAN_POINT('Ctrl Pts',(71.7663297925677,-69.4514997697602,-420.004464228877));
#36821=CARTESIAN_POINT('Ctrl Pts',(71.6665242759986,-67.2352993224928,-420.178695493911));
#36822=CARTESIAN_POINT('Ctrl Pts',(71.60056809321,-65.8216385836969,-420.421054474862));
#36823=CARTESIAN_POINT('Ctrl Pts',(71.5182723428083,-64.1845886707567,-421.040376650859));
#36824=CARTESIAN_POINT('Ctrl Pts',(71.4918603696667,-63.6955909228312,-421.330095000737));
#36825=CARTESIAN_POINT('Ctrl Pts',(71.4436586475032,-62.8895206864909,-422.074609843585));
#36826=CARTESIAN_POINT('Ctrl Pts',(71.4213410766748,-62.5645635997133,-422.539913205919));
#36827=CARTESIAN_POINT('Ctrl Pts',(71.3770638450802,-62.0257982080005,-423.727790377744));
#36828=CARTESIAN_POINT('Ctrl Pts',(71.354594264779,-61.8059481386615,-424.464451567814));
#36829=CARTESIAN_POINT('Ctrl Pts',(71.3080373014504,-61.4528374554223,-426.246752571476));
#36830=CARTESIAN_POINT('Ctrl Pts',(71.2860320806886,-61.3272098966048,-427.192293569671));
#36831=CARTESIAN_POINT('Ctrl Pts',(71.2680022706313,-61.2374772862774,-427.999999999981));
#36832=CARTESIAN_POINT('Origin',(64.4008420083176,-77.3577815719416,-409.614647527464));
#36833=CARTESIAN_POINT('Ctrl Pts',(71.7845769902984,47.5507006514563,-419.975141527627));
#36834=CARTESIAN_POINT('Ctrl Pts',(71.7777670028513,47.5511220435636,-419.984638846302));
#36835=CARTESIAN_POINT('Ctrl Pts',(66.0304070683082,47.9067603076004,-427.999999999993));
#36836=CARTESIAN_POINT('Ctrl Pts',(66.0236629564188,47.9071776234241,-428.009405447549));
#36837=CARTESIAN_POINT('Ctrl Pts',(71.7845890408676,47.5477971654049,-419.975141527627));
#36838=CARTESIAN_POINT('Ctrl Pts',(71.7777818414427,47.5482188608126,-419.984638846302));
#36839=CARTESIAN_POINT('Ctrl Pts',(66.0327748872881,47.9041130984382,-427.999999999993));
#36840=CARTESIAN_POINT('Ctrl Pts',(66.0260335364513,47.9045307146284,-428.009405447549));
#36841=CARTESIAN_POINT('Ctrl Pts',(71.7846010914369,47.5448936793535,-419.975141527627));
#36842=CARTESIAN_POINT('Ctrl Pts',(71.7777966800341,47.5453156780617,-419.984638846302));
#36843=CARTESIAN_POINT('Ctrl Pts',(66.0351427062678,47.901465889276,-427.999999999993));
#36844=CARTESIAN_POINT('Ctrl Pts',(66.0284041164837,47.9018838058327,-428.009405447549));
#36845=CARTESIAN_POINT('Ctrl Pts',(71.7846131420061,47.5419901933021,-419.975141527627));
#36846=CARTESIAN_POINT('Ctrl Pts',(71.7778115186255,47.5424124953107,-419.984638846302));
#36847=CARTESIAN_POINT('Ctrl Pts',(66.0375105252477,47.8988186801138,-427.999999999993));
#36848=CARTESIAN_POINT('Ctrl Pts',(66.0307746965162,47.899236897037,-428.009405447549));
#36849=CARTESIAN_POINT('Ctrl Pts',(71.7904992990764,46.1237688133607,-419.975141527627));
#36850=CARTESIAN_POINT('Ctrl Pts',(71.7850594982006,46.1243392639028,-419.984638846302));
#36851=CARTESIAN_POINT('Ctrl Pts',(67.1940828116472,46.6057769487113,-427.999999999993));
#36852=CARTESIAN_POINT('Ctrl Pts',(67.1886956320016,46.6063418810718,-428.009405447549));
#36853=CARTESIAN_POINT('Ctrl Pts',(71.7896867258443,44.698202583494,-419.975141527626));
#36854=CARTESIAN_POINT('Ctrl Pts',(71.7854748505759,44.6987743707749,-419.984638846302));
#36855=CARTESIAN_POINT('Ctrl Pts',(68.2308187876864,45.1813402102757,-427.999999999993));
#36856=CARTESIAN_POINT('Ctrl Pts',(68.2266476554641,45.1819064664442,-428.009405447549));
#36857=CARTESIAN_POINT('Ctrl Pts',(71.7706298993564,41.8368906599961,-419.975141527626));
#36858=CARTESIAN_POINT('Ctrl Pts',(71.7685254439183,41.8372616495662,-419.984638846302));
#36859=CARTESIAN_POINT('Ctrl Pts',(69.9924483273799,42.1503621667298,-427.999999999992));
#36860=CARTESIAN_POINT('Ctrl Pts',(69.9903642291271,42.1507295675789,-428.009405447548));
#36861=CARTESIAN_POINT('Ctrl Pts',(71.7523647807903,40.4011808662495,-419.975141527626));
#36862=CARTESIAN_POINT('Ctrl Pts',(71.7511394025111,40.4013504389513,-419.984638846301));
#36863=CARTESIAN_POINT('Ctrl Pts',(70.7169686230137,40.5444630892552,-427.999999999992));
#36864=CARTESIAN_POINT('Ctrl Pts',(70.7157550982773,40.5446310216167,-428.009405447548));
#36865=CARTESIAN_POINT('Ctrl Pts',(71.7244019315222,38.9632861635067,-419.975141527626));
#36866=CARTESIAN_POINT('Ctrl Pts',(71.7238617882864,38.9632106465062,-419.984638846301));
#36867=CARTESIAN_POINT('Ctrl Pts',(71.2680022706226,38.8994772862712,-427.999999999992));
#36868=CARTESIAN_POINT('Ctrl Pts',(71.2674673523943,38.899402499775,-428.009405447548));
#36869=CARTESIAN_POINT('Ctrl Pts',(71.7243772829291,38.9620186931902,-419.975141527626));
#36870=CARTESIAN_POINT('Ctrl Pts',(71.7238377437118,38.9619429601488,-419.984638846301));
#36871=CARTESIAN_POINT('Ctrl Pts',(71.2684879938055,38.8980272700272,-427.999999999992));
#36872=CARTESIAN_POINT('Ctrl Pts',(71.2679536737529,38.8979522695799,-428.009405447548));
#36873=CARTESIAN_POINT('Ctrl Pts',(71.7243526343361,38.9607512228738,-419.975141527626));
#36874=CARTESIAN_POINT('Ctrl Pts',(71.7238136991373,38.9606752737917,-419.984638846301));
#36875=CARTESIAN_POINT('Ctrl Pts',(71.2689737169883,38.8965772537831,-427.999999999992));
#36876=CARTESIAN_POINT('Ctrl Pts',(71.2684399951114,38.8965020393849,-428.009405447549));
#36877=CARTESIAN_POINT('Ctrl Pts',(71.724327985743,38.9594837525574,-419.975141527626));
#36878=CARTESIAN_POINT('Ctrl Pts',(71.7237896545628,38.9594075874345,-419.984638846301));
#36879=CARTESIAN_POINT('Ctrl Pts',(71.2694594401712,38.8951272375391,-427.999999999992));
#36880=CARTESIAN_POINT('Ctrl Pts',(71.2689263164701,38.8950518091899,-428.009405447549));
#36881=CARTESIAN_POINT('',(71.6057458573101,47.5530957793322,-420.224899491064));
#36882=CARTESIAN_POINT('',(66.0375105252219,47.898818680116,-427.999999999993));
#36883=CARTESIAN_POINT('',(68.8215314165122,47.7259632383151,-424.112584875133));
#36884=CARTESIAN_POINT('',(71.7786391684187,47.3861353502518,-419.984557726008));
#36885=CARTESIAN_POINT('Origin',(64.4003613790409,55.0197702565038,-409.614309286759));
#36886=CARTESIAN_POINT('',(71.2658001249267,38.9060482850192,-428.000000003827));
#36887=CARTESIAN_POINT('Ctrl Pts',(71.2658001318634,38.9060483074633,-428.000000006487));
#36888=CARTESIAN_POINT('Ctrl Pts',(71.2847793839212,39.0007231868482,-427.151708897607));
#36889=CARTESIAN_POINT('Ctrl Pts',(71.306654613254,39.1265604842562,-426.216057544933));
#36890=CARTESIAN_POINT('Ctrl Pts',(71.3535698042164,39.4855033680191,-424.433577913956));
#36891=CARTESIAN_POINT('Ctrl Pts',(71.3760120589591,39.706267418997,-423.704408309738));
#36892=CARTESIAN_POINT('Ctrl Pts',(71.4203644905395,40.2470716344453,-422.526424835325));
#36893=CARTESIAN_POINT('Ctrl Pts',(71.4427828497872,40.5733100297556,-422.064118343691));
#36894=CARTESIAN_POINT('Ctrl Pts',(71.4914697497189,41.3852894835831,-421.320566931233));
#36895=CARTESIAN_POINT('Ctrl Pts',(71.5183087371882,41.8804392463264,-421.030345873091));
#36896=CARTESIAN_POINT('Ctrl Pts',(71.6043042830006,43.5837088832162,-420.394309344988));
#36897=CARTESIAN_POINT('Ctrl Pts',(71.67321649527,45.0589041174777,-420.162231586715));
#36898=CARTESIAN_POINT('Ctrl Pts',(71.7699783245184,47.1946696740857,-419.99846094143));
#36899=CARTESIAN_POINT('Ctrl Pts',(71.7743121912236,47.2904318327341,-419.991385923449));
#36900=CARTESIAN_POINT('Ctrl Pts',(71.7786391684188,47.3861353502518,-419.984557726009));
#36901=CARTESIAN_POINT('Ctrl Pts',(66.0375105252324,47.8988186801254,-428.));
#36902=CARTESIAN_POINT('Ctrl Pts',(67.1940828116486,46.605776948712,-427.999999999994));
#36903=CARTESIAN_POINT('Ctrl Pts',(68.2308187876859,45.1813402102759,-427.999999999994));
#36904=CARTESIAN_POINT('Ctrl Pts',(69.1116335575328,43.6658511885029,-427.999999999994));
#36905=CARTESIAN_POINT('Ctrl Pts',(69.9912754750915,42.1523801219546,-427.999999999994));
#36906=CARTESIAN_POINT('Ctrl Pts',(70.7150388674181,40.5487396111317,-428.00000000066));
#36907=CARTESIAN_POINT('Ctrl Pts',(71.2658001433482,38.9060482734612,-428.000000005073));
#36908=CARTESIAN_POINT('Ctrl Pts',(58.7165065275772,60.4445253144006,-420.221597501103));
#36909=CARTESIAN_POINT('Ctrl Pts',(58.7166543483028,60.4421594297898,-420.224899490944));
#36910=CARTESIAN_POINT('Ctrl Pts',(59.0647235592219,54.8712789827216,-427.999999999994));
#36911=CARTESIAN_POINT('Ctrl Pts',(59.0648834786915,54.8687194565731,-428.003572249165));
#36912=CARTESIAN_POINT('Ctrl Pts',(58.7183206700676,60.4427204158123,-420.221597501103));
#36913=CARTESIAN_POINT('Ctrl Pts',(58.7184681586435,60.4403549056508,-420.224899490944));
#36914=CARTESIAN_POINT('Ctrl Pts',(59.0657552661854,54.8703561635636,-427.999999999994));
#36915=CARTESIAN_POINT('Ctrl Pts',(59.0659148263198,54.8677970425123,-428.003572249165));
#36916=CARTESIAN_POINT('Ctrl Pts',(58.7201348125581,60.4409155172241,-420.221597501103));
#36917=CARTESIAN_POINT('Ctrl Pts',(58.7202819689841,60.4385503815119,-420.224899490944));
#36918=CARTESIAN_POINT('Ctrl Pts',(59.0667869731489,54.8694333444057,-427.999999999994));
#36919=CARTESIAN_POINT('Ctrl Pts',(59.0669461739481,54.8668746284513,-428.003572249165));
#36920=CARTESIAN_POINT('Ctrl Pts',(58.7219489550484,60.4391106186359,-420.221597501103));
#36921=CARTESIAN_POINT('Ctrl Pts',(58.7220957793248,60.436745857373,-420.224899490944));
#36922=CARTESIAN_POINT('Ctrl Pts',(59.0678186801124,54.8685105252478,-427.999999999994));
#36923=CARTESIAN_POINT('Ctrl Pts',(59.0679775215763,54.8659522143904,-428.003572249165));
#36924=CARTESIAN_POINT('Ctrl Pts',(60.8749752248954,58.2970550218832,-420.221597501103));
#36925=CARTESIAN_POINT('Ctrl Pts',(60.8747278535326,58.2951346574465,-420.224899490944));
#36926=CARTESIAN_POINT('Ctrl Pts',(60.2922496203792,53.7733077504804,-427.999999999994));
#36927=CARTESIAN_POINT('Ctrl Pts',(60.2919820023102,53.7712302091802,-428.003572249165));
#36928=CARTESIAN_POINT('Ctrl Pts',(63.0254878424152,56.1520277409106,-420.221597501103));
#36929=CARTESIAN_POINT('Ctrl Pts',(63.0248347730807,56.1505381750392,-420.224899490944));
#36930=CARTESIAN_POINT('Ctrl Pts',(61.4870711942792,52.64310025933,-427.999999999994));
#36931=CARTESIAN_POINT('Ctrl Pts',(61.4863646729084,52.6414887763439,-428.003572249165));
#36932=CARTESIAN_POINT('Ctrl Pts',(67.3210277409081,51.8564878424186,-420.221597501103));
#36933=CARTESIAN_POINT('Ctrl Pts',(67.3195381750366,51.8558347730841,-420.224899490943));
#36934=CARTESIAN_POINT('Ctrl Pts',(63.8121002593296,50.3180711942801,-427.999999999994));
#36935=CARTESIAN_POINT('Ctrl Pts',(63.8104887763433,50.3173646729094,-428.003572249165));
#36936=CARTESIAN_POINT('Ctrl Pts',(69.4660550218811,49.7059752248992,-420.221597501103));
#36937=CARTESIAN_POINT('Ctrl Pts',(69.4641346574443,49.7057278535363,-420.224899490943));
#36938=CARTESIAN_POINT('Ctrl Pts',(64.94230775048,49.1232496203804,-427.999999999994));
#36939=CARTESIAN_POINT('Ctrl Pts',(64.9402302091799,49.1229820023112,-428.003572249164));
#36940=CARTESIAN_POINT('Ctrl Pts',(71.6081106186342,47.5529489550527,-420.221597501102));
#36941=CARTESIAN_POINT('Ctrl Pts',(71.6057458573713,47.5530957793291,-420.224899490943));
#36942=CARTESIAN_POINT('Ctrl Pts',(66.0375105252477,47.8988186801138,-427.999999999993));
#36943=CARTESIAN_POINT('Ctrl Pts',(66.0349522143902,47.8989775215776,-428.003572249164));
#36944=CARTESIAN_POINT('Ctrl Pts',(71.6099155172282,47.5511348125565,-420.221597501102));
#36945=CARTESIAN_POINT('Ctrl Pts',(71.607550381516,47.5512819689826,-420.224899490943));
#36946=CARTESIAN_POINT('Ctrl Pts',(66.0384333444085,47.8977869731469,-427.999999999993));
#36947=CARTESIAN_POINT('Ctrl Pts',(66.0358746284541,47.897946173946,-428.003572249164));
#36948=CARTESIAN_POINT('Ctrl Pts',(71.6117204158223,47.5493206700602,-420.221597501102));
#36949=CARTESIAN_POINT('Ctrl Pts',(71.6093549056608,47.5494681586361,-420.224899490943));
#36950=CARTESIAN_POINT('Ctrl Pts',(66.0393561635695,47.8967552661801,-427.999999999993));
#36951=CARTESIAN_POINT('Ctrl Pts',(66.0367970425181,47.8969148263145,-428.003572249164));
#36952=CARTESIAN_POINT('Ctrl Pts',(71.6135253144163,47.5475065275639,-420.221597501102));
#36953=CARTESIAN_POINT('Ctrl Pts',(71.6111594298055,47.5476543482895,-420.224899490943));
#36954=CARTESIAN_POINT('Ctrl Pts',(66.0402789827303,47.8957235592132,-427.999999999993));
#36955=CARTESIAN_POINT('Ctrl Pts',(66.037719456582,47.8958834786829,-428.003572249164));
#36956=CARTESIAN_POINT('',(58.7220957792977,60.4367458573386,-420.224899491211));
#36957=CARTESIAN_POINT('',(59.0678186801968,54.8685105250433,-427.999999999994));
#36958=CARTESIAN_POINT('',(58.8896451722718,57.7381845310678,-423.992984762199));
#36959=CARTESIAN_POINT('Ctrl Pts',(71.6057458573105,47.5530957793328,-420.224899491028));
#36960=CARTESIAN_POINT('Ctrl Pts',(71.5788313549573,47.5800050273333,-420.225112345486));
#36961=CARTESIAN_POINT('Ctrl Pts',(71.3433705542102,47.815420487381,-420.226949102679));
#36962=CARTESIAN_POINT('Ctrl Pts',(71.0675267615548,48.0912133341899,-420.229012925044));
#36963=CARTESIAN_POINT('Ctrl Pts',(70.933028253816,48.2256877198568,-420.229990113084));
#36964=CARTESIAN_POINT('Ctrl Pts',(70.5296622520642,48.6289835944733,-420.232830971772));
#36965=CARTESIAN_POINT('Ctrl Pts',(70.2608984859449,48.8977035865951,-420.234604261675));
#36966=CARTESIAN_POINT('Ctrl Pts',(69.4547425199343,49.7037375567473,-420.239546328577));
#36967=CARTESIAN_POINT('Ctrl Pts',(68.9182881782743,50.2401231051503,-420.242333151697));
#36968=CARTESIAN_POINT('Ctrl Pts',(67.305913743342,51.8523309309769,-420.249082506609));
#36969=CARTESIAN_POINT('Ctrl Pts',(66.2386375096525,52.9195503715613,-420.251383202126));
#36970=CARTESIAN_POINT('Ctrl Pts',(64.0885415293445,55.0696463522429,-420.251383186968));
#36971=CARTESIAN_POINT('Ctrl Pts',(63.0213238305098,56.1369208443656,-420.249082484032));
#36972=CARTESIAN_POINT('Ctrl Pts',(61.409118673553,57.7492926104162,-420.242333129574));
#36973=CARTESIAN_POINT('Ctrl Pts',(60.8727340072911,58.2857460698852,-420.239546308474));
#36974=CARTESIAN_POINT('Ctrl Pts',(60.0667013674838,59.0919007054106,-420.23460424724));
#36975=CARTESIAN_POINT('Ctrl Pts',(59.7979818185451,59.3606640282894,-420.232830959659));
#36976=CARTESIAN_POINT('Ctrl Pts',(59.3946866092094,59.7640293646592,-420.229990105064));
#36977=CARTESIAN_POINT('Ctrl Pts',(59.2602124453863,59.898527650518,-420.229012918491));
#36978=CARTESIAN_POINT('Ctrl Pts',(58.9844329063737,60.1743581329234,-420.226949195513));
#36979=CARTESIAN_POINT('Ctrl Pts',(58.7490391213161,60.4097972543148,-420.225112615174));
#36980=CARTESIAN_POINT('Ctrl Pts',(58.7220957793007,60.4367458573401,-420.224899491029));
#36981=CARTESIAN_POINT('Origin',(31.3096343625947,20.140634036236,-428.000000005605));
#36982=CARTESIAN_POINT('Ctrl Pts',(52.3339462257355,60.6512190129386,-419.982643458044));
#36983=CARTESIAN_POINT('Ctrl Pts',(52.3338974363804,60.6510302761279,-419.985958630343));
#36984=CARTESIAN_POINT('Ctrl Pts',(52.2159548757098,60.194781106073,-427.999999999994));
#36985=CARTESIAN_POINT('Ctrl Pts',(52.215905926027,60.19459174905,-428.003326066353));
#36986=CARTESIAN_POINT('Ctrl Pts',(52.3347807659306,60.6512172558263,-419.982643458044));
#36987=CARTESIAN_POINT('Ctrl Pts',(52.3347320200057,60.651028258566,-419.985958630343));
#36988=CARTESIAN_POINT('Ctrl Pts',(52.2168944466177,60.1941494822845,-427.999999999994));
#36989=CARTESIAN_POINT('Ctrl Pts',(52.2168455405077,60.1939598639562,-428.003326066353));
#36990=CARTESIAN_POINT('Ctrl Pts',(52.3356153061257,60.6512154987138,-419.982643458044));
#36991=CARTESIAN_POINT('Ctrl Pts',(52.335566603631,60.6510262410041,-419.985958630343));
#36992=CARTESIAN_POINT('Ctrl Pts',(52.2178340175256,60.1935178584959,-427.999999999994));
#36993=CARTESIAN_POINT('Ctrl Pts',(52.2177851549885,60.1933279788623,-428.003326066353));
#36994=CARTESIAN_POINT('Ctrl Pts',(52.3364498463208,60.6512137416015,-419.982643458044));
#36995=CARTESIAN_POINT('Ctrl Pts',(52.3364011872562,60.6510242234422,-419.985958630343));
#36996=CARTESIAN_POINT('Ctrl Pts',(52.2187735884335,60.1928862347074,-427.999999999994));
#36997=CARTESIAN_POINT('Ctrl Pts',(52.2187247694692,60.1926960937683,-428.003326066353));
#36998=CARTESIAN_POINT('Ctrl Pts',(53.4022460080427,60.648969723097,-419.982643458044));
#36999=CARTESIAN_POINT('Ctrl Pts',(53.4022528138625,60.6484475833501,-419.985958630343));
#37000=CARTESIAN_POINT('Ctrl Pts',(53.4187050874362,59.3862358020305,-427.999999999994));
#37001=CARTESIAN_POINT('Ctrl Pts',(53.4187119156207,59.3857119464688,-428.003326066353));
#37002=CARTESIAN_POINT('Ctrl Pts',(54.4665375661037,60.6443135760932,-419.982643458044));
#37003=CARTESIAN_POINT('Ctrl Pts',(54.4665894999893,60.6434422462875,-419.985958630343));
#37004=CARTESIAN_POINT('Ctrl Pts',(54.5921335951925,58.5371043305541,-427.999999999994));
#37005=CARTESIAN_POINT('Ctrl Pts',(54.592185699739,58.5362301374525,-428.003326066353));
#37006=CARTESIAN_POINT('Ctrl Pts',(56.5916495236165,60.6305361381316,-419.982643458044));
#37007=CARTESIAN_POINT('Ctrl Pts',(56.5917678710043,60.6289357581116,-419.985958630343));
#37008=CARTESIAN_POINT('Ctrl Pts',(56.8778588421339,56.7602042011328,-427.999999999994));
#37009=CARTESIAN_POINT('Ctrl Pts',(56.8779775784257,56.7585985620691,-428.003326066352));
#37010=CARTESIAN_POINT('Ctrl Pts',(57.6524699230681,60.621414847174,-419.982643458044));
#37011=CARTESIAN_POINT('Ctrl Pts',(57.6526095558927,60.6194346069985,-419.985958630343));
#37012=CARTESIAN_POINT('Ctrl Pts',(57.990155581319,55.832435543188,-427.999999999994));
#37013=CARTESIAN_POINT('Ctrl Pts',(57.9902956729941,55.8304487957018,-428.003326066352));
#37014=CARTESIAN_POINT('Ctrl Pts',(58.711323769583,60.6102405408494,-419.982643458044));
#37015=CARTESIAN_POINT('Ctrl Pts',(58.7114711800225,60.607866338805,-419.985958630343));
#37016=CARTESIAN_POINT('Ctrl Pts',(59.0678186801124,54.8685105252478,-427.999999999994));
#37017=CARTESIAN_POINT('Ctrl Pts',(59.0679665749608,54.8661285212862,-428.003326066352));
#37018=CARTESIAN_POINT('Ctrl Pts',(58.7119775738259,60.6102336411164,-419.982643458044));
#37019=CARTESIAN_POINT('Ctrl Pts',(58.7121249890678,60.6078591958146,-419.985958630343));
#37020=CARTESIAN_POINT('Ctrl Pts',(59.0684840983935,54.8679153361491,-427.999999999994));
#37021=CARTESIAN_POINT('Ctrl Pts',(59.0686319980599,54.8655330881308,-428.003326066352));
#37022=CARTESIAN_POINT('Ctrl Pts',(58.7126313780688,60.6102267413832,-419.982643458044));
#37023=CARTESIAN_POINT('Ctrl Pts',(58.7127787981132,60.6078520528242,-419.985958630343));
#37024=CARTESIAN_POINT('Ctrl Pts',(59.0691495166747,54.8673201470504,-427.999999999994));
#37025=CARTESIAN_POINT('Ctrl Pts',(59.0692974211592,54.8649376549753,-428.003326066352));
#37026=CARTESIAN_POINT('Ctrl Pts',(58.7132851823118,60.6102198416502,-419.982643458044));
#37027=CARTESIAN_POINT('Ctrl Pts',(58.7134326071585,60.6078449098338,-419.985958630343));
#37028=CARTESIAN_POINT('Ctrl Pts',(59.0698149349556,54.8667249579515,-427.999999999994));
#37029=CARTESIAN_POINT('Ctrl Pts',(59.0699628442584,54.8643422218199,-428.003326066352));
#37030=CARTESIAN_POINT('',(52.2187735884339,60.1928862347074,-427.999999999994));
#37031=CARTESIAN_POINT('Origin',(36.4516651763393,32.8363615764921,-427.999999997771));
#37032=CARTESIAN_POINT('',(58.5551812881547,60.6095586489222,-419.985958630427));
#37033=CARTESIAN_POINT('Ctrl Pts',(58.5551812881547,60.6095586489222,-419.985958630428));
#37034=CARTESIAN_POINT('Ctrl Pts',(57.8905656231904,60.579613056112,-420.039064310979));
#37035=CARTESIAN_POINT('Ctrl Pts',(57.1413284898495,60.5455711556876,-420.115158862097));
#37036=CARTESIAN_POINT('Ctrl Pts',(55.795021970294,60.4827534710867,-420.346199566438));
#37037=CARTESIAN_POINT('Ctrl Pts',(55.2653957129864,60.4571327211903,-420.489103173694));
#37038=CARTESIAN_POINT('Ctrl Pts',(54.4868753060455,60.4174201214811,-420.816585135814));
#37039=CARTESIAN_POINT('Ctrl Pts',(54.1948026574575,60.4016105264185,-420.991578345459));
#37040=CARTESIAN_POINT('Ctrl Pts',(53.6669859901669,60.3705778942932,-421.448755462825));
#37041=CARTESIAN_POINT('Ctrl Pts',(53.4423116413425,60.3556681374191,-421.74067122796));
#37042=CARTESIAN_POINT('Ctrl Pts',(52.9255518670193,60.3157041841555,-422.736667045547));
#37043=CARTESIAN_POINT('Ctrl Pts',(52.7154746644318,60.2918022892675,-423.579729317975));
#37044=CARTESIAN_POINT('Ctrl Pts',(52.4080044297822,60.2427721479772,-425.617637073544));
#37045=CARTESIAN_POINT('Ctrl Pts',(52.3028359111884,60.2177714544809,-426.785751435106));
#37046=CARTESIAN_POINT('Ctrl Pts',(52.2187735884335,60.1928862347074,-427.999999999994));
#37047=CARTESIAN_POINT('Origin',(65.4233329644767,53.9721173749241,-410.627910492205));
#37048=CARTESIAN_POINT('Ctrl Pts',(-52.3339462257464,60.6512190129295,-419.982643458044));
#37049=CARTESIAN_POINT('Ctrl Pts',(-52.3338974363913,60.6510302761188,-419.985958630342));
#37050=CARTESIAN_POINT('Ctrl Pts',(-52.2159548757207,60.1947811060639,-427.999999999992));
#37051=CARTESIAN_POINT('Ctrl Pts',(-52.2159059260379,60.1945917490409,-428.003326066352));
#37052=CARTESIAN_POINT('Ctrl Pts',(-52.3347807659415,60.6512172558172,-419.982643458044));
#37053=CARTESIAN_POINT('Ctrl Pts',(-52.3347320200165,60.6510282585569,-419.985958630342));
#37054=CARTESIAN_POINT('Ctrl Pts',(-52.2168944466286,60.1941494822754,-427.999999999992));
#37055=CARTESIAN_POINT('Ctrl Pts',(-52.2168455405186,60.1939598639471,-428.003326066352));
#37056=CARTESIAN_POINT('Ctrl Pts',(-52.3356153061366,60.6512154987047,-419.982643458044));
#37057=CARTESIAN_POINT('Ctrl Pts',(-52.3355666036418,60.651026240995,-419.985958630342));
#37058=CARTESIAN_POINT('Ctrl Pts',(-52.2178340175365,60.1935178584868,-427.999999999992));
#37059=CARTESIAN_POINT('Ctrl Pts',(-52.2177851549993,60.1933279788531,-428.003326066352));
#37060=CARTESIAN_POINT('Ctrl Pts',(-52.3364498463317,60.6512137415924,-419.982643458044));
#37061=CARTESIAN_POINT('Ctrl Pts',(-52.336401187267,60.6510242234331,-419.985958630342));
#37062=CARTESIAN_POINT('Ctrl Pts',(-52.2187735884443,60.1928862346983,-427.999999999992));
#37063=CARTESIAN_POINT('Ctrl Pts',(-52.2187247694801,60.1926960937592,-428.003326066352));
#37064=CARTESIAN_POINT('Ctrl Pts',(-53.4022460080535,60.6489697230877,-419.982643458044));
#37065=CARTESIAN_POINT('Ctrl Pts',(-53.4022528138733,60.6484475833408,-419.985958630342));
#37066=CARTESIAN_POINT('Ctrl Pts',(-53.418705087447,59.3862358020211,-427.999999999992));
#37067=CARTESIAN_POINT('Ctrl Pts',(-53.4187119156315,59.3857119464594,-428.003326066352));
#37068=CARTESIAN_POINT('Ctrl Pts',(-54.4665375661146,60.6443135760836,-419.982643458044));
#37069=CARTESIAN_POINT('Ctrl Pts',(-54.4665895,60.6434422462781,-419.985958630342));
#37070=CARTESIAN_POINT('Ctrl Pts',(-54.5921335952031,58.5371043305445,-427.999999999992));
#37071=CARTESIAN_POINT('Ctrl Pts',(-54.5921856997496,58.536230137443,-428.003326066352));
#37072=CARTESIAN_POINT('Ctrl Pts',(-56.5916495236273,60.6305361381218,-419.982643458044));
#37073=CARTESIAN_POINT('Ctrl Pts',(-56.5917678710151,60.6289357581018,-419.985958630342));
#37074=CARTESIAN_POINT('Ctrl Pts',(-56.8778588421441,56.760204201123,-427.999999999992));
#37075=CARTESIAN_POINT('Ctrl Pts',(-56.8779775784359,56.7585985620592,-428.003326066351));
#37076=CARTESIAN_POINT('Ctrl Pts',(-57.652469923079,60.6214148471639,-419.982643458044));
#37077=CARTESIAN_POINT('Ctrl Pts',(-57.6526095559036,60.6194346069884,-419.985958630342));
#37078=CARTESIAN_POINT('Ctrl Pts',(-57.9901555813291,55.8324355431779,-427.999999999992));
#37079=CARTESIAN_POINT('Ctrl Pts',(-57.9902956730042,55.8304487956918,-428.003326066351));
#37080=CARTESIAN_POINT('Ctrl Pts',(-58.7113237695938,60.6102405408391,-419.982643458044));
#37081=CARTESIAN_POINT('Ctrl Pts',(-58.7114711800333,60.6078663387948,-419.985958630342));
#37082=CARTESIAN_POINT('Ctrl Pts',(-59.0678186801224,54.8685105252375,-427.999999999992));
#37083=CARTESIAN_POINT('Ctrl Pts',(-59.0679665749706,54.8661285212758,-428.003326066351));
#37084=CARTESIAN_POINT('Ctrl Pts',(-58.7119775738368,60.6102336411061,-419.982643458044));
#37085=CARTESIAN_POINT('Ctrl Pts',(-58.7121249890787,60.6078591958044,-419.985958630342));
#37086=CARTESIAN_POINT('Ctrl Pts',(-59.0684840984036,54.8679153361386,-427.999999999992));
#37087=CARTESIAN_POINT('Ctrl Pts',(-59.06863199807,54.8655330881203,-428.003326066351));
#37088=CARTESIAN_POINT('Ctrl Pts',(-58.7126313780798,60.610226741373,-419.982643458044));
#37089=CARTESIAN_POINT('Ctrl Pts',(-58.7127787981242,60.6078520528141,-419.985958630342));
#37090=CARTESIAN_POINT('Ctrl Pts',(-59.0691495166847,54.8673201470398,-427.999999999992));
#37091=CARTESIAN_POINT('Ctrl Pts',(-59.0692974211693,54.8649376549648,-428.003326066351));
#37092=CARTESIAN_POINT('Ctrl Pts',(-58.7132851823228,60.6102198416399,-419.982643458044));
#37093=CARTESIAN_POINT('Ctrl Pts',(-58.7134326071696,60.6078449098237,-419.985958630342));
#37094=CARTESIAN_POINT('Ctrl Pts',(-59.0698149349659,54.8667249579411,-427.999999999992));
#37095=CARTESIAN_POINT('Ctrl Pts',(-59.0699628442686,54.8643422218093,-428.003326066351));
#37096=CARTESIAN_POINT('',(-59.0678186801055,54.8685105255263,-427.999999999992));
#37097=CARTESIAN_POINT('',(-52.2187735884448,60.1928862346983,-427.999999999992));
#37098=CARTESIAN_POINT('Origin',(-36.4516627737165,32.8363581330575,-427.999999989399));
#37099=CARTESIAN_POINT('',(-58.7220957793505,60.4367458573009,-420.22489949061));
#37100=CARTESIAN_POINT('',(-58.8949632383227,57.6525314165029,-424.112584875133));
#37101=CARTESIAN_POINT('',(-58.5551812881654,60.609558648911,-419.985958630427));
#37102=CARTESIAN_POINT('Origin',(-65.4233332963058,53.9721185186547,-410.627911078019));
#37103=CARTESIAN_POINT('Ctrl Pts',(-52.2187735884443,60.1928862346983,-427.999999999992));
#37104=CARTESIAN_POINT('Ctrl Pts',(-52.3048068721005,60.2183549238976,-426.757281647839));
#37105=CARTESIAN_POINT('Ctrl Pts',(-52.4145242813431,60.2444171332054,-425.539778431885));
#37106=CARTESIAN_POINT('Ctrl Pts',(-52.7414645491196,60.2952148912895,-423.449355059722));
#37107=CARTESIAN_POINT('Ctrl Pts',(-52.9555637437187,60.3179344965143,-422.684012418721));
#37108=CARTESIAN_POINT('Ctrl Pts',(-53.4350583564631,60.3551633628339,-421.751436601779));
#37109=CARTESIAN_POINT('Ctrl Pts',(-53.6588138203951,60.3700593220912,-421.458014299146));
#37110=CARTESIAN_POINT('Ctrl Pts',(-54.1844910544222,60.401037189882,-420.998625299011));
#37111=CARTESIAN_POINT('Ctrl Pts',(-54.475305566902,60.4168068389036,-420.822774395234));
#37112=CARTESIAN_POINT('Ctrl Pts',(-55.2486929141825,60.4563082169502,-420.494554521714));
#37113=CARTESIAN_POINT('Ctrl Pts',(-55.7731969610708,60.4817083073866,-420.35148029123));
#37114=CARTESIAN_POINT('Ctrl Pts',(-57.1207377485714,60.5446364896661,-420.117199581875));
#37115=CARTESIAN_POINT('Ctrl Pts',(-57.8825166626905,60.5792503940301,-420.039707457912));
#37116=CARTESIAN_POINT('Ctrl Pts',(-58.5551812881653,60.609558648912,-419.985958630427));
#37117=CARTESIAN_POINT('Ctrl Pts',(-58.7165065275705,60.4445253144079,-420.221597501101));
#37118=CARTESIAN_POINT('Ctrl Pts',(-58.7166543482962,60.4421594297969,-420.224899490943));
#37119=CARTESIAN_POINT('Ctrl Pts',(-59.0647235592219,54.8712789827201,-427.999999999992));
#37120=CARTESIAN_POINT('Ctrl Pts',(-59.0648834786916,54.8687194565718,-428.003572249163));
#37121=CARTESIAN_POINT('Ctrl Pts',(-58.7183206700667,60.4427204158139,-420.221597501101));
#37122=CARTESIAN_POINT('Ctrl Pts',(-58.7184681586425,60.4403549056522,-420.224899490943));
#37123=CARTESIAN_POINT('Ctrl Pts',(-59.0657552661887,54.8703561635592,-427.999999999992));
#37124=CARTESIAN_POINT('Ctrl Pts',(-59.0659148263231,54.8677970425078,-428.003572249163));
#37125=CARTESIAN_POINT('Ctrl Pts',(-58.720134812563,60.4409155172199,-420.221597501101));
#37126=CARTESIAN_POINT('Ctrl Pts',(-58.720281968989,60.4385503815075,-420.224899490943));
#37127=CARTESIAN_POINT('Ctrl Pts',(-59.0667869731556,54.8694333443983,-427.999999999992));
#37128=CARTESIAN_POINT('Ctrl Pts',(-59.0669461739546,54.8668746284439,-428.003572249163));
#37129=CARTESIAN_POINT('Ctrl Pts',(-58.7219489550591,60.4391106186259,-420.221597501101));
#37130=CARTESIAN_POINT('Ctrl Pts',(-58.7220957793355,60.4367458573628,-420.224899490943));
#37131=CARTESIAN_POINT('Ctrl Pts',(-59.0678186801224,54.8685105252375,-427.999999999992));
#37132=CARTESIAN_POINT('Ctrl Pts',(-59.0679775215862,54.8659522143801,-428.003572249163));
#37133=CARTESIAN_POINT('Ctrl Pts',(-60.8749752249057,58.2970550218727,-420.221597501101));
#37134=CARTESIAN_POINT('Ctrl Pts',(-60.874727853543,58.2951346574359,-420.224899490943));
#37135=CARTESIAN_POINT('Ctrl Pts',(-60.292249620389,53.7733077504698,-427.999999999992));
#37136=CARTESIAN_POINT('Ctrl Pts',(-60.2919820023199,53.7712302091697,-428.003572249163));
#37137=CARTESIAN_POINT('Ctrl Pts',(-63.0254878424252,56.1520277408997,-420.221597501101));
#37138=CARTESIAN_POINT('Ctrl Pts',(-63.0248347730907,56.1505381750281,-420.224899490943));
#37139=CARTESIAN_POINT('Ctrl Pts',(-61.4870711942888,52.6431002593193,-427.999999999992));
#37140=CARTESIAN_POINT('Ctrl Pts',(-61.486364672918,52.6414887763331,-428.003572249163));
#37141=CARTESIAN_POINT('Ctrl Pts',(-67.3210277409174,51.8564878424069,-420.221597501101));
#37142=CARTESIAN_POINT('Ctrl Pts',(-67.3195381750458,51.8558347730723,-420.224899490942));
#37143=CARTESIAN_POINT('Ctrl Pts',(-63.8121002593388,50.3180711942689,-427.999999999992));
#37144=CARTESIAN_POINT('Ctrl Pts',(-63.8104887763525,50.3173646728982,-428.003572249163));
#37145=CARTESIAN_POINT('Ctrl Pts',(-69.46605502189,49.7059752248871,-420.221597501101));
#37146=CARTESIAN_POINT('Ctrl Pts',(-69.4641346574531,49.7057278535242,-420.224899490941));
#37147=CARTESIAN_POINT('Ctrl Pts',(-64.942307750489,49.123249620369,-427.999999999991));
#37148=CARTESIAN_POINT('Ctrl Pts',(-64.9402302091889,49.1229820022998,-428.003572249162));
#37149=CARTESIAN_POINT('Ctrl Pts',(-71.6081106186428,47.5529489550402,-420.2215975011));
#37150=CARTESIAN_POINT('Ctrl Pts',(-71.6057458573797,47.5530957793166,-420.224899490941));
#37151=CARTESIAN_POINT('Ctrl Pts',(-66.0375105252564,47.8988186801022,-427.999999999991));
#37152=CARTESIAN_POINT('Ctrl Pts',(-66.034952214399,47.898977521566,-428.003572249162));
#37153=CARTESIAN_POINT('Ctrl Pts',(-71.6099155172309,47.5511348125498,-420.2215975011));
#37154=CARTESIAN_POINT('Ctrl Pts',(-71.6075503815186,47.5512819689759,-420.224899490941));
#37155=CARTESIAN_POINT('Ctrl Pts',(-66.0384333444143,47.8977869731387,-427.999999999991));
#37156=CARTESIAN_POINT('Ctrl Pts',(-66.0358746284599,47.8979461739377,-428.003572249162));
#37157=CARTESIAN_POINT('Ctrl Pts',(-71.6117204158191,47.5493206700594,-420.2215975011));
#37158=CARTESIAN_POINT('Ctrl Pts',(-71.6093549056575,47.5494681586352,-420.224899490941));
#37159=CARTESIAN_POINT('Ctrl Pts',(-66.0393561635722,47.8967552661752,-427.999999999991));
#37160=CARTESIAN_POINT('Ctrl Pts',(-66.0367970425208,47.8969148263095,-428.003572249162));
#37161=CARTESIAN_POINT('Ctrl Pts',(-71.6135253144073,47.5475065275691,-420.2215975011));
#37162=CARTESIAN_POINT('Ctrl Pts',(-71.6111594297964,47.5476543482947,-420.224899490941));
#37163=CARTESIAN_POINT('Ctrl Pts',(-66.04027898273,47.8957235592116,-427.999999999991));
#37164=CARTESIAN_POINT('Ctrl Pts',(-66.0377194565817,47.8958834786813,-428.003572249162));
#37165=CARTESIAN_POINT('',(-66.0375105252203,47.8988186801189,-427.999999999992));
#37166=CARTESIAN_POINT('Origin',(-31.3096249078695,20.1406251047006,-427.999999986154));
#37167=CARTESIAN_POINT('',(-71.6057458573148,47.5530957793236,-420.224899491057));
#37168=CARTESIAN_POINT('',(-68.9076650111372,47.720615340018,-423.992313852913));
#37169=CARTESIAN_POINT('Ctrl Pts',(-58.7220957793437,60.4367458572975,-420.224899491029));
#37170=CARTESIAN_POINT('Ctrl Pts',(-58.7490050273443,60.4098313549443,-420.225112345487));
#37171=CARTESIAN_POINT('Ctrl Pts',(-58.9844219604456,60.1743690808714,-420.226949113703));
#37172=CARTESIAN_POINT('Ctrl Pts',(-59.2602133340583,59.8985267616844,-420.229012925044));
#37173=CARTESIAN_POINT('Ctrl Pts',(-59.394687719799,59.7640282538717,-420.229990113084));
#37174=CARTESIAN_POINT('Ctrl Pts',(-59.7979835947372,59.3606622517981,-420.232830971774));
#37175=CARTESIAN_POINT('Ctrl Pts',(-60.0667035867286,59.0918984858094,-420.234604261676));
#37176=CARTESIAN_POINT('Ctrl Pts',(-60.8727375567052,58.2857425199744,-420.239546328577));
#37177=CARTESIAN_POINT('Ctrl Pts',(-61.4091231051397,57.7492881782828,-420.242333151698));
#37178=CARTESIAN_POINT('Ctrl Pts',(-63.0213309310531,56.1369137432638,-420.249082506609));
#37179=CARTESIAN_POINT('Ctrl Pts',(-64.0885503716052,55.0696375096067,-420.251383202125));
#37180=CARTESIAN_POINT('Ctrl Pts',(-66.238646352251,52.9195415293347,-420.251383186966));
#37181=CARTESIAN_POINT('Ctrl Pts',(-67.3059208443576,51.852323830516,-420.249082484029));
#37182=CARTESIAN_POINT('Ctrl Pts',(-68.9182926103748,50.2401186735927,-420.242333129571));
#37183=CARTESIAN_POINT('Ctrl Pts',(-69.4547460697976,49.703734007377,-420.239546308471));
#37184=CARTESIAN_POINT('Ctrl Pts',(-70.2609007054035,48.8977013674892,-420.234604247237));
#37185=CARTESIAN_POINT('Ctrl Pts',(-70.5296640282886,48.6289818185442,-420.232830959655));
#37186=CARTESIAN_POINT('Ctrl Pts',(-70.9330293646132,48.2256866092536,-420.229990105061));
#37187=CARTESIAN_POINT('Ctrl Pts',(-71.0675276504441,48.0912124454586,-420.229012918488));
#37188=CARTESIAN_POINT('Ctrl Pts',(-71.3433692203882,47.8154218209551,-420.226949112555));
#37189=CARTESIAN_POINT('Ctrl Pts',(-71.5788313994088,47.5800049828864,-420.225112345133));
#37190=CARTESIAN_POINT('Ctrl Pts',(-71.605745857315,47.5530957793241,-420.224899491026));
#37191=CARTESIAN_POINT('Ctrl Pts',(-71.7845249352717,47.5507056437107,-419.975214114147));
#37192=CARTESIAN_POINT('Ctrl Pts',(-71.7777669938055,47.5511238150004,-419.984638846301));
#37193=CARTESIAN_POINT('Ctrl Pts',(-66.0304056235332,47.9067619228495,-427.999999999991));
#37194=CARTESIAN_POINT('Ctrl Pts',(-66.0236556702644,47.9071795998414,-428.009413591679));
#37195=CARTESIAN_POINT('Ctrl Pts',(-71.7845370096047,47.547801569433,-419.975214114147));
#37196=CARTESIAN_POINT('Ctrl Pts',(-71.777781835415,47.5482200417663,-419.984638846301));
#37197=CARTESIAN_POINT('Ctrl Pts',(-66.0327739241075,47.9041141752671,-427.999999999991));
#37198=CARTESIAN_POINT('Ctrl Pts',(-66.0260267348443,47.9045321529467,-428.009413591679));
#37199=CARTESIAN_POINT('Ctrl Pts',(-71.7845490839377,47.5448974951555,-419.975214114147));
#37200=CARTESIAN_POINT('Ctrl Pts',(-71.7777966770244,47.5453162685322,-419.984638846301));
#37201=CARTESIAN_POINT('Ctrl Pts',(-66.035142224682,47.9014664276846,-427.999999999991));
#37202=CARTESIAN_POINT('Ctrl Pts',(-66.0283977994242,47.9018847060521,-428.009413591679));
#37203=CARTESIAN_POINT('Ctrl Pts',(-71.7845611582707,47.5419934208777,-419.975214114147));
#37204=CARTESIAN_POINT('Ctrl Pts',(-71.7778115186339,47.5424124952982,-419.984638846301));
#37205=CARTESIAN_POINT('Ctrl Pts',(-66.0375105252564,47.8988186801022,-427.999999999991));
#37206=CARTESIAN_POINT('Ctrl Pts',(-66.0307688640041,47.8992372591574,-428.009413591679));
#37207=CARTESIAN_POINT('Ctrl Pts',(-71.7904577235372,46.1237731732124,-419.975214114147));
#37208=CARTESIAN_POINT('Ctrl Pts',(-71.7850594982088,46.1243392638902,-419.984638846301));
#37209=CARTESIAN_POINT('Ctrl Pts',(-67.1940828116557,46.6057769486995,-427.999999999991));
#37210=CARTESIAN_POINT('Ctrl Pts',(-67.1886909672778,46.6063423702321,-428.009413591679));
#37211=CARTESIAN_POINT('Ctrl Pts',(-71.7896545351483,44.6982069535623,-419.975214114147));
#37212=CARTESIAN_POINT('Ctrl Pts',(-71.7854748505838,44.6987743707624,-419.9846388463));
#37213=CARTESIAN_POINT('Ctrl Pts',(-68.2308187876946,45.1813402102638,-427.999999999991));
#37214=CARTESIAN_POINT('Ctrl Pts',(-68.2266440437095,45.1819069567506,-428.009413591679));
#37215=CARTESIAN_POINT('Ctrl Pts',(-71.77061381534,41.8368934953987,-419.975214114147));
#37216=CARTESIAN_POINT('Ctrl Pts',(-71.7685254439257,41.8372616495537,-419.9846388463));
#37217=CARTESIAN_POINT('Ctrl Pts',(-69.9924483273876,42.1503621667176,-427.999999999991));
#37218=CARTESIAN_POINT('Ctrl Pts',(-69.9903624245244,42.1507298856973,-428.009413591678));
#37219=CARTESIAN_POINT('Ctrl Pts',(-71.7523554154229,40.4011821622547,-419.975214114146));
#37220=CARTESIAN_POINT('Ctrl Pts',(-71.7511394025183,40.4013504389388,-419.9846388463));
#37221=CARTESIAN_POINT('Ctrl Pts',(-70.7169686230211,40.5444630892429,-427.99999999999));
#37222=CARTESIAN_POINT('Ctrl Pts',(-70.7157540474996,40.5446311670161,-428.009413591678));
#37223=CARTESIAN_POINT('Ctrl Pts',(-71.7243978032989,38.9632855863295,-419.975214114146));
#37224=CARTESIAN_POINT('Ctrl Pts',(-71.7238617882933,38.9632106464937,-419.9846388463));
#37225=CARTESIAN_POINT('Ctrl Pts',(-71.2680022706297,38.8994772862588,-427.99999999999));
#37226=CARTESIAN_POINT('Ctrl Pts',(-71.2674668892185,38.8994024350053,-428.009413591677));
#37227=CARTESIAN_POINT('Ctrl Pts',(-71.7243358633182,38.9600999320719,-419.975214114146));
#37228=CARTESIAN_POINT('Ctrl Pts',(-71.7238013548453,38.9600244533907,-419.9846388463));
#37229=CARTESIAN_POINT('Ctrl Pts',(-71.2692230835275,38.895832826626,-427.99999999999));
#37230=CARTESIAN_POINT('Ctrl Pts',(-71.2686892068682,38.8957574371642,-428.009413591677));
#37231=CARTESIAN_POINT('Ctrl Pts',(-71.7242739233376,38.9569142778141,-419.975214114145));
#37232=CARTESIAN_POINT('Ctrl Pts',(-71.7237409213973,38.9568382602878,-419.9846388463));
#37233=CARTESIAN_POINT('Ctrl Pts',(-71.2704438964254,38.8921883669931,-427.99999999999));
#37234=CARTESIAN_POINT('Ctrl Pts',(-71.2699115245179,38.892112439323,-428.009413591677));
#37235=CARTESIAN_POINT('Ctrl Pts',(-71.7242119833569,38.9537286235565,-419.975214114145));
#37236=CARTESIAN_POINT('Ctrl Pts',(-71.7236804879494,38.9536520671848,-419.9846388463));
#37237=CARTESIAN_POINT('Ctrl Pts',(-71.2716647093232,38.8885439073604,-427.99999999999));
#37238=CARTESIAN_POINT('Ctrl Pts',(-71.2711338421677,38.8884674414819,-428.009413591677));
#37239=CARTESIAN_POINT('',(-71.2680022706297,38.8994772862588,-427.99999999999));
#37240=CARTESIAN_POINT('Ctrl Pts',(-71.2680022706297,38.8994772862588,-427.99999999999));
#37241=CARTESIAN_POINT('Ctrl Pts',(-70.7169686230207,40.544463089243,-427.999999999993));
#37242=CARTESIAN_POINT('Ctrl Pts',(-69.9924483273869,42.1503621667178,-427.999999999994));
#37243=CARTESIAN_POINT('Ctrl Pts',(-68.2308187876938,45.1813402102631,-427.999999999994));
#37244=CARTESIAN_POINT('Ctrl Pts',(-67.1940828116546,46.6057769486988,-427.999999999994));
#37245=CARTESIAN_POINT('Ctrl Pts',(-66.0375105252203,47.8988186801189,-427.999999999992));
#37246=CARTESIAN_POINT('',(-71.7785821060461,47.3861904101294,-419.984638846405));
#37247=CARTESIAN_POINT('Ctrl Pts',(-71.7785821060662,47.3861904101271,-419.984638846386));
#37248=CARTESIAN_POINT('Ctrl Pts',(-71.7724611885407,47.2498667926128,-419.994305902311));
#37249=CARTESIAN_POINT('Ctrl Pts',(-71.7663232076033,47.113353314811,-420.004475138088));
#37250=CARTESIAN_POINT('Ctrl Pts',(-71.6665187924467,44.8971811433478,-420.178714023205));
#37251=CARTESIAN_POINT('Ctrl Pts',(-71.600564905539,43.4835729440167,-420.421072892069));
#37252=CARTESIAN_POINT('Ctrl Pts',(-71.5182713684043,41.8465706212519,-421.040387316386));
#37253=CARTESIAN_POINT('Ctrl Pts',(-71.4918599114317,41.3575832154767,-421.330101967646));
#37254=CARTESIAN_POINT('Ctrl Pts',(-71.443658195456,40.5515131717966,-422.07461693779));
#37255=CARTESIAN_POINT('Ctrl Pts',(-71.4213402659048,40.2265518059047,-422.539930138472));
#37256=CARTESIAN_POINT('Ctrl Pts',(-71.3770625254436,39.6877840871316,-423.727830620286));
#37257=CARTESIAN_POINT('Ctrl Pts',(-71.3545927816378,39.4679345708994,-424.464502550804));
#37258=CARTESIAN_POINT('Ctrl Pts',(-71.3080362258214,39.1148313554367,-426.246798891955));
#37259=CARTESIAN_POINT('Ctrl Pts',(-71.2860316626743,38.9892078161781,-427.192312295973));
#37260=CARTESIAN_POINT('Ctrl Pts',(-71.2680022706297,38.8994772862587,-427.99999999999));
#37261=CARTESIAN_POINT('Origin',(-64.400842226757,55.0197816364623,-409.61464763811));
#37262=CARTESIAN_POINT('Origin',(8.04911692853239E-13,-11.1690000000094,
-427.999999999986));
#37263=CARTESIAN_POINT('Origin',(47.765853049082,-53.3647801549723,-427.999999999982));
#37264=CARTESIAN_POINT('',(43.3329036555858,-83.6944436817575,-427.999999999976));
#37265=CARTESIAN_POINT('Origin',(42.1957801549698,-58.9348530490775,-427.99999999998));
#37266=CARTESIAN_POINT('',(-43.3329036555715,-83.6944436817652,-427.999999999975));
#37267=CARTESIAN_POINT('Origin',(-7.51898543427387E-11,859.831,-428.000000000083));
#37268=CARTESIAN_POINT('Origin',(-42.1957801549599,-58.9348530490849,-427.999999999979));
#37269=CARTESIAN_POINT('',(-72.5254436817472,-54.5019036555938,-427.999999999977));
#37270=CARTESIAN_POINT('Origin',(-47.7658530490669,-53.3647801549782,-427.99999999998));
#37271=CARTESIAN_POINT('',(-72.525443681755,32.1639036555634,-427.999999999987));
#37272=CARTESIAN_POINT('Origin',(871.,-11.1689999999327,-427.99999999999));
#37273=CARTESIAN_POINT('Origin',(-47.7658530490746,31.0267801549515,-427.99999999999));
#37274=CARTESIAN_POINT('',(-42.3714057377688,64.2789556966095,-427.999999999994));
#37275=CARTESIAN_POINT('Origin',(-34.2237874382673,30.734273111837,-427.99999999999));
#37276=CARTESIAN_POINT('',(42.3714057377573,64.278955696617,-427.999999999995));
#37277=CARTESIAN_POINT('Origin',(9.43689570931383E-12,-110.169000000009,
-427.999999999975));
#37278=CARTESIAN_POINT('Origin',(34.2237874382616,30.7342731118431,-427.999999999991));
#37279=CARTESIAN_POINT('Origin',(47.7658530490689,31.0267801549598,-427.999999999991));
#37280=CARTESIAN_POINT('Origin',(26.9899999999942,67.2000000000338,-73.7599999999943));
#37281=CARTESIAN_POINT('',(28.4333756729943,67.2000000000342,-71.2599999999944));
#37282=CARTESIAN_POINT('',(29.8767513458943,67.200000000034,-73.7599999999943));
#37283=CARTESIAN_POINT('',(29.1550635094443,67.2000000000341,-72.5099999999943));
#37284=CARTESIAN_POINT('',(28.4333756729943,67.2000000000336,-76.2599999999943));
#37285=CARTESIAN_POINT('',(29.1550635094443,67.2000000000338,-75.0099999999943));
#37286=CARTESIAN_POINT('',(25.5466243269943,67.2000000000334,-76.2599999999943));
#37287=CARTESIAN_POINT('',(26.9899999999942,67.2000000000335,-76.2599999999943));
#37288=CARTESIAN_POINT('',(24.1032486540943,67.2000000000335,-73.7599999999943));
#37289=CARTESIAN_POINT('',(24.8249364905443,67.2000000000334,-75.0099999999943));
#37290=CARTESIAN_POINT('',(25.5466243269943,67.2000000000339,-71.2599999999944));
#37291=CARTESIAN_POINT('',(24.8249364905443,67.2000000000337,-72.5099999999943));
#37292=CARTESIAN_POINT('',(27.7116878364943,67.2000000000341,-71.2599999999944));
#37293=CARTESIAN_POINT('Origin',(26.9999999999943,67.2000000000295,-110.759999999994));
#37294=CARTESIAN_POINT('',(28.4433756729943,67.2000000000299,-108.259999999994));
#37295=CARTESIAN_POINT('',(29.8867513458943,67.2000000000298,-110.759999999994));
#37296=CARTESIAN_POINT('',(29.1650635094443,67.2000000000299,-109.509999999994));
#37297=CARTESIAN_POINT('',(28.4433756729943,67.2000000000294,-113.259999999994));
#37298=CARTESIAN_POINT('',(29.1650635094443,67.2000000000295,-112.009999999994));
#37299=CARTESIAN_POINT('',(25.5566243269942,67.2000000000291,-113.259999999994));
#37300=CARTESIAN_POINT('',(26.9999999999943,67.2000000000292,-113.259999999994));
#37301=CARTESIAN_POINT('',(24.1132486540943,67.2000000000293,-110.759999999994));
#37302=CARTESIAN_POINT('',(24.8349364905443,67.2000000000291,-112.009999999994));
#37303=CARTESIAN_POINT('',(25.5566243269942,67.2000000000296,-108.259999999994));
#37304=CARTESIAN_POINT('',(24.8349364905443,67.2000000000295,-109.509999999994));
#37305=CARTESIAN_POINT('',(27.7216878364943,67.2000000000299,-108.259999999994));
#37306=CARTESIAN_POINT('Origin',(-55.0000000000061,71.331,-304.499999999995));
#37307=CARTESIAN_POINT('',(-1.50000000000603,70.3310000000047,-304.499999999994));
#37308=CARTESIAN_POINT('Origin',(50.9999999999939,71.3309999999974,-407.499999999995));
#37309=CARTESIAN_POINT('',(50.999999999994,70.3310000000034,-355.499999999994));
#37310=CARTESIAN_POINT('Origin',(-55.0000000000061,71.3309999999883,-406.499999999995));
#37311=CARTESIAN_POINT('',(-1.50000000000603,70.330999999993,-406.499999999995));
#37312=CARTESIAN_POINT('Origin',(-54.0000000000061,71.3309999999883,-407.499999999995));
#37313=CARTESIAN_POINT('',(-54.000000000006,70.3309999999942,-355.499999999994));
#37314=CARTESIAN_POINT('Origin',(-47.7658530490666,-53.3647801549749,-400.49999999998));
#37315=CARTESIAN_POINT('',(-73.0049525312943,-54.5239258606288,-400.499999999979));
#37316=CARTESIAN_POINT('',(-71.7514247672298,-61.3050642049046,-400.499999999979));
#37317=CARTESIAN_POINT('Origin',(-47.7658530490666,-53.3647801549749,-400.49999999998));
#37318=CARTESIAN_POINT('',(-73.0049525312945,-54.5239258606286,-400.499999999977));
#37319=CARTESIAN_POINT('Ctrl Pts',(-71.7514247672298,-61.3050642049046,
-400.499999999979));
#37320=CARTESIAN_POINT('Ctrl Pts',(-71.5902902839036,-61.2826808326117,
-409.666667134937));
#37321=CARTESIAN_POINT('Ctrl Pts',(-71.4291495149372,-61.2601533109042,
-418.833333808622));
#37322=CARTESIAN_POINT('Ctrl Pts',(-71.2680022706209,-61.2374772862897,
-427.999999999979));
#37323=CARTESIAN_POINT('Origin',(-72.1248916810212,-69.8588628384965,-400.499999999977));
#37324=CARTESIAN_POINT('',(-72.1248916810212,-69.8588628384965,-400.499999999977));
#37325=CARTESIAN_POINT('',(-72.1248916810212,-69.8588628384965,-400.499999999977));
#37326=CARTESIAN_POINT('',(-71.7514247672298,-61.3050642049048,-400.499999999978));
#37327=CARTESIAN_POINT('Origin',(-58.6898628384754,-83.2938916810397,-400.499999999976));
#37328=CARTESIAN_POINT('',(-58.6898628384754,-83.2938916810397,-400.499999999976));
#37329=CARTESIAN_POINT('',(-58.6898628384754,-83.2938916810397,-400.499999999976));
#37330=CARTESIAN_POINT('',(-72.1248916810212,-69.8588628384965,-400.499999999977));
#37331=CARTESIAN_POINT('Origin',(-50.136064204883,-82.9204247672467,-400.499999999976));
#37332=CARTESIAN_POINT('',(-50.1360642048832,-82.9204247672467,-400.499999999977));
#37333=CARTESIAN_POINT('Ctrl Pts',(-50.1360642048832,-82.9204247672467,
-400.499999999977));
#37334=CARTESIAN_POINT('Ctrl Pts',(-50.1136808325894,-82.7592902839214,
-409.666667134934));
#37335=CARTESIAN_POINT('Ctrl Pts',(-50.0911533108812,-82.5981495149561,
-418.83333380862));
#37336=CARTESIAN_POINT('Ctrl Pts',(-50.0684772862639,-82.4370022706413,
-427.999999999976));
#37337=CARTESIAN_POINT('',(-58.6898628384754,-83.2938916810397,-400.499999999976));
#37338=CARTESIAN_POINT('Origin',(-42.1957801549596,-58.9348530490817,-400.499999999979));
#37339=CARTESIAN_POINT('',(-43.3549258606093,-84.1739525313094,-400.499999999977));
#37340=CARTESIAN_POINT('Origin',(-42.1957801549596,-58.9348530490817,-400.49999999998));
#37341=CARTESIAN_POINT('',(-43.3549258606094,-84.1739525313095,-400.499999999977));
#37342=CARTESIAN_POINT('Origin',(-7.49122985865824E-11,859.831,-400.500000000088));
#37343=CARTESIAN_POINT('',(43.3549258606242,-84.1739525313017,-400.499999999978));
#37344=CARTESIAN_POINT('',(43.3549258606243,-84.1739525313017,-400.499999999977));
#37345=CARTESIAN_POINT('Origin',(-7.49122985865824E-11,859.831,-400.500000000087));
#37346=CARTESIAN_POINT('Origin',(42.1957801549702,-58.9348530490743,-400.499999999981));
#37347=CARTESIAN_POINT('',(50.1360642048978,-82.920424767238,-400.499999999978));
#37348=CARTESIAN_POINT('Origin',(42.1957801549702,-58.9348530490743,-400.499999999981));
#37349=CARTESIAN_POINT('Ctrl Pts',(50.1360642048978,-82.920424767238,-400.499999999978));
#37350=CARTESIAN_POINT('Ctrl Pts',(50.1136808326039,-82.7592902839127,-409.666667134936));
#37351=CARTESIAN_POINT('Ctrl Pts',(50.0911533108953,-82.5981495149473,-418.833333808621));
#37352=CARTESIAN_POINT('Ctrl Pts',(50.0684772862795,-82.4370022706321,-427.999999999977));
#37353=CARTESIAN_POINT('Origin',(50.1360642048978,-82.920424767238,-400.499999999978));
#37354=CARTESIAN_POINT('',(58.6898628384902,-83.2938916810294,-400.499999999977));
#37355=CARTESIAN_POINT('',(58.6898628384902,-83.2938916810295,-400.499999999978));
#37356=CARTESIAN_POINT('',(50.1360642048981,-82.920424767238,-400.499999999977));
#37357=CARTESIAN_POINT('Origin',(58.6898628384903,-83.2938916810294,-400.499999999978));
#37358=CARTESIAN_POINT('',(72.1248916810336,-69.8588628384839,-400.499999999979));
#37359=CARTESIAN_POINT('',(72.1248916810336,-69.8588628384839,-400.49999999998));
#37360=CARTESIAN_POINT('',(58.6898628384902,-83.2938916810294,-400.499999999977));
#37361=CARTESIAN_POINT('Origin',(72.1248916810336,-69.8588628384839,-400.49999999998));
#37362=CARTESIAN_POINT('',(71.7514247672407,-61.3050642048926,-400.499999999981));
#37363=CARTESIAN_POINT('Ctrl Pts',(71.7514247672407,-61.3050642048926,-400.499999999981));
#37364=CARTESIAN_POINT('Ctrl Pts',(71.5902902839144,-61.2826808325999,-409.666667134939));
#37365=CARTESIAN_POINT('Ctrl Pts',(71.4291495149477,-61.2601533108924,-418.833333808624));
#37366=CARTESIAN_POINT('Ctrl Pts',(71.2680022706319,-61.2374772862763,-427.999999999981));
#37367=CARTESIAN_POINT('',(72.1248916810336,-69.8588628384839,-400.499999999979));
#37368=CARTESIAN_POINT('Origin',(47.7658530490823,-53.3647801549691,-400.499999999981));
#37369=CARTESIAN_POINT('Origin',(47.7658530490823,-53.3647801549691,-400.499999999981));
#37370=CARTESIAN_POINT('Origin',(47.7658530490691,31.026780154963,-400.499999999991));
#37371=CARTESIAN_POINT('',(71.7491203026103,38.9740220215422,-400.499999999992));
#37372=CARTESIAN_POINT('Origin',(47.7658530490691,31.026780154963,-400.499999999991));
#37373=CARTESIAN_POINT('Ctrl Pts',(71.7491203026103,38.9740220215422,-400.499999999992));
#37374=CARTESIAN_POINT('Ctrl Pts',(71.5880199233528,38.9515086021118,-409.666667134328));
#37375=CARTESIAN_POINT('Ctrl Pts',(71.4269132622027,38.928852118611,-418.833333808083));
#37376=CARTESIAN_POINT('Ctrl Pts',(71.2658001171997,38.906048264694,-428.000000004049));
#37377=CARTESIAN_POINT('Origin',(72.1248916810234,47.5208628384841,-400.499999999993));
#37378=CARTESIAN_POINT('',(72.1248916810234,47.5208628384841,-400.499999999992));
#37379=CARTESIAN_POINT('',(72.1248916810234,47.5208628384841,-400.499999999993));
#37380=CARTESIAN_POINT('',(71.74912030261,38.9740220215367,-400.499999999992));
#37381=CARTESIAN_POINT('Origin',(58.6898628384777,60.9558916810272,-400.499999999994));
#37382=CARTESIAN_POINT('',(58.6898628384777,60.9558916810272,-400.499999999994));
#37383=CARTESIAN_POINT('',(58.6898628384777,60.9558916810272,-400.499999999994));
#37384=CARTESIAN_POINT('',(72.1248916810234,47.5208628384841,-400.499999999992));
#37385=CARTESIAN_POINT('Origin',(52.3435336415238,60.6788049642798,-400.499999999994));
#37386=CARTESIAN_POINT('',(52.3435287413493,60.6788047503336,-400.499999999994));
#37387=CARTESIAN_POINT('Ctrl Pts',(52.3435287413493,60.6788047503336,-400.499999999994));
#37388=CARTESIAN_POINT('Ctrl Pts',(52.3021261363478,60.5168398606716,-409.666667632972));
#37389=CARTESIAN_POINT('Ctrl Pts',(52.260542466553,60.3548670822409,-418.833334310633));
#37390=CARTESIAN_POINT('Ctrl Pts',(52.2187735884339,60.1928862347074,-427.999999999994));
#37391=CARTESIAN_POINT('',(58.6898628384777,60.9558916810272,-400.499999999994));
#37392=CARTESIAN_POINT('Origin',(34.2237874382619,30.7342731118462,-400.49999999999));
#37393=CARTESIAN_POINT('',(42.4847016472408,64.745407999866,-400.499999999994));
#37394=CARTESIAN_POINT('Origin',(34.2237874382619,30.7342731118462,-400.49999999999));
#37395=CARTESIAN_POINT('',(42.4847016472409,64.745407999866,-400.499999999994));
#37396=CARTESIAN_POINT('Origin',(9.74220704108575E-12,-110.169000000006,
-400.499999999973));
#37397=CARTESIAN_POINT('',(-42.4847016472518,64.7454079998587,-400.499999999984));
#37398=CARTESIAN_POINT('',(-42.4847016474569,64.7454080007027,-400.499999950222));
#37399=CARTESIAN_POINT('Origin',(9.74220704108575E-12,-110.169000000006,
-400.499999999973));
#37400=CARTESIAN_POINT('Origin',(-34.223787438267,30.7342731118402,-400.499999999974));
#37401=CARTESIAN_POINT('',(-52.3435287413598,60.6788047503246,-400.499999999984));
#37402=CARTESIAN_POINT('Origin',(-34.223787438267,30.7342731118402,-400.499999999974));
#37403=CARTESIAN_POINT('Ctrl Pts',(-52.3435287413598,60.6788047503246,-400.499999999984));
#37404=CARTESIAN_POINT('Ctrl Pts',(-52.3021261363584,60.5168398606624,-409.666667632968));
#37405=CARTESIAN_POINT('Ctrl Pts',(-52.2605424665637,60.3548670822318,-418.83333431063));
#37406=CARTESIAN_POINT('Ctrl Pts',(-52.2187735884448,60.1928862346983,-427.999999999992));
#37407=CARTESIAN_POINT('Origin',(-52.3435336415342,60.6788049642707,-400.499999999992));
#37408=CARTESIAN_POINT('',(-58.689862838488,60.955891681017,-400.499999999992));
#37409=CARTESIAN_POINT('',(-58.689862838488,60.955891681017,-400.499999999992));
#37410=CARTESIAN_POINT('',(-52.3435287413607,60.6788047503247,-400.499999999992));
#37411=CARTESIAN_POINT('Origin',(-58.689862838488,60.955891681017,-400.499999999992));
#37412=CARTESIAN_POINT('',(-72.1248916810314,47.5208628384715,-400.499999999991));
#37413=CARTESIAN_POINT('',(-72.1248916810314,47.5208628384715,-400.499999999991));
#37414=CARTESIAN_POINT('',(-58.689862838488,60.955891681017,-400.499999999992));
#37415=CARTESIAN_POINT('Origin',(-72.1248916810314,47.5208628384715,-400.499999999991));
#37416=CARTESIAN_POINT('',(-71.7514247672385,38.96706420488,-400.49999999999));
#37417=CARTESIAN_POINT('Ctrl Pts',(-71.7514247672385,38.96706420488,-400.49999999999));
#37418=CARTESIAN_POINT('Ctrl Pts',(-71.5902902839124,38.944680832585,-409.666667134948));
#37419=CARTESIAN_POINT('Ctrl Pts',(-71.4291495149459,38.9221533108755,-418.833333808634));
#37420=CARTESIAN_POINT('Ctrl Pts',(-71.2680022706297,38.8994772862588,-427.99999999999));
#37421=CARTESIAN_POINT('',(-72.1248916810314,47.5208628384715,-400.499999999991));
#37422=CARTESIAN_POINT('Origin',(-47.7658530490743,31.0267801549546,-400.49999999999));
#37423=CARTESIAN_POINT('',(-73.004952531302,32.1859258606045,-400.499999999989));
#37424=CARTESIAN_POINT('Origin',(-47.7658530490743,31.0267801549546,-400.49999999999));
#37425=CARTESIAN_POINT('',(-73.0049525313019,32.1859258606049,-400.499999999988));
#37426=CARTESIAN_POINT('Origin',(871.,-11.1689999999296,-400.499999999992));
#37427=CARTESIAN_POINT('Origin',(871.,-11.1689999999296,-400.499999999994));
#37428=CARTESIAN_POINT('Origin',(27.7116878364939,71.2000000000341,-71.2599999999948));
#37429=CARTESIAN_POINT('',(28.4333756729939,71.0000000000342,-71.2599999999948));
#37430=CARTESIAN_POINT('',(28.4333756729939,71.2000000000342,-71.2599999999948));
#37431=CARTESIAN_POINT('',(25.5466243269939,71.0000000000339,-71.2599999999948));
#37432=CARTESIAN_POINT('',(25.5466243269939,71.2000000000339,-71.2599999999948));
#37433=CARTESIAN_POINT('',(26.9899999999939,71.0000000000341,-71.2599999999948));
#37434=CARTESIAN_POINT('Origin',(24.8249364905439,71.2000000000337,-72.5099999999948));
#37435=CARTESIAN_POINT('',(24.1032486540939,71.0000000000336,-73.7599999999948));
#37436=CARTESIAN_POINT('',(24.1032486540939,71.2000000000335,-73.7599999999948));
#37437=CARTESIAN_POINT('',(25.5466243269939,71.0000000000339,-71.2599999999948));
#37438=CARTESIAN_POINT('Origin',(24.8249364905439,71.2000000000334,-75.0099999999948));
#37439=CARTESIAN_POINT('',(25.5466243269939,71.0000000000333,-76.2599999999948));
#37440=CARTESIAN_POINT('',(25.5466243269939,71.2000000000333,-76.2599999999948));
#37441=CARTESIAN_POINT('',(24.1032486540939,71.0000000000336,-73.7599999999948));
#37442=CARTESIAN_POINT('Origin',(26.9899999999939,71.2000000000334,-76.2599999999948));
#37443=CARTESIAN_POINT('',(28.4333756729939,71.0000000000336,-76.2599999999948));
#37444=CARTESIAN_POINT('',(28.4333756729939,71.2000000000336,-76.2599999999948));
#37445=CARTESIAN_POINT('',(26.9899999999939,71.0000000000334,-76.2599999999948));
#37446=CARTESIAN_POINT('Origin',(29.1550635094439,71.2000000000338,-75.0099999999948));
#37447=CARTESIAN_POINT('',(29.876751345894,71.0000000000341,-73.7599999999948));
#37448=CARTESIAN_POINT('',(29.8767513458939,71.200000000034,-73.7599999999948));
#37449=CARTESIAN_POINT('',(28.4333756729939,71.0000000000336,-76.2599999999948));
#37450=CARTESIAN_POINT('Origin',(29.1550635094439,71.2000000000341,-72.5099999999948));
#37451=CARTESIAN_POINT('',(29.876751345894,71.0000000000341,-73.7599999999948));
#37452=CARTESIAN_POINT('Origin',(27.7216878364939,71.2000000000299,-108.259999999995));
#37453=CARTESIAN_POINT('',(28.443375672994,71.0000000000299,-108.259999999995));
#37454=CARTESIAN_POINT('',(28.4433756729939,71.2000000000299,-108.259999999995));
#37455=CARTESIAN_POINT('',(25.5566243269939,71.0000000000297,-108.259999999995));
#37456=CARTESIAN_POINT('',(25.5566243269939,71.2000000000296,-108.259999999995));
#37457=CARTESIAN_POINT('',(26.9999999999939,71.0000000000298,-108.259999999995));
#37458=CARTESIAN_POINT('Origin',(24.8349364905439,71.2000000000295,-109.509999999995));
#37459=CARTESIAN_POINT('',(24.1132486540939,71.0000000000293,-110.759999999995));
#37460=CARTESIAN_POINT('',(24.1132486540939,71.2000000000293,-110.759999999995));
#37461=CARTESIAN_POINT('',(25.5566243269939,71.0000000000297,-108.259999999995));
#37462=CARTESIAN_POINT('Origin',(24.8349364905439,71.2000000000291,-112.009999999995));
#37463=CARTESIAN_POINT('',(25.5566243269939,71.0000000000291,-113.259999999995));
#37464=CARTESIAN_POINT('',(25.5566243269939,71.2000000000291,-113.259999999995));
#37465=CARTESIAN_POINT('',(24.1132486540939,71.0000000000293,-110.759999999995));
#37466=CARTESIAN_POINT('Origin',(26.9999999999939,71.2000000000292,-113.259999999995));
#37467=CARTESIAN_POINT('',(28.443375672994,71.0000000000294,-113.259999999995));
#37468=CARTESIAN_POINT('',(28.4433756729939,71.2000000000294,-113.259999999995));
#37469=CARTESIAN_POINT('',(26.9999999999939,71.0000000000292,-113.259999999995));
#37470=CARTESIAN_POINT('Origin',(29.165063509444,71.2000000000295,-112.009999999995));
#37471=CARTESIAN_POINT('',(29.8867513458939,71.0000000000298,-110.759999999995));
#37472=CARTESIAN_POINT('',(29.8867513458939,71.2000000000298,-110.759999999995));
#37473=CARTESIAN_POINT('',(28.443375672994,71.0000000000294,-113.259999999995));
#37474=CARTESIAN_POINT('Origin',(29.165063509444,71.2000000000299,-109.509999999995));
#37475=CARTESIAN_POINT('',(29.8867513458939,71.0000000000298,-110.759999999995));
#37476=CARTESIAN_POINT('Origin',(1.11022302462516E-12,-11.1690000000053,
-392.499999999986));
#37477=CARTESIAN_POINT('',(59.7537315194951,21.2885348647401,-400.499999999989));
#37478=CARTESIAN_POINT('',(59.7537315195008,-43.6265348647421,-400.499999999981));
#37479=CARTESIAN_POINT('Origin',(1.11022302462516E-12,-11.1690000000062,
-400.499999999986));
#37480=CARTESIAN_POINT('',(59.7537315194951,21.2885348647406,-395.499999999989));
#37481=CARTESIAN_POINT('',(59.7537315194951,21.288534864741,-392.499999999989));
#37482=CARTESIAN_POINT('',(59.7537315195008,-43.6265348647416,-395.499999999981));
#37483=CARTESIAN_POINT('Origin',(1.11022302462516E-12,-11.1690000000057,
-395.499999999985));
#37484=CARTESIAN_POINT('',(59.7537315195008,-43.6265348647412,-392.499999999982));
#37485=CARTESIAN_POINT('Origin',(1.11022302462516E-12,-11.1690000000053,
-392.499999999986));
#37486=CARTESIAN_POINT('',(50.0390320947648,47.355313469007,-392.499999999992));
#37487=CARTESIAN_POINT('',(58.524313469004,38.8700320947692,-392.499999999991));
#37488=CARTESIAN_POINT('Origin',(1.11022302462516E-12,-11.1690000000053,
-392.499999999986));
#37489=CARTESIAN_POINT('',(58.524313469004,38.8700320947683,-400.499999999991));
#37490=CARTESIAN_POINT('',(58.524313469004,38.8700320947692,-392.499999999991));
#37491=CARTESIAN_POINT('',(50.0390320947648,47.3553134690061,-400.499999999992));
#37492=CARTESIAN_POINT('Origin',(1.11022302462516E-12,-11.1690000000062,
-400.499999999986));
#37493=CARTESIAN_POINT('',(50.0390320947648,47.355313469007,-392.499999999992));
#37494=CARTESIAN_POINT('Origin',(-1.50000000000603,70.3309999999988,-355.499999999994));
#37495=CARTESIAN_POINT('',(42.499999999994,70.3310000000076,-312.999999999994));
#37496=CARTESIAN_POINT('',(42.499999999994,70.3309999999978,-397.999999999994));
#37497=CARTESIAN_POINT('',(42.499999999994,70.3310000000076,-312.999999999994));
#37498=CARTESIAN_POINT('',(-42.5000000000061,70.3309999999903,-397.999999999994));
#37499=CARTESIAN_POINT('',(42.499999999994,70.3309999999978,-397.999999999994));
#37500=CARTESIAN_POINT('',(-42.5000000000061,70.331,-312.999999999995));
#37501=CARTESIAN_POINT('',(-42.5000000000061,70.331,-312.999999999994));
#37502=CARTESIAN_POINT('',(42.499999999994,70.3310000000076,-312.999999999994));
#37503=CARTESIAN_POINT('Origin',(42.499999999994,70.3309999999978,-397.999999999994));
#37504=CARTESIAN_POINT('',(32.4575348647363,48.5847315194942,-397.999999999992));
#37505=CARTESIAN_POINT('',(42.4999999999959,47.8824939485326,-397.999999999992));
#37506=CARTESIAN_POINT('',(32.4575348647364,48.5847315194942,-397.999999999992));
#37507=CARTESIAN_POINT('',(-32.4575348647446,48.5847315194885,-397.999999999992));
#37508=CARTESIAN_POINT('Origin',(1.11022302462516E-12,-11.1690000000059,
-397.999999999985));
#37509=CARTESIAN_POINT('',(-42.5000000000041,47.8824939485251,-397.999999999992));
#37510=CARTESIAN_POINT('',(-50.0390320947728,47.3553134689976,-397.999999999992));
#37511=CARTESIAN_POINT('',(-42.5000000000061,70.3309999999903,-397.999999999994));
#37512=CARTESIAN_POINT('',(42.499999999994,70.3309999999978,-397.999999999994));
#37513=CARTESIAN_POINT('Origin',(1.11022302462516E-12,-11.1690000000053,
-392.499999999986));
#37514=CARTESIAN_POINT('',(-32.4575348647446,48.5847315194882,-400.499999999992));
#37515=CARTESIAN_POINT('',(-32.4575348647446,48.5847315194891,-392.499999999992));
#37516=CARTESIAN_POINT('',(32.4575348647363,48.5847315194939,-400.499999999992));
#37517=CARTESIAN_POINT('',(32.4575348647364,48.5847315194948,-392.499999999992));
#37518=CARTESIAN_POINT('Origin',(1.11022302462516E-12,-11.1690000000062,
-400.499999999986));
#37519=CARTESIAN_POINT('Origin',(1.11022302462516E-12,-11.1690000000053,
-392.499999999986));
#37520=CARTESIAN_POINT('',(-58.5243134690106,38.8700320947589,-392.499999999991));
#37521=CARTESIAN_POINT('',(-50.0390320947728,47.3553134689982,-392.499999999992));
#37522=CARTESIAN_POINT('Origin',(1.11022302462516E-12,-11.1690000000053,
-392.499999999986));
#37523=CARTESIAN_POINT('',(-50.0390320947728,47.3553134689973,-400.499999999992));
#37524=CARTESIAN_POINT('',(-50.0390320947728,47.3553134689982,-392.499999999992));
#37525=CARTESIAN_POINT('',(-58.5243134690106,38.8700320947581,-400.499999999991));
#37526=CARTESIAN_POINT('Origin',(1.11022302462516E-12,-11.1690000000062,
-400.499999999986));
#37527=CARTESIAN_POINT('',(-58.5243134690106,38.870032094759,-392.499999999991));
#37528=CARTESIAN_POINT('Origin',(1.11022302462516E-12,-11.1690000000053,
-392.499999999986));
#37529=CARTESIAN_POINT('',(-59.753731519493,-43.6265348647525,-400.499999999981));
#37530=CARTESIAN_POINT('',(-59.7537315194986,21.2885348647297,-400.499999999989));
#37531=CARTESIAN_POINT('Origin',(1.11022302462516E-12,-11.1690000000062,
-400.499999999986));
#37532=CARTESIAN_POINT('',(-59.753731519493,-43.626534864752,-395.499999999981));
#37533=CARTESIAN_POINT('',(-59.753731519493,-43.6265348647516,-392.499999999982));
#37534=CARTESIAN_POINT('',(-59.7537315194986,21.2885348647302,-395.499999999989));
#37535=CARTESIAN_POINT('Origin',(1.11022302462516E-12,-11.1690000000057,
-395.499999999985));
#37536=CARTESIAN_POINT('',(-59.7537315194986,21.2885348647306,-392.499999999989));
#37537=CARTESIAN_POINT('Origin',(1.11022302462516E-12,-11.1690000000053,
-392.499999999986));
#37538=CARTESIAN_POINT('',(-50.0390320947626,-69.6933134690176,-392.499999999978));
#37539=CARTESIAN_POINT('',(-58.5243134690019,-61.2080320947798,-392.49999999998));
#37540=CARTESIAN_POINT('Origin',(1.11022302462516E-12,-11.1690000000053,
-392.499999999986));
#37541=CARTESIAN_POINT('',(-58.5243134690019,-61.2080320947807,-400.49999999998));
#37542=CARTESIAN_POINT('',(-58.5243134690019,-61.2080320947798,-392.49999999998));
#37543=CARTESIAN_POINT('',(-50.0390320947626,-69.6933134690185,-400.499999999979));
#37544=CARTESIAN_POINT('Origin',(1.11022302462516E-12,-11.1690000000062,
-400.499999999986));
#37545=CARTESIAN_POINT('',(-50.0390320947626,-69.6933134690176,-392.499999999978));
#37546=CARTESIAN_POINT('Origin',(-47.7658530490666,-53.3647801549749,-400.49999999998));
#37547=CARTESIAN_POINT('',(-58.5243134690019,-61.2080320947808,-400.49999999998));
#37548=CARTESIAN_POINT('',(-59.7537315194986,21.2885348647297,-400.499999999989));
#37549=CARTESIAN_POINT('',(-50.0390320947728,47.3553134689973,-400.499999999992));
#37550=CARTESIAN_POINT('',(32.4575348647364,48.5847315194939,-400.499999999992));
#37551=CARTESIAN_POINT('',(58.524313469004,38.8700320947682,-400.499999999991));
#37552=CARTESIAN_POINT('',(58.5243134690129,-61.2080320947705,-400.49999999998));
#37553=CARTESIAN_POINT('',(59.7537315195008,-43.6265348647421,-400.499999999981));
#37554=CARTESIAN_POINT('',(50.039032094775,-69.6933134690098,-400.499999999979));
#37555=CARTESIAN_POINT('Origin',(1.11022302462516E-12,-11.1690000000062,
-400.499999999986));
#37556=CARTESIAN_POINT('',(50.039032094775,-69.6933134690098,-400.499999999979));
#37557=CARTESIAN_POINT('',(-32.4575348647342,-70.9227315195064,-400.499999999979));
#37558=CARTESIAN_POINT('Origin',(1.11022302462516E-12,-11.1690000000053,
-392.499999999986));
#37559=CARTESIAN_POINT('',(58.5243134690129,-61.2080320947695,-392.49999999998));
#37560=CARTESIAN_POINT('',(50.039032094775,-69.6933134690089,-392.499999999978));
#37561=CARTESIAN_POINT('Origin',(1.11022302462516E-12,-11.1690000000053,
-392.499999999986));
#37562=CARTESIAN_POINT('',(50.039032094775,-69.6933134690089,-392.499999999978));
#37563=CARTESIAN_POINT('',(58.5243134690129,-61.2080320947695,-392.49999999998));
#37564=CARTESIAN_POINT('Origin',(26.9899999999939,71.0000000000338,-73.7599999999948));
#37565=CARTESIAN_POINT('Origin',(26.9999999999939,71.0000000000295,-110.759999999995));
#37566=CARTESIAN_POINT('Origin',(59.7537315195008,-43.6265348647412,-392.499999999982));
#37567=CARTESIAN_POINT('',(58.8129254661913,-57.0806882454319,-395.49999999998));
#37568=CARTESIAN_POINT('',(59.7537315195008,-43.6265348647416,-395.499999999981));
#37569=CARTESIAN_POINT('',(58.8129254661914,-57.0806882454316,-392.49999999998));
#37570=CARTESIAN_POINT('',(58.8129254661913,-57.0806882454319,-395.49999999998));
#37571=CARTESIAN_POINT('',(58.8129254661914,-57.0806882454316,-392.49999999998));
#37572=CARTESIAN_POINT('Origin',(58.524313469004,38.8700320947692,-392.499999999991));
#37573=CARTESIAN_POINT('',(58.8129254661833,34.7426882454313,-392.49999999999));
#37574=CARTESIAN_POINT('',(58.524313469004,38.8700320947692,-392.499999999991));
#37575=CARTESIAN_POINT('',(58.8129254661833,34.7426882454309,-395.49999999999));
#37576=CARTESIAN_POINT('',(58.8129254661833,34.7426882454309,-395.49999999999));
#37577=CARTESIAN_POINT('',(58.8129254661833,34.742688245431,-395.49999999999));
#37578=CARTESIAN_POINT('Origin',(-41.9116882454246,-76.0623577133481,-395.499999999978));
#37579=CARTESIAN_POINT('',(64.8933577133359,34.7426882454314,-395.49999999999));
#37580=CARTESIAN_POINT('',(50.9116882454285,34.7426882454302,-395.49999999999));
#37581=CARTESIAN_POINT('',(68.6020931316032,32.2411146190954,-395.49999999999));
#37582=CARTESIAN_POINT('Origin',(64.8933577133362,30.7426882454314,-395.49999999999));
#37583=CARTESIAN_POINT('',(71.999999999998,23.8310000000006,-395.49999999999));
#37584=CARTESIAN_POINT('',(68.6020931316032,32.2411146190954,-395.49999999999));
#37585=CARTESIAN_POINT('',(72.0000000000041,-46.1689999999994,-395.499999999981));
#37586=CARTESIAN_POINT('',(72.0000000000041,-46.1689999999994,-395.499999999981));
#37587=CARTESIAN_POINT('',(68.6020931316108,-54.5791146190948,-395.499999999981));
#37588=CARTESIAN_POINT('',(68.6020931316108,-54.5791146190948,-395.499999999981));
#37589=CARTESIAN_POINT('',(64.8933577133439,-57.0806882454314,-395.49999999998));
#37590=CARTESIAN_POINT('Origin',(64.8933577133436,-53.0806882454314,-395.499999999981));
#37591=CARTESIAN_POINT('',(50.9116882454365,-57.0806882454326,-395.49999999998));
#37592=CARTESIAN_POINT('Origin',(50.9116882454281,39.7426882454302,-395.499999999991));
#37593=CARTESIAN_POINT('',(45.9116882454281,39.7426882454301,-392.499999999991));
#37594=CARTESIAN_POINT('',(45.9116882454281,39.7426882454482,-235.499999999991));
#37595=CARTESIAN_POINT('',(45.9116882454281,39.7426882454298,-395.499999999991));
#37596=CARTESIAN_POINT('',(50.9116882454285,34.7426882454486,-235.499999999991));
#37597=CARTESIAN_POINT('Origin',(50.9116882454281,39.7426882454486,-235.499999999991));
#37598=CARTESIAN_POINT('',(50.9116882454285,34.7426882454305,-392.49999999999));
#37599=CARTESIAN_POINT('',(50.9116882454285,34.7426882454302,-395.49999999999));
#37600=CARTESIAN_POINT('Origin',(50.9116882454281,39.7426882454305,-392.499999999991));
#37601=CARTESIAN_POINT('Origin',(32.4575348647364,48.5847315194948,-392.499999999992));
#37602=CARTESIAN_POINT('',(42.4999999999959,47.8824939485329,-395.499999999992));
#37603=CARTESIAN_POINT('',(42.4999999999959,47.8824939485424,-312.999999999992));
#37604=CARTESIAN_POINT('',(45.9116882454274,47.6439254661849,-395.499999999992));
#37605=CARTESIAN_POINT('',(42.4999999999959,47.8824939485329,-395.499999999992));
#37606=CARTESIAN_POINT('',(45.9116882454274,47.6439254661853,-392.499999999992));
#37607=CARTESIAN_POINT('',(45.9116882454274,47.6439254661849,-395.499999999992));
#37608=CARTESIAN_POINT('',(45.9116882454274,47.6439254661854,-392.499999999992));
#37609=CARTESIAN_POINT('Origin',(1.11022302462516E-12,-11.1690000000053,
-392.499999999986));
#37610=CARTESIAN_POINT('',(45.9116882454281,39.7426882454301,-392.499999999991));
#37611=CARTESIAN_POINT('',(50.9116882454285,34.7426882454305,-392.49999999999));
#37612=CARTESIAN_POINT('Origin',(-41.9116882454246,-76.0623577133481,-395.499999999978));
#37613=CARTESIAN_POINT('',(43.4101146190902,57.4330931316041,-395.499999999993));
#37614=CARTESIAN_POINT('',(42.4999999999951,57.8008033062343,-395.499999999993));
#37615=CARTESIAN_POINT('',(43.4101146190903,57.433093131604,-395.499999999993));
#37616=CARTESIAN_POINT('',(45.9116882454268,53.7243577133371,-395.499999999993));
#37617=CARTESIAN_POINT('Origin',(41.9116882454268,53.7243577133368,-395.499999999993));
#37618=CARTESIAN_POINT('',(45.9116882454281,39.7426882454298,-395.499999999991));
#37619=CARTESIAN_POINT('',(42.499999999994,70.3309999999981,-395.499999999994));
#37620=CARTESIAN_POINT('Origin',(42.499999999994,70.3310000000076,-312.999999999994));
#37621=CARTESIAN_POINT('',(42.4999999999951,57.8008033062439,-312.999999999993));
#37622=CARTESIAN_POINT('',(42.4999999999951,57.8008033062344,-395.499999999993));
#37623=CARTESIAN_POINT('',(42.499999999994,70.3310000000076,-312.999999999994));
#37624=CARTESIAN_POINT('Origin',(-42.5000000000061,70.331,-312.999999999994));
#37625=CARTESIAN_POINT('',(-42.500000000005,57.8008033062269,-395.499999999993));
#37626=CARTESIAN_POINT('',(-42.500000000005,57.8008033062364,-312.999999999993));
#37627=CARTESIAN_POINT('',(-42.500000000005,57.800803306227,-395.499999999993));
#37628=CARTESIAN_POINT('',(-42.5000000000061,70.331,-312.999999999995));
#37629=CARTESIAN_POINT('',(-42.5000000000041,47.8824939485254,-395.499999999992));
#37630=CARTESIAN_POINT('',(-42.5000000000041,47.8824939485258,-392.499999999992));
#37631=CARTESIAN_POINT('',(-42.4999999999932,-76.0623577133482,-395.499999999978));
#37632=CARTESIAN_POINT('Origin',(42.499999999994,70.3310000000076,-312.999999999994));
#37633=CARTESIAN_POINT('',(-35.0000000000052,60.8310000000008,-312.999999999993));
#37634=CARTESIAN_POINT('',(-43.4101146191,57.433093131606,-312.999999999993));
#37635=CARTESIAN_POINT('',(34.9999999999948,60.8310000000069,-312.999999999993));
#37636=CARTESIAN_POINT('',(34.9999999999948,60.8310000000069,-312.999999999993));
#37637=CARTESIAN_POINT('',(43.4101146190902,57.4330931316135,-312.999999999993));
#37638=CARTESIAN_POINT('Origin',(-50.0390320947728,47.3553134689982,-392.499999999992));
#37639=CARTESIAN_POINT('',(-45.9116882454354,47.6439254661774,-392.499999999992));
#37640=CARTESIAN_POINT('',(-45.9116882454354,47.643925466177,-395.499999999992));
#37641=CARTESIAN_POINT('',(-45.9116882454354,47.6439254661771,-395.499999999992));
#37642=CARTESIAN_POINT('',(-45.9116882454354,47.643925466177,-395.499999999992));
#37643=CARTESIAN_POINT('',(-50.0390320947728,47.3553134689982,-392.499999999992));
#37644=CARTESIAN_POINT('Origin',(-41.9116882454246,-76.0623577133481,-395.499999999978));
#37645=CARTESIAN_POINT('',(-45.911688245436,53.7243577133291,-395.499999999993));
#37646=CARTESIAN_POINT('',(-45.9116882454348,39.7426882454218,-395.499999999991));
#37647=CARTESIAN_POINT('',(-43.4101146191,57.4330931315965,-395.499999999993));
#37648=CARTESIAN_POINT('Origin',(-41.911688245436,53.7243577133295,-395.499999999993));
#37649=CARTESIAN_POINT('',(-43.4101146191,57.4330931315965,-395.499999999993));
#37650=CARTESIAN_POINT('Origin',(-50.9116882454347,39.7426882454213,-395.499999999991));
#37651=CARTESIAN_POINT('',(-50.9116882454343,34.7426882454217,-392.49999999999));
#37652=CARTESIAN_POINT('',(-50.9116882454343,34.7426882454398,-235.499999999991));
#37653=CARTESIAN_POINT('',(-50.9116882454343,34.7426882454213,-395.49999999999));
#37654=CARTESIAN_POINT('',(-45.9116882454348,39.7426882454402,-235.499999999991));
#37655=CARTESIAN_POINT('Origin',(-50.9116882454347,39.7426882454398,-235.499999999991));
#37656=CARTESIAN_POINT('',(-45.9116882454348,39.7426882454221,-392.499999999991));
#37657=CARTESIAN_POINT('',(-45.9116882454348,39.7426882454218,-395.499999999991));
#37658=CARTESIAN_POINT('Origin',(-50.9116882454347,39.7426882454217,-392.499999999991));
#37659=CARTESIAN_POINT('Origin',(-59.7537315194986,21.2885348647306,-392.499999999989));
#37660=CARTESIAN_POINT('',(-58.8129254661891,34.7426882454206,-395.49999999999));
#37661=CARTESIAN_POINT('',(-59.7537315194986,21.2885348647302,-395.499999999989));
#37662=CARTESIAN_POINT('',(-58.8129254661891,34.742688245421,-392.49999999999));
#37663=CARTESIAN_POINT('',(-58.8129254661891,34.7426882454206,-395.49999999999));
#37664=CARTESIAN_POINT('',(-58.8129254661891,34.742688245421,-392.49999999999));
#37665=CARTESIAN_POINT('Origin',(1.11022302462516E-12,-11.1690000000053,
-392.499999999986));
#37666=CARTESIAN_POINT('',(-50.9116882454343,34.7426882454217,-392.49999999999));
#37667=CARTESIAN_POINT('',(-45.9116882454348,39.7426882454221,-392.499999999991));
#37668=CARTESIAN_POINT('Origin',(-58.5243134690019,-61.2080320947798,-392.49999999998));
#37669=CARTESIAN_POINT('',(-58.8129254661811,-57.0806882454418,-392.49999999998));
#37670=CARTESIAN_POINT('',(-58.5243134690019,-61.2080320947798,-392.49999999998));
#37671=CARTESIAN_POINT('',(-58.8129254661811,-57.0806882454422,-395.49999999998));
#37672=CARTESIAN_POINT('',(-58.8129254661811,-57.0806882454422,-395.49999999998));
#37673=CARTESIAN_POINT('',(-58.8129254661811,-57.0806882454422,-395.49999999998));
#37674=CARTESIAN_POINT('Origin',(-41.9116882454246,-76.0623577133481,-395.499999999978));
#37675=CARTESIAN_POINT('',(-64.8933577133337,-57.0806882454427,-395.49999999998));
#37676=CARTESIAN_POINT('',(-50.9116882454263,-57.0806882454415,-395.49999999998));
#37677=CARTESIAN_POINT('',(-68.602093131601,-54.5791146191067,-395.499999999981));
#37678=CARTESIAN_POINT('Origin',(-64.893357713334,-53.0806882454427,-395.499999999981));
#37679=CARTESIAN_POINT('',(-71.9999999999959,-46.1690000000119,-395.499999999981));
#37680=CARTESIAN_POINT('',(-68.602093131601,-54.5791146191067,-395.499999999981));
#37681=CARTESIAN_POINT('',(-72.000000000002,23.8309999999881,-395.49999999999));
#37682=CARTESIAN_POINT('',(-72.000000000002,23.8309999999881,-395.49999999999));
#37683=CARTESIAN_POINT('',(-68.6020931316086,32.2411146190835,-395.49999999999));
#37684=CARTESIAN_POINT('',(-68.6020931316086,32.2411146190835,-395.49999999999));
#37685=CARTESIAN_POINT('',(-64.8933577133417,34.7426882454201,-395.49999999999));
#37686=CARTESIAN_POINT('Origin',(-64.8933577133413,30.7426882454201,-395.49999999999));
#37687=CARTESIAN_POINT('',(-50.9116882454343,34.7426882454213,-395.49999999999));
#37688=CARTESIAN_POINT('Origin',(-50.9116882454259,-62.0806882454415,-395.49999999998));
#37689=CARTESIAN_POINT('',(-45.9116882454259,-62.0806882454407,-392.49999999998));
#37690=CARTESIAN_POINT('',(-45.9116882454259,-62.0806882454226,-235.49999999998));
#37691=CARTESIAN_POINT('',(-45.9116882454259,-62.0806882454411,-395.49999999998));
#37692=CARTESIAN_POINT('',(-50.9116882454263,-57.0806882454231,-235.49999999998));
#37693=CARTESIAN_POINT('Origin',(-50.9116882454259,-62.0806882454231,-235.49999999998));
#37694=CARTESIAN_POINT('',(-50.9116882454263,-57.0806882454411,-392.49999999998));
#37695=CARTESIAN_POINT('',(-50.9116882454263,-57.0806882454415,-395.49999999998));
#37696=CARTESIAN_POINT('Origin',(-50.9116882454259,-62.0806882454412,-392.49999999998));
#37697=CARTESIAN_POINT('Origin',(-32.4575348647342,-70.9227315195055,-392.499999999978));
#37698=CARTESIAN_POINT('',(-45.9116882454252,-69.9819254661964,-395.499999999979));
#37699=CARTESIAN_POINT('',(-32.4575348647341,-70.9227315195058,-395.499999999979));
#37700=CARTESIAN_POINT('',(-45.9116882454252,-69.981925466196,-392.499999999978));
#37701=CARTESIAN_POINT('',(-45.9116882454252,-69.9819254661964,-395.499999999979));
#37702=CARTESIAN_POINT('',(-45.9116882454252,-69.981925466196,-392.499999999978));
#37703=CARTESIAN_POINT('Origin',(1.11022302462516E-12,-11.1690000000053,
-392.499999999986));
#37704=CARTESIAN_POINT('',(-45.9116882454259,-62.0806882454407,-392.49999999998));
#37705=CARTESIAN_POINT('',(-50.9116882454263,-57.0806882454411,-392.49999999998));
#37706=CARTESIAN_POINT('Origin',(50.9116882454369,-62.0806882454326,-395.49999999998));
#37707=CARTESIAN_POINT('',(50.9116882454365,-57.0806882454323,-392.49999999998));
#37708=CARTESIAN_POINT('',(50.9116882454365,-57.0806882454142,-235.49999999998));
#37709=CARTESIAN_POINT('',(50.9116882454365,-57.0806882454326,-395.49999999998));
#37710=CARTESIAN_POINT('',(45.9116882454369,-62.0806882454146,-235.49999999998));
#37711=CARTESIAN_POINT('Origin',(50.9116882454369,-62.0806882454142,-235.49999999998));
#37712=CARTESIAN_POINT('',(45.9116882454369,-62.0806882454327,-392.49999999998));
#37713=CARTESIAN_POINT('',(45.9116882454369,-62.0806882454331,-395.49999999998));
#37714=CARTESIAN_POINT('Origin',(50.9116882454369,-62.0806882454323,-392.49999999998));
#37715=CARTESIAN_POINT('Origin',(1.11022302462516E-12,-11.1690000000053,
-392.499999999986));
#37716=CARTESIAN_POINT('',(50.9116882454365,-57.0806882454323,-392.49999999998));
#37717=CARTESIAN_POINT('',(45.9116882454377,-69.981925466188,-392.499999999978));
#37718=CARTESIAN_POINT('',(45.9116882454369,-62.0806882454327,-392.49999999998));
#37719=CARTESIAN_POINT('',(50.039032094775,-69.6933134690089,-392.499999999978));
#37720=CARTESIAN_POINT('Origin',(50.039032094775,-69.6933134690089,-392.499999999978));
#37721=CARTESIAN_POINT('',(45.9116882454377,-69.9819254661884,-395.499999999979));
#37722=CARTESIAN_POINT('',(45.9116882454377,-69.9819254661884,-395.499999999979));
#37723=CARTESIAN_POINT('',(45.9116882454377,-69.9819254661884,-395.499999999979));
#37724=CARTESIAN_POINT('Origin',(-41.9116882454246,-76.0623577133481,-395.499999999978));
#37725=CARTESIAN_POINT('',(45.9116882454382,-76.0623577133405,-395.499999999978));
#37726=CARTESIAN_POINT('',(45.9116882454369,-62.0806882454331,-395.49999999998));
#37727=CARTESIAN_POINT('',(43.4101146191022,-79.7710931316078,-395.499999999977));
#37728=CARTESIAN_POINT('Origin',(41.9116882454381,-76.0623577133408,-395.499999999978));
#37729=CARTESIAN_POINT('',(35.0000000000074,-83.1690000000026,-395.499999999977));
#37730=CARTESIAN_POINT('',(43.4101146191022,-79.7710931316078,-395.499999999977));
#37731=CARTESIAN_POINT('',(-34.9999999999926,-83.1690000000087,-395.499999999977));
#37732=CARTESIAN_POINT('',(-34.9999999999926,-83.1690000000087,-395.499999999977));
#37733=CARTESIAN_POINT('',(-43.410114619088,-79.7710931316154,-395.499999999977));
#37734=CARTESIAN_POINT('',(-43.4101146190881,-79.7710931316153,-395.499999999977));
#37735=CARTESIAN_POINT('',(-45.9116882454247,-76.0623577133485,-395.499999999978));
#37736=CARTESIAN_POINT('Origin',(-41.9116882454246,-76.0623577133481,-395.499999999978));
#37737=CARTESIAN_POINT('',(-45.9116882454259,-62.0806882454411,-395.49999999998));
#37738=CARTESIAN_POINT('Origin',(-58.8178305978845,-25.7906133403662,-211.686857166486));
#37739=CARTESIAN_POINT('',(-59.591244465674,-33.9502909241456,-201.14447126204));
#37740=CARTESIAN_POINT('',(-59.1711016649654,-32.5796982421243,-203.651996219616));
#37741=CARTESIAN_POINT('',(-59.5912444656741,-33.9502909241456,-201.14447126204));
#37742=CARTESIAN_POINT('',(-57.7748829601655,-33.9034515013528,-205.804258601751));
#37743=CARTESIAN_POINT('',(-59.1711016649654,-32.5796982421241,-203.651996219616));
#37744=CARTESIAN_POINT('',(-56.7988070560068,-36.5977974427891,-205.448996026285));
#37745=CARTESIAN_POINT('',(-57.7748829601653,-33.9034515013528,-205.804258601751));
#37746=CARTESIAN_POINT('',(-57.2189498567156,-37.9683901248104,-202.941471068708));
#37747=CARTESIAN_POINT('',(-56.7988070560068,-36.5977974427891,-205.448996026285));
#37748=CARTESIAN_POINT('',(-58.6151685615154,-36.6446368655819,-200.789208686573));
#37749=CARTESIAN_POINT('',(-57.2189498567156,-37.9683901248105,-202.941471068708));
#37750=CARTESIAN_POINT('',(-58.6151685615154,-36.6446368655819,-200.789208686573));
#37751=CARTESIAN_POINT('Origin',(-1.720845688169E-12,21.037500000044,35.000000000011));
#37752=CARTESIAN_POINT('',(3.96999999999828,21.037500000041,7.00000000001097));
#37753=CARTESIAN_POINT('',(-3.97000000000172,21.0375000000404,7.00000000001097));
#37754=CARTESIAN_POINT('',(-1.720845688169E-12,21.0375000000407,7.00000000001097));
#37755=CARTESIAN_POINT('',(-3.97000000000172,21.0375000000469,63.0000000000109));
#37756=CARTESIAN_POINT('',(-3.97000000000172,21.0375000000436,35.000000000011));
#37757=CARTESIAN_POINT('',(3.96999999999828,21.0375000000475,63.0000000000109));
#37758=CARTESIAN_POINT('',(-1.720845688169E-12,21.0375000000472,63.0000000000109));
#37759=CARTESIAN_POINT('',(3.96999999999828,21.0375000000443,35.000000000011));
#37760=CARTESIAN_POINT('Origin',(8.32667268468867E-13,-8.23124999995205,
70.0000000000143));
#37761=CARTESIAN_POINT('Origin',(1.11022302462516E-12,-11.1689999999872,
-235.499999999986));
#37762=CARTESIAN_POINT('',(50.039032094775,-69.6933134689908,-235.499999999979));
#37763=CARTESIAN_POINT('',(45.9116882454377,-69.9819254661699,-235.499999999979));
#37764=CARTESIAN_POINT('',(50.039032094775,-69.6933134689908,-235.499999999979));
#37765=CARTESIAN_POINT('',(45.9116882454369,-62.0806882454146,-235.49999999998));
#37766=CARTESIAN_POINT('',(58.8129254661914,-57.0806882454135,-235.49999999998));
#37767=CARTESIAN_POINT('',(50.9116882454365,-57.0806882454142,-235.49999999998));
#37768=CARTESIAN_POINT('',(58.5243134690129,-61.2080320947514,-235.49999999998));
#37769=CARTESIAN_POINT('',(58.5243134690129,-61.2080320947515,-235.49999999998));
#37770=CARTESIAN_POINT('Origin',(1.11022302462516E-12,-11.1689999999872,
-235.499999999986));
#37771=CARTESIAN_POINT('Origin',(1.11022302462516E-12,-11.1689999999872,
-235.499999999986));
#37772=CARTESIAN_POINT('',(58.5243134690129,-61.2080320947505,-227.49999999998));
#37773=CARTESIAN_POINT('',(58.5243134690129,-61.2080320947514,-235.49999999998));
#37774=CARTESIAN_POINT('',(50.039032094775,-69.6933134689899,-227.499999999979));
#37775=CARTESIAN_POINT('Origin',(1.11022302462516E-12,-11.1689999999863,
-227.499999999986));
#37776=CARTESIAN_POINT('',(50.039032094775,-69.6933134689908,-235.499999999979));
#37777=CARTESIAN_POINT('Origin',(50.9116882454365,-57.0806882454326,-395.49999999998));
#37778=CARTESIAN_POINT('',(64.8933577133439,-57.0806882454126,-232.49999999998));
#37779=CARTESIAN_POINT('',(64.8933577133439,-57.0806882454314,-395.49999999998));
#37780=CARTESIAN_POINT('',(58.8129254661914,-57.0806882454131,-232.49999999998));
#37781=CARTESIAN_POINT('',(-41.9116882454263,-57.0806882454219,-232.49999999998));
#37782=CARTESIAN_POINT('',(58.8129254661914,-57.0806882454135,-235.49999999998));
#37783=CARTESIAN_POINT('Origin',(64.8933577133436,-53.0806882454314,-395.499999999981));
#37784=CARTESIAN_POINT('',(68.6020931316108,-54.579114619076,-232.499999999981));
#37785=CARTESIAN_POINT('',(68.6020931316108,-54.5791146190948,-395.499999999981));
#37786=CARTESIAN_POINT('Origin',(64.8933577133436,-53.0806882454126,-232.499999999981));
#37787=CARTESIAN_POINT('Origin',(68.6020931316108,-54.5791146190948,-395.499999999981));
#37788=CARTESIAN_POINT('',(72.0000000000041,-46.1689999999806,-232.499999999982));
#37789=CARTESIAN_POINT('',(72.0000000000041,-46.1689999999994,-395.499999999981));
#37790=CARTESIAN_POINT('',(68.6020931316108,-54.579114619076,-232.499999999981));
#37791=CARTESIAN_POINT('Origin',(72.0000000000041,-46.1689999999994,-395.499999999981));
#37792=CARTESIAN_POINT('',(71.999999999998,23.8310000000193,-232.49999999999));
#37793=CARTESIAN_POINT('',(71.999999999998,23.8310000000006,-395.49999999999));
#37794=CARTESIAN_POINT('',(72.0000000000068,-76.0623577133194,-232.499999999978));
#37795=CARTESIAN_POINT('Origin',(68.6020931316032,32.2411146190954,-395.49999999999));
#37796=CARTESIAN_POINT('',(68.6020931316032,32.2411146191142,-232.499999999991));
#37797=CARTESIAN_POINT('',(68.6020931316032,32.2411146190954,-395.49999999999));
#37798=CARTESIAN_POINT('',(71.999999999998,23.8310000000194,-232.49999999999));
#37799=CARTESIAN_POINT('Origin',(64.8933577133362,30.7426882454314,-395.49999999999));
#37800=CARTESIAN_POINT('',(64.8933577133359,34.7426882454502,-232.499999999991));
#37801=CARTESIAN_POINT('',(64.8933577133359,34.7426882454314,-395.49999999999));
#37802=CARTESIAN_POINT('Origin',(64.8933577133362,30.7426882454502,-232.49999999999));
#37803=CARTESIAN_POINT('Origin',(50.9116882454285,34.7426882454302,-395.49999999999));
#37804=CARTESIAN_POINT('',(58.8129254661834,34.7426882454493,-235.499999999991));
#37805=CARTESIAN_POINT('',(-2.91433543964104E-12,34.7426882454442,-235.499999999991));
#37806=CARTESIAN_POINT('',(58.8129254661834,34.7426882454497,-232.499999999991));
#37807=CARTESIAN_POINT('',(58.8129254661834,34.7426882454493,-235.499999999991));
#37808=CARTESIAN_POINT('',(-41.9116882454343,34.7426882454409,-232.499999999991));
#37809=CARTESIAN_POINT('Origin',(1.11022302462516E-12,-11.1689999999872,
-235.499999999986));
#37810=CARTESIAN_POINT('',(58.5243134690041,38.8700320947872,-235.499999999991));
#37811=CARTESIAN_POINT('',(58.5243134690041,38.8700320947873,-235.499999999991));
#37812=CARTESIAN_POINT('',(45.9116882454274,47.6439254662035,-235.499999999992));
#37813=CARTESIAN_POINT('',(45.9116882454281,39.7426882454482,-235.499999999991));
#37814=CARTESIAN_POINT('',(50.0390320947648,47.355313469025,-235.499999999992));
#37815=CARTESIAN_POINT('',(50.0390320947648,47.355313469025,-235.499999999992));
#37816=CARTESIAN_POINT('Origin',(1.11022302462516E-12,-11.1689999999872,
-235.499999999986));
#37817=CARTESIAN_POINT('Origin',(1.11022302462516E-12,-11.1689999999872,
-235.499999999986));
#37818=CARTESIAN_POINT('',(50.0390320947648,47.355313469026,-227.499999999992));
#37819=CARTESIAN_POINT('',(50.0390320947648,47.355313469025,-235.499999999992));
#37820=CARTESIAN_POINT('',(58.5243134690041,38.8700320947882,-227.499999999991));
#37821=CARTESIAN_POINT('Origin',(1.11022302462516E-12,-11.1689999999863,
-227.499999999986));
#37822=CARTESIAN_POINT('',(58.5243134690041,38.8700320947873,-235.499999999991));
#37823=CARTESIAN_POINT('Origin',(45.9116882454281,39.7426882454298,-395.499999999991));
#37824=CARTESIAN_POINT('',(45.9116882454268,53.7243577133559,-232.499999999993));
#37825=CARTESIAN_POINT('',(45.9116882454268,53.7243577133371,-395.499999999993));
#37826=CARTESIAN_POINT('',(45.9116882454274,47.6439254662038,-232.499999999992));
#37827=CARTESIAN_POINT('',(45.9116882454382,-76.0623577133217,-232.499999999978));
#37828=CARTESIAN_POINT('',(45.9116882454274,47.6439254662035,-235.499999999992));
#37829=CARTESIAN_POINT('Origin',(41.9116882454268,53.7243577133368,-395.499999999993));
#37830=CARTESIAN_POINT('',(43.4101146190902,57.4330931316228,-232.499999999993));
#37831=CARTESIAN_POINT('',(43.4101146190902,57.433093131604,-395.499999999993));
#37832=CARTESIAN_POINT('Origin',(41.9116882454268,53.7243577133556,-232.499999999993));
#37833=CARTESIAN_POINT('Origin',(43.4101146190902,57.433093131604,-395.499999999993));
#37834=CARTESIAN_POINT('',(34.9999999999948,60.8310000000162,-232.499999999994));
#37835=CARTESIAN_POINT('',(34.9999999999948,60.8309999999974,-395.499999999994));
#37836=CARTESIAN_POINT('',(43.4101146190903,57.4330931316228,-232.499999999993));
#37837=CARTESIAN_POINT('Origin',(34.9999999999948,60.8309999999974,-395.499999999994));
#37838=CARTESIAN_POINT('',(-35.0000000000052,60.8310000000101,-232.499999999994));
#37839=CARTESIAN_POINT('',(-35.0000000000052,60.8309999999913,-395.499999999994));
#37840=CARTESIAN_POINT('',(-41.9116882454366,60.8310000000095,-232.499999999994));
#37841=CARTESIAN_POINT('Origin',(-43.4101146191,57.4330931315965,-395.499999999993));
#37842=CARTESIAN_POINT('',(-43.4101146191,57.4330931316153,-232.499999999993));
#37843=CARTESIAN_POINT('',(-43.4101146191,57.4330931315965,-395.499999999993));
#37844=CARTESIAN_POINT('',(-35.0000000000052,60.8310000000101,-232.499999999994));
#37845=CARTESIAN_POINT('Origin',(-41.911688245436,53.7243577133295,-395.499999999993));
#37846=CARTESIAN_POINT('',(-45.911688245436,53.7243577133479,-232.499999999993));
#37847=CARTESIAN_POINT('',(-45.911688245436,53.7243577133291,-395.499999999993));
#37848=CARTESIAN_POINT('Origin',(-41.911688245436,53.7243577133483,-232.499999999993));
#37849=CARTESIAN_POINT('Origin',(-45.9116882454348,39.7426882454218,-395.499999999991));
#37850=CARTESIAN_POINT('',(-45.9116882454354,47.6439254661955,-235.499999999992));
#37851=CARTESIAN_POINT('',(-45.9116882454303,-11.1689999999912,-235.499999999986));
#37852=CARTESIAN_POINT('',(-45.9116882454354,47.6439254661958,-232.499999999992));
#37853=CARTESIAN_POINT('',(-45.9116882454354,47.6439254661955,-235.499999999992));
#37854=CARTESIAN_POINT('',(-45.9116882454247,-76.0623577133297,-232.499999999978));
#37855=CARTESIAN_POINT('Origin',(1.11022302462516E-12,-11.1689999999872,
-235.499999999986));
#37856=CARTESIAN_POINT('',(-50.0390320947728,47.3553134690163,-235.499999999992));
#37857=CARTESIAN_POINT('',(-50.0390320947728,47.3553134690163,-235.499999999992));
#37858=CARTESIAN_POINT('',(-58.8129254661892,34.7426882454391,-235.499999999991));
#37859=CARTESIAN_POINT('',(-50.9116882454343,34.7426882454398,-235.499999999991));
#37860=CARTESIAN_POINT('',(-58.5243134690107,38.870032094777,-235.499999999991));
#37861=CARTESIAN_POINT('',(-58.5243134690107,38.870032094777,-235.499999999991));
#37862=CARTESIAN_POINT('Origin',(1.11022302462516E-12,-11.1689999999872,
-235.499999999986));
#37863=CARTESIAN_POINT('Origin',(1.11022302462516E-12,-11.1689999999872,
-235.499999999986));
#37864=CARTESIAN_POINT('',(-58.5243134690107,38.870032094778,-227.499999999991));
#37865=CARTESIAN_POINT('',(-58.5243134690107,38.870032094777,-235.499999999991));
#37866=CARTESIAN_POINT('',(-50.0390320947728,47.3553134690172,-227.499999999992));
#37867=CARTESIAN_POINT('Origin',(1.11022302462516E-12,-11.1689999999863,
-227.499999999986));
#37868=CARTESIAN_POINT('',(-50.0390320947728,47.3553134690163,-235.499999999992));
#37869=CARTESIAN_POINT('Origin',(-50.9116882454343,34.7426882454213,-395.49999999999));
#37870=CARTESIAN_POINT('',(-64.8933577133417,34.7426882454388,-232.499999999991));
#37871=CARTESIAN_POINT('',(-64.8933577133417,34.7426882454201,-395.49999999999));
#37872=CARTESIAN_POINT('',(-58.8129254661891,34.7426882454394,-232.499999999991));
#37873=CARTESIAN_POINT('',(-41.9116882454343,34.7426882454409,-232.499999999991));
#37874=CARTESIAN_POINT('',(-58.8129254661892,34.7426882454391,-235.499999999991));
#37875=CARTESIAN_POINT('Origin',(-64.8933577133413,30.7426882454201,-395.49999999999));
#37876=CARTESIAN_POINT('',(-68.6020931316086,32.2411146191022,-232.499999999991));
#37877=CARTESIAN_POINT('',(-68.6020931316086,32.2411146190835,-395.49999999999));
#37878=CARTESIAN_POINT('Origin',(-64.8933577133413,30.7426882454389,-232.49999999999));
#37879=CARTESIAN_POINT('Origin',(-68.6020931316086,32.2411146190835,-395.49999999999));
#37880=CARTESIAN_POINT('',(-72.000000000002,23.8310000000068,-232.49999999999));
#37881=CARTESIAN_POINT('',(-72.000000000002,23.8309999999881,-395.49999999999));
#37882=CARTESIAN_POINT('',(-68.6020931316086,32.2411146191022,-232.499999999991));
#37883=CARTESIAN_POINT('Origin',(-72.000000000002,23.8309999999881,-395.49999999999));
#37884=CARTESIAN_POINT('',(-71.9999999999959,-46.1689999999932,-232.499999999982));
#37885=CARTESIAN_POINT('',(-71.9999999999959,-46.1690000000119,-395.499999999981));
#37886=CARTESIAN_POINT('',(-71.9999999999933,-76.062357713332,-232.499999999978));
#37887=CARTESIAN_POINT('Origin',(-68.602093131601,-54.5791146191067,-395.499999999981));
#37888=CARTESIAN_POINT('',(-68.602093131601,-54.579114619088,-232.499999999981));
#37889=CARTESIAN_POINT('',(-68.602093131601,-54.5791146191068,-395.499999999981));
#37890=CARTESIAN_POINT('',(-71.9999999999959,-46.1689999999932,-232.499999999982));
#37891=CARTESIAN_POINT('Origin',(-64.893357713334,-53.0806882454427,-395.499999999981));
#37892=CARTESIAN_POINT('',(-64.8933577133337,-57.0806882454239,-232.49999999998));
#37893=CARTESIAN_POINT('',(-64.8933577133337,-57.0806882454427,-395.49999999998));
#37894=CARTESIAN_POINT('Origin',(-64.893357713334,-53.0806882454239,-232.499999999981));
#37895=CARTESIAN_POINT('Origin',(-50.9116882454263,-57.0806882454415,-395.49999999998));
#37896=CARTESIAN_POINT('',(-58.8129254661811,-57.0806882454238,-235.49999999998));
#37897=CARTESIAN_POINT('',(5.10702591327572E-12,-57.0806882454186,-235.49999999998));
#37898=CARTESIAN_POINT('',(-58.8129254661811,-57.0806882454234,-232.49999999998));
#37899=CARTESIAN_POINT('',(-58.8129254661812,-57.0806882454238,-235.49999999998));
#37900=CARTESIAN_POINT('',(-41.9116882454263,-57.0806882454219,-232.49999999998));
#37901=CARTESIAN_POINT('Origin',(1.11022302462516E-12,-11.1689999999872,
-235.499999999986));
#37902=CARTESIAN_POINT('',(-58.5243134690019,-61.2080320947617,-235.49999999998));
#37903=CARTESIAN_POINT('',(-58.5243134690019,-61.2080320947617,-235.49999999998));
#37904=CARTESIAN_POINT('',(-45.9116882454252,-69.9819254661779,-235.499999999979));
#37905=CARTESIAN_POINT('',(-45.9116882454259,-62.0806882454226,-235.49999999998));
#37906=CARTESIAN_POINT('',(-50.0390320947626,-69.6933134689995,-235.499999999979));
#37907=CARTESIAN_POINT('',(-50.0390320947626,-69.6933134689995,-235.499999999979));
#37908=CARTESIAN_POINT('Origin',(1.11022302462516E-12,-11.1689999999872,
-235.499999999986));
#37909=CARTESIAN_POINT('Origin',(1.11022302462516E-12,-11.1689999999872,
-235.499999999986));
#37910=CARTESIAN_POINT('',(-50.0390320947626,-69.6933134689986,-227.499999999979));
#37911=CARTESIAN_POINT('',(-50.0390320947626,-69.6933134689995,-235.499999999979));
#37912=CARTESIAN_POINT('',(-58.5243134690019,-61.2080320947608,-227.49999999998));
#37913=CARTESIAN_POINT('Origin',(1.11022302462516E-12,-11.1689999999863,
-227.499999999986));
#37914=CARTESIAN_POINT('',(-58.5243134690019,-61.2080320947617,-235.49999999998));
#37915=CARTESIAN_POINT('Origin',(-45.9116882454259,-62.0806882454411,-395.49999999998));
#37916=CARTESIAN_POINT('',(-45.9116882454246,-76.0623577133297,-232.499999999978));
#37917=CARTESIAN_POINT('',(-45.9116882454246,-76.0623577133485,-395.499999999978));
#37918=CARTESIAN_POINT('',(-45.9116882454252,-69.9819254661776,-232.499999999979));
#37919=CARTESIAN_POINT('',(-45.9116882454247,-76.0623577133297,-232.499999999978));
#37920=CARTESIAN_POINT('',(-45.9116882454252,-69.9819254661779,-235.499999999979));
#37921=CARTESIAN_POINT('Origin',(-41.9116882454246,-76.0623577133481,-395.499999999978));
#37922=CARTESIAN_POINT('',(-43.410114619088,-79.7710931315966,-232.499999999978));
#37923=CARTESIAN_POINT('',(-43.4101146190881,-79.7710931316153,-395.499999999977));
#37924=CARTESIAN_POINT('Origin',(-41.9116882454246,-76.0623577133294,-232.499999999978));
#37925=CARTESIAN_POINT('Origin',(-43.4101146190881,-79.7710931316153,-395.499999999977));
#37926=CARTESIAN_POINT('',(-34.9999999999926,-83.1689999999899,-232.499999999977));
#37927=CARTESIAN_POINT('',(-34.9999999999926,-83.1690000000087,-395.499999999977));
#37928=CARTESIAN_POINT('',(-43.4101146190881,-79.7710931315966,-232.499999999978));
#37929=CARTESIAN_POINT('Origin',(-34.9999999999926,-83.1690000000087,-395.499999999977));
#37930=CARTESIAN_POINT('',(35.0000000000075,-83.1689999999838,-232.499999999977));
#37931=CARTESIAN_POINT('',(35.0000000000074,-83.1690000000026,-395.499999999977));
#37932=CARTESIAN_POINT('',(-41.911688245424,-83.1689999999905,-232.499999999977));
#37933=CARTESIAN_POINT('Origin',(43.4101146191022,-79.7710931316078,-395.499999999977));
#37934=CARTESIAN_POINT('',(43.4101146191022,-79.771093131589,-232.499999999978));
#37935=CARTESIAN_POINT('',(43.4101146191022,-79.7710931316078,-395.499999999977));
#37936=CARTESIAN_POINT('',(35.0000000000074,-83.1689999999838,-232.499999999977));
#37937=CARTESIAN_POINT('Origin',(41.9116882454381,-76.0623577133408,-395.499999999978));
#37938=CARTESIAN_POINT('',(45.9116882454382,-76.0623577133217,-232.499999999978));
#37939=CARTESIAN_POINT('',(45.9116882454382,-76.0623577133405,-395.499999999978));
#37940=CARTESIAN_POINT('Origin',(41.9116882454381,-76.062357713322,-232.499999999978));
#37941=CARTESIAN_POINT('Origin',(45.9116882454369,-62.0806882454331,-395.49999999998));
#37942=CARTESIAN_POINT('',(45.9116882454377,-69.9819254661696,-232.499999999979));
#37943=CARTESIAN_POINT('',(45.9116882454377,-69.9819254661699,-235.499999999979));
#37944=CARTESIAN_POINT('',(45.9116882454382,-76.0623577133217,-232.499999999978));
#37945=CARTESIAN_POINT('Origin',(-62.7912238833522,-36.1419811084888,-202.309168520235));
#37946=CARTESIAN_POINT('',(-62.0126566584211,-38.1422389714875,-202.02579322501));
#37947=CARTESIAN_POINT('',(-58.6151685615155,-36.644636865582,-200.789208686573));
#37948=CARTESIAN_POINT('',(-63.0507462916694,-35.4752284874923,-202.403626951979));
#37949=CARTESIAN_POINT('',(-63.0507462916927,-35.4752284875026,-202.403626951987));
#37950=CARTESIAN_POINT('',(-63.0507462916617,-35.4752284874888,-202.403626951975));
#37951=CARTESIAN_POINT('Origin',(-61.3256090710095,-38.8089915924427,-203.10595056927));
#37952=CARTESIAN_POINT('',(-60.6385614835859,-39.4757442133925,-204.186107913527));
#37953=CARTESIAN_POINT('',(-57.2189498567157,-37.9683901248103,-202.941471068708));
#37954=CARTESIAN_POINT('',(-62.0126566584124,-38.1422389714836,-202.025793225006));
#37955=CARTESIAN_POINT('Origin',(-60.4705587127634,-38.8089915924429,-205.45518212126));
#37956=CARTESIAN_POINT('',(-60.3025559419268,-38.1422389714871,-206.724256328988));
#37957=CARTESIAN_POINT('',(-56.7988070560067,-36.5977974427891,-205.448996026285));
#37958=CARTESIAN_POINT('',(-60.6385614835583,-39.4757442133804,-204.186107913517));
#37959=CARTESIAN_POINT('Origin',(-60.8216007585505,-36.8087337294892,-206.913173192472));
#37960=CARTESIAN_POINT('',(-61.3406455751751,-35.4752284874919,-207.102090055957));
#37961=CARTESIAN_POINT('',(-57.7748829601656,-33.9034515013526,-205.804258601751));
#37962=CARTESIAN_POINT('',(-60.3025559419125,-38.1422389714808,-206.724256328982));
#37963=CARTESIAN_POINT('Origin',(-62.0276931625839,-34.8084758665355,-206.021932711695));
#37964=CARTESIAN_POINT('',(-62.7147407500105,-34.1417232455869,-204.941775367439));
#37965=CARTESIAN_POINT('',(-59.1711016649653,-32.5796982421245,-203.651996219616));
#37966=CARTESIAN_POINT('',(-61.3406455751928,-35.4752284874997,-207.102090055963));
#37967=CARTESIAN_POINT('Origin',(-62.8827435208299,-34.8084758665353,-203.672701159705));
#37968=CARTESIAN_POINT('',(-62.7147407500469,-34.141723245603,-204.941775367452));
#37969=CARTESIAN_POINT('Origin',(26.9899999999942,67.0000000000338,-73.7599999999943));
#37970=CARTESIAN_POINT('Origin',(26.9999999999943,67.0000000000297,-110.759999999994));
#37971=CARTESIAN_POINT('Origin',(-3.9700000000008,10.5187500000436,35.0000000000122));
#37972=CARTESIAN_POINT('',(-3.9700000000008,10.5187500000468,63.0000000000122));
#37973=CARTESIAN_POINT('',(-3.9700000000008,10.5187500000404,7.00000000001219));
#37974=CARTESIAN_POINT('Origin',(-8.04911692853239E-13,10.5187500000407,
7.00000000001219));
#37975=CARTESIAN_POINT('',(3.96999999999919,10.518750000041,7.00000000001219));
#37976=CARTESIAN_POINT('Origin',(3.96999999999919,10.5187500000443,35.0000000000122));
#37977=CARTESIAN_POINT('',(3.96999999999919,10.5187500000475,63.0000000000122));
#37978=CARTESIAN_POINT('Origin',(-8.04911692853239E-13,10.5187500000472,
63.0000000000122));
#37979=CARTESIAN_POINT('Origin',(-64.9999999999989,-11.1689999999867,-181.499999999986));
#37980=CARTESIAN_POINT('Origin',(-4.57966997657877E-12,53.831000000019,
-181.499999999993));
#37981=CARTESIAN_POINT('Origin',(65.0000000000011,-11.1689999999753,-181.499999999986));
#37982=CARTESIAN_POINT('Origin',(6.77236045021346E-12,-76.168999999981,
-181.499999999978));
#37983=CARTESIAN_POINT('Origin',(50.039032094775,-69.6933134689908,-235.499999999979));
#37984=CARTESIAN_POINT('',(32.4575348647468,-70.9227315194807,-227.499999999979));
#37985=CARTESIAN_POINT('',(50.039032094775,-69.6933134689898,-227.499999999979));
#37986=CARTESIAN_POINT('',(32.4575348647468,-70.9227315194813,-232.499999999979));
#37987=CARTESIAN_POINT('',(32.4575348647468,-70.9227315194816,-235.499999999979));
#37988=CARTESIAN_POINT('',(45.9116882454377,-69.9819254661696,-232.499999999979));
#37989=CARTESIAN_POINT('Origin',(1.11022302462516E-12,-11.1689999999863,
-227.499999999986));
#37990=CARTESIAN_POINT('',(58.1696747238672,-60.8533933496047,-227.49999999998));
#37991=CARTESIAN_POINT('',(59.3192302506027,-44.413983418182,-227.499999999982));
#37992=CARTESIAN_POINT('',(59.3192302506027,-44.4139834181821,-227.499999999982));
#37993=CARTESIAN_POINT('',(49.6843933496294,-69.338674723844,-227.499999999979));
#37994=CARTESIAN_POINT('Origin',(1.11022302462516E-12,-11.1689999999863,
-227.499999999986));
#37995=CARTESIAN_POINT('',(33.2449834182068,-70.4882302505823,-227.499999999979));
#37996=CARTESIAN_POINT('',(33.2449834182068,-70.4882302505823,-227.499999999979));
#37997=CARTESIAN_POINT('Origin',(1.11022302462516E-12,-11.1689999999863,
-227.499999999986));
#37998=CARTESIAN_POINT('',(59.7537315195009,-43.6265348647221,-227.499999999982));
#37999=CARTESIAN_POINT('',(58.5243134690129,-61.2080320947506,-227.49999999998));
#38000=CARTESIAN_POINT('Origin',(1.11022302462516E-12,-11.1689999999863,
-227.499999999986));
#38001=CARTESIAN_POINT('Origin',(58.5243134690129,-61.2080320947515,-235.49999999998));
#38002=CARTESIAN_POINT('',(59.7537315195008,-43.6265348647228,-232.499999999982));
#38003=CARTESIAN_POINT('',(59.7537315195008,-43.6265348647228,-232.499999999982));
#38004=CARTESIAN_POINT('',(59.7537315195008,-43.6265348647231,-235.499999999981));
#38005=CARTESIAN_POINT('Origin',(-41.9116882454246,-76.0623577133294,-232.499999999978));
#38006=CARTESIAN_POINT('',(59.7537315194952,21.2885348647593,-232.499999999989));
#38007=CARTESIAN_POINT('',(58.5243134690041,38.8700320947876,-232.499999999991));
#38008=CARTESIAN_POINT('Origin',(1.11022302462516E-12,-11.1689999999869,
-232.499999999986));
#38009=CARTESIAN_POINT('Origin',(58.5243134690041,38.8700320947873,-235.499999999991));
#38010=CARTESIAN_POINT('',(59.7537315194952,21.2885348647599,-227.499999999989));
#38011=CARTESIAN_POINT('',(58.5243134690041,38.8700320947882,-227.499999999991));
#38012=CARTESIAN_POINT('',(59.7537315194952,21.2885348647591,-235.499999999989));
#38013=CARTESIAN_POINT('Origin',(1.11022302462516E-12,-11.1689999999863,
-227.499999999986));
#38014=CARTESIAN_POINT('',(49.6843933496193,47.0006747238801,-227.499999999992));
#38015=CARTESIAN_POINT('',(33.2449834181965,48.1502302506155,-227.499999999992));
#38016=CARTESIAN_POINT('',(58.1696747238586,38.5153933496423,-227.499999999991));
#38017=CARTESIAN_POINT('Origin',(1.11022302462516E-12,-11.1689999999863,
-227.499999999986));
#38018=CARTESIAN_POINT('',(59.3192302505969,22.0759834182197,-227.499999999989));
#38019=CARTESIAN_POINT('',(59.3192302505969,22.0759834182197,-227.499999999989));
#38020=CARTESIAN_POINT('Origin',(1.11022302462516E-12,-11.1689999999863,
-227.499999999986));
#38021=CARTESIAN_POINT('',(50.0390320947648,47.355313469026,-227.499999999992));
#38022=CARTESIAN_POINT('Origin',(50.0390320947648,47.355313469025,-235.499999999992));
#38023=CARTESIAN_POINT('',(32.4575348647364,48.5847315195132,-232.499999999992));
#38024=CARTESIAN_POINT('Origin',(-41.9116882454246,-76.0623577133294,-232.499999999978));
#38025=CARTESIAN_POINT('',(-50.0390320947728,47.3553134690167,-232.499999999992));
#38026=CARTESIAN_POINT('Origin',(-50.0390320947728,47.3553134690163,-235.499999999992));
#38027=CARTESIAN_POINT('',(-50.0390320947728,47.3553134690172,-227.499999999992));
#38028=CARTESIAN_POINT('Origin',(1.11022302462516E-12,-11.1689999999863,
-227.499999999986));
#38029=CARTESIAN_POINT('',(-59.7537315194987,21.2885348647495,-227.499999999989));
#38030=CARTESIAN_POINT('',(-58.5243134690107,38.870032094778,-227.499999999991));
#38031=CARTESIAN_POINT('',(-59.3192302506006,22.0759834182094,-227.499999999989));
#38032=CARTESIAN_POINT('Origin',(1.11022302462516E-12,-11.1689999999863,
-227.499999999986));
#38033=CARTESIAN_POINT('',(-58.169674723865,38.5153933496321,-227.499999999991));
#38034=CARTESIAN_POINT('',(-59.3192302506005,22.0759834182094,-227.499999999989));
#38035=CARTESIAN_POINT('',(-49.6843933496272,47.0006747238714,-227.499999999992));
#38036=CARTESIAN_POINT('Origin',(1.11022302462516E-12,-11.1689999999863,
-227.499999999986));
#38037=CARTESIAN_POINT('',(-33.2449834182046,48.1502302506097,-227.499999999992));
#38038=CARTESIAN_POINT('Origin',(-58.5243134690107,38.870032094777,-235.499999999991));
#38039=CARTESIAN_POINT('',(-59.7537315194986,21.288534864749,-232.499999999989));
#38040=CARTESIAN_POINT('',(-59.7537315194986,21.288534864749,-232.499999999989));
#38041=CARTESIAN_POINT('',(-59.7537315194986,21.2885348647486,-235.499999999989));
#38042=CARTESIAN_POINT('Origin',(-41.9116882454246,-76.0623577133294,-232.499999999978));
#38043=CARTESIAN_POINT('',(-59.753731519493,-43.6265348647331,-232.499999999982));
#38044=CARTESIAN_POINT('',(-58.5243134690019,-61.2080320947614,-232.49999999998));
#38045=CARTESIAN_POINT('Origin',(1.11022302462516E-12,-11.1689999999869,
-232.499999999986));
#38046=CARTESIAN_POINT('Origin',(-58.5243134690019,-61.2080320947617,-235.49999999998));
#38047=CARTESIAN_POINT('',(-59.753731519493,-43.6265348647326,-227.499999999982));
#38048=CARTESIAN_POINT('',(-58.5243134690019,-61.2080320947608,-227.49999999998));
#38049=CARTESIAN_POINT('',(-59.753731519493,-43.6265348647336,-235.499999999981));
#38050=CARTESIAN_POINT('Origin',(1.11022302462516E-12,-11.1689999999863,
-227.499999999986));
#38051=CARTESIAN_POINT('',(-32.4575348647341,-70.9227315194864,-227.499999999979));
#38052=CARTESIAN_POINT('',(-50.0390320947626,-69.6933134689986,-227.499999999979));
#38053=CARTESIAN_POINT('',(-33.2449834181943,-70.4882302505881,-227.499999999979));
#38054=CARTESIAN_POINT('Origin',(1.11022302462516E-12,-11.1689999999863,
-227.499999999986));
#38055=CARTESIAN_POINT('',(-49.6843933496171,-69.3386747238527,-227.499999999979));
#38056=CARTESIAN_POINT('',(-33.2449834181943,-70.4882302505881,-227.499999999979));
#38057=CARTESIAN_POINT('',(-58.1696747238564,-60.8533933496149,-227.49999999998));
#38058=CARTESIAN_POINT('Origin',(1.11022302462516E-12,-11.1689999999863,
-227.499999999986));
#38059=CARTESIAN_POINT('',(-59.3192302505947,-44.4139834181924,-227.499999999982));
#38060=CARTESIAN_POINT('',(-59.3192302505947,-44.4139834181924,-227.499999999982));
#38061=CARTESIAN_POINT('Origin',(1.11022302462516E-12,-11.1689999999863,
-227.499999999986));
#38062=CARTESIAN_POINT('Origin',(-50.0390320947626,-69.6933134689995,-235.499999999979));
#38063=CARTESIAN_POINT('',(-32.4575348647341,-70.922731519487,-232.499999999979));
#38064=CARTESIAN_POINT('',(-32.4575348647342,-70.922731519487,-232.499999999979));
#38065=CARTESIAN_POINT('',(-32.4575348647341,-70.9227315194873,-235.499999999979));
#38066=CARTESIAN_POINT('Origin',(-41.9116882454246,-76.0623577133294,-232.499999999978));
#38067=CARTESIAN_POINT('Origin',(1.11022302462516E-12,-11.1689999999869,
-232.499999999986));
#38068=CARTESIAN_POINT('Origin',(-60.650590686874,-36.8087337296458,-207.383019502761));
#38069=CARTESIAN_POINT('Origin',(-6.02295990859147E-12,70.5000000000294,
-92.2599999999947));
#38070=CARTESIAN_POINT('',(4.88675134594208,70.5000000000261,-126.259999999995));
#38071=CARTESIAN_POINT('',(7.7735026918902,70.5000000000257,-131.259999999995));
#38072=CARTESIAN_POINT('',(4.88675134594205,70.5000000000261,-126.259999999995));
#38073=CARTESIAN_POINT('',(4.8867513459421,70.500000000025,-136.259999999995));
#38074=CARTESIAN_POINT('',(7.77350269189023,70.5000000000257,-131.259999999995));
#38075=CARTESIAN_POINT('',(-0.886751345954173,70.5000000000245,-136.259999999995));
#38076=CARTESIAN_POINT('',(4.88675134594208,70.500000000025,-136.259999999995));
#38077=CARTESIAN_POINT('',(-3.77350269190227,70.5000000000247,-131.259999999995));
#38078=CARTESIAN_POINT('',(-0.886751345954173,70.5000000000245,-136.259999999995));
#38079=CARTESIAN_POINT('',(-0.886751345954145,70.5000000000256,-126.259999999995));
#38080=CARTESIAN_POINT('',(-3.77350269190227,70.5000000000247,-131.259999999995));
#38081=CARTESIAN_POINT('',(-0.886751345954145,70.5000000000256,-126.259999999995));
#38082=CARTESIAN_POINT('Origin',(33.2449834182068,-70.48823025058,-207.499999999936));
#38083=CARTESIAN_POINT('',(49.6843933496294,-69.3386747238393,-186.499999999978));
#38084=CARTESIAN_POINT('',(33.2449834182068,-70.48823025058,-207.499999999936));
#38085=CARTESIAN_POINT('Origin',(1.11022302462516E-12,-11.1689999999816,
-186.499999999986));
#38086=CARTESIAN_POINT('',(58.1696747238672,-60.8533933496024,-207.499999999937));
#38087=CARTESIAN_POINT('Origin',(59.3192302506027,-44.4139834181798,-207.499999999939));
#38088=CARTESIAN_POINT('',(59.3192302506028,-44.4139834181829,-235.499999999981));
#38089=CARTESIAN_POINT('Origin',(1.11022302462516E-12,-11.1689999999872,
-235.499999999986));
#38090=CARTESIAN_POINT('',(59.3192302505969,22.075983418222,-207.499999999946));
#38091=CARTESIAN_POINT('Origin',(59.3192302505969,22.075983418222,-207.499999999946));
#38092=CARTESIAN_POINT('',(58.1696747238586,38.515393349647,-186.499999999991));
#38093=CARTESIAN_POINT('Origin',(1.11022302462516E-12,-11.1689999999816,
-186.499999999986));
#38094=CARTESIAN_POINT('',(49.6843933496193,47.0006747238824,-207.499999999949));
#38095=CARTESIAN_POINT('Origin',(33.2449834181965,48.1502302506178,-207.499999999949));
#38096=CARTESIAN_POINT('Origin',(-33.2449834182046,48.150230250612,-207.499999999949));
#38097=CARTESIAN_POINT('',(-49.6843933496272,47.0006747238761,-186.499999999992));
#38098=CARTESIAN_POINT('Origin',(1.11022302462516E-12,-11.1689999999816,
-186.499999999986));
#38099=CARTESIAN_POINT('',(-58.169674723865,38.5153933496345,-207.499999999948));
#38100=CARTESIAN_POINT('Origin',(-59.3192302506005,22.0759834182117,-207.499999999946));
#38101=CARTESIAN_POINT('',(-59.3192302506006,22.0759834182084,-235.499999999989));
#38102=CARTESIAN_POINT('Origin',(1.11022302462516E-12,-11.1689999999872,
-235.499999999986));
#38103=CARTESIAN_POINT('',(-59.3192302505947,-44.41398341819,-207.499999999939));
#38104=CARTESIAN_POINT('Origin',(-59.3192302505947,-44.4139834181901,-207.499999999939));
#38105=CARTESIAN_POINT('',(-58.1696747238564,-60.8533933496102,-186.499999999979));
#38106=CARTESIAN_POINT('Origin',(1.11022302462516E-12,-11.1689999999816,
-186.499999999986));
#38107=CARTESIAN_POINT('',(-49.6843933496171,-69.3386747238504,-207.499999999936));
#38108=CARTESIAN_POINT('Origin',(-33.2449834181943,-70.4882302505858,-207.499999999936));
#38109=CARTESIAN_POINT('',(-33.2449834181943,-70.488230250589,-235.499999999979));
#38110=CARTESIAN_POINT('Origin',(1.11022302462516E-12,-11.1689999999872,
-235.499999999986));
#38111=CARTESIAN_POINT('Origin',(37.489999999994,70.500000000036,-63.2599999999947));
#38112=CARTESIAN_POINT('',(35.999999999994,70.5000000000358,-63.2599999999947));
#38113=CARTESIAN_POINT('',(17.9999999999939,70.5000000000342,-63.2599999999947));
#38114=CARTESIAN_POINT('',(37.489999999994,70.500000000036,-63.2599999999947));
#38115=CARTESIAN_POINT('',(37.489999999994,70.500000000036,-63.2599999999947));
#38116=CARTESIAN_POINT('',(37.489999999994,70.500000000036,-63.2599999999947));
#38117=CARTESIAN_POINT('',(37.489999999994,70.5000000000336,-84.2599999999947));
#38118=CARTESIAN_POINT('',(37.489999999994,70.500000000036,-63.2599999999948));
#38119=CARTESIAN_POINT('',(35.999999999994,70.5000000000335,-84.2599999999948));
#38120=CARTESIAN_POINT('',(37.489999999994,70.5000000000336,-84.2599999999948));
#38121=CARTESIAN_POINT('',(17.9999999999939,70.5000000000319,-84.2599999999948));
#38122=CARTESIAN_POINT('',(37.489999999994,70.5000000000336,-84.2599999999948));
#38123=CARTESIAN_POINT('',(16.489999999994,70.5000000000317,-84.2599999999948));
#38124=CARTESIAN_POINT('',(37.489999999994,70.5000000000336,-84.2599999999947));
#38125=CARTESIAN_POINT('',(16.489999999994,70.5000000000342,-63.2599999999947));
#38126=CARTESIAN_POINT('',(16.489999999994,70.5000000000342,-63.2599999999948));
#38127=CARTESIAN_POINT('',(37.489999999994,70.500000000036,-63.2599999999947));
#38128=CARTESIAN_POINT('Origin',(37.4899999999976,29.8015151901986,-84.2599999999901));
#38129=CARTESIAN_POINT('Origin',(35.999999999995,58.5000000000335,-84.2599999999934));
#38130=CARTESIAN_POINT('Origin',(17.999999999995,58.5000000000319,-84.2599999999934));
#38131=CARTESIAN_POINT('Origin',(16.4999999999975,29.801515190195,-100.25999999999));
#38132=CARTESIAN_POINT('',(35.999999999994,70.5000000000317,-100.259999999995));
#38133=CARTESIAN_POINT('Origin',(35.999999999995,58.5000000000317,-100.259999999993));
#38134=CARTESIAN_POINT('',(17.9999999999939,70.5000000000301,-100.259999999995));
#38135=CARTESIAN_POINT('',(37.4999999999939,70.5000000000318,-100.259999999995));
#38136=CARTESIAN_POINT('Origin',(17.999999999995,58.5000000000301,-100.259999999993));
#38137=CARTESIAN_POINT('Origin',(37.4999999999939,70.5000000000318,-100.259999999995));
#38138=CARTESIAN_POINT('',(37.4999999999939,70.5000000000295,-121.259999999995));
#38139=CARTESIAN_POINT('',(37.4999999999939,70.5000000000319,-100.259999999995));
#38140=CARTESIAN_POINT('',(37.4999999999939,70.5000000000319,-100.259999999995));
#38141=CARTESIAN_POINT('',(35.999999999994,70.5000000000294,-121.259999999995));
#38142=CARTESIAN_POINT('',(16.4999999999939,70.5000000000277,-121.259999999995));
#38143=CARTESIAN_POINT('',(17.9999999999939,70.5000000000278,-121.259999999995));
#38144=CARTESIAN_POINT('',(16.4999999999939,70.5000000000277,-121.259999999995));
#38145=CARTESIAN_POINT('',(16.4999999999939,70.5000000000276,-121.259999999995));
#38146=CARTESIAN_POINT('',(37.4999999999939,70.5000000000295,-121.259999999995));
#38147=CARTESIAN_POINT('',(16.4999999999939,70.50000000003,-100.259999999995));
#38148=CARTESIAN_POINT('',(16.4999999999939,70.50000000003,-100.259999999995));
#38149=CARTESIAN_POINT('',(16.4999999999939,70.50000000003,-100.259999999995));
#38150=CARTESIAN_POINT('',(16.4999999999939,70.50000000003,-100.259999999995));
#38151=CARTESIAN_POINT('Origin',(-6.02295990859147E-12,70.5000000000294,
-92.2599999999947));
#38152=CARTESIAN_POINT('',(4.8867513459421,70.5000000000348,-48.2599999999947));
#38153=CARTESIAN_POINT('',(7.77350269189023,70.5000000000344,-53.2599999999947));
#38154=CARTESIAN_POINT('',(4.88675134594208,70.5000000000348,-48.2599999999946));
#38155=CARTESIAN_POINT('',(4.88675134594208,70.5000000000336,-58.2599999999947));
#38156=CARTESIAN_POINT('',(7.77350269189026,70.5000000000344,-53.2599999999946));
#38157=CARTESIAN_POINT('',(-0.886751345954145,70.5000000000331,-58.2599999999947));
#38158=CARTESIAN_POINT('',(4.88675134594208,70.5000000000336,-58.2599999999947));
#38159=CARTESIAN_POINT('',(-3.7735026919023,70.5000000000334,-53.2599999999947));
#38160=CARTESIAN_POINT('',(-0.886751345954173,70.5000000000331,-58.2599999999946));
#38161=CARTESIAN_POINT('',(-0.886751345954173,70.5000000000343,-48.2599999999947));
#38162=CARTESIAN_POINT('',(-3.77350269190227,70.5000000000334,-53.2599999999946));
#38163=CARTESIAN_POINT('',(-0.886751345954145,70.5000000000343,-48.2599999999946));
#38164=CARTESIAN_POINT('Origin',(-4.96824803519758E-12,58.5000000000244,
-137.259999999993));
#38165=CARTESIAN_POINT('Ctrl Pts',(4.499999999994,69.6242977306701,-121.577541634476));
#38166=CARTESIAN_POINT('Ctrl Pts',(3.69670943613483,69.9492447632731,-121.370132902743));
#38167=CARTESIAN_POINT('Ctrl Pts',(2.8492207351751,70.1886150627173,-121.259999999995));
#38168=CARTESIAN_POINT('Ctrl Pts',(1.3641526653201,70.439637382277,-121.259999999995));
#38169=CARTESIAN_POINT('Ctrl Pts',(0.706314881107781,70.496946126364,-121.32175471629));
#38170=CARTESIAN_POINT('Ctrl Pts',(-0.598427958263334,70.5028113810441,
-121.580614035387));
#38171=CARTESIAN_POINT('Ctrl Pts',(-1.24533966867664,70.4515055296131,-121.777681955094));
#38172=CARTESIAN_POINT('Ctrl Pts',(-2.83779978405687,70.2014113531424,-122.444371841402));
#38173=CARTESIAN_POINT('Ctrl Pts',(-3.73964423272937,69.9318767829018,-123.010297347601));
#38174=CARTESIAN_POINT('Ctrl Pts',(-4.50000000000616,69.6242977306689,-123.660657923209));
#38175=CARTESIAN_POINT('Origin',(-3.7735026919036,85.7752523165442,-131.259999999996));
#38176=CARTESIAN_POINT('',(-3.77350269190194,66.5000000000247,-131.259999999994));
#38177=CARTESIAN_POINT('',(-3.7735026919036,85.7752523165442,-131.259999999996));
#38178=CARTESIAN_POINT('',(-0.886751345953785,66.5000000000256,-126.259999999994));
#38179=CARTESIAN_POINT('',(-3.77350269190197,66.5000000000247,-131.259999999994));
#38180=CARTESIAN_POINT('',(-0.886751345955478,85.775252316545,-126.259999999996));
#38181=CARTESIAN_POINT('Origin',(-0.886751345955478,85.775252316545,-126.259999999996));
#38182=CARTESIAN_POINT('',(4.88675134594241,66.5000000000261,-126.259999999994));
#38183=CARTESIAN_POINT('',(18.1658075373038,66.5000000000273,-126.259999999994));
#38184=CARTESIAN_POINT('',(4.88675134594074,85.7752523165455,-126.259999999996));
#38185=CARTESIAN_POINT('Origin',(4.88675134594074,85.7752523165455,-126.259999999996));
#38186=CARTESIAN_POINT('',(7.77350269189056,66.5000000000257,-131.259999999994));
#38187=CARTESIAN_POINT('',(4.88675134594244,66.5000000000261,-126.259999999994));
#38188=CARTESIAN_POINT('',(7.7735026918889,85.7752523165452,-131.259999999996));
#38189=CARTESIAN_POINT('Origin',(7.77350269188887,85.7752523165452,-131.259999999996));
#38190=CARTESIAN_POINT('',(4.88675134594244,66.5000000000249,-136.259999999994));
#38191=CARTESIAN_POINT('',(7.77350269189056,66.5000000000257,-131.259999999994));
#38192=CARTESIAN_POINT('',(4.88675134594074,85.7752523165443,-136.259999999996));
#38193=CARTESIAN_POINT('Origin',(4.88675134594074,85.7752523165443,-136.259999999996));
#38194=CARTESIAN_POINT('',(-0.886751345953812,66.5000000000244,-136.259999999994));
#38195=CARTESIAN_POINT('',(18.1658075373038,66.5000000000261,-136.259999999994));
#38196=CARTESIAN_POINT('',(-0.886751345955478,85.7752523165438,-136.259999999996));
#38197=CARTESIAN_POINT('Origin',(-0.886751345955478,85.7752523165438,-136.259999999996));
#38198=CARTESIAN_POINT('',(-0.886751345953812,66.5000000000244,-136.259999999994));
#38199=CARTESIAN_POINT('Origin',(1.99999999999398,70.5000000000252,-131.259999999995));
#38200=CARTESIAN_POINT('',(10.6602540378387,66.5000000000266,-126.259999999994));
#38201=CARTESIAN_POINT('',(10.6602540378383,70.5000000000266,-126.259999999995));
#38202=CARTESIAN_POINT('',(-6.66025403785003,66.5000000000251,-126.259999999994));
#38203=CARTESIAN_POINT('Origin',(1.99999999999431,66.5000000000253,-131.259999999994));
#38204=CARTESIAN_POINT('',(-6.66025403785042,70.5000000000251,-126.259999999995));
#38205=CARTESIAN_POINT('Origin',(16.4999999999975,29.8015151901927,-121.25999999999));
#38206=CARTESIAN_POINT('Origin',(35.999999999995,58.5000000000293,-121.259999999993));
#38207=CARTESIAN_POINT('Origin',(17.999999999995,58.5000000000277,-121.259999999993));
#38208=CARTESIAN_POINT('Origin',(1.11022302462516E-13,3.99005915113771E-11,
1.34059430223488E-11));
#38209=CARTESIAN_POINT('Origin',(1.11022302462516E-12,-11.1689999999816,
-186.499999999986));
#38210=CARTESIAN_POINT('Origin',(1.11022302462516E-12,-11.1689999999816,
-186.499999999986));
#38211=CARTESIAN_POINT('Origin',(1.11022302462516E-12,-11.1689999999816,
-186.499999999986));
#38212=CARTESIAN_POINT('Origin',(1.11022302462516E-12,-11.1689999999816,
-186.499999999986));
#38213=CARTESIAN_POINT('Origin',(-54.7313488832587,-33.7472662704153,-202.036058359604));
#38214=CARTESIAN_POINT('',(-60.4268711256452,-32.5555280806013,-200.48984153347));
#38215=CARTESIAN_POINT('',(-55.9721573516798,-38.3905798567208,-205.662355821745));
#38216=CARTESIAN_POINT('Origin',(-58.1950257608648,-35.2740441835029,-203.296733644063));
#38217=CARTESIAN_POINT('Origin',(-58.2040000000278,-35.2780000000023,-203.299999999994));
#38218=CARTESIAN_POINT('Origin',(-56.2373841760092,-35.2780000001109,-208.70323256955));
#38219=CARTESIAN_POINT('',(-61.668735249239,-30.9288598303501,-199.047872363434));
#38220=CARTESIAN_POINT('',(-55.9721573516797,-38.390579856721,-205.662355821745));
#38221=CARTESIAN_POINT('Origin',(-88.6,2.20815119661433E-11,-87.4999999999866));
#38222=CARTESIAN_POINT('',(-88.6,-1.44337567297821,-89.9999999999864));
#38223=CARTESIAN_POINT('',(-88.6,-2.88675134587792,-87.4999999999863));
#38224=CARTESIAN_POINT('',(-88.6,-2.16506350942806,-88.7499999999863));
#38225=CARTESIAN_POINT('',(-88.6,-1.44337567297763,-84.9999999999864));
#38226=CARTESIAN_POINT('',(-88.6,-2.16506350942778,-86.2499999999863));
#38227=CARTESIAN_POINT('',(-88.6,1.44337567302237,-84.9999999999868));
#38228=CARTESIAN_POINT('',(-88.6,2.23590677222995E-11,-84.9999999999866));
#38229=CARTESIAN_POINT('',(-88.6,2.88675134592208,-87.4999999999869));
#38230=CARTESIAN_POINT('',(-88.6,2.16506350947222,-86.2499999999868));
#38231=CARTESIAN_POINT('',(-88.6,1.44337567302179,-89.9999999999867));
#38232=CARTESIAN_POINT('',(-88.6,2.16506350947194,-88.7499999999868));
#38233=CARTESIAN_POINT('',(-88.6,-0.721687836478203,-89.9999999999865));
#38234=CARTESIAN_POINT('Origin',(-6.02295990859147E-12,70.5000000000294,
-92.2599999999947));
#38235=CARTESIAN_POINT('',(-66.1132486540579,70.5000000000198,-126.259999999995));
#38236=CARTESIAN_POINT('',(-63.2264973081098,70.5000000000196,-131.259999999995));
#38237=CARTESIAN_POINT('',(-66.113248654058,70.5000000000198,-126.259999999995));
#38238=CARTESIAN_POINT('',(-66.1132486540579,70.5000000000187,-136.259999999995));
#38239=CARTESIAN_POINT('',(-63.2264973081098,70.5000000000196,-131.259999999995));
#38240=CARTESIAN_POINT('',(-71.8867513459542,70.5000000000182,-136.259999999995));
#38241=CARTESIAN_POINT('',(-66.1132486540579,70.5000000000187,-136.259999999995));
#38242=CARTESIAN_POINT('',(-74.7735026919022,70.5000000000185,-131.259999999995));
#38243=CARTESIAN_POINT('',(-71.8867513459543,70.5000000000182,-136.259999999995));
#38244=CARTESIAN_POINT('',(-71.8867513459541,70.5000000000193,-126.259999999995));
#38245=CARTESIAN_POINT('',(-74.7735026919022,70.5000000000185,-131.259999999995));
#38246=CARTESIAN_POINT('',(-71.8867513459541,70.5000000000194,-126.259999999995));
#38247=CARTESIAN_POINT('Origin',(-6.02295990859147E-12,70.5000000000294,
-92.2599999999947));
#38248=CARTESIAN_POINT('',(-66.1132486540579,70.5000000000286,-48.2599999999947));
#38249=CARTESIAN_POINT('',(-63.2264973081098,70.5000000000283,-53.2599999999947));
#38250=CARTESIAN_POINT('',(-66.113248654058,70.5000000000286,-48.2599999999946));
#38251=CARTESIAN_POINT('',(-66.1132486540579,70.5000000000274,-58.2599999999947));
#38252=CARTESIAN_POINT('',(-63.2264973081098,70.5000000000283,-53.2599999999946));
#38253=CARTESIAN_POINT('',(-71.8867513459541,70.5000000000269,-58.2599999999947));
#38254=CARTESIAN_POINT('',(-66.1132486540579,70.5000000000274,-58.2599999999947));
#38255=CARTESIAN_POINT('',(-74.7735026919022,70.5000000000272,-53.2599999999947));
#38256=CARTESIAN_POINT('',(-71.8867513459542,70.5000000000269,-58.2599999999946));
#38257=CARTESIAN_POINT('',(-71.8867513459541,70.5000000000281,-48.2599999999947));
#38258=CARTESIAN_POINT('',(-74.7735026919022,70.5000000000272,-53.2599999999946));
#38259=CARTESIAN_POINT('',(-71.8867513459541,70.5000000000281,-48.2599999999946));
#38260=CARTESIAN_POINT('Origin',(16.4999999999975,29.8015151901927,-121.25999999999));
#38261=CARTESIAN_POINT('',(37.4999999999939,70.4058808998202,-121.259999999995));
#38262=CARTESIAN_POINT('Origin',(35.999999999995,58.5000000000293,-121.259999999993));
#38263=CARTESIAN_POINT('',(37.4999999999975,29.8015151901944,-121.25999999999));
#38264=CARTESIAN_POINT('Origin',(37.4999999999975,29.8015151901968,-100.25999999999));
#38265=CARTESIAN_POINT('',(37.4999999999939,70.4058808998225,-100.259999999995));
#38266=CARTESIAN_POINT('',(37.4999999999975,29.8015151901968,-100.25999999999));
#38267=CARTESIAN_POINT('',(37.4999999999939,70.4058808998183,-137.259999999995));
#38268=CARTESIAN_POINT('Origin',(16.4999999999975,29.801515190195,-100.25999999999));
#38269=CARTESIAN_POINT('Origin',(35.999999999995,58.5000000000317,-100.259999999993));
#38270=CARTESIAN_POINT('Origin',(37.4899999999976,29.8015151901986,-84.2599999999901));
#38271=CARTESIAN_POINT('',(37.489999999994,70.407136515586,-84.2599999999947));
#38272=CARTESIAN_POINT('Origin',(35.999999999995,58.5000000000335,-84.2599999999934));
#38273=CARTESIAN_POINT('',(37.4899999999976,29.8015151901986,-84.25999999999));
#38274=CARTESIAN_POINT('Origin',(37.4899999999976,29.801515190201,-63.2599999999901));
#38275=CARTESIAN_POINT('',(37.489999999994,70.4071365155883,-63.2599999999947));
#38276=CARTESIAN_POINT('',(37.4899999999976,29.801515190201,-63.2599999999901));
#38277=CARTESIAN_POINT('',(37.489999999994,70.40713651558,-137.259999999995));
#38278=CARTESIAN_POINT('Origin',(37.4899999999976,29.801515190201,-63.2599999999901));
#38279=CARTESIAN_POINT('Origin',(35.999999999995,58.5000000000358,-63.2599999999934));
#38280=CARTESIAN_POINT('Origin',(37.4899999999976,29.801515190201,-63.2599999999901));
#38281=CARTESIAN_POINT('Origin',(35.999999999995,58.5000000000358,-63.2599999999934));
#38282=CARTESIAN_POINT('Origin',(17.999999999995,58.5000000000342,-63.2599999999934));
#38283=CARTESIAN_POINT('Origin',(37.4899999999976,29.801515190201,-63.2599999999901));
#38284=CARTESIAN_POINT('',(16.489999999994,70.4046167515302,-63.2599999999947));
#38285=CARTESIAN_POINT('Origin',(17.999999999995,58.5000000000342,-63.2599999999934));
#38286=CARTESIAN_POINT('',(16.4899999999976,29.8015151901991,-63.25999999999));
#38287=CARTESIAN_POINT('Origin',(16.4899999999976,29.8015151901991,-63.2599999999901));
#38288=CARTESIAN_POINT('',(16.489999999994,70.4046167515278,-84.2599999999947));
#38289=CARTESIAN_POINT('',(16.4899999999976,29.8015151901967,-84.2599999999901));
#38290=CARTESIAN_POINT('',(16.489999999994,70.4046167515219,-137.259999999995));
#38291=CARTESIAN_POINT('Origin',(37.4899999999976,29.8015151901986,-84.2599999999901));
#38292=CARTESIAN_POINT('Origin',(17.999999999995,58.5000000000319,-84.2599999999934));
#38293=CARTESIAN_POINT('Origin',(16.4999999999975,29.801515190195,-100.25999999999));
#38294=CARTESIAN_POINT('',(16.499999999994,70.4058808998207,-100.259999999995));
#38295=CARTESIAN_POINT('Origin',(17.999999999995,58.5000000000301,-100.259999999993));
#38296=CARTESIAN_POINT('',(16.4999999999975,29.801515190195,-100.25999999999));
#38297=CARTESIAN_POINT('Origin',(16.4999999999975,29.801515190195,-100.25999999999));
#38298=CARTESIAN_POINT('',(16.499999999994,70.4058808998183,-121.259999999995));
#38299=CARTESIAN_POINT('',(16.4999999999975,29.8015151901927,-121.25999999999));
#38300=CARTESIAN_POINT('',(16.499999999994,70.4058808998165,-137.259999999995));
#38301=CARTESIAN_POINT('Origin',(16.4999999999975,29.8015151901927,-121.25999999999));
#38302=CARTESIAN_POINT('Origin',(17.999999999995,58.5000000000277,-121.259999999993));
#38303=CARTESIAN_POINT('Origin',(-3.7735026919036,85.7752523165529,-53.2599999999964));
#38304=CARTESIAN_POINT('',(-3.77350269190194,66.5000000000334,-53.2599999999943));
#38305=CARTESIAN_POINT('',(-3.77350269190358,85.7752523165529,-53.2599999999965));
#38306=CARTESIAN_POINT('',(-0.886751345953812,66.5000000000343,-48.2599999999942));
#38307=CARTESIAN_POINT('',(-0.886751345953812,66.5000000000343,-48.2599999999943));
#38308=CARTESIAN_POINT('',(-0.886751345955478,85.7752523165537,-48.2599999999964));
#38309=CARTESIAN_POINT('Origin',(-0.886751345955478,85.7752523165526,-58.2599999999964));
#38310=CARTESIAN_POINT('',(-0.886751345953812,66.5000000000331,-58.2599999999942));
#38311=CARTESIAN_POINT('',(-0.886751345955478,85.7752523165526,-58.2599999999964));
#38312=CARTESIAN_POINT('',(-3.77350269190194,66.5000000000334,-53.2599999999943));
#38313=CARTESIAN_POINT('Origin',(4.88675134594074,85.7752523165531,-58.2599999999964));
#38314=CARTESIAN_POINT('',(4.88675134594244,66.5000000000336,-58.2599999999942));
#38315=CARTESIAN_POINT('',(4.88675134594072,85.7752523165531,-58.2599999999965));
#38316=CARTESIAN_POINT('',(1.99999999999431,66.5000000000334,-58.2599999999943));
#38317=CARTESIAN_POINT('Origin',(7.7735026918889,85.7752523165539,-53.2599999999964));
#38318=CARTESIAN_POINT('',(7.77350269189056,66.5000000000344,-53.2599999999942));
#38319=CARTESIAN_POINT('',(7.77350269188895,85.7752523165538,-53.2599999999965));
#38320=CARTESIAN_POINT('',(4.88675134594244,66.5000000000337,-58.2599999999943));
#38321=CARTESIAN_POINT('Origin',(4.88675134594077,85.7752523165542,-48.2599999999964));
#38322=CARTESIAN_POINT('',(4.88675134594246,66.5000000000348,-48.2599999999942));
#38323=CARTESIAN_POINT('',(4.88675134594077,85.7752523165542,-48.2599999999964));
#38324=CARTESIAN_POINT('',(7.77350269189056,66.5000000000344,-53.2599999999943));
#38325=CARTESIAN_POINT('Origin',(-0.886751345955478,85.7752523165537,-48.2599999999964));
#38326=CARTESIAN_POINT('',(1.99999999999431,66.5000000000345,-48.2599999999943));
#38327=CARTESIAN_POINT('Origin',(-6.66025403785042,70.5000000000251,-126.259999999995));
#38328=CARTESIAN_POINT('',(-12.4337567297464,67.8166247903788,-136.259999999994));
#38329=CARTESIAN_POINT('Origin',(-9.54700538352068,64.4999999997427,-131.259999999512));
#38330=CARTESIAN_POINT('',(-12.4337567297463,66.5000000000234,-136.259999999994));
#38331=CARTESIAN_POINT('',(-6.66025403785006,66.5000000000251,-126.259999999994));
#38332=CARTESIAN_POINT('',(-12.4337567297467,70.5000000000234,-136.259999999995));
#38333=CARTESIAN_POINT('Origin',(-14.1658075373155,70.5000000000234,-135.259999999995));
#38334=CARTESIAN_POINT('',(-13.0456138058833,66.5000000000233,-136.916854249487));
#38335=CARTESIAN_POINT('Origin',(-14.1658075373152,66.5000000000234,-135.259999999994));
#38336=CARTESIAN_POINT('Ctrl Pts',(-12.4337567297465,67.8166247903788,-136.259999999994));
#38337=CARTESIAN_POINT('Ctrl Pts',(-12.527412483404,67.5720741794269,-136.42221652375));
#38338=CARTESIAN_POINT('Ctrl Pts',(-12.6384034068036,67.3227889604539,-136.561022994229));
#38339=CARTESIAN_POINT('Ctrl Pts',(-12.8407204020393,66.8991702874016,-136.763339989465));
#38340=CARTESIAN_POINT('Ctrl Pts',(-12.9396941466076,66.7025491386428,-136.845242314766));
#38341=CARTESIAN_POINT('Ctrl Pts',(-13.0456138058835,66.5000000000234,-136.916854249487));
#38342=CARTESIAN_POINT('Origin',(18.1658075373038,66.5000000000262,-135.259999999994));
#38343=CARTESIAN_POINT('',(16.4337567297349,66.5000000000259,-136.259999999994));
#38344=CARTESIAN_POINT('',(16.4337567297349,66.5000000000259,-136.259999999994));
#38345=CARTESIAN_POINT('',(17.0456138058719,66.500000000026,-136.916854249486));
#38346=CARTESIAN_POINT('Origin',(18.1658075373038,66.5000000000262,-135.259999999994));
#38347=CARTESIAN_POINT('',(74.4999999999943,66.500000000031,-136.916854249487));
#38348=CARTESIAN_POINT('Origin',(18.1658075373035,70.5000000000262,-135.259999999995));
#38349=CARTESIAN_POINT('',(16.4337567297348,67.8166247903813,-136.259999999994));
#38350=CARTESIAN_POINT('',(16.4337567297346,70.5000000000259,-136.259999999995));
#38351=CARTESIAN_POINT('Ctrl Pts',(17.0456138058721,66.5000000000261,-136.916854249487));
#38352=CARTESIAN_POINT('Ctrl Pts',(16.9396941465962,66.7025491386454,-136.845242314766));
#38353=CARTESIAN_POINT('Ctrl Pts',(16.8407204020279,66.8991702874042,-136.763339989465));
#38354=CARTESIAN_POINT('Ctrl Pts',(16.6384034067921,67.3227889604565,-136.561022994229));
#38355=CARTESIAN_POINT('Ctrl Pts',(16.5274124833925,67.5720741794294,-136.42221652375));
#38356=CARTESIAN_POINT('Ctrl Pts',(16.4337567297349,67.8166247903813,-136.259999999994));
#38357=CARTESIAN_POINT('Origin',(16.4337567297346,70.5000000000259,-136.259999999995));
#38358=CARTESIAN_POINT('',(14.8295692198259,70.0736065540853,-133.481465727965));
#38359=CARTESIAN_POINT('Origin',(17.9999999908615,58.5000000268696,-138.972812905301));
#38360=CARTESIAN_POINT('Origin',(13.5470053838188,64.5000000000939,-131.260000000049));
#38361=CARTESIAN_POINT('Origin',(-6.02295990859147E-12,70.5000000000294,
-92.2599999999947));
#38362=CARTESIAN_POINT('',(71.8867513459421,70.5000000000319,-126.259999999995));
#38363=CARTESIAN_POINT('',(74.7735026918903,70.5000000000316,-131.259999999995));
#38364=CARTESIAN_POINT('',(71.8867513459421,70.5000000000319,-126.259999999995));
#38365=CARTESIAN_POINT('',(71.8867513459421,70.5000000000308,-136.259999999995));
#38366=CARTESIAN_POINT('',(74.7735026918903,70.5000000000316,-131.259999999995));
#38367=CARTESIAN_POINT('',(66.1132486540459,70.5000000000303,-136.259999999995));
#38368=CARTESIAN_POINT('',(71.8867513459421,70.5000000000308,-136.259999999995));
#38369=CARTESIAN_POINT('',(63.2264973080978,70.5000000000306,-131.259999999995));
#38370=CARTESIAN_POINT('',(66.1132486540459,70.5000000000303,-136.259999999995));
#38371=CARTESIAN_POINT('',(66.1132486540459,70.5000000000314,-126.259999999995));
#38372=CARTESIAN_POINT('',(63.2264973080978,70.5000000000306,-131.259999999995));
#38373=CARTESIAN_POINT('',(66.1132486540459,70.5000000000314,-126.259999999995));
#38374=CARTESIAN_POINT('Origin',(-6.02295990859147E-12,70.5000000000294,
-92.2599999999947));
#38375=CARTESIAN_POINT('',(71.8867513459421,70.5000000000406,-48.2599999999947));
#38376=CARTESIAN_POINT('',(74.7735026918903,70.5000000000403,-53.2599999999947));
#38377=CARTESIAN_POINT('',(71.8867513459421,70.5000000000406,-48.2599999999946));
#38378=CARTESIAN_POINT('',(71.8867513459421,70.5000000000394,-58.2599999999947));
#38379=CARTESIAN_POINT('',(74.7735026918903,70.5000000000403,-53.2599999999946));
#38380=CARTESIAN_POINT('',(66.1132486540459,70.5000000000389,-58.2599999999947));
#38381=CARTESIAN_POINT('',(71.8867513459421,70.5000000000394,-58.2599999999947));
#38382=CARTESIAN_POINT('',(63.2264973080978,70.5000000000393,-53.2599999999947));
#38383=CARTESIAN_POINT('',(66.1132486540459,70.5000000000389,-58.2599999999946));
#38384=CARTESIAN_POINT('',(66.1132486540459,70.5000000000401,-48.2599999999947));
#38385=CARTESIAN_POINT('',(63.2264973080978,70.5000000000393,-53.2599999999946));
#38386=CARTESIAN_POINT('',(66.1132486540459,70.5000000000401,-48.2599999999946));
#38387=CARTESIAN_POINT('Origin',(88.6000000000047,-51.9999999999593,-60.4999999999806));
#38388=CARTESIAN_POINT('',(88.6000000000048,-53.4433756729591,-57.9999999999804));
#38389=CARTESIAN_POINT('',(88.6000000000049,-54.8867513458593,-60.4999999999803));
#38390=CARTESIAN_POINT('',(88.6000000000049,-54.1650635094092,-59.2499999999804));
#38391=CARTESIAN_POINT('',(88.6000000000048,-53.4433756729596,-62.9999999999804));
#38392=CARTESIAN_POINT('',(88.6000000000049,-54.1650635094095,-61.7499999999804));
#38393=CARTESIAN_POINT('',(88.6000000000045,-50.5566243269596,-62.9999999999808));
#38394=CARTESIAN_POINT('',(88.6000000000047,-52.7216878364596,-62.9999999999805));
#38395=CARTESIAN_POINT('',(88.6000000000044,-49.1132486540593,-60.4999999999809));
#38396=CARTESIAN_POINT('',(88.6000000000045,-49.8349364905095,-61.7499999999809));
#38397=CARTESIAN_POINT('',(88.6000000000045,-50.5566243269591,-57.9999999999808));
#38398=CARTESIAN_POINT('',(88.6000000000045,-49.8349364905092,-59.2499999999809));
#38399=CARTESIAN_POINT('',(88.6000000000047,-51.999999999959,-57.9999999999806));
#38400=CARTESIAN_POINT('Origin',(-44.5975847992976,-39.383454275573,-196.399999999982));
#38401=CARTESIAN_POINT('',(-57.0363320232113,-44.53575207465,-196.499999999982));
#38402=CARTESIAN_POINT('',(-44.8103167727357,-39.4715707441215,-196.499999999982));
#38403=CARTESIAN_POINT('',(-51.9295288153114,-42.4204449255687,-211.686857166484));
#38404=CARTESIAN_POINT('Origin',(-58.8178305978845,-25.7906133403662,-211.686857166486));
#38405=CARTESIAN_POINT('',(-63.9246338057844,-27.9059204894474,-196.499999999984));
#38406=CARTESIAN_POINT('',(-57.0363320232113,-44.53575207465,-196.499999999982));
#38407=CARTESIAN_POINT('',(-63.9246338057844,-27.9059204894474,-196.499999999984));
#38408=CARTESIAN_POINT('Origin',(-51.4858865818706,-22.7536226903704,-196.399999999984));
#38409=CARTESIAN_POINT('',(-63.9246338057844,-27.9059204894474,-196.499999999984));
#38410=CARTESIAN_POINT('Origin',(-66.0000000000025,29.5000000000287,-47.29999999999));
#38411=CARTESIAN_POINT('',(-68.5000000000023,28.0566243270285,-47.2999999999898));
#38412=CARTESIAN_POINT('',(-66.0000000000022,26.6132486541287,-47.2999999999897));
#38413=CARTESIAN_POINT('',(-67.2500000000023,27.3349364905786,-47.2999999999897));
#38414=CARTESIAN_POINT('',(-63.5000000000023,28.0566243270289,-47.2999999999898));
#38415=CARTESIAN_POINT('',(-64.7500000000023,27.3349364905788,-47.2999999999897));
#38416=CARTESIAN_POINT('',(-63.5000000000026,30.9433756730289,-47.2999999999902));
#38417=CARTESIAN_POINT('',(-63.5000000000025,29.5000000000289,-47.29999999999));
#38418=CARTESIAN_POINT('',(-66.0000000000027,32.3867513459287,-47.2999999999903));
#38419=CARTESIAN_POINT('',(-64.7500000000026,31.6650635094788,-47.2999999999902));
#38420=CARTESIAN_POINT('',(-68.5000000000026,30.9433756730285,-47.2999999999902));
#38421=CARTESIAN_POINT('',(-67.2500000000026,31.6650635094786,-47.2999999999902));
#38422=CARTESIAN_POINT('',(-68.5000000000024,28.7783121635285,-47.2999999999899));
#38423=CARTESIAN_POINT('Origin',(88.2000000000047,-51.9999999999594,-60.4999999999806));
#38424=CARTESIAN_POINT('',(88.2000000000048,-53.4433756729597,-62.9999999999804));
#38425=CARTESIAN_POINT('',(88.2000000000049,-54.8867513458594,-60.4999999999803));
#38426=CARTESIAN_POINT('',(88.2000000000049,-54.1650635094095,-61.7499999999804));
#38427=CARTESIAN_POINT('',(88.2000000000048,-53.4433756729591,-57.9999999999804));
#38428=CARTESIAN_POINT('',(88.2000000000049,-54.1650635094092,-59.2499999999804));
#38429=CARTESIAN_POINT('',(88.2000000000045,-50.5566243269591,-57.9999999999808));
#38430=CARTESIAN_POINT('',(88.2000000000047,-51.9999999999591,-57.9999999999806));
#38431=CARTESIAN_POINT('',(88.2000000000044,-49.1132486540594,-60.4999999999809));
#38432=CARTESIAN_POINT('',(88.2000000000045,-49.8349364905093,-59.2499999999809));
#38433=CARTESIAN_POINT('',(88.2000000000045,-50.5566243269597,-62.9999999999808));
#38434=CARTESIAN_POINT('',(88.2000000000045,-49.8349364905095,-61.7499999999809));
#38435=CARTESIAN_POINT('',(88.2000000000047,-52.7216878364597,-62.9999999999805));
#38436=CARTESIAN_POINT('Origin',(-92.6,-0.721687836478536,-89.9999999999865));
#38437=CARTESIAN_POINT('',(-92.4,-1.44337567297854,-89.9999999999864));
#38438=CARTESIAN_POINT('',(-92.6,-1.44337567297854,-89.9999999999864));
#38439=CARTESIAN_POINT('',(-92.4,1.44337567302146,-89.9999999999867));
#38440=CARTESIAN_POINT('',(-92.6,1.44337567302146,-89.9999999999867));
#38441=CARTESIAN_POINT('',(-92.4,2.14708893025995E-11,-89.9999999999866));
#38442=CARTESIAN_POINT('Origin',(-92.6,2.16506350947161,-88.7499999999868));
#38443=CARTESIAN_POINT('',(-92.4,2.88675134592174,-87.4999999999869));
#38444=CARTESIAN_POINT('',(-92.6,2.88675134592174,-87.4999999999869));
#38445=CARTESIAN_POINT('',(-92.4,1.44337567302146,-89.9999999999867));
#38446=CARTESIAN_POINT('Origin',(-92.6,2.16506350947189,-86.2499999999868));
#38447=CARTESIAN_POINT('',(-92.4,1.44337567302204,-84.9999999999868));
#38448=CARTESIAN_POINT('',(-92.6,1.44337567302204,-84.9999999999868));
#38449=CARTESIAN_POINT('',(-92.4,2.88675134592174,-87.4999999999869));
#38450=CARTESIAN_POINT('Origin',(-92.6,2.2026000814912E-11,-84.9999999999866));
#38451=CARTESIAN_POINT('',(-92.4,-1.44337567297796,-84.9999999999864));
#38452=CARTESIAN_POINT('',(-92.6,-1.44337567297796,-84.9999999999864));
#38453=CARTESIAN_POINT('',(-92.4,2.2026000814912E-11,-84.9999999999866));
#38454=CARTESIAN_POINT('Origin',(-92.6,-2.16506350942812,-86.2499999999863));
#38455=CARTESIAN_POINT('',(-92.4,-2.88675134587825,-87.4999999999863));
#38456=CARTESIAN_POINT('',(-92.6,-2.88675134587825,-87.4999999999863));
#38457=CARTESIAN_POINT('',(-92.4,-1.44337567297796,-84.9999999999864));
#38458=CARTESIAN_POINT('Origin',(-92.6,-2.16506350942839,-88.7499999999863));
#38459=CARTESIAN_POINT('',(-92.4,-2.88675134587825,-87.4999999999863));
#38460=CARTESIAN_POINT('Origin',(-59.000000000006,70.5000000000192,-137.259999999995));
#38461=CARTESIAN_POINT('',(-59.0000000000057,66.50000000002,-131.259999999994));
#38462=CARTESIAN_POINT('',(-59.0000000000061,70.50000000002,-131.259999999995));
#38463=CARTESIAN_POINT('',(-59.0000000000061,70.5000000000199,-131.259999999995));
#38464=CARTESIAN_POINT('',(-59.0000000000057,66.5000000000193,-136.916854249486));
#38465=CARTESIAN_POINT('Origin',(-59.0000000000055,64.5000000000199,-131.259999999994));
#38466=CARTESIAN_POINT('',(-59.0000000000057,66.5000000000199,-131.259999999994));
#38467=CARTESIAN_POINT('Origin',(-69.000000000006,70.5000000000191,-131.259999999995));
#38468=CARTESIAN_POINT('',(-69.000000000006,70.5000000000203,-121.259999999995));
#38469=CARTESIAN_POINT('',(-69.0000000000057,66.5000000000203,-121.259999999994));
#38470=CARTESIAN_POINT('',(-69.000000000006,70.5000000000202,-121.259999999995));
#38471=CARTESIAN_POINT('Origin',(-69.000000000006,70.5000000000191,-131.259999999995));
#38472=CARTESIAN_POINT('Origin',(-69.0000000000057,66.5000000000191,-131.259999999994));
#38473=CARTESIAN_POINT('Origin',(-69.000000000006,70.5000000000202,-121.259999999995));
#38474=CARTESIAN_POINT('',(-77.0000000000057,66.5000000000195,-121.259999999994));
#38475=CARTESIAN_POINT('',(-69.0000000000057,66.5000000000202,-121.259999999994));
#38476=CARTESIAN_POINT('',(-77.0000000000058,68.0000000000195,-121.259999999994));
#38477=CARTESIAN_POINT('',(-77.000000000006,70.5000000000195,-121.259999999995));
#38478=CARTESIAN_POINT('',(-74.500000000006,70.5000000000197,-121.259999999995));
#38479=CARTESIAN_POINT('Origin',(-74.5000000000058,68.0000000000197,-121.259999999994));
#38480=CARTESIAN_POINT('',(74.499999999994,70.5000000000327,-121.259999999995));
#38481=CARTESIAN_POINT('Origin',(-74.7735026919036,85.7752523165379,-131.259999999996));
#38482=CARTESIAN_POINT('',(-74.7735026919019,66.5000000000185,-131.259999999994));
#38483=CARTESIAN_POINT('',(-74.7735026919037,85.775252316538,-131.259999999996));
#38484=CARTESIAN_POINT('',(-71.8867513459538,66.5000000000193,-126.259999999994));
#38485=CARTESIAN_POINT('',(-74.7735026919019,66.5000000000185,-131.259999999994));
#38486=CARTESIAN_POINT('',(-71.8867513459555,85.7752523165388,-126.259999999996));
#38487=CARTESIAN_POINT('Origin',(-71.8867513459555,85.7752523165388,-126.259999999996));
#38488=CARTESIAN_POINT('',(-66.1132486540576,66.5000000000198,-126.259999999994));
#38489=CARTESIAN_POINT('',(-69.0000000000057,66.5000000000197,-126.259999999994));
#38490=CARTESIAN_POINT('',(-66.1132486540593,85.7752523165393,-126.259999999996));
#38491=CARTESIAN_POINT('Origin',(-66.1132486540593,85.7752523165393,-126.259999999996));
#38492=CARTESIAN_POINT('',(-63.2264973081095,66.5000000000196,-131.259999999994));
#38493=CARTESIAN_POINT('',(-66.1132486540576,66.5000000000199,-126.259999999994));
#38494=CARTESIAN_POINT('',(-63.2264973081112,85.775252316539,-131.259999999996));
#38495=CARTESIAN_POINT('Origin',(-63.2264973081112,85.775252316539,-131.259999999996));
#38496=CARTESIAN_POINT('',(-66.1132486540576,66.5000000000187,-136.259999999994));
#38497=CARTESIAN_POINT('',(-63.2264973081095,66.5000000000196,-131.259999999994));
#38498=CARTESIAN_POINT('',(-66.1132486540593,85.7752523165382,-136.259999999996));
#38499=CARTESIAN_POINT('Origin',(-66.1132486540593,85.7752523165382,-136.259999999996));
#38500=CARTESIAN_POINT('',(-71.8867513459539,66.5000000000182,-136.259999999994));
#38501=CARTESIAN_POINT('',(-69.0000000000057,66.5000000000185,-136.259999999994));
#38502=CARTESIAN_POINT('',(-71.8867513459556,85.7752523165377,-136.259999999996));
#38503=CARTESIAN_POINT('Origin',(-71.8867513459556,85.7752523165377,-136.259999999996));
#38504=CARTESIAN_POINT('',(-71.8867513459539,66.5000000000182,-136.259999999994));
#38505=CARTESIAN_POINT('Origin',(-69.000000000006,70.5000000000279,-53.2599999999947));
#38506=CARTESIAN_POINT('',(-59.0000000000061,70.5000000000287,-53.2599999999947));
#38507=CARTESIAN_POINT('',(-59.0000000000057,66.5000000000286,-53.2599999999943));
#38508=CARTESIAN_POINT('',(-59.0000000000061,70.5000000000286,-53.2599999999947));
#38509=CARTESIAN_POINT('',(-69.000000000006,70.5000000000268,-63.2599999999947));
#38510=CARTESIAN_POINT('Origin',(-69.000000000006,70.5000000000278,-53.2599999999947));
#38511=CARTESIAN_POINT('',(-69.0000000000057,66.5000000000267,-63.2599999999943));
#38512=CARTESIAN_POINT('',(-69.000000000006,70.5000000000267,-63.2599999999947));
#38513=CARTESIAN_POINT('Origin',(-69.0000000000057,66.5000000000278,-53.2599999999943));
#38514=CARTESIAN_POINT('Origin',(-69.000000000006,70.5000000000267,-63.2599999999947));
#38515=CARTESIAN_POINT('',(-74.500000000006,70.5000000000262,-63.2599999999947));
#38516=CARTESIAN_POINT('',(74.499999999994,70.5000000000394,-63.2599999999947));
#38517=CARTESIAN_POINT('',(-77.0000000000058,68.000000000026,-63.2599999999944));
#38518=CARTESIAN_POINT('Origin',(-74.5000000000058,68.000000000026,-63.2599999999944));
#38519=CARTESIAN_POINT('',(-77.0000000000057,66.5000000000259,-63.2599999999942));
#38520=CARTESIAN_POINT('',(-77.000000000006,70.500000000026,-63.2599999999947));
#38521=CARTESIAN_POINT('',(-69.0000000000057,66.5000000000267,-63.2599999999942));
#38522=CARTESIAN_POINT('Origin',(-74.7735026919036,85.7752523165467,-53.2599999999964));
#38523=CARTESIAN_POINT('',(-74.7735026919019,66.5000000000272,-53.2599999999943));
#38524=CARTESIAN_POINT('',(-74.7735026919035,85.7752523165467,-53.2599999999965));
#38525=CARTESIAN_POINT('',(-71.8867513459538,66.5000000000281,-48.2599999999942));
#38526=CARTESIAN_POINT('',(-71.8867513459538,66.5000000000281,-48.2599999999943));
#38527=CARTESIAN_POINT('',(-71.8867513459555,85.7752523165475,-48.2599999999964));
#38528=CARTESIAN_POINT('Origin',(-71.8867513459555,85.7752523165464,-58.2599999999964));
#38529=CARTESIAN_POINT('',(-71.8867513459538,66.5000000000269,-58.2599999999942));
#38530=CARTESIAN_POINT('',(-71.8867513459555,85.7752523165464,-58.2599999999964));
#38531=CARTESIAN_POINT('',(-74.7735026919019,66.5000000000272,-53.2599999999943));
#38532=CARTESIAN_POINT('Origin',(-66.1132486540593,85.7752523165469,-58.2599999999964));
#38533=CARTESIAN_POINT('',(-66.1132486540576,66.5000000000274,-58.2599999999942));
#38534=CARTESIAN_POINT('',(-66.1132486540593,85.7752523165469,-58.2599999999964));
#38535=CARTESIAN_POINT('',(-69.0000000000057,66.5000000000272,-58.2599999999943));
#38536=CARTESIAN_POINT('Origin',(-63.2264973081112,85.7752523165478,-53.2599999999964));
#38537=CARTESIAN_POINT('',(-63.2264973081095,66.5000000000283,-53.2599999999942));
#38538=CARTESIAN_POINT('',(-63.2264973081111,85.7752523165477,-53.2599999999965));
#38539=CARTESIAN_POINT('',(-66.1132486540576,66.5000000000274,-58.2599999999943));
#38540=CARTESIAN_POINT('Origin',(-66.1132486540593,85.775252316548,-48.2599999999964));
#38541=CARTESIAN_POINT('',(-66.1132486540576,66.5000000000286,-48.2599999999942));
#38542=CARTESIAN_POINT('',(-66.1132486540593,85.775252316548,-48.2599999999964));
#38543=CARTESIAN_POINT('',(-63.2264973081095,66.5000000000283,-53.2599999999943));
#38544=CARTESIAN_POINT('Origin',(-71.8867513459555,85.7752523165475,-48.2599999999964));
#38545=CARTESIAN_POINT('',(-69.0000000000057,66.5000000000283,-48.2599999999943));
#38546=CARTESIAN_POINT('Origin',(53.999999999995,58.5000000000291,-137.259999999993));
#38547=CARTESIAN_POINT('',(53.999999999994,70.5000000000387,-53.2599999999947));
#38548=CARTESIAN_POINT('',(53.999999999994,70.5000000000298,-131.259999999995));
#38549=CARTESIAN_POINT('',(53.999999999994,70.5000000000291,-137.259999999995));
#38550=CARTESIAN_POINT('Ctrl Pts',(49.4999999999941,69.6242977306726,-134.381149270331));
#38551=CARTESIAN_POINT('Ctrl Pts',(49.8539422620161,69.7674744252977,-134.146082008947));
#38552=CARTESIAN_POINT('Ctrl Pts',(50.2140176820507,69.8933981532635,-133.902800848474));
#38553=CARTESIAN_POINT('Ctrl Pts',(51.7309088331643,70.3448922127441,-132.865641552744));
#38554=CARTESIAN_POINT('Ctrl Pts',(52.913589003477,70.5000000000296,-132.028208582787));
#38555=CARTESIAN_POINT('Ctrl Pts',(53.999999999994,70.5000000000298,-131.259999999995));
#38556=CARTESIAN_POINT('Ctrl Pts',(53.999999999994,70.5000000000385,-53.2599999999947));
#38557=CARTESIAN_POINT('Ctrl Pts',(52.913589003477,70.5000000000385,-52.4917914172019));
#38558=CARTESIAN_POINT('Ctrl Pts',(51.7309088331643,70.3448922127531,-51.6543584472452));
#38559=CARTESIAN_POINT('Ctrl Pts',(50.2140176820507,69.8933981532728,-50.617199151515));
#38560=CARTESIAN_POINT('Ctrl Pts',(49.8539422620161,69.7674744253071,-50.373917991042));
#38561=CARTESIAN_POINT('Ctrl Pts',(49.4999999999941,69.624297730682,-50.1388507296581));
#38562=CARTESIAN_POINT('Origin',(35.999999999995,58.5000000000275,-137.259999999993));
#38563=CARTESIAN_POINT('',(35.999999999994,70.5000000000369,-53.2599999999947));
#38564=CARTESIAN_POINT('Ctrl Pts',(35.999999999994,70.500000000037,-53.2599999999947));
#38565=CARTESIAN_POINT('Ctrl Pts',(34.913589003477,70.5000000000369,-52.4917914172019));
#38566=CARTESIAN_POINT('Ctrl Pts',(33.7309088331644,70.3448922127515,-51.6543584472451));
#38567=CARTESIAN_POINT('Ctrl Pts',(32.2140176820507,69.8933981532712,-50.6171991515149));
#38568=CARTESIAN_POINT('Ctrl Pts',(31.8539422620161,69.7674744253055,-50.3739179910419));
#38569=CARTESIAN_POINT('Ctrl Pts',(31.4999999999941,69.6242977306804,-50.138850729658));
#38570=CARTESIAN_POINT('Ctrl Pts',(40.499999999994,69.6242977306811,-50.138850729658));
#38571=CARTESIAN_POINT('Ctrl Pts',(40.146057737972,69.7674744253062,-50.3739179910419));
#38572=CARTESIAN_POINT('Ctrl Pts',(39.7859823179373,69.8933981532718,-50.6171991515149));
#38573=CARTESIAN_POINT('Ctrl Pts',(38.2690911668236,70.3448922127519,-51.6543584472451));
#38574=CARTESIAN_POINT('Ctrl Pts',(37.0864109965109,70.5000000000371,-52.4917914172019));
#38575=CARTESIAN_POINT('Ctrl Pts',(35.999999999994,70.500000000037,-53.2599999999947));
#38576=CARTESIAN_POINT('',(35.999999999994,70.5000000000282,-131.259999999995));
#38577=CARTESIAN_POINT('Ctrl Pts',(35.999999999994,70.5000000000283,-131.259999999995));
#38578=CARTESIAN_POINT('Ctrl Pts',(37.0864109965109,70.5000000000283,-132.028208582787));
#38579=CARTESIAN_POINT('Ctrl Pts',(38.2690911668235,70.3448922127429,-132.865641552744));
#38580=CARTESIAN_POINT('Ctrl Pts',(39.7859823179373,69.8933981532626,-133.902800848474));
#38581=CARTESIAN_POINT('Ctrl Pts',(40.1460577379719,69.7674744252968,-134.146082008947));
#38582=CARTESIAN_POINT('Ctrl Pts',(40.4999999999939,69.6242977306718,-134.381149270331));
#38583=CARTESIAN_POINT('Ctrl Pts',(31.4999999999942,69.624297730671,-134.381149270331));
#38584=CARTESIAN_POINT('Ctrl Pts',(31.8539422620161,69.7674744252961,-134.146082008947));
#38585=CARTESIAN_POINT('Ctrl Pts',(32.2140176820507,69.8933981532619,-133.902800848474));
#38586=CARTESIAN_POINT('Ctrl Pts',(33.7309088331644,70.3448922127425,-132.865641552744));
#38587=CARTESIAN_POINT('Ctrl Pts',(34.913589003477,70.5000000000281,-132.028208582787));
#38588=CARTESIAN_POINT('Ctrl Pts',(35.999999999994,70.5000000000283,-131.259999999995));
#38589=CARTESIAN_POINT('Origin',(17.999999999995,58.5000000000259,-137.259999999993));
#38590=CARTESIAN_POINT('',(17.9999999999939,70.5000000000266,-131.259999999995));
#38591=CARTESIAN_POINT('Ctrl Pts',(17.999999999994,70.5000000000267,-131.259999999995));
#38592=CARTESIAN_POINT('Ctrl Pts',(19.0864109965109,70.5000000000267,-132.028208582787));
#38593=CARTESIAN_POINT('Ctrl Pts',(20.2690911668235,70.3448922127413,-132.865641552744));
#38594=CARTESIAN_POINT('Ctrl Pts',(21.7859823179372,69.893398153261,-133.902800848474));
#38595=CARTESIAN_POINT('Ctrl Pts',(22.1460577379719,69.7674744252952,-134.146082008947));
#38596=CARTESIAN_POINT('Ctrl Pts',(22.4999999999939,69.6242977306702,-134.381149270331));
#38597=CARTESIAN_POINT('Ctrl Pts',(14.829569219826,70.0736065540853,-133.481465727965));
#38598=CARTESIAN_POINT('Ctrl Pts',(15.9026718230638,70.3675682943341,-132.743922464767));
#38599=CARTESIAN_POINT('Ctrl Pts',(16.9928110658882,70.5000000000265,-131.972190125237));
#38600=CARTESIAN_POINT('Ctrl Pts',(17.999999999994,70.5000000000267,-131.259999999995));
#38601=CARTESIAN_POINT('',(14.8295692198259,70.0736065540945,-51.038534272024));
#38602=CARTESIAN_POINT('Origin',(17.9999999898631,58.5000000290889,-45.547187096471));
#38603=CARTESIAN_POINT('',(17.9999999999939,70.5000000000353,-53.2599999999947));
#38604=CARTESIAN_POINT('Ctrl Pts',(17.999999999994,70.5000000000354,-53.2599999999947));
#38605=CARTESIAN_POINT('Ctrl Pts',(16.9928110658882,70.5000000000354,-52.5478098747524));
#38606=CARTESIAN_POINT('Ctrl Pts',(15.9026718230638,70.3675682943431,-51.7760775352227));
#38607=CARTESIAN_POINT('Ctrl Pts',(14.829569219826,70.0736065540945,-51.0385342720238));
#38608=CARTESIAN_POINT('Ctrl Pts',(22.499999999994,69.6242977306796,-50.138850729658));
#38609=CARTESIAN_POINT('Ctrl Pts',(22.146057737972,69.7674744253046,-50.3739179910419));
#38610=CARTESIAN_POINT('Ctrl Pts',(21.7859823179373,69.8933981532703,-50.6171991515149));
#38611=CARTESIAN_POINT('Ctrl Pts',(20.2690911668235,70.3448922127504,-51.654358447245));
#38612=CARTESIAN_POINT('Ctrl Pts',(19.0864109965109,70.5000000000356,-52.4917914172019));
#38613=CARTESIAN_POINT('Ctrl Pts',(17.999999999994,70.5000000000354,-53.2599999999947));
#38614=CARTESIAN_POINT('Origin',(16.4337567297346,70.5000000000358,-48.2599999999947));
#38615=CARTESIAN_POINT('',(16.4337567297348,67.8166247903912,-48.2599999999944));
#38616=CARTESIAN_POINT('',(16.4337567297349,66.5000000000358,-48.2599999999943));
#38617=CARTESIAN_POINT('',(16.4337567297346,70.5000000000358,-48.2599999999947));
#38618=CARTESIAN_POINT('Origin',(13.5470053837932,64.5000000000491,-53.2599999999832));
#38619=CARTESIAN_POINT('',(16.4337567297349,66.5000000000358,-48.2599999999943));
#38620=CARTESIAN_POINT('Origin',(18.1658075373035,70.5000000000358,-49.2599999999947));
#38621=CARTESIAN_POINT('',(17.0456138058721,66.5000000000359,-47.6031457505019));
#38622=CARTESIAN_POINT('Origin',(18.1658075373038,66.5000000000358,-49.2599999999943));
#38623=CARTESIAN_POINT('Ctrl Pts',(16.4337567297349,67.8166247903912,-48.2599999999944));
#38624=CARTESIAN_POINT('Ctrl Pts',(16.5274124833924,67.5720741794393,-48.0977834762383));
#38625=CARTESIAN_POINT('Ctrl Pts',(16.6384034067921,67.3227889604663,-47.9589770057598));
#38626=CARTESIAN_POINT('Ctrl Pts',(16.8407204020279,66.8991702874141,-47.756660010524));
#38627=CARTESIAN_POINT('Ctrl Pts',(16.9396941465962,66.7025491386553,-47.6747576852225));
#38628=CARTESIAN_POINT('Ctrl Pts',(17.0456138058721,66.500000000036,-47.6031457505018));
#38629=CARTESIAN_POINT('Origin',(1.99999999999431,66.5000000000339,-53.2599999999943));
#38630=CARTESIAN_POINT('',(-13.0456138058834,66.5000000000333,-47.6031457505019));
#38631=CARTESIAN_POINT('',(-12.4337567297463,66.5000000000332,-48.2599999999943));
#38632=CARTESIAN_POINT('Origin',(-14.1658075373152,66.500000000033,-49.2599999999943));
#38633=CARTESIAN_POINT('',(74.4999999999943,66.5000000000409,-47.6031457505019));
#38634=CARTESIAN_POINT('',(-6.66025403785006,66.5000000000326,-58.2599999999943));
#38635=CARTESIAN_POINT('Origin',(-14.1658075373155,70.500000000033,-49.2599999999947));
#38636=CARTESIAN_POINT('',(-12.4337567297464,67.8166247903887,-48.2599999999944));
#38637=CARTESIAN_POINT('',(-12.4337567297466,70.5000000000333,-48.2599999999947));
#38638=CARTESIAN_POINT('Ctrl Pts',(-13.0456138058834,66.5000000000333,-47.6031457505018));
#38639=CARTESIAN_POINT('Ctrl Pts',(-12.9396941466076,66.7025491386527,-47.6747576852225));
#38640=CARTESIAN_POINT('Ctrl Pts',(-12.8407204020393,66.8991702874115,-47.756660010524));
#38641=CARTESIAN_POINT('Ctrl Pts',(-12.6384034068036,67.3227889604638,-47.9589770057598));
#38642=CARTESIAN_POINT('Ctrl Pts',(-12.5274124834039,67.5720741794367,-48.0977834762384));
#38643=CARTESIAN_POINT('Ctrl Pts',(-12.4337567297464,67.8166247903887,-48.2599999999944));
#38644=CARTESIAN_POINT('Origin',(-6.66025403785042,70.5000000000327,-58.2599999999947));
#38645=CARTESIAN_POINT('Origin',(-9.54700538384715,64.4999999999613,-53.2599999999105));
#38646=CARTESIAN_POINT('Origin',(-18.000000000005,58.5000000000228,-137.259999999993));
#38647=CARTESIAN_POINT('',(-18.0000000000061,70.5000000000322,-53.2599999999947));
#38648=CARTESIAN_POINT('Ctrl Pts',(-18.000000000006,70.5000000000323,-53.2599999999947));
#38649=CARTESIAN_POINT('Ctrl Pts',(-19.086410996523,70.5000000000323,-52.4917914172019));
#38650=CARTESIAN_POINT('Ctrl Pts',(-20.2690911668356,70.3448922127468,-51.6543584472451));
#38651=CARTESIAN_POINT('Ctrl Pts',(-21.7859823179493,69.8933981532665,-50.6171991515149));
#38652=CARTESIAN_POINT('Ctrl Pts',(-22.1460577379839,69.7674744253008,-50.3739179910419));
#38653=CARTESIAN_POINT('Ctrl Pts',(-22.5000000000059,69.6242977306757,-50.138850729658));
#38654=CARTESIAN_POINT('Ctrl Pts',(-13.500000000006,69.6242977306764,-50.138850729658));
#38655=CARTESIAN_POINT('Ctrl Pts',(-13.853942262028,69.7674744253015,-50.3739179910419));
#38656=CARTESIAN_POINT('Ctrl Pts',(-14.2140176820627,69.8933981532672,-50.6171991515149));
#38657=CARTESIAN_POINT('Ctrl Pts',(-15.7309088331764,70.3448922127472,-51.6543584472451));
#38658=CARTESIAN_POINT('Ctrl Pts',(-16.9135890034891,70.5000000000324,-52.4917914172019));
#38659=CARTESIAN_POINT('Ctrl Pts',(-18.000000000006,70.5000000000323,-53.2599999999947));
#38660=CARTESIAN_POINT('',(-18.0000000000061,70.5000000000236,-131.259999999995));
#38661=CARTESIAN_POINT('Ctrl Pts',(-18.000000000006,70.5000000000236,-131.259999999995));
#38662=CARTESIAN_POINT('Ctrl Pts',(-16.9135890034891,70.5000000000236,-132.028208582787));
#38663=CARTESIAN_POINT('Ctrl Pts',(-15.7309088331765,70.3448922127382,-132.865641552744));
#38664=CARTESIAN_POINT('Ctrl Pts',(-14.2140176820627,69.8933981532579,-133.902800848474));
#38665=CARTESIAN_POINT('Ctrl Pts',(-13.8539422620281,69.7674744252922,-134.146082008947));
#38666=CARTESIAN_POINT('Ctrl Pts',(-13.5000000000062,69.6242977306671,-134.381149270331));
#38667=CARTESIAN_POINT('Ctrl Pts',(-22.5000000000058,69.6242977306663,-134.381149270331));
#38668=CARTESIAN_POINT('Ctrl Pts',(-22.1460577379839,69.7674744252914,-134.146082008947));
#38669=CARTESIAN_POINT('Ctrl Pts',(-21.7859823179493,69.8933981532572,-133.902800848474));
#38670=CARTESIAN_POINT('Ctrl Pts',(-20.2690911668356,70.3448922127378,-132.865641552744));
#38671=CARTESIAN_POINT('Ctrl Pts',(-19.086410996523,70.5000000000234,-132.028208582787));
#38672=CARTESIAN_POINT('Ctrl Pts',(-18.000000000006,70.5000000000236,-131.259999999995));
#38673=CARTESIAN_POINT('Origin',(-36.000000000005,58.5000000000212,-137.259999999993));
#38674=CARTESIAN_POINT('',(-36.000000000006,70.5000000000306,-53.2599999999948));
#38675=CARTESIAN_POINT('Ctrl Pts',(-36.000000000006,70.5000000000307,-53.2599999999947));
#38676=CARTESIAN_POINT('Ctrl Pts',(-37.086410996523,70.5000000000307,-52.4917914172019));
#38677=CARTESIAN_POINT('Ctrl Pts',(-38.2690911668355,70.3448922127453,-51.654358447245));
#38678=CARTESIAN_POINT('Ctrl Pts',(-39.7859823179492,69.8933981532649,-50.6171991515149));
#38679=CARTESIAN_POINT('Ctrl Pts',(-40.1460577379839,69.7674744252992,-50.3739179910419));
#38680=CARTESIAN_POINT('Ctrl Pts',(-40.5000000000059,69.6242977306741,-50.138850729658));
#38681=CARTESIAN_POINT('Ctrl Pts',(-31.5000000000061,69.6242977306749,-50.138850729658));
#38682=CARTESIAN_POINT('Ctrl Pts',(-31.8539422620281,69.7674744252999,-50.3739179910419));
#38683=CARTESIAN_POINT('Ctrl Pts',(-32.2140176820627,69.8933981532656,-50.6171991515149));
#38684=CARTESIAN_POINT('Ctrl Pts',(-33.7309088331765,70.3448922127456,-51.654358447245));
#38685=CARTESIAN_POINT('Ctrl Pts',(-34.9135890034891,70.5000000000309,-52.4917914172019));
#38686=CARTESIAN_POINT('Ctrl Pts',(-36.000000000006,70.5000000000307,-53.2599999999947));
#38687=CARTESIAN_POINT('',(-36.000000000006,70.500000000022,-131.259999999995));
#38688=CARTESIAN_POINT('Ctrl Pts',(-36.000000000006,70.500000000022,-131.259999999995));
#38689=CARTESIAN_POINT('Ctrl Pts',(-34.9135890034891,70.500000000022,-132.028208582787));
#38690=CARTESIAN_POINT('Ctrl Pts',(-33.7309088331766,70.3448922127366,-132.865641552744));
#38691=CARTESIAN_POINT('Ctrl Pts',(-32.2140176820628,69.8933981532563,-133.902800848474));
#38692=CARTESIAN_POINT('Ctrl Pts',(-31.8539422620281,69.7674744252905,-134.146082008947));
#38693=CARTESIAN_POINT('Ctrl Pts',(-31.5000000000061,69.6242977306655,-134.381149270331));
#38694=CARTESIAN_POINT('Ctrl Pts',(-40.5000000000058,69.6242977306647,-134.381149270331));
#38695=CARTESIAN_POINT('Ctrl Pts',(-40.1460577379838,69.7674744252898,-134.146082008947));
#38696=CARTESIAN_POINT('Ctrl Pts',(-39.7859823179492,69.8933981532556,-133.902800848474));
#38697=CARTESIAN_POINT('Ctrl Pts',(-38.2690911668355,70.3448922127362,-132.865641552744));
#38698=CARTESIAN_POINT('Ctrl Pts',(-37.086410996523,70.5000000000218,-132.028208582787));
#38699=CARTESIAN_POINT('Ctrl Pts',(-36.000000000006,70.500000000022,-131.259999999995));
#38700=CARTESIAN_POINT('Origin',(-54.000000000005,58.5000000000197,-137.259999999993));
#38701=CARTESIAN_POINT('',(-54.000000000006,70.5000000000204,-131.259999999995));
#38702=CARTESIAN_POINT('Ctrl Pts',(-54.0000000000061,70.5000000000204,-131.259999999995));
#38703=CARTESIAN_POINT('Ctrl Pts',(-52.9135890034891,70.5000000000204,-132.028208582787));
#38704=CARTESIAN_POINT('Ctrl Pts',(-51.7309088331764,70.344892212735,-132.865641552744));
#38705=CARTESIAN_POINT('Ctrl Pts',(-50.2140176820627,69.8933981532547,-133.902800848474));
#38706=CARTESIAN_POINT('Ctrl Pts',(-49.8539422620281,69.767474425289,-134.146082008947));
#38707=CARTESIAN_POINT('Ctrl Pts',(-49.5000000000061,69.624297730664,-134.381149270331));
#38708=CARTESIAN_POINT('',(-54.000000000006,70.5000000000292,-53.2599999999947));
#38709=CARTESIAN_POINT('',(-54.000000000006,70.5000000000197,-137.259999999995));
#38710=CARTESIAN_POINT('Ctrl Pts',(-49.500000000006,69.6242977306733,-50.1388507296581));
#38711=CARTESIAN_POINT('Ctrl Pts',(-49.853942262028,69.7674744252984,-50.373917991042));
#38712=CARTESIAN_POINT('Ctrl Pts',(-50.2140176820627,69.893398153264,-50.617199151515));
#38713=CARTESIAN_POINT('Ctrl Pts',(-51.7309088331764,70.3448922127441,-51.6543584472451));
#38714=CARTESIAN_POINT('Ctrl Pts',(-52.9135890034891,70.5000000000293,-52.4917914172019));
#38715=CARTESIAN_POINT('Ctrl Pts',(-54.0000000000061,70.5000000000291,-53.2599999999947));
#38716=CARTESIAN_POINT('Origin',(74.499999999994,70.5000000000309,-137.259999999995));
#38717=CARTESIAN_POINT('',(-74.500000000006,70.5000000000179,-137.259999999995));
#38718=CARTESIAN_POINT('',(74.499999999994,70.5000000000403,-53.2599999999947));
#38719=CARTESIAN_POINT('',(74.499999999994,70.5000000000316,-131.259999999995));
#38720=CARTESIAN_POINT('Origin',(-59.000000000006,70.5000000000293,-47.2599999999947));
#38721=CARTESIAN_POINT('',(-59.0000000000057,66.5000000000293,-47.6031457505019));
#38722=CARTESIAN_POINT('',(-59.0000000000057,66.5000000000286,-53.2599999999943));
#38723=CARTESIAN_POINT('Origin',(-59.0000000000055,64.5000000000287,-53.259999999994));
#38724=CARTESIAN_POINT('Ctrl Pts',(-73.0104689725931,67.9465182387393,-136.171365597276));
#38725=CARTESIAN_POINT('Ctrl Pts',(-73.8703570864329,67.3703570864452,-136.57568286515));
#38726=CARTESIAN_POINT('Ctrl Pts',(-74.4465182387269,66.5104689726054,-136.171365597276));
#38727=CARTESIAN_POINT('Ctrl Pts',(-72.7182901970741,67.4456403378437,-136.522853342713));
#38728=CARTESIAN_POINT('Ctrl Pts',(-73.4169322419492,66.9169322419576,-136.80863897917));
#38729=CARTESIAN_POINT('Ctrl Pts',(-73.9456403378363,66.2182901970746,-136.52285334271));
#38730=CARTESIAN_POINT('Ctrl Pts',(-72.3945521743876,66.8906608703868,-136.79707108069));
#38731=CARTESIAN_POINT('Ctrl Pts',(-72.9358474574371,66.4358474574396,-136.981577743066));
#38732=CARTESIAN_POINT('Ctrl Pts',(-73.3906608703737,65.8945521743998,-136.797071080691));
#38733=CARTESIAN_POINT('Ctrl Pts',(-71.7138256723184,65.7237011525547,-137.16567278462));
#38734=CARTESIAN_POINT('Ctrl Pts',(-71.9760256068087,65.476025606831,-137.204292118055));
#38735=CARTESIAN_POINT('Ctrl Pts',(-72.2237011525427,65.2138256723311,-137.16567278462));
#38736=CARTESIAN_POINT('Ctrl Pts',(-71.3569625715572,65.1119358369451,-137.259999999994));
#38737=CARTESIAN_POINT('Ctrl Pts',(-71.4844140292029,64.9844140291876,-137.259999999994));
#38738=CARTESIAN_POINT('Ctrl Pts',(-71.6119358369396,64.8569625715567,-137.259999999994));
#38739=CARTESIAN_POINT('Ctrl Pts',(-71.0000000000055,64.5000000000182,-137.259999999994));
#38740=CARTESIAN_POINT('Ctrl Pts',(-71.0000000000055,64.5000000000182,-137.259999999994));
#38741=CARTESIAN_POINT('Ctrl Pts',(-71.0000000000055,64.5000000000182,-137.259999999994));
#38742=CARTESIAN_POINT('',(-71.0000000000055,64.5000000000182,-137.259999999994));
#38743=CARTESIAN_POINT('',(-72.1666666648479,66.4999929738548,-136.916834384971));
#38744=CARTESIAN_POINT('Ctrl Pts',(-71.0000000000055,64.5000000000182,-137.259999999994));
#38745=CARTESIAN_POINT('Ctrl Pts',(-71.0461016235444,64.579031354654,-137.259999999994));
#38746=CARTESIAN_POINT('Ctrl Pts',(-71.0901862514509,64.6546050024919,-137.258430124937));
#38747=CARTESIAN_POINT('Ctrl Pts',(-71.1322321415784,64.7266836712807,-137.255691250101));
#38748=CARTESIAN_POINT('Ctrl Pts',(-71.1769086032859,64.8032718913493,-137.252781019485));
#38749=CARTESIAN_POINT('Ctrl Pts',(-71.2192833734128,64.8759143544232,-137.248551330288));
#38750=CARTESIAN_POINT('Ctrl Pts',(-71.2593483300541,64.9445971372364,-137.243432561143));
#38751=CARTESIAN_POINT('Ctrl Pts',(-71.3005720467883,65.0152663659233,-137.238165746776));
#38752=CARTESIAN_POINT('Ctrl Pts',(-71.3393520927811,65.0817464447679,-137.231957549005));
#38753=CARTESIAN_POINT('Ctrl Pts',(-71.3756897878606,65.1440396363329,-137.22522199684));
#38754=CARTESIAN_POINT('Ctrl Pts',(-71.4119624699439,65.2062213770471,-137.218498495478));
#38755=CARTESIAN_POINT('Ctrl Pts',(-71.4458000279303,65.2642286193098,-137.211249696265));
#38756=CARTESIAN_POINT('Ctrl Pts',(-71.4772099370766,65.3180741778466,-137.203835335352));
#38757=CARTESIAN_POINT('Ctrl Pts',(-71.4992812448217,65.35591070541,-137.198625366718));
#38758=CARTESIAN_POINT('Ctrl Pts',(-71.5201539937003,65.3916925606305,-137.193332564077));
#38759=CARTESIAN_POINT('Ctrl Pts',(-71.5398318905126,65.4254260980235,-137.18806669589));
#38760=CARTESIAN_POINT('Ctrl Pts',(-71.5490219770469,65.4411805320823,-137.185607399311));
#38761=CARTESIAN_POINT('Ctrl Pts',(-71.5579523745364,65.4564872937506,-137.183153944699));
#38762=CARTESIAN_POINT('Ctrl Pts',(-71.5666244905579,65.4713462493087,-137.180716763366));
#38763=CARTESIAN_POINT('Ctrl Pts',(-71.5709605485687,65.4787757270877,-137.1794981727));
#38764=CARTESIAN_POINT('Ctrl Pts',(-71.5752312809214,65.4860939885622,-137.178283521247));
#38765=CARTESIAN_POINT('Ctrl Pts',(-71.5794366876175,65.4933011826271,-137.177074024157));
#38766=CARTESIAN_POINT('Ctrl Pts',(-71.5815393909655,65.4969047796595,-137.176469275612));
#38767=CARTESIAN_POINT('Ctrl Pts',(-71.5836257628995,65.5004806097435,-137.1758658151));
#38768=CARTESIAN_POINT('Ctrl Pts',(-71.5856958034194,65.504028691868,-137.175263791));
#38769=CARTESIAN_POINT('Ctrl Pts',(-71.5867308236794,65.5058027329303,-137.174962778951));
#38770=CARTESIAN_POINT('Ctrl Pts',(-71.5877617610859,65.5075698369966,-137.17466212597));
#38771=CARTESIAN_POINT('Ctrl Pts',(-71.5887886156389,65.5093300064616,-137.174361850386));
#38772=CARTESIAN_POINT('Ctrl Pts',(-71.5898154701919,65.5110901759266,-137.174061574802));
#38773=CARTESIAN_POINT('Ctrl Pts',(-71.5901645498526,65.5116885240887,-137.173959747421));
#38774=CARTESIAN_POINT('Ctrl Pts',(-71.5918569307377,65.5145897134391,-137.173462174011));
#38775=CARTESIAN_POINT('Ctrl Pts',(-71.6518002518728,65.6173484519944,-137.15583836189));
#38776=CARTESIAN_POINT('Ctrl Pts',(-71.7098470458656,65.7168576128275,-137.136026817555));
#38777=CARTESIAN_POINT('Ctrl Pts',(-71.7659715645342,65.8130727552615,-137.11446823468));
#38778=CARTESIAN_POINT('Ctrl Pts',(-71.8241491395591,65.9128074844008,-137.092121030599));
#38779=CARTESIAN_POINT('Ctrl Pts',(-71.8802613524022,66.0090029944704,-137.067896759689));
#38780=CARTESIAN_POINT('Ctrl Pts',(-71.9343032167983,66.1016493462721,-137.0422526908));
#38781=CARTESIAN_POINT('Ctrl Pts',(-71.9754646443761,66.1722141971086,-137.022720676201));
#38782=CARTESIAN_POINT('Ctrl Pts',(-72.0154255326638,66.2407209632734,-137.002364302726));
#38783=CARTESIAN_POINT('Ctrl Pts',(-72.0541916345281,66.3071785462513,-136.981372711329));
#38784=CARTESIAN_POINT('Ctrl Pts',(-72.0928696558172,66.3734851307576,-136.960428814989));
#38785=CARTESIAN_POINT('Ctrl Pts',(-72.1303568121008,66.4377492555433,-136.938853587582));
#38786=CARTESIAN_POINT('Ctrl Pts',(-72.1666666648479,66.4999929738547,-136.916834384971));
#38787=CARTESIAN_POINT('',(-74.4285713480856,66.4999999931934,-136.183910712889));
#38788=CARTESIAN_POINT('Ctrl Pts',(-74.4285712620137,66.4999999864247,-136.183910589276));
#38789=CARTESIAN_POINT('Ctrl Pts',(-74.3391637351035,66.447846586649,-136.246162395812));
#38790=CARTESIAN_POINT('Ctrl Pts',(-74.2459677079227,66.3934823597197,-136.307411277845));
#38791=CARTESIAN_POINT('Ctrl Pts',(-74.1489208833848,66.3368715577722,-136.367216310645));
#38792=CARTESIAN_POINT('Ctrl Pts',(-74.0544352094021,66.2817547643873,-136.425443036336));
#38793=CARTESIAN_POINT('Ctrl Pts',(-73.9562991774979,66.2245083351006,-136.482301080738));
#38794=CARTESIAN_POINT('Ctrl Pts',(-73.8544881487993,66.1651183162972,-136.53735222905));
#38795=CARTESIAN_POINT('Ctrl Pts',(-73.7991624013817,66.1328448266622,-136.567267906806));
#38796=CARTESIAN_POINT('Ctrl Pts',(-73.7427520100897,66.0999386725625,-136.596649461807));
#38797=CARTESIAN_POINT('Ctrl Pts',(-73.685257471521,66.0664001917311,-136.625422584916));
#38798=CARTESIAN_POINT('Ctrl Pts',(-73.5833222371684,66.0069379716926,-136.676436039762));
#38799=CARTESIAN_POINT('Ctrl Pts',(-73.4779732706246,65.9454844078761,-136.725541064569));
#38800=CARTESIAN_POINT('Ctrl Pts',(-73.3692181586471,65.88204392589,-136.772307970056));
#38801=CARTESIAN_POINT('Ctrl Pts',(-73.2532698589162,65.8144074177144,-136.822168092274));
#38802=CARTESIAN_POINT('Ctrl Pts',(-73.1334511973744,65.7445131984825,-136.869370640943));
#38803=CARTESIAN_POINT('Ctrl Pts',(-73.0098028938484,65.6723850214261,-136.913354442426));
#38804=CARTESIAN_POINT('Ctrl Pts',(-72.943363784672,65.6336288744067,-136.936987961896));
#38805=CARTESIAN_POINT('Ctrl Pts',(-72.8758195815183,65.5942280892339,-136.959691412332));
#38806=CARTESIAN_POINT('Ctrl Pts',(-72.8071810114582,65.5541889233654,-136.981371932656));
#38807=CARTESIAN_POINT('Ctrl Pts',(-72.8062002761416,65.5536168277641,-136.981681712593));
#38808=CARTESIAN_POINT('Ctrl Pts',(-72.8052193178398,65.553044602088,-136.981991283528));
#38809=CARTESIAN_POINT('Ctrl Pts',(-72.8042381365472,65.552472246334,-136.982300645237));
#38810=CARTESIAN_POINT('Ctrl Pts',(-72.8017395376995,65.5510147303395,-136.983088441353));
#38811=CARTESIAN_POINT('Ctrl Pts',(-72.7982538835131,65.548981439413,-136.984184208637));
#38812=CARTESIAN_POINT('Ctrl Pts',(-72.7967379885939,65.5480971731278,-136.984659963736));
#38813=CARTESIAN_POINT('Ctrl Pts',(-72.7414940646765,65.5158717604272,-137.001997958729));
#38814=CARTESIAN_POINT('Ctrl Pts',(-72.6820631103128,65.4812037746268,-137.019769083906));
#38815=CARTESIAN_POINT('Ctrl Pts',(-72.6183862784162,65.4440589628055,-137.037593809158));
#38816=CARTESIAN_POINT('Ctrl Pts',(-72.5555242070729,65.4073894278867,-137.055190462715));
#38817=CARTESIAN_POINT('Ctrl Pts',(-72.488523722678,65.3683057566253,-137.072839273218));
#38818=CARTESIAN_POINT('Ctrl Pts',(-72.4173412109389,65.32678256416,-137.09012722741));
#38819=CARTESIAN_POINT('Ctrl Pts',(-72.3480489944229,65.2863620455178,-137.106956089383));
#38820=CARTESIAN_POINT('Ctrl Pts',(-72.2747934881158,65.2436296031994,-137.123442835596));
#38821=CARTESIAN_POINT('Ctrl Pts',(-72.1975535325183,65.1985729267082,-137.139162840554));
#38822=CARTESIAN_POINT('Ctrl Pts',(-72.1522112972097,65.1721232684726,-137.148390968125));
#38823=CARTESIAN_POINT('Ctrl Pts',(-72.1054963903019,65.1448728943557,-137.157354060421));
#38824=CARTESIAN_POINT('Ctrl Pts',(-72.0574086363209,65.1168217045333,-137.165959242809));
#38825=CARTESIAN_POINT('Ctrl Pts',(-71.9810177539599,65.0722603564892,-137.179629198693));
#38826=CARTESIAN_POINT('Ctrl Pts',(-71.9011695232922,65.0256822219329,-137.192396570263));
#38827=CARTESIAN_POINT('Ctrl Pts',(-71.8178491645093,64.9770786793099,-137.203866314643));
#38828=CARTESIAN_POINT('Ctrl Pts',(-71.7364284600082,64.9295832683514,-137.21507455572));
#38829=CARTESIAN_POINT('Ctrl Pts',(-71.6516918329836,64.8801535692547,-137.225043624773));
#38830=CARTESIAN_POINT('Ctrl Pts',(-71.56365242532,64.8287972481189,-137.233368196345));
#38831=CARTESIAN_POINT('Ctrl Pts',(-71.476167290577,64.7777642528534,-137.241640358608));
#38832=CARTESIAN_POINT('Ctrl Pts',(-71.3854204310927,64.7248285848223,-137.24828872839));
#38833=CARTESIAN_POINT('Ctrl Pts',(-71.2914570392138,64.6700166062268,-137.252878611791));
#38834=CARTESIAN_POINT('Ctrl Pts',(-71.1974936473348,64.6152046276313,-137.257468495192));
#38835=CARTESIAN_POINT('Ctrl Pts',(-71.1003132543675,64.5585160650665,-137.259999999994));
#38836=CARTESIAN_POINT('Ctrl Pts',(-71.0000000000055,64.5000000000182,-137.259999999994));
#38837=CARTESIAN_POINT('Ctrl Pts',(-74.4285712620158,66.5000000000181,-136.183910589275));
#38838=CARTESIAN_POINT('Ctrl Pts',(-74.0993880304178,66.5000000000181,-136.413114927177));
#38839=CARTESIAN_POINT('Ctrl Pts',(-73.7389828108934,66.500000000018,-136.595513985264));
#38840=CARTESIAN_POINT('Ctrl Pts',(-72.9737426228516,66.5000000000181,-136.848440511399));
#38841=CARTESIAN_POINT('Ctrl Pts',(-72.570991520028,66.5000000000181,-136.916795227754));
#38842=CARTESIAN_POINT('Ctrl Pts',(-72.1666666658345,66.5000000000182,-136.91683189978));
#38843=CARTESIAN_POINT('Origin',(74.499999999994,70.5000000000309,-137.259999999995));
#38844=CARTESIAN_POINT('',(74.499999999994,70.5000000000391,-63.2599999999947));
#38845=CARTESIAN_POINT('',(68.999999999994,70.5000000000387,-63.2599999999947));
#38846=CARTESIAN_POINT('',(68.999999999994,70.5000000000387,-63.2599999999947));
#38847=CARTESIAN_POINT('',(74.499999999994,70.5000000000327,-121.259999999995));
#38848=CARTESIAN_POINT('',(74.499999999994,70.5000000000309,-137.259999999995));
#38849=CARTESIAN_POINT('',(68.999999999994,70.5000000000323,-121.259999999995));
#38850=CARTESIAN_POINT('',(68.999999999994,70.5000000000322,-121.259999999995));
#38851=CARTESIAN_POINT('',(58.999999999994,70.5000000000303,-131.259999999995));
#38852=CARTESIAN_POINT('Origin',(68.999999999994,70.5000000000311,-131.259999999995));
#38853=CARTESIAN_POINT('',(74.499999999994,70.5000000000316,-131.259999999995));
#38854=CARTESIAN_POINT('',(58.999999999994,70.500000000039,-53.2599999999947));
#38855=CARTESIAN_POINT('',(74.499999999994,70.5000000000403,-53.2599999999947));
#38856=CARTESIAN_POINT('Origin',(68.999999999994,70.5000000000399,-53.2599999999947));
#38857=CARTESIAN_POINT('Origin',(58.999999999994,70.5000000000296,-137.259999999995));
#38858=CARTESIAN_POINT('',(58.9999999999943,66.5000000000296,-136.916854249486));
#38859=CARTESIAN_POINT('',(58.9999999999943,66.5000000000302,-131.259999999994));
#38860=CARTESIAN_POINT('',(58.9999999999943,66.5000000000302,-131.259999999994));
#38861=CARTESIAN_POINT('Origin',(58.9999999999945,64.5000000000302,-131.259999999994));
#38862=CARTESIAN_POINT('',(58.999999999994,70.5000000000302,-131.259999999995));
#38863=CARTESIAN_POINT('Origin',(68.999999999994,70.5000000000311,-131.259999999995));
#38864=CARTESIAN_POINT('',(68.9999999999943,66.5000000000322,-121.259999999994));
#38865=CARTESIAN_POINT('',(68.999999999994,70.5000000000322,-121.259999999995));
#38866=CARTESIAN_POINT('Origin',(68.9999999999943,66.5000000000311,-131.259999999994));
#38867=CARTESIAN_POINT('Origin',(68.999999999994,70.5000000000322,-121.259999999995));
#38868=CARTESIAN_POINT('',(76.9999999999942,68.0000000000328,-121.259999999994));
#38869=CARTESIAN_POINT('Origin',(74.4999999999942,68.0000000000327,-121.259999999994));
#38870=CARTESIAN_POINT('',(76.9999999999943,66.5000000000329,-121.259999999994));
#38871=CARTESIAN_POINT('',(76.999999999994,70.5000000000329,-121.259999999995));
#38872=CARTESIAN_POINT('',(68.9999999999943,66.5000000000322,-121.259999999994));
#38873=CARTESIAN_POINT('Origin',(74.4999999999945,64.5000000000316,-131.259999999994));
#38874=CARTESIAN_POINT('',(72.1666658662162,66.4999968842164,-136.916844121822));
#38875=CARTESIAN_POINT('',(68.9999999999943,66.5000000000304,-136.916854249486));
#38876=CARTESIAN_POINT('',(70.9999999999945,64.5000000000306,-137.259999999994));
#38877=CARTESIAN_POINT('Origin',(71.1254265028578,64.7149703218329,-132.635568492653));
#38878=CARTESIAN_POINT('',(74.4999999999945,64.5000000000309,-137.259999999994));
#38879=CARTESIAN_POINT('',(-69.0000000000057,66.5000000000185,-136.916854249486));
#38880=CARTESIAN_POINT('Origin',(63.2264973080965,85.77525231655,-131.259999999996));
#38881=CARTESIAN_POINT('',(63.2264973080981,66.5000000000306,-131.259999999994));
#38882=CARTESIAN_POINT('',(63.2264973080965,85.7752523165501,-131.259999999996));
#38883=CARTESIAN_POINT('',(66.1132486540463,66.5000000000314,-126.259999999994));
#38884=CARTESIAN_POINT('',(66.1132486540463,66.5000000000314,-126.259999999994));
#38885=CARTESIAN_POINT('',(66.1132486540445,85.7752523165508,-126.259999999996));
#38886=CARTESIAN_POINT('Origin',(66.1132486540445,85.7752523165498,-136.259999999996));
#38887=CARTESIAN_POINT('',(66.1132486540462,66.5000000000303,-136.259999999994));
#38888=CARTESIAN_POINT('',(66.1132486540445,85.7752523165498,-136.259999999996));
#38889=CARTESIAN_POINT('',(63.2264973080981,66.5000000000306,-131.259999999994));
#38890=CARTESIAN_POINT('Origin',(71.8867513459408,85.7752523165503,-136.259999999996));
#38891=CARTESIAN_POINT('',(71.8867513459424,66.5000000000308,-136.259999999994));
#38892=CARTESIAN_POINT('',(71.8867513459408,85.7752523165502,-136.259999999996));
#38893=CARTESIAN_POINT('',(68.9999999999943,66.5000000000305,-136.259999999994));
#38894=CARTESIAN_POINT('Origin',(74.773502691889,85.7752523165511,-131.259999999996));
#38895=CARTESIAN_POINT('',(74.7735026918906,66.5000000000316,-131.259999999994));
#38896=CARTESIAN_POINT('',(74.7735026918889,85.7752523165511,-131.259999999996));
#38897=CARTESIAN_POINT('',(71.8867513459424,66.5000000000308,-136.259999999994));
#38898=CARTESIAN_POINT('Origin',(71.8867513459408,85.7752523165513,-126.259999999996));
#38899=CARTESIAN_POINT('',(71.8867513459424,66.5000000000319,-126.259999999994));
#38900=CARTESIAN_POINT('',(71.8867513459408,85.7752523165513,-126.259999999996));
#38901=CARTESIAN_POINT('',(74.7735026918906,66.5000000000316,-131.259999999994));
#38902=CARTESIAN_POINT('Origin',(66.1132486540445,85.7752523165508,-126.259999999996));
#38903=CARTESIAN_POINT('',(68.9999999999943,66.5000000000316,-126.259999999994));
#38904=CARTESIAN_POINT('Ctrl Pts',(74.4465182387155,66.5104689726184,-136.171365597276));
#38905=CARTESIAN_POINT('Ctrl Pts',(73.8703570864215,67.3703570864582,-136.57568286515));
#38906=CARTESIAN_POINT('Ctrl Pts',(73.0104689725816,67.9465182387521,-136.171365597276));
#38907=CARTESIAN_POINT('Ctrl Pts',(73.9456403378197,66.2182901970983,-136.522853342714));
#38908=CARTESIAN_POINT('Ctrl Pts',(73.4169322419408,66.916932241965,-136.808638979169));
#38909=CARTESIAN_POINT('Ctrl Pts',(72.7182901970583,67.4456403378574,-136.522853342713));
#38910=CARTESIAN_POINT('Ctrl Pts',(73.3906608703643,65.8945521744123,-136.79707108069));
#38911=CARTESIAN_POINT('Ctrl Pts',(72.9358474574211,66.435847457458,-136.981577743062));
#38912=CARTESIAN_POINT('Ctrl Pts',(72.3945521743758,66.8906608704009,-136.79707108069));
#38913=CARTESIAN_POINT('Ctrl Pts',(72.2237011525298,65.2138256723439,-137.165672784621));
#38914=CARTESIAN_POINT('Ctrl Pts',(71.9760256068021,65.476025606838,-137.204292118059));
#38915=CARTESIAN_POINT('Ctrl Pts',(71.7138256723076,65.7237011525658,-137.165672784621));
#38916=CARTESIAN_POINT('Ctrl Pts',(71.6119358369269,64.8569625715743,-137.259999999994));
#38917=CARTESIAN_POINT('Ctrl Pts',(71.4844140291782,64.9844140292143,-137.259999999994));
#38918=CARTESIAN_POINT('Ctrl Pts',(71.3569625715387,65.1119358369628,-137.259999999994));
#38919=CARTESIAN_POINT('Ctrl Pts',(70.9999999999945,64.5000000000306,-137.259999999994));
#38920=CARTESIAN_POINT('Ctrl Pts',(70.9999999999945,64.5000000000306,-137.259999999994));
#38921=CARTESIAN_POINT('Ctrl Pts',(70.9999999999945,64.5000000000306,-137.259999999994));
#38922=CARTESIAN_POINT('',(74.4285713427324,66.5000000000331,-136.183910716608));
#38923=CARTESIAN_POINT('Ctrl Pts',(74.4285712566625,66.500000000031,-136.183910592995));
#38924=CARTESIAN_POINT('Ctrl Pts',(74.0993879142635,66.500000000031,-136.413115007304));
#38925=CARTESIAN_POINT('Ctrl Pts',(73.7389825693774,66.500000000031,-136.595514107423));
#38926=CARTESIAN_POINT('Ctrl Pts',(72.9737427869456,66.5000000000309,-136.848440414353));
#38927=CARTESIAN_POINT('Ctrl Pts',(72.5709914841384,66.5000000000308,-136.9167952487));
#38928=CARTESIAN_POINT('Ctrl Pts',(72.166666480424,66.5000000000307,-136.916831899798));
#38929=CARTESIAN_POINT('Ctrl Pts',(70.9999999999945,64.5000000000306,-137.259999999994));
#38930=CARTESIAN_POINT('Ctrl Pts',(71.0957024837609,64.5558264488943,-137.259999999994));
#38931=CARTESIAN_POINT('Ctrl Pts',(71.1885540281554,64.6099898497911,-137.257695594979));
#38932=CARTESIAN_POINT('Ctrl Pts',(71.2784807358408,64.662447095941,-137.253498369066));
#38933=CARTESIAN_POINT('Ctrl Pts',(71.3721446992566,64.7170844079336,-137.249126711029));
#38934=CARTESIAN_POINT('Ctrl Pts',(71.4626358478783,64.7698709112963,-137.242701781837));
#38935=CARTESIAN_POINT('Ctrl Pts',(71.5499081224735,64.8207797381435,-137.23465187225));
#38936=CARTESIAN_POINT('Ctrl Pts',(71.6395131549217,64.873049340405,-137.226386791352));
#38937=CARTESIAN_POINT('Ctrl Pts',(71.7257252428347,64.923339725021,-137.216408761768));
#38938=CARTESIAN_POINT('Ctrl Pts',(71.8085292801494,64.9716420801213,-137.205141858606));
#38939=CARTESIAN_POINT('Ctrl Pts',(71.8898271555678,65.019065840782,-137.194079894489));
#38940=CARTESIAN_POINT('Ctrl Pts',(71.9678403250929,65.064573523005,-137.181775307674));
#38941=CARTESIAN_POINT('Ctrl Pts',(72.0425811727914,65.1081723508292,-137.168593448589));
#38942=CARTESIAN_POINT('Ctrl Pts',(72.1076226249628,65.1461131979292,-137.157122247985));
#38943=CARTESIAN_POINT('Ctrl Pts',(72.1701809791262,65.1826055711912,-137.144986872136));
#38944=CARTESIAN_POINT('Ctrl Pts',(72.2302564698221,65.2176496074305,-137.132412503954));
#38945=CARTESIAN_POINT('Ctrl Pts',(72.3102097945727,65.2642890468684,-137.115677517171));
#38946=CARTESIAN_POINT('Ctrl Pts',(72.3857667799575,65.3083639550095,-137.098166525896));
#38947=CARTESIAN_POINT('Ctrl Pts',(72.4569627922973,65.3498949622077,-137.08036161178));
#38948=CARTESIAN_POINT('Ctrl Pts',(72.5277434635707,65.3911836871171,-137.062660567414));
#38949=CARTESIAN_POINT('Ctrl Pts',(72.5942132886545,65.4299577517494,-137.044669104252));
#38950=CARTESIAN_POINT('Ctrl Pts',(72.6564170382027,65.4662432723191,-137.026812358299));
#38951=CARTESIAN_POINT('Ctrl Pts',(72.7041780482294,65.4941038615013,-137.013101669977));
#38952=CARTESIAN_POINT('Ctrl Pts',(72.749424449516,65.5204975955851,-136.999469395453));
#38953=CARTESIAN_POINT('Ctrl Pts',(72.7921804221301,65.5454385796099,-136.986088323429));
#38954=CARTESIAN_POINT('Ctrl Pts',(72.7937027701776,65.5463266159709,-136.985611883587));
#38955=CARTESIAN_POINT('Ctrl Pts',(72.7942365687616,65.5466380145225,-136.985445020286));
#38956=CARTESIAN_POINT('Ctrl Pts',(72.7967379868563,65.548097175037,-136.984659964278));
#38957=CARTESIAN_POINT('Ctrl Pts',(72.8002217706516,65.5501293821942,-136.983566598318));
#38958=CARTESIAN_POINT('Ctrl Pts',(72.8037027766303,65.5521599690388,-136.982470585208));
#38959=CARTESIAN_POINT('Ctrl Pts',(72.8071810018965,65.5541889338815,-136.981371935672));
#38960=CARTESIAN_POINT('Ctrl Pts',(72.9237260583972,65.622173553661,-136.944559434345));
#38961=CARTESIAN_POINT('Ctrl Pts',(73.0371375340389,65.6883303450419,-136.90479193608));
#38962=CARTESIAN_POINT('Ctrl Pts',(73.1473464497032,65.752619050548,-136.862522044316));
#38963=CARTESIAN_POINT('Ctrl Pts',(73.2595780988789,65.8180876870811,-136.819476346656));
#38964=CARTESIAN_POINT('Ctrl Pts',(73.3684886881679,65.8816191152061,-136.773835536597));
#38965=CARTESIAN_POINT('Ctrl Pts',(73.4740420120092,65.943192153817,-136.726043991574));
#38966=CARTESIAN_POINT('Ctrl Pts',(73.5826686561035,66.0065579703311,-136.67686093449));
#38967=CARTESIAN_POINT('Ctrl Pts',(73.6877397828133,66.0678497509414,-136.625400110897));
#38968=CARTESIAN_POINT('Ctrl Pts',(73.7892526840887,66.1270658118495,-136.572110387094));
#38969=CARTESIAN_POINT('Ctrl Pts',(73.892600078187,66.1873519972184,-136.517857636773));
#38970=CARTESIAN_POINT('Ctrl Pts',(73.9922596634551,66.2454868689079,-136.461709251839));
#38971=CARTESIAN_POINT('Ctrl Pts',(74.0882638810283,66.3014892089543,-136.404102734114));
#38972=CARTESIAN_POINT('Ctrl Pts',(74.1868725239103,66.3590107938365,-136.344933453038));
#38973=CARTESIAN_POINT('Ctrl Pts',(74.2816249422558,66.414282667277,-136.284225864962));
#38974=CARTESIAN_POINT('Ctrl Pts',(74.3725906165779,66.4673451790332,-136.222416363546));
#38975=CARTESIAN_POINT('Ctrl Pts',(74.3914125813985,66.4783244933406,-136.209627184882));
#38976=CARTESIAN_POINT('Ctrl Pts',(74.4100725340541,66.4892092821663,-136.196790704302));
#38977=CARTESIAN_POINT('Ctrl Pts',(74.4285712566605,66.5000000000353,-136.183910592996));
#38978=CARTESIAN_POINT('Origin',(58.999999999994,70.5000000000397,-47.2599999999947));
#38979=CARTESIAN_POINT('',(58.9999999999943,66.5000000000389,-53.2599999999943));
#38980=CARTESIAN_POINT('',(58.999999999994,70.5000000000391,-53.2599999999947));
#38981=CARTESIAN_POINT('',(58.9999999999943,66.5000000000396,-47.6031457505019));
#38982=CARTESIAN_POINT('Origin',(58.9999999999945,64.5000000000389,-53.259999999994));
#38983=CARTESIAN_POINT('',(58.9999999999943,66.5000000000389,-53.2599999999943));
#38984=CARTESIAN_POINT('Origin',(68.999999999994,70.5000000000399,-53.2599999999947));
#38985=CARTESIAN_POINT('',(68.9999999999943,66.5000000000386,-63.2599999999943));
#38986=CARTESIAN_POINT('',(68.999999999994,70.5000000000387,-63.2599999999947));
#38987=CARTESIAN_POINT('Origin',(68.9999999999943,66.5000000000397,-53.2599999999943));
#38988=CARTESIAN_POINT('Origin',(68.999999999994,70.5000000000387,-63.2599999999947));
#38989=CARTESIAN_POINT('',(76.9999999999943,66.5000000000393,-63.2599999999942));
#38990=CARTESIAN_POINT('',(68.9999999999943,66.5000000000386,-63.2599999999942));
#38991=CARTESIAN_POINT('',(76.9999999999942,68.0000000000393,-63.2599999999944));
#38992=CARTESIAN_POINT('',(76.999999999994,70.5000000000394,-63.2599999999947));
#38993=CARTESIAN_POINT('Origin',(74.4999999999942,68.000000000039,-63.2599999999944));
#38994=CARTESIAN_POINT('Origin',(63.2264973080965,85.7752523165588,-53.2599999999964));
#38995=CARTESIAN_POINT('',(63.2264973080981,66.5000000000393,-53.2599999999942));
#38996=CARTESIAN_POINT('',(63.2264973080965,85.7752523165588,-53.2599999999965));
#38997=CARTESIAN_POINT('',(66.1132486540463,66.5000000000401,-48.2599999999942));
#38998=CARTESIAN_POINT('',(63.2264973080981,66.5000000000393,-53.2599999999943));
#38999=CARTESIAN_POINT('',(66.1132486540445,85.7752523165595,-48.2599999999964));
#39000=CARTESIAN_POINT('Origin',(66.1132486540445,85.7752523165595,-48.2599999999964));
#39001=CARTESIAN_POINT('',(71.8867513459424,66.5000000000406,-48.2599999999942));
#39002=CARTESIAN_POINT('',(68.9999999999943,66.5000000000403,-48.2599999999943));
#39003=CARTESIAN_POINT('',(71.8867513459408,85.77525231656,-48.2599999999964));
#39004=CARTESIAN_POINT('Origin',(71.8867513459408,85.77525231656,-48.2599999999964));
#39005=CARTESIAN_POINT('',(74.7735026918906,66.5000000000403,-53.2599999999943));
#39006=CARTESIAN_POINT('',(71.8867513459424,66.5000000000406,-48.2599999999943));
#39007=CARTESIAN_POINT('',(74.7735026918889,85.7752523165598,-53.2599999999965));
#39008=CARTESIAN_POINT('Origin',(74.773502691889,85.7752523165598,-53.2599999999964));
#39009=CARTESIAN_POINT('',(71.8867513459424,66.5000000000394,-58.2599999999942));
#39010=CARTESIAN_POINT('',(74.7735026918906,66.5000000000403,-53.2599999999943));
#39011=CARTESIAN_POINT('',(71.8867513459408,85.7752523165589,-58.2599999999964));
#39012=CARTESIAN_POINT('Origin',(71.8867513459408,85.7752523165589,-58.2599999999964));
#39013=CARTESIAN_POINT('',(66.1132486540463,66.5000000000389,-58.2599999999942));
#39014=CARTESIAN_POINT('',(68.9999999999943,66.5000000000392,-58.2599999999943));
#39015=CARTESIAN_POINT('',(66.1132486540446,85.7752523165584,-58.2599999999965));
#39016=CARTESIAN_POINT('Origin',(66.1132486540445,85.7752523165584,-58.2599999999964));
#39017=CARTESIAN_POINT('',(66.1132486540463,66.5000000000389,-58.2599999999943));
#39018=CARTESIAN_POINT('Origin',(88.6000000000047,-52.7216878364596,-62.9999999999805));
#39019=CARTESIAN_POINT('',(92.4000000000046,-50.5566243269593,-62.9999999999808));
#39020=CARTESIAN_POINT('',(88.6000000000045,-50.5566243269596,-62.9999999999808));
#39021=CARTESIAN_POINT('',(92.4000000000048,-53.4433756729593,-62.9999999999804));
#39022=CARTESIAN_POINT('',(88.6000000000048,-53.4433756729596,-62.9999999999804));
#39023=CARTESIAN_POINT('',(92.4000000000047,-51.9999999999593,-62.9999999999806));
#39024=CARTESIAN_POINT('Origin',(88.6000000000049,-54.1650635094095,-61.7499999999804));
#39025=CARTESIAN_POINT('',(92.4000000000049,-54.886751345859,-60.4999999999803));
#39026=CARTESIAN_POINT('',(88.6000000000049,-54.8867513458593,-60.4999999999803));
#39027=CARTESIAN_POINT('',(92.4000000000048,-53.4433756729593,-62.9999999999804));
#39028=CARTESIAN_POINT('Origin',(88.6000000000049,-54.1650635094092,-59.2499999999804));
#39029=CARTESIAN_POINT('',(92.4000000000048,-53.4433756729587,-57.9999999999804));
#39030=CARTESIAN_POINT('',(88.6000000000048,-53.4433756729591,-57.9999999999804));
#39031=CARTESIAN_POINT('',(92.4000000000049,-54.886751345859,-60.4999999999803));
#39032=CARTESIAN_POINT('Origin',(88.6000000000047,-51.999999999959,-57.9999999999806));
#39033=CARTESIAN_POINT('',(92.4000000000046,-50.5566243269587,-57.9999999999808));
#39034=CARTESIAN_POINT('',(88.6000000000045,-50.5566243269591,-57.9999999999808));
#39035=CARTESIAN_POINT('',(92.4000000000047,-51.9999999999587,-57.9999999999806));
#39036=CARTESIAN_POINT('Origin',(88.6000000000045,-49.8349364905092,-59.2499999999809));
#39037=CARTESIAN_POINT('',(92.4000000000045,-49.113248654059,-60.4999999999809));
#39038=CARTESIAN_POINT('',(88.6000000000044,-49.1132486540593,-60.4999999999809));
#39039=CARTESIAN_POINT('',(92.4000000000046,-50.5566243269587,-57.9999999999808));
#39040=CARTESIAN_POINT('Origin',(88.6000000000045,-49.8349364905095,-61.7499999999809));
#39041=CARTESIAN_POINT('',(92.4000000000045,-49.113248654059,-60.4999999999809));
#39042=CARTESIAN_POINT('Origin',(1.11022302462516E-13,3.94842578771426E-11,
-3.4999999999866));
#39043=CARTESIAN_POINT('Origin',(-95.1999999999911,-100.749999999987,-164.999999999975));
#39044=CARTESIAN_POINT('',(-95.199999999991,-102.193375672988,-167.499999999975));
#39045=CARTESIAN_POINT('',(-95.1999999999908,-103.636751345887,-164.999999999975));
#39046=CARTESIAN_POINT('',(-95.1999999999909,-102.915063509438,-166.249999999975));
#39047=CARTESIAN_POINT('',(-95.199999999991,-102.193375672987,-162.499999999975));
#39048=CARTESIAN_POINT('',(-95.1999999999909,-102.915063509437,-163.749999999975));
#39049=CARTESIAN_POINT('',(-95.1999999999912,-99.3066243269871,-162.499999999975));
#39050=CARTESIAN_POINT('',(-95.1999999999911,-100.749999999987,-162.499999999975));
#39051=CARTESIAN_POINT('',(-95.1999999999913,-97.8632486540874,-164.999999999976));
#39052=CARTESIAN_POINT('',(-95.1999999999913,-98.5849364905373,-163.749999999975));
#39053=CARTESIAN_POINT('',(-95.1999999999912,-99.3066243269877,-167.499999999975));
#39054=CARTESIAN_POINT('',(-95.1999999999913,-98.5849364905376,-166.249999999975));
#39055=CARTESIAN_POINT('',(-95.199999999991,-101.471687836488,-167.499999999975));
#39056=CARTESIAN_POINT('Origin',(-79.9999999999989,-11.1689999999897,-196.499999999986));
#39057=CARTESIAN_POINT('Origin',(1.74860126378462E-12,-18.7858057259555,
-153.999999999984));
#39058=CARTESIAN_POINT('',(74.5682819382939,71.0000000000287,-153.999999999995));
#39059=CARTESIAN_POINT('',(-74.5682819383061,71.0000000000157,-153.999999999995));
#39060=CARTESIAN_POINT('',(-6.07847105982273E-12,71.0000000000222,-153.999999999995));
#39061=CARTESIAN_POINT('',(76.9999999999951,59.5000000000279,-153.999999999993));
#39062=CARTESIAN_POINT('',(75.7841409691445,65.2500000000288,-153.999999999994));
#39063=CARTESIAN_POINT('',(74.6696035241941,69.0000000000287,-153.999999999995));
#39064=CARTESIAN_POINT('',(75.8348017620945,64.2500000000288,-153.999999999994));
#39065=CARTESIAN_POINT('',(-74.6696035242059,69.0000000000157,-153.999999999995));
#39066=CARTESIAN_POINT('',(-5.91193760612896E-12,69.0000000000222,-153.999999999995));
#39067=CARTESIAN_POINT('',(-77.0000000000051,59.5000000000154,-153.999999999993));
#39068=CARTESIAN_POINT('',(-75.8348017621055,64.2500000000156,-153.999999999994));
#39069=CARTESIAN_POINT('',(-75.7841409691556,65.2500000000156,-153.999999999994));
#39070=CARTESIAN_POINT('Origin',(-6.07847105982273E-12,71.0000000000233,
-143.999999999995));
#39071=CARTESIAN_POINT('',(-74.5682819383061,71.0000000000168,-143.999999999995));
#39072=CARTESIAN_POINT('',(74.5682819382939,71.0000000000298,-143.999999999995));
#39073=CARTESIAN_POINT('',(-6.07847105982273E-12,71.0000000000233,-143.999999999995));
#39074=CARTESIAN_POINT('',(74.5682819382939,71.0000000000298,-143.999999999995));
#39075=CARTESIAN_POINT('',(-74.5682819383061,71.0000000000168,-143.999999999995));
#39076=CARTESIAN_POINT('Origin',(1.74860126378462E-12,-18.7858057259544,
-143.999999999984));
#39077=CARTESIAN_POINT('',(77.0000000000095,59.4999999999543,-143.999999999993));
#39078=CARTESIAN_POINT('',(75.7841409691445,65.2500000000299,-143.999999999994));
#39079=CARTESIAN_POINT('',(-77.0000000000013,59.500000000037,-143.999999999993));
#39080=CARTESIAN_POINT('',(-75.7841409691556,65.2500000000167,-143.999999999994));
#39081=CARTESIAN_POINT('',(-74.6696035242059,69.0000000000168,-143.999999999994));
#39082=CARTESIAN_POINT('',(-75.8348017621055,64.2500000000167,-143.999999999994));
#39083=CARTESIAN_POINT('',(74.6696035241941,69.0000000000298,-143.999999999994));
#39084=CARTESIAN_POINT('',(-5.91193760612896E-12,69.0000000000233,-143.999999999994));
#39085=CARTESIAN_POINT('',(75.8348017620945,64.2500000000299,-143.999999999994));
#39086=CARTESIAN_POINT('Origin',(-5.91193760612896E-12,69.0000000000237,
-140.499999999994));
#39087=CARTESIAN_POINT('',(-74.6696035242059,69.0000000000172,-140.499999999994));
#39088=CARTESIAN_POINT('',(74.6696035241941,69.0000000000302,-140.499999999994));
#39089=CARTESIAN_POINT('',(-5.91193760612896E-12,69.0000000000237,-140.499999999994));
#39090=CARTESIAN_POINT('',(74.6696035241941,69.0000000000302,-140.499999999994));
#39091=CARTESIAN_POINT('',(-74.6696035242059,69.0000000000172,-140.499999999994));
#39092=CARTESIAN_POINT('Origin',(-68.5000000000024,28.778312163529,-43.2999999999899));
#39093=CARTESIAN_POINT('',(-68.5000000000023,28.056624327029,-43.4999999999899));
#39094=CARTESIAN_POINT('',(-68.5000000000023,28.056624327029,-43.2999999999898));
#39095=CARTESIAN_POINT('',(-68.5000000000026,30.943375673029,-43.4999999999902));
#39096=CARTESIAN_POINT('',(-68.5000000000026,30.943375673029,-43.2999999999901));
#39097=CARTESIAN_POINT('',(-68.5000000000025,29.5000000000289,-43.49999999999));
#39098=CARTESIAN_POINT('Origin',(-67.2500000000026,31.6650635094791,-43.2999999999902));
#39099=CARTESIAN_POINT('',(-66.0000000000027,32.3867513459292,-43.4999999999904));
#39100=CARTESIAN_POINT('',(-66.0000000000027,32.3867513459292,-43.2999999999903));
#39101=CARTESIAN_POINT('',(-68.5000000000026,30.943375673029,-43.4999999999902));
#39102=CARTESIAN_POINT('Origin',(-64.7500000000026,31.6650635094792,-43.2999999999902));
#39103=CARTESIAN_POINT('',(-63.5000000000026,30.9433756730294,-43.4999999999902));
#39104=CARTESIAN_POINT('',(-63.5000000000026,30.9433756730294,-43.2999999999901));
#39105=CARTESIAN_POINT('',(-66.0000000000027,32.3867513459292,-43.4999999999904));
#39106=CARTESIAN_POINT('Origin',(-63.5000000000025,29.5000000000294,-43.29999999999));
#39107=CARTESIAN_POINT('',(-63.5000000000023,28.0566243270294,-43.4999999999899));
#39108=CARTESIAN_POINT('',(-63.5000000000023,28.0566243270294,-43.2999999999898));
#39109=CARTESIAN_POINT('',(-63.5000000000025,29.5000000000294,-43.49999999999));
#39110=CARTESIAN_POINT('Origin',(-64.7500000000023,27.3349364905792,-43.2999999999898));
#39111=CARTESIAN_POINT('',(-66.0000000000022,26.6132486541292,-43.4999999999897));
#39112=CARTESIAN_POINT('',(-66.0000000000022,26.6132486541292,-43.2999999999896));
#39113=CARTESIAN_POINT('',(-63.5000000000023,28.0566243270294,-43.4999999999899));
#39114=CARTESIAN_POINT('Origin',(-67.2500000000023,27.3349364905791,-43.2999999999898));
#39115=CARTESIAN_POINT('',(-66.0000000000022,26.6132486541292,-43.4999999999897));
#39116=CARTESIAN_POINT('Origin',(84.2000000000047,-52.72168783646,-62.9999999999805));
#39117=CARTESIAN_POINT('',(84.4000000000048,-53.0627460667662,-62.9999999999805));
#39118=CARTESIAN_POINT('',(85.0000000000047,-52.4302858857085,-62.9999999999805));
#39119=CARTESIAN_POINT('Origin',(93.4000000000055,-60.9999999999592,-62.9999999999796));
#39120=CARTESIAN_POINT('',(84.4000000000048,-53.44337567296,-62.9999999999804));
#39121=CARTESIAN_POINT('',(84.4000000000047,-52.72168783646,-62.9999999999805));
#39122=CARTESIAN_POINT('',(84.2000000000048,-53.44337567296,-62.9999999999804));
#39123=CARTESIAN_POINT('',(85.0000000000045,-50.55662432696,-62.9999999999808));
#39124=CARTESIAN_POINT('',(84.2000000000046,-50.55662432696,-62.9999999999808));
#39125=CARTESIAN_POINT('',(85.0000000000052,-57.49999999996,-62.99999999998));
#39126=CARTESIAN_POINT('Origin',(84.2000000000045,-49.8349364905099,-61.7499999999809));
#39127=CARTESIAN_POINT('',(85.0000000000044,-49.1132486540597,-60.4999999999809));
#39128=CARTESIAN_POINT('',(84.2000000000044,-49.1132486540597,-60.4999999999809));
#39129=CARTESIAN_POINT('',(85.0000000000045,-50.55662432696,-62.9999999999808));
#39130=CARTESIAN_POINT('Origin',(84.2000000000045,-49.8349364905096,-59.2499999999809));
#39131=CARTESIAN_POINT('',(85.0000000000045,-50.5566243269594,-57.9999999999808));
#39132=CARTESIAN_POINT('',(84.2000000000046,-50.5566243269594,-57.9999999999808));
#39133=CARTESIAN_POINT('',(85.0000000000044,-49.1132486540597,-60.4999999999809));
#39134=CARTESIAN_POINT('Origin',(84.2000000000047,-51.9999999999594,-57.9999999999806));
#39135=CARTESIAN_POINT('',(84.4000000000048,-53.4433756729594,-57.9999999999804));
#39136=CARTESIAN_POINT('',(84.2000000000048,-53.4433756729594,-57.9999999999804));
#39137=CARTESIAN_POINT('',(84.4000000000048,-53.0627460667657,-57.9999999999805));
#39138=CARTESIAN_POINT('',(84.4000000000047,-51.9999999999594,-57.9999999999806));
#39139=CARTESIAN_POINT('',(85.0000000000047,-52.430285885708,-57.9999999999806));
#39140=CARTESIAN_POINT('Origin',(93.4000000000055,-60.9999999999586,-57.9999999999796));
#39141=CARTESIAN_POINT('',(85.0000000000052,-57.4999999999594,-57.99999999998));
#39142=CARTESIAN_POINT('Origin',(84.2000000000049,-54.1650635094096,-59.2499999999804));
#39143=CARTESIAN_POINT('',(84.4000000000049,-54.8867513458597,-60.4999999999803));
#39144=CARTESIAN_POINT('',(84.2000000000049,-54.8867513458597,-60.4999999999803));
#39145=CARTESIAN_POINT('',(84.4000000000048,-53.4433756729594,-57.9999999999804));
#39146=CARTESIAN_POINT('Origin',(84.2000000000049,-54.1650635094099,-61.7499999999804));
#39147=CARTESIAN_POINT('',(84.4000000000049,-54.8867513458597,-60.4999999999803));
#39148=CARTESIAN_POINT('Origin',(-92.4,2.17484450587558E-11,-87.4999999999866));
#39149=CARTESIAN_POINT('Origin',(-74.5000000000058,68.0000000000179,-137.259999999994));
#39150=CARTESIAN_POINT('',(-77.0000000000058,68.0000000000177,-137.259999999994));
#39151=CARTESIAN_POINT('Origin',(-69.0000000000057,66.5000000000191,-131.259999999994));
#39152=CARTESIAN_POINT('',(-77.0000000000057,66.5000000000183,-131.259999999994));
#39153=CARTESIAN_POINT('Origin',(-71.0000000000057,66.5000000000189,-131.259999999994));
#39154=CARTESIAN_POINT('',(-77.0000000000057,66.5000000000177,-137.259999999994));
#39155=CARTESIAN_POINT('Ctrl Pts',(-74.4465182387269,66.5104689726153,-48.3486344027126));
#39156=CARTESIAN_POINT('Ctrl Pts',(-73.8703570864329,67.3703570864552,-47.9443171348385));
#39157=CARTESIAN_POINT('Ctrl Pts',(-73.0104689725931,67.9465182387492,-48.3486344027127));
#39158=CARTESIAN_POINT('Ctrl Pts',(-73.9456403378346,66.2182901970878,-47.9971466572771));
#39159=CARTESIAN_POINT('Ctrl Pts',(-73.4169322419534,66.9169322419637,-47.7113610208082));
#39160=CARTESIAN_POINT('Ctrl Pts',(-72.718290197077,67.4456403378527,-47.9971466572743));
#39161=CARTESIAN_POINT('Ctrl Pts',(-73.3906608703745,65.8945521744096,-47.7229289192979));
#39162=CARTESIAN_POINT('Ctrl Pts',(-72.9358474574371,66.4358474574548,-47.5384222569253));
#39163=CARTESIAN_POINT('Ctrl Pts',(-72.3945521743876,66.8906608703965,-47.7229289192978));
#39164=CARTESIAN_POINT('Ctrl Pts',(-72.2237011525419,65.2138256723413,-47.3543272153676));
#39165=CARTESIAN_POINT('Ctrl Pts',(-71.9760256068088,65.476025606836,-47.3157078819302));
#39166=CARTESIAN_POINT('Ctrl Pts',(-71.7138256723184,65.7237011525651,-47.3543272153679));
#39167=CARTESIAN_POINT('Ctrl Pts',(-71.6119358369362,64.8569625715737,-47.2599999999941));
#39168=CARTESIAN_POINT('Ctrl Pts',(-71.4844140291975,64.984414029207,-47.2599999999941));
#39169=CARTESIAN_POINT('Ctrl Pts',(-71.3569625715513,65.1119358369585,-47.2599999999941));
#39170=CARTESIAN_POINT('Ctrl Pts',(-71.0000000000055,64.5000000000283,-47.259999999994));
#39171=CARTESIAN_POINT('Ctrl Pts',(-71.0000000000055,64.5000000000283,-47.259999999994));
#39172=CARTESIAN_POINT('Ctrl Pts',(-71.0000000000055,64.5000000000283,-47.259999999994));
#39173=CARTESIAN_POINT('',(-74.4285713427437,66.50000000003,-48.3360892833802));
#39174=CARTESIAN_POINT('',(-72.1666664804358,66.5000000000282,-47.603168100191));
#39175=CARTESIAN_POINT('Ctrl Pts',(-74.4285712566737,66.5000000000279,-48.336089406994));
#39176=CARTESIAN_POINT('Ctrl Pts',(-74.099387914276,66.5000000000279,-48.1068849926858));
#39177=CARTESIAN_POINT('Ctrl Pts',(-73.7389825693898,66.500000000028,-47.9244858925642));
#39178=CARTESIAN_POINT('Ctrl Pts',(-72.9737427869555,66.5000000000281,-47.6715595856325));
#39179=CARTESIAN_POINT('Ctrl Pts',(-72.5709914841508,66.5000000000281,-47.6032047512884));
#39180=CARTESIAN_POINT('Ctrl Pts',(-72.1666664804358,66.5000000000282,-47.603168100191));
#39181=CARTESIAN_POINT('',(-71.0000000000055,64.5000000000283,-47.259999999994));
#39182=CARTESIAN_POINT('Ctrl Pts',(-71.0000000000055,64.5000000000283,-47.259999999994));
#39183=CARTESIAN_POINT('Ctrl Pts',(-71.0957024839778,64.5558264490125,-47.259999999994));
#39184=CARTESIAN_POINT('Ctrl Pts',(-71.1885540285871,64.6099898500349,-47.2623044050192));
#39185=CARTESIAN_POINT('Ctrl Pts',(-71.278480736496,64.6624470963152,-47.2665016309523));
#39186=CARTESIAN_POINT('Ctrl Pts',(-71.3721447001262,64.7170844084331,-47.270873289009));
#39187=CARTESIAN_POINT('Ctrl Pts',(-71.4626358489729,64.769870911927,-47.2772982182316));
#39188=CARTESIAN_POINT('Ctrl Pts',(-71.5499081238032,64.8207797389114,-47.2853481278595));
#39189=CARTESIAN_POINT('Ctrl Pts',(-71.6395131564995,64.8730493413176,-47.2936132088008));
#39190=CARTESIAN_POINT('Ctrl Pts',(-71.7257252446709,64.9233397260842,-47.3035912384393));
#39191=CARTESIAN_POINT('Ctrl Pts',(-71.8085292822539,64.9716420813409,-47.3148581416667));
#39192=CARTESIAN_POINT('Ctrl Pts',(-71.8898271580062,65.0190658421964,-47.3259201058587));
#39193=CARTESIAN_POINT('Ctrl Pts',(-71.9678403278692,65.0645735246163,-47.3382246927615));
#39194=CARTESIAN_POINT('Ctrl Pts',(-72.0425811759093,65.1081723526396,-47.3514065519475));
#39195=CARTESIAN_POINT('Ctrl Pts',(-72.1076226269018,65.1461131990518,-47.3628777523782));
#39196=CARTESIAN_POINT('Ctrl Pts',(-72.1701809800006,65.1826055716927,-47.3750131280339));
#39197=CARTESIAN_POINT('Ctrl Pts',(-72.2302564697472,65.2176496073781,-47.3875874960164));
#39198=CARTESIAN_POINT('Ctrl Pts',(-72.3102097951455,65.2642890471937,-47.4043224829341));
#39199=CARTESIAN_POINT('Ctrl Pts',(-72.3857667811711,65.3083639557085,-47.4218334743689));
#39200=CARTESIAN_POINT('Ctrl Pts',(-72.4569627941448,65.3498949632764,-47.4396383886675));
#39201=CARTESIAN_POINT('Ctrl Pts',(-72.5277434860066,65.3911837001956,-47.4573394382061));
#39202=CARTESIAN_POINT('Ctrl Pts',(-72.59421332924,65.4299577754151,-47.4753309067242));
#39203=CARTESIAN_POINT('Ctrl Pts',(-72.6564170945389,65.4662433051727,-47.4931876578589));
#39204=CARTESIAN_POINT('Ctrl Pts',(-72.7041780837353,65.4941038822038,-47.5068983407079));
#39205=CARTESIAN_POINT('Ctrl Pts',(-72.7494244662453,65.5204976053346,-47.5205306097676));
#39206=CARTESIAN_POINT('Ctrl Pts',(-72.7921804221062,65.5454385795868,-47.5339116765479));
#39207=CARTESIAN_POINT('Ctrl Pts',(-72.7937027701653,65.5463266159546,-47.5343881163943));
#39208=CARTESIAN_POINT('Ctrl Pts',(-72.7942365687792,65.5466380145231,-47.5345549797046));
#39209=CARTESIAN_POINT('Ctrl Pts',(-72.7967379868677,65.548097175034,-47.5353400357101));
#39210=CARTESIAN_POINT('Ctrl Pts',(-72.8002217706629,65.5501293821912,-47.5364334016704));
#39211=CARTESIAN_POINT('Ctrl Pts',(-72.8037027766417,65.5521599690358,-47.5375294147803));
#39212=CARTESIAN_POINT('Ctrl Pts',(-72.807181001908,65.5541889338785,-47.5386280643162));
#39213=CARTESIAN_POINT('Ctrl Pts',(-72.9237260589525,65.6221735539754,-47.5754405658148));
#39214=CARTESIAN_POINT('Ctrl Pts',(-73.0371375351493,65.68833034568,-47.6152080642929));
#39215=CARTESIAN_POINT('Ctrl Pts',(-73.1473464513777,65.7526190515151,-47.6574779563107));
#39216=CARTESIAN_POINT('Ctrl Pts',(-73.2595781011115,65.8180876883735,-47.7005236542232));
#39217=CARTESIAN_POINT('Ctrl Pts',(-73.3684886909689,65.8816191168299,-47.7461644645764));
#39218=CARTESIAN_POINT('Ctrl Pts',(-73.4740420153865,65.9431921557768,-47.7939560099388));
#39219=CARTESIAN_POINT('Ctrl Pts',(-73.5826686600627,66.0065579726303,-47.8431390673672));
#39220=CARTESIAN_POINT('Ctrl Pts',(-73.6877397873635,66.0678497535853,-47.8945998913498));
#39221=CARTESIAN_POINT('Ctrl Pts',(-73.7892526892365,66.1270658148421,-47.9478896155913));
#39222=CARTESIAN_POINT('Ctrl Pts',(-73.892600083934,66.1873520005605,-48.002142366354));
#39223=CARTESIAN_POINT('Ctrl Pts',(-73.9922596698087,66.2454868726039,-48.0582907517788));
#39224=CARTESIAN_POINT('Ctrl Pts',(-74.088263887993,66.3014892130069,-48.1158972700473));
#39225=CARTESIAN_POINT('Ctrl Pts',(-74.1868725314681,66.3590107982352,-48.1750665516603));
#39226=CARTESIAN_POINT('Ctrl Pts',(-74.2816249504143,66.4142826720263,-48.2357741403271));
#39227=CARTESIAN_POINT('Ctrl Pts',(-74.3725906253415,66.4673451841354,-48.2975836423898));
#39228=CARTESIAN_POINT('Ctrl Pts',(-74.3914125871913,66.4783244967099,-48.3103728190844));
#39229=CARTESIAN_POINT('Ctrl Pts',(-74.4100725369295,66.4892092838339,-48.3232092976808));
#39230=CARTESIAN_POINT('Ctrl Pts',(-74.4285712566717,66.5000000000321,-48.3360894069926));
#39231=CARTESIAN_POINT('Origin',(-71.1248546100925,64.7150556883937,-51.8728787160349));
#39232=CARTESIAN_POINT('Origin',(-69.0000000000057,66.5000000000278,-53.2599999999943));
#39233=CARTESIAN_POINT('',(74.4999999999943,66.5000000000409,-47.6031457505019));
#39234=CARTESIAN_POINT('',(-77.0000000000057,66.5000000000271,-53.2599999999943));
#39235=CARTESIAN_POINT('',(-77.0000000000057,66.5000000000174,-137.259999999994));
#39236=CARTESIAN_POINT('Origin',(-71.0000000000057,66.5000000000276,-53.2599999999943));
#39237=CARTESIAN_POINT('Origin',(74.4999999999945,64.5000000000403,-53.259999999994));
#39238=CARTESIAN_POINT('',(70.9999999999945,64.5000000000407,-47.259999999994));
#39239=CARTESIAN_POINT('',(74.4999999999945,64.500000000041,-47.259999999994));
#39240=CARTESIAN_POINT('',(72.1666666657488,66.4999964869591,-47.6031556827593));
#39241=CARTESIAN_POINT('Origin',(71.1254680349722,64.7151828220995,-51.8829521166587));
#39242=CARTESIAN_POINT('',(68.9999999999943,66.5000000000404,-47.6031457505019));
#39243=CARTESIAN_POINT('Ctrl Pts',(73.0104689725816,67.9465182387619,-48.3486344027127));
#39244=CARTESIAN_POINT('Ctrl Pts',(73.8703570864216,67.3703570864681,-47.9443171348386));
#39245=CARTESIAN_POINT('Ctrl Pts',(74.4465182387155,66.5104689726283,-48.3486344027126));
#39246=CARTESIAN_POINT('Ctrl Pts',(72.7182901970595,67.4456403378679,-47.9971466572761));
#39247=CARTESIAN_POINT('Ctrl Pts',(73.4169322419358,66.9169322419847,-47.7113610208115));
#39248=CARTESIAN_POINT('Ctrl Pts',(73.9456403378217,66.2182901971061,-47.9971466572759));
#39249=CARTESIAN_POINT('Ctrl Pts',(72.3945521743758,66.8906608704091,-47.7229289192979));
#39250=CARTESIAN_POINT('Ctrl Pts',(72.935847457421,66.4358474574675,-47.5384222569253));
#39251=CARTESIAN_POINT('Ctrl Pts',(73.3906608703627,65.8945521744223,-47.7229289192977));
#39252=CARTESIAN_POINT('Ctrl Pts',(71.7138256723076,65.7237011525775,-47.3543272153679));
#39253=CARTESIAN_POINT('Ctrl Pts',(71.9760256068023,65.4760256068485,-47.3157078819302));
#39254=CARTESIAN_POINT('Ctrl Pts',(72.2237011525313,65.213825672354,-47.3543272153678));
#39255=CARTESIAN_POINT('Ctrl Pts',(71.356962571538,65.1119358369719,-47.2599999999941));
#39256=CARTESIAN_POINT('Ctrl Pts',(71.484414029178,64.9844140292242,-47.2599999999941));
#39257=CARTESIAN_POINT('Ctrl Pts',(71.611935836926,64.8569625715837,-47.2599999999941));
#39258=CARTESIAN_POINT('Ctrl Pts',(70.9999999999945,64.5000000000407,-47.259999999994));
#39259=CARTESIAN_POINT('Ctrl Pts',(70.9999999999945,64.5000000000407,-47.259999999994));
#39260=CARTESIAN_POINT('Ctrl Pts',(70.9999999999945,64.5000000000407,-47.259999999994));
#39261=CARTESIAN_POINT('',(74.4285713480745,66.4999999932162,-48.3360892871001));
#39262=CARTESIAN_POINT('Ctrl Pts',(74.4285712620025,66.4999999864476,-48.3360894107125));
#39263=CARTESIAN_POINT('Ctrl Pts',(74.3391637338871,66.4478465859688,-48.2738376033375));
#39264=CARTESIAN_POINT('Ctrl Pts',(74.2459677055059,66.3934823583403,-48.2125887205665));
#39265=CARTESIAN_POINT('Ctrl Pts',(74.1489208797793,66.3368715557003,-48.1527836871288));
#39266=CARTESIAN_POINT('Ctrl Pts',(74.0544352045465,66.2817547615872,-48.0945569607586));
#39267=CARTESIAN_POINT('Ctrl Pts',(73.956299171396,66.2245083315743,-48.037698915775));
#39268=CARTESIAN_POINT('Ctrl Pts',(73.8544881414612,66.1651183120502,-47.9826477669765));
#39269=CARTESIAN_POINT('Ctrl Pts',(73.7991623958305,66.1328448234576,-47.9527320902855));
#39270=CARTESIAN_POINT('Ctrl Pts',(73.7427520064248,66.0999386704583,-47.9233505363308));
#39271=CARTESIAN_POINT('Ctrl Pts',(73.6852574698426,66.0664001907854,-47.8945774142381));
#39272=CARTESIAN_POINT('Ctrl Pts',(73.5833222344415,66.0069379701348,-47.8435639589066));
#39273=CARTESIAN_POINT('Ctrl Pts',(73.4779732668583,65.9454844057112,-47.7944589336936));
#39274=CARTESIAN_POINT('Ctrl Pts',(73.3692181538548,65.8820439231259,-47.7476920278763));
#39275=CARTESIAN_POINT('Ctrl Pts',(73.253269855067,65.8144074154997,-47.6978319061833));
#39276=CARTESIAN_POINT('Ctrl Pts',(73.1334511946194,65.7445131969053,-47.650629358033));
#39277=CARTESIAN_POINT('Ctrl Pts',(73.0098028923415,65.6723850205766,-47.6066455570301));
#39278=CARTESIAN_POINT('Ctrl Pts',(72.9433637836261,65.633628873826,-47.5830120377442));
#39279=CARTESIAN_POINT('Ctrl Pts',(72.8758195809709,65.5942280889438,-47.5603085874872));
#39280=CARTESIAN_POINT('Ctrl Pts',(72.807181011447,65.5541889233882,-47.5386280673328));
#39281=CARTESIAN_POINT('Ctrl Pts',(72.8062002761214,65.5536168277816,-47.5383182873921));
#39282=CARTESIAN_POINT('Ctrl Pts',(72.8052193178106,65.5530446021003,-47.5380087164549));
#39283=CARTESIAN_POINT('Ctrl Pts',(72.8042381365091,65.552472246341,-47.5376993547426));
#39284=CARTESIAN_POINT('Ctrl Pts',(72.8017395376703,65.5510147303518,-47.53691155863));
#39285=CARTESIAN_POINT('Ctrl Pts',(72.7982538835186,65.548981439446,-47.5358157913566));
#39286=CARTESIAN_POINT('Ctrl Pts',(72.7967379885827,65.5480971731505,-47.5353400362519));
#39287=CARTESIAN_POINT('Ctrl Pts',(72.7414940634015,65.5158717596956,-47.5180020408631));
#39288=CARTESIAN_POINT('Ctrl Pts',(72.6820631077528,65.4812037731397,-47.5002309153228));
#39289=CARTESIAN_POINT('Ctrl Pts',(72.6183862745531,65.4440589605577,-47.4824061897516));
#39290=CARTESIAN_POINT('Ctrl Pts',(72.5555242019548,65.4073894249063,-47.4648095358888));
#39291=CARTESIAN_POINT('Ctrl Pts',(72.4885237162915,65.3683057529095,-47.4471607251225));
#39292=CARTESIAN_POINT('Ctrl Pts',(72.4173412032736,65.3267825597032,-47.4298727707195));
#39293=CARTESIAN_POINT('Ctrl Pts',(72.3480489855588,65.2863620403667,-47.4130439085518));
#39294=CARTESIAN_POINT('Ctrl Pts',(72.2747934780487,65.2436295973518,-47.3965571621923));
#39295=CARTESIAN_POINT('Ctrl Pts',(72.197553521247,65.1985729201613,-47.3808371571426));
#39296=CARTESIAN_POINT('Ctrl Pts',(72.152211288388,65.1721232633565,-47.3716090301599));
#39297=CARTESIAN_POINT('Ctrl Pts',(72.1054963841207,65.144872890781,-47.3626459384347));
#39298=CARTESIAN_POINT('Ctrl Pts',(72.0574086329714,65.1168217026105,-47.3540407565818));
#39299=CARTESIAN_POINT('Ctrl Pts',(71.9810177499806,65.0722603541992,-47.3403708006298));
#39300=CARTESIAN_POINT('Ctrl Pts',(71.9011695186989,65.0256822192849,-47.327603429021));
#39301=CARTESIAN_POINT('Ctrl Pts',(71.817849159319,64.9770786763137,-47.3161336846326));
#39302=CARTESIAN_POINT('Ctrl Pts',(71.7364284542443,64.9295832650206,-47.3049254435486));
#39303=CARTESIAN_POINT('Ctrl Pts',(71.6516918266631,64.8801535655991,-47.2949563745174));
#39304=CARTESIAN_POINT('Ctrl Pts',(71.5636524184613,64.828797244149,-47.2866318029957));
#39305=CARTESIAN_POINT('Ctrl Pts',(71.4761672846119,64.7777642494044,-47.2783596409185));
#39306=CARTESIAN_POINT('Ctrl Pts',(71.3854204261458,64.7248285819669,-47.271711271297));
#39307=CARTESIAN_POINT('Ctrl Pts',(71.2914570354089,64.6700166040371,-47.2671213880119));
#39308=CARTESIAN_POINT('Ctrl Pts',(71.197493644672,64.6152046261073,-47.2625315047268));
#39309=CARTESIAN_POINT('Ctrl Pts',(71.1003132529705,64.5585160642805,-47.259999999994));
#39310=CARTESIAN_POINT('Ctrl Pts',(70.9999999999945,64.5000000000407,-47.259999999994));
#39311=CARTESIAN_POINT('Ctrl Pts',(74.4285712620046,66.5000000000409,-48.3360894107137));
#39312=CARTESIAN_POINT('Ctrl Pts',(74.0993880304052,66.5000000000409,-48.1068850728108));
#39313=CARTESIAN_POINT('Ctrl Pts',(73.7389828108834,66.5000000000408,-47.9244860147235));
#39314=CARTESIAN_POINT('Ctrl Pts',(72.9737426228402,66.5000000000408,-47.6715594885888));
#39315=CARTESIAN_POINT('Ctrl Pts',(72.5709915200155,66.5000000000408,-47.6032047722343));
#39316=CARTESIAN_POINT('Ctrl Pts',(72.166666665823,66.5000000000407,-47.6031681002079));
#39317=CARTESIAN_POINT('Origin',(1.83186799063151E-12,-19.6933104181538,
-140.499999999984));
#39318=CARTESIAN_POINT('',(76.9999999999949,59.5000000000303,-140.499999999993));
#39319=CARTESIAN_POINT('',(75.8348017620945,64.2500000000304,-140.499999999994));
#39320=CARTESIAN_POINT('',(-77.0000000000051,59.5000000000171,-140.499999999993));
#39321=CARTESIAN_POINT('',(-75.8348017621055,64.2500000000171,-140.499999999994));
#39322=CARTESIAN_POINT('',(-5.07927033766009E-12,59.5000000000237,-140.499999999993));
#39323=CARTESIAN_POINT('Origin',(-71.0000000000058,68.0000000000186,-131.259999999994));
#39324=CARTESIAN_POINT('',(-77.000000000005,59.5000000000182,-131.259999999993));
#39325=CARTESIAN_POINT('',(-71.0000000000051,59.500000000018,-137.259999999993));
#39326=CARTESIAN_POINT('Origin',(-71.0000000000051,59.5000000000188,-131.259999999993));
#39327=CARTESIAN_POINT('',(-77.0000000000058,68.0000000000184,-131.259999999994));
#39328=CARTESIAN_POINT('',(-71.0000000000058,68.0000000000182,-137.259999999994));
#39329=CARTESIAN_POINT('Origin',(74.4999999999942,68.0000000000309,-137.259999999994));
#39330=CARTESIAN_POINT('',(70.9999999999949,59.5000000000305,-137.259999999993));
#39331=CARTESIAN_POINT('',(-5.07927033766009E-12,59.5000000000241,-137.259999999993));
#39332=CARTESIAN_POINT('',(70.9999999999942,68.0000000000307,-137.259999999994));
#39333=CARTESIAN_POINT('Origin',(74.4999999999942,68.0000000000309,-137.259999999994));
#39334=CARTESIAN_POINT('',(76.9999999999942,68.0000000000308,-137.259999999994));
#39335=CARTESIAN_POINT('Origin',(68.9999999999943,66.5000000000311,-131.259999999994));
#39336=CARTESIAN_POINT('',(76.9999999999943,66.5000000000318,-131.259999999994));
#39337=CARTESIAN_POINT('',(76.9999999999943,66.5000000000311,-137.259999999994));
#39338=CARTESIAN_POINT('Origin',(70.9999999999943,66.5000000000313,-131.259999999994));
#39339=CARTESIAN_POINT('Origin',(70.9999999999942,68.0000000000313,-131.259999999994));
#39340=CARTESIAN_POINT('',(76.9999999999949,59.5000000000317,-131.259999999993));
#39341=CARTESIAN_POINT('Origin',(70.9999999999949,59.5000000000313,-131.259999999993));
#39342=CARTESIAN_POINT('',(76.9999999999949,59.5000000000318,-131.259999999993));
#39343=CARTESIAN_POINT('Origin',(68.9999999999943,66.5000000000398,-53.2599999999943));
#39344=CARTESIAN_POINT('',(76.9999999999943,66.5000000000405,-53.2599999999942));
#39345=CARTESIAN_POINT('Origin',(70.9999999999944,66.50000000004,-53.2599999999942));
#39346=CARTESIAN_POINT('',(76.9999999999943,66.5000000000308,-137.259999999994));
#39347=CARTESIAN_POINT('Origin',(92.4000000000047,-51.999999999959,-60.4999999999806));
#39348=CARTESIAN_POINT('Origin',(-99.199999999991,-101.471687836488,-167.499999999975));
#39349=CARTESIAN_POINT('',(-98.999999999991,-102.193375672988,-167.499999999975));
#39350=CARTESIAN_POINT('',(-99.199999999991,-102.193375672988,-167.499999999975));
#39351=CARTESIAN_POINT('',(-98.9999999999912,-99.306624326988,-167.499999999975));
#39352=CARTESIAN_POINT('',(-99.1999999999912,-99.3066243269881,-167.499999999975));
#39353=CARTESIAN_POINT('',(-98.9999999999911,-100.749999999988,-167.499999999975));
#39354=CARTESIAN_POINT('Origin',(-99.1999999999913,-98.5849364905379,-166.249999999975));
#39355=CARTESIAN_POINT('',(-98.9999999999913,-97.8632486540878,-164.999999999976));
#39356=CARTESIAN_POINT('',(-99.1999999999914,-97.8632486540878,-164.999999999976));
#39357=CARTESIAN_POINT('',(-98.9999999999912,-99.306624326988,-167.499999999975));
#39358=CARTESIAN_POINT('Origin',(-99.1999999999913,-98.5849364905376,-163.749999999975));
#39359=CARTESIAN_POINT('',(-98.9999999999912,-99.3066243269875,-162.499999999975));
#39360=CARTESIAN_POINT('',(-99.1999999999912,-99.3066243269875,-162.499999999975));
#39361=CARTESIAN_POINT('',(-98.9999999999913,-97.8632486540878,-164.999999999976));
#39362=CARTESIAN_POINT('Origin',(-99.1999999999911,-100.749999999987,-162.499999999975));
#39363=CARTESIAN_POINT('',(-98.999999999991,-102.193375672987,-162.499999999975));
#39364=CARTESIAN_POINT('',(-99.199999999991,-102.193375672987,-162.499999999975));
#39365=CARTESIAN_POINT('',(-98.9999999999911,-100.749999999987,-162.499999999975));
#39366=CARTESIAN_POINT('Origin',(-99.1999999999909,-102.915063509438,-163.749999999975));
#39367=CARTESIAN_POINT('',(-98.9999999999908,-103.636751345888,-164.999999999975));
#39368=CARTESIAN_POINT('',(-99.1999999999908,-103.636751345888,-164.999999999975));
#39369=CARTESIAN_POINT('',(-98.999999999991,-102.193375672987,-162.499999999975));
#39370=CARTESIAN_POINT('Origin',(-99.1999999999909,-102.915063509438,-166.249999999975));
#39371=CARTESIAN_POINT('',(-98.9999999999908,-103.636751345888,-164.999999999975));
#39372=CARTESIAN_POINT('Origin',(-75.8348017621055,64.2500000000171,-140.499999999994));
#39373=CARTESIAN_POINT('',(-77.0000000000051,59.500000000017,-140.499999999993));
#39374=CARTESIAN_POINT('Origin',(-75.7841409691556,65.2500000000167,-143.999999999994));
#39375=CARTESIAN_POINT('',(-77.0000000000051,59.5000000000166,-143.999999999993));
#39376=CARTESIAN_POINT('Origin',(-75.8348017621055,64.2500000000171,-140.499999999994));
#39377=CARTESIAN_POINT('',(-77.0000000000053,59.5000000000123,-172.499999999994));
#39378=CARTESIAN_POINT('',(-74.6696035242059,69.0000000000135,-172.499999999995));
#39379=CARTESIAN_POINT('',(-77.0000000000051,59.5000000000133,-172.499999999994));
#39380=CARTESIAN_POINT('',(-77.0000000000051,59.500000000017,-140.499999999993));
#39381=CARTESIAN_POINT('',(-74.6696035242059,69.0000000000172,-140.499999999994));
#39382=CARTESIAN_POINT('Origin',(-5.91193760612896E-12,69.0000000000237,
-140.499999999994));
#39383=CARTESIAN_POINT('',(74.6696035241941,69.0000000000265,-172.499999999995));
#39384=CARTESIAN_POINT('',(-5.91193760612896E-12,69.00000000002,-172.499999999995));
#39385=CARTESIAN_POINT('',(74.6696035241941,69.0000000000302,-140.499999999994));
#39386=CARTESIAN_POINT('Origin',(75.8348017620945,64.2500000000304,-140.499999999994));
#39387=CARTESIAN_POINT('',(76.999999999995,59.5000000000266,-172.499999999994));
#39388=CARTESIAN_POINT('',(74.6696035241941,69.0000000000265,-172.499999999995));
#39389=CARTESIAN_POINT('',(76.9999999999949,59.5000000000304,-140.499999999993));
#39390=CARTESIAN_POINT('Origin',(75.7841409691445,65.2500000000299,-143.999999999994));
#39391=CARTESIAN_POINT('',(76.9999999999949,59.50000000003,-143.999999999993));
#39392=CARTESIAN_POINT('Origin',(75.8348017620945,64.2500000000304,-140.499999999994));
#39393=CARTESIAN_POINT('',(76.9999999999949,59.5000000000304,-140.499999999993));
#39394=CARTESIAN_POINT('Origin',(-66.0000000000025,29.5000000000292,-43.49999999999));
#39395=CARTESIAN_POINT('Origin',(85.0000000000052,-57.4999999999582,-47.49999999998));
#39396=CARTESIAN_POINT('',(85.0000000000047,-52.4302858857102,-77.7499999999805));
#39397=CARTESIAN_POINT('Origin',(84.4000000000047,-51.9999999999597,-60.4999999999806));
#39398=CARTESIAN_POINT('',(84.4000000000048,-53.0627460667679,-77.7499999999805));
#39399=CARTESIAN_POINT('',(84.4000000000048,-53.0627460667679,-77.7499999999805));
#39400=CARTESIAN_POINT('Origin',(-93.3999999999946,-60.9999999999807,-107.99999999998));
#39401=CARTESIAN_POINT('',(-84.9999999999938,-69.5697141142314,-107.999999999979));
#39402=CARTESIAN_POINT('',(-84.9999999999953,-52.4302858857286,-107.99999999998));
#39403=CARTESIAN_POINT('',(-84.9999999999949,-57.49999999998,-107.99999999998));
#39404=CARTESIAN_POINT('Origin',(-93.3999999999946,-60.9999999999807,-107.99999999998));
#39405=CARTESIAN_POINT('Origin',(-93.3999999999967,-36.9999999999807,-107.999999999982));
#39406=CARTESIAN_POINT('',(-84.9999999999959,-45.5697141142313,-107.999999999981));
#39407=CARTESIAN_POINT('',(-84.9999999999974,-28.4302858857285,-107.999999999983));
#39408=CARTESIAN_POINT('',(-84.9999999999949,-57.49999999998,-107.99999999998));
#39409=CARTESIAN_POINT('Origin',(-93.3999999999967,-36.9999999999807,-107.999999999982));
#39410=CARTESIAN_POINT('Origin',(-84.4,2.24700900247621E-11,-87.4999999999866));
#39411=CARTESIAN_POINT('',(-84.4,4.46250000002703,-47.4999999999871));
#39412=CARTESIAN_POINT('Origin',(-77.0000000000058,68.0000000000177,-137.259999999994));
#39413=CARTESIAN_POINT('',(-77.0000000000051,59.5000000000271,-53.2599999999935));
#39414=CARTESIAN_POINT('',(-77.0000000000051,59.5000000000277,-47.4999999999935));
#39415=CARTESIAN_POINT('',(-77.0000000000058,68.0000000000272,-53.2599999999944));
#39416=CARTESIAN_POINT('Origin',(-71.0000000000058,68.0000000000277,-53.2599999999944));
#39417=CARTESIAN_POINT('',(-72.680000000005,59.5000000000281,-47.4999999999935));
#39418=CARTESIAN_POINT('',(-71.0000000000051,59.5000000000283,-47.2599999999935));
#39419=CARTESIAN_POINT('Origin',(-71.0000000000051,59.5000000000276,-53.2599999999935));
#39420=CARTESIAN_POINT('',(-71.0000000000058,68.0000000000282,-47.2599999999944));
#39421=CARTESIAN_POINT('Origin',(-71.0000000000051,59.5000000000275,-53.2599999999935));
#39422=CARTESIAN_POINT('Origin',(74.4999999999942,68.0000000000409,-47.2599999999944));
#39423=CARTESIAN_POINT('',(70.9999999999949,59.5000000000407,-47.2599999999935));
#39424=CARTESIAN_POINT('',(70.9999999999949,59.5000000000407,-47.2599999999935));
#39425=CARTESIAN_POINT('',(-77.0000000000051,59.5000000000277,-47.2599999999935));
#39426=CARTESIAN_POINT('Origin',(70.9999999999949,59.50000000004,-53.2599999999935));
#39427=CARTESIAN_POINT('',(76.9999999999949,59.5000000000407,-53.2599999999935));
#39428=CARTESIAN_POINT('',(72.6799999999949,59.5000000000408,-47.4999999999935));
#39429=CARTESIAN_POINT('Origin',(70.9999999999949,59.50000000004,-53.2599999999935));
#39430=CARTESIAN_POINT('',(76.9999999999949,59.5000000000408,-53.2599999999935));
#39431=CARTESIAN_POINT('Origin',(70.9999999999949,59.50000000004,-53.2599999999935));
#39432=CARTESIAN_POINT('Origin',(-5.07927033766009E-12,59.5000000000344,
-47.4999999999935));
#39433=CARTESIAN_POINT('',(76.9999999999949,59.5000000000411,-47.4999999999935));
#39434=CARTESIAN_POINT('',(-77.000000000005,59.500000000028,-47.4999999999935));
#39435=CARTESIAN_POINT('Origin',(76.9999999999949,59.5000000000311,-137.259999999993));
#39436=CARTESIAN_POINT('',(76.9999999999949,59.5000000000414,-47.4999999999935));
#39437=CARTESIAN_POINT('Origin',(93.4000000000055,-60.9999999999644,-107.99999999998));
#39438=CARTESIAN_POINT('',(85.0000000000047,-52.4302858857137,-107.99999999998));
#39439=CARTESIAN_POINT('',(85.0000000000062,-69.5697141142165,-107.999999999979));
#39440=CARTESIAN_POINT('',(85.0000000000052,-57.4999999999652,-107.99999999998));
#39441=CARTESIAN_POINT('Origin',(93.4000000000055,-60.9999999999644,-107.99999999998));
#39442=CARTESIAN_POINT('Origin',(93.4000000000033,-36.9999999999644,-107.999999999982));
#39443=CARTESIAN_POINT('',(85.0000000000026,-28.4302858857138,-107.999999999983));
#39444=CARTESIAN_POINT('',(85.0000000000041,-45.5697141142166,-107.999999999981));
#39445=CARTESIAN_POINT('',(85.0000000000052,-57.4999999999652,-107.99999999998));
#39446=CARTESIAN_POINT('Origin',(93.4000000000033,-36.9999999999644,-107.999999999982));
#39447=CARTESIAN_POINT('Origin',(-26.6999999999944,-62.6999999999668,-37.4999999999794));
#39448=CARTESIAN_POINT('',(-41.0454358677504,-48.0555993716003,-37.499999999981));
#39449=CARTESIAN_POINT('Origin',(-4.16333634234434E-12,49.0000000000356,
-37.4999999999922));
#39450=CARTESIAN_POINT('Origin',(-26.6999999999944,-62.6999999999668,-37.4999999999794));
#39451=CARTESIAN_POINT('Origin',(38.0550000000051,-57.5569999999592,-21.24999999998));
#39452=CARTESIAN_POINT('',(44.6720415240432,-35.0078367900033,-6.99999999998255));
#39453=CARTESIAN_POINT('Origin',(38.0550000000051,-57.5569999999576,-6.99999999997997));
#39454=CARTESIAN_POINT('',(50.3997394425481,-37.5605651153198,-42.4999999999823));
#39455=CARTESIAN_POINT('Origin',(38.0550000000051,-57.5569999999617,-42.49999999998));
#39456=CARTESIAN_POINT('Ctrl Pts',(44.6720415240431,-35.0078367900032,-6.99999999998257));
#39457=CARTESIAN_POINT('Ctrl Pts',(45.2291351252888,-35.1713156498573,-10.284076887157));
#39458=CARTESIAN_POINT('Ctrl Pts',(45.7750777634791,-35.3550218145083,-13.5491785717897));
#39459=CARTESIAN_POINT('Ctrl Pts',(47.3525593525942,-35.9434876571267,-23.0977381265645));
#39460=CARTESIAN_POINT('Ctrl Pts',(48.5132847234971,-36.4730775652569,-30.3142603319532));
#39461=CARTESIAN_POINT('Ctrl Pts',(49.8914593873258,-37.2534035206445,-39.187988167187));
#39462=CARTESIAN_POINT('Ctrl Pts',(50.1472572750543,-37.4046960021711,-40.8480746317634));
#39463=CARTESIAN_POINT('Ctrl Pts',(50.3997394425481,-37.5605651153197,-42.4999999999823));
#39464=CARTESIAN_POINT('Origin',(1.11022302462516E-13,3.90956798185238E-11,
-6.9999999999866));
#39465=CARTESIAN_POINT('',(41.8306113344324,41.8306113344787,-6.99999999999143));
#39466=CARTESIAN_POINT('Origin',(-49.,3.4821321173717E-11,-6.9999999999866));
#39467=CARTESIAN_POINT('',(-41.8306113344394,41.8306113344714,-6.99999999999143));
#39468=CARTESIAN_POINT('Origin',(4.38538094726937E-12,-48.9999999999609,
-6.99999999998097));
#39469=CARTESIAN_POINT('',(-41.8306113344321,-41.8306113344005,-6.99999999998177));
#39470=CARTESIAN_POINT('Origin',(49.,4.33700384633307E-11,-6.9999999999866));
#39471=CARTESIAN_POINT('',(-35.8473473659403,-44.3539912741743,-6.99999999998147));
#39472=CARTESIAN_POINT('Origin',(-4.16333634234434E-12,49.0000000000391,
-6.99999999999224));
#39473=CARTESIAN_POINT('Origin',(-26.6999999999944,-62.6999999999632,-6.99999999997936));
#39474=CARTESIAN_POINT('Origin',(-26.6999999999944,-62.6999999999646,-18.7499999999794));
#39475=CARTESIAN_POINT('Ctrl Pts',(-41.0454358677504,-48.0555993716003,
-37.499999999981));
#39476=CARTESIAN_POINT('Ctrl Pts',(-40.5741646895959,-47.5939491727217,
-34.0475842300223));
#39477=CARTESIAN_POINT('Ctrl Pts',(-40.0664661275859,-47.1411670911225,
-30.5660187146972));
#39478=CARTESIAN_POINT('Ctrl Pts',(-38.6752029150759,-46.0261353656994,
-21.709527141894));
#39479=CARTESIAN_POINT('Ctrl Pts',(-37.7390814105853,-45.3849092793414,
-16.3423326679795));
#39480=CARTESIAN_POINT('Ctrl Pts',(-36.4217135929675,-44.6490164361965,
-9.73375317041888));
#39481=CARTESIAN_POINT('Ctrl Pts',(-36.1385428528838,-44.499181779111,-8.36069357089042));
#39482=CARTESIAN_POINT('Ctrl Pts',(-35.8473473659402,-44.3539912741743,
-6.99999999998149));
#39483=CARTESIAN_POINT('Origin',(38.0550000000051,-57.5569999999617,-42.49999999998));
#39484=CARTESIAN_POINT('Origin',(-49.,3.07412515582195E-11,-42.4999999999866));
#39485=CARTESIAN_POINT('Origin',(-98.9999999999911,-100.749999999988,-164.999999999975));
#39486=CARTESIAN_POINT('Origin',(1.83186799063151E-12,-19.6933104181538,
-140.499999999984));
#39487=CARTESIAN_POINT('',(-85.,1.63083522380925E-11,-140.499999999987));
#39488=CARTESIAN_POINT('',(-84.9999999999919,-90.9999999999837,-140.499999999976));
#39489=CARTESIAN_POINT('',(-84.9999999999949,-57.4999999999837,-140.49999999998));
#39490=CARTESIAN_POINT('',(-81.0000000000025,29.7500000000166,-140.49999999999));
#39491=CARTESIAN_POINT('',(-99.9999999999942,-65.168999999985,-140.499999999979));
#39492=CARTESIAN_POINT('',(-88.5,-2.83449999998398,-140.499999999986));
#39493=CARTESIAN_POINT('',(-94.9999999999913,-98.4999999999846,-140.499999999975));
#39494=CARTESIAN_POINT('',(-97.4999999999927,-81.8344999999848,-140.499999999977));
#39495=CARTESIAN_POINT('',(-90.6698729810919,-90.9999999999842,-140.499999999976));
#39496=CARTESIAN_POINT('',(-92.8349364905416,-94.7499999999844,-140.499999999976));
#39497=CARTESIAN_POINT('',(-67.4999999999919,-90.9999999999822,-140.499999999976));
#39498=CARTESIAN_POINT('Origin',(-88.5,-2.83449999998398,-140.499999999986));
#39499=CARTESIAN_POINT('',(-99.9999999999942,-65.1689999999854,-143.999999999979));
#39500=CARTESIAN_POINT('',(-77.0000000000051,59.5000000000166,-143.999999999993));
#39501=CARTESIAN_POINT('',(-99.9999999999942,-65.168999999985,-140.499999999979));
#39502=CARTESIAN_POINT('Origin',(1.74860126378462E-12,-18.7858057259544,
-143.999999999984));
#39503=CARTESIAN_POINT('',(-100.999999999994,-65.1689999999855,-143.999999999979));
#39504=CARTESIAN_POINT('',(-89.,-2.83449999998446,-143.999999999986));
#39505=CARTESIAN_POINT('',(-94.9999999999913,-98.499999999985,-143.999999999975));
#39506=CARTESIAN_POINT('',(-97.9999999999927,-81.8344999999852,-143.999999999977));
#39507=CARTESIAN_POINT('',(-97.4999999999927,-81.8344999999852,-143.999999999977));
#39508=CARTESIAN_POINT('Origin',(-89.,-2.83449999998446,-143.999999999986));
#39509=CARTESIAN_POINT('',(-100.999999999994,-65.1689999999867,-153.999999999979));
#39510=CARTESIAN_POINT('',(-100.999999999994,-65.1689999999867,-153.999999999979));
#39511=CARTESIAN_POINT('',(-100.999999999994,-65.1689999999855,-143.999999999979));
#39512=CARTESIAN_POINT('Origin',(1.74860126378462E-12,-18.7858057259555,
-153.999999999984));
#39513=CARTESIAN_POINT('',(-94.9999999999913,-98.4999999999861,-153.999999999975));
#39514=CARTESIAN_POINT('',(-97.9999999999927,-81.8344999999864,-153.999999999977));
#39515=CARTESIAN_POINT('',(-99.9999999999942,-65.1689999999866,-153.999999999979));
#39516=CARTESIAN_POINT('',(-88.5,-2.83449999998554,-153.999999999986));
#39517=CARTESIAN_POINT('',(-97.4999999999927,-81.8344999999864,-153.999999999977));
#39518=CARTESIAN_POINT('Origin',(-88.5,-2.83449999998398,-140.499999999986));
#39519=CARTESIAN_POINT('',(-99.9999999999942,-65.1689999999887,-172.499999999979));
#39520=CARTESIAN_POINT('',(-99.9999999999942,-65.1689999999887,-172.499999999979));
#39521=CARTESIAN_POINT('',(-99.9999999999942,-65.168999999985,-140.499999999979));
#39522=CARTESIAN_POINT('Origin',(1.83186799063151E-12,-19.6933104181575,
-172.499999999985));
#39523=CARTESIAN_POINT('',(40.0000000000088,-98.4999999999765,-172.499999999975));
#39524=CARTESIAN_POINT('',(44.330127018908,-90.9999999999761,-172.499999999976));
#39525=CARTESIAN_POINT('',(42.1650635094584,-94.7499999999763,-172.499999999976));
#39526=CARTESIAN_POINT('',(-39.9999999999913,-98.4999999999835,-172.499999999975));
#39527=CARTESIAN_POINT('',(8.71525074330748E-12,-98.49999999998,-172.499999999975));
#39528=CARTESIAN_POINT('',(-44.330127018892,-90.9999999999838,-172.499999999976));
#39529=CARTESIAN_POINT('',(-42.1650635094416,-94.7499999999837,-172.499999999976));
#39530=CARTESIAN_POINT('',(-90.6698729810919,-90.9999999999879,-172.499999999976));
#39531=CARTESIAN_POINT('',(-67.4999999999919,-90.9999999999859,-172.499999999976));
#39532=CARTESIAN_POINT('',(-94.9999999999913,-98.4999999999883,-172.499999999975));
#39533=CARTESIAN_POINT('',(-92.8349364905416,-94.7499999999881,-172.499999999976));
#39534=CARTESIAN_POINT('',(-97.4999999999927,-81.8344999999885,-172.499999999977));
#39535=CARTESIAN_POINT('',(100.000000000006,-65.1689999999712,-172.499999999979));
#39536=CARTESIAN_POINT('',(88.5,-2.83449999997224,-172.499999999986));
#39537=CARTESIAN_POINT('',(95.0000000000087,-98.4999999999717,-172.499999999975));
#39538=CARTESIAN_POINT('',(97.5000000000073,-81.8344999999715,-172.499999999977));
#39539=CARTESIAN_POINT('',(90.669872981108,-90.9999999999721,-172.499999999976));
#39540=CARTESIAN_POINT('',(92.8349364905584,-94.7499999999719,-172.499999999976));
#39541=CARTESIAN_POINT('',(67.5000000000081,-90.9999999999741,-172.499999999976));
#39542=CARTESIAN_POINT('Origin',(88.5,-2.83449999996856,-140.499999999986));
#39543=CARTESIAN_POINT('',(100.000000000006,-65.1689999999691,-153.999999999979));
#39544=CARTESIAN_POINT('',(100.000000000006,-65.1689999999691,-153.999999999979));
#39545=CARTESIAN_POINT('',(100.000000000006,-65.1689999999676,-140.499999999979));
#39546=CARTESIAN_POINT('Origin',(1.74860126378462E-12,-18.7858057259555,
-153.999999999984));
#39547=CARTESIAN_POINT('',(95.0000000000091,-98.4999999999673,-153.999999999975));
#39548=CARTESIAN_POINT('',(101.000000000006,-65.168999999969,-153.999999999979));
#39549=CARTESIAN_POINT('',(98.0000000000073,-81.8344999999693,-153.999999999977));
#39550=CARTESIAN_POINT('',(97.5000000000073,-81.8344999999693,-153.999999999977));
#39551=CARTESIAN_POINT('',(89.,-2.83449999997005,-153.999999999986));
#39552=CARTESIAN_POINT('Origin',(89.,-2.83449999996892,-143.999999999986));
#39553=CARTESIAN_POINT('',(101.000000000006,-65.1689999999679,-143.999999999979));
#39554=CARTESIAN_POINT('',(76.9999999999949,59.50000000003,-143.999999999993));
#39555=CARTESIAN_POINT('',(101.000000000006,-65.1689999999679,-143.999999999979));
#39556=CARTESIAN_POINT('Origin',(1.74860126378462E-12,-18.7858057259544,
-143.999999999984));
#39557=CARTESIAN_POINT('',(95.0000000000091,-98.4999999999662,-143.999999999975));
#39558=CARTESIAN_POINT('',(100.000000000006,-65.168999999968,-143.999999999979));
#39559=CARTESIAN_POINT('',(97.5000000000073,-81.8344999999682,-143.999999999977));
#39560=CARTESIAN_POINT('',(98.0000000000073,-81.8344999999681,-143.999999999977));
#39561=CARTESIAN_POINT('',(88.5,-2.83449999996897,-143.999999999986));
#39562=CARTESIAN_POINT('Origin',(88.5,-2.83449999996856,-140.499999999986));
#39563=CARTESIAN_POINT('',(100.000000000006,-65.1689999999675,-140.499999999979));
#39564=CARTESIAN_POINT('',(76.9999999999949,59.5000000000304,-140.499999999993));
#39565=CARTESIAN_POINT('',(100.000000000006,-65.1689999999676,-140.499999999979));
#39566=CARTESIAN_POINT('Origin',(1.83186799063151E-12,-19.6933104181538,
-140.499999999984));
#39567=CARTESIAN_POINT('',(95.0000000000087,-98.499999999968,-140.499999999975));
#39568=CARTESIAN_POINT('',(90.669872981108,-90.9999999999684,-140.499999999976));
#39569=CARTESIAN_POINT('',(92.8349364905584,-94.7499999999682,-140.499999999976));
#39570=CARTESIAN_POINT('',(97.5000000000073,-81.8344999999678,-140.499999999977));
#39571=CARTESIAN_POINT('',(85.,3.11298296168383E-11,-140.499999999987));
#39572=CARTESIAN_POINT('',(80.9999999999976,29.7500000000308,-140.49999999999));
#39573=CARTESIAN_POINT('',(85.000000000008,-90.9999999999689,-140.499999999976));
#39574=CARTESIAN_POINT('',(85.0000000000052,-57.4999999999689,-140.49999999998));
#39575=CARTESIAN_POINT('',(67.5000000000081,-90.9999999999704,-140.499999999976));
#39576=CARTESIAN_POINT('Origin',(85.0000000000052,-57.4999999999582,-47.49999999998));
#39577=CARTESIAN_POINT('',(85.0000000000041,-45.5697141142096,-47.4999999999814));
#39578=CARTESIAN_POINT('',(85.0000000000047,-52.4302858857068,-47.4999999999806));
#39579=CARTESIAN_POINT('',(85.0000000000027,-29.729655935319,-47.4999999999832));
#39580=CARTESIAN_POINT('',(85.0000000000047,-52.4302858857102,-77.7499999999805));
#39581=CARTESIAN_POINT('',(85.0000000000041,-45.5697141142131,-77.7499999999813));
#39582=CARTESIAN_POINT('Origin',(93.4000000000055,-60.9999999999609,-77.7499999999796));
#39583=CARTESIAN_POINT('',(85.0000000000062,-69.5697141142096,-47.4999999999786));
#39584=CARTESIAN_POINT('Origin',(93.4000000000055,-60.9999999999574,-47.4999999999796));
#39585=CARTESIAN_POINT('',(85.0000000000062,-69.5697141142096,-47.4999999999786));
#39586=CARTESIAN_POINT('',(85.0000000000047,-52.4302858857068,-47.4999999999806));
#39587=CARTESIAN_POINT('Origin',(-93.3999999999946,-60.9999999999772,-77.7499999999796));
#39588=CARTESIAN_POINT('',(-84.9999999999938,-69.5697141142244,-47.4999999999786));
#39589=CARTESIAN_POINT('',(-84.9999999999953,-52.4302858857216,-47.4999999999806));
#39590=CARTESIAN_POINT('Origin',(-93.3999999999946,-60.9999999999737,-47.4999999999796));
#39591=CARTESIAN_POINT('',(-84.9999999999953,-52.4302858857216,-47.4999999999806));
#39592=CARTESIAN_POINT('',(-84.9999999999938,-69.5697141142244,-47.4999999999786));
#39593=CARTESIAN_POINT('Origin',(-93.3999999999967,-36.9999999999772,-77.7499999999823));
#39594=CARTESIAN_POINT('',(-84.9999999999959,-45.5697141142244,-47.4999999999814));
#39595=CARTESIAN_POINT('',(-84.9999999999974,-28.4302858857216,-47.4999999999833));
#39596=CARTESIAN_POINT('Origin',(-93.3999999999967,-36.9999999999737,-47.4999999999823));
#39597=CARTESIAN_POINT('',(-84.9999999999974,-28.4302858857216,-47.4999999999833));
#39598=CARTESIAN_POINT('',(-84.9999999999959,-45.5697141142244,-47.4999999999814));
#39599=CARTESIAN_POINT('Origin',(-84.9999999999949,-57.499999999973,-47.49999999998));
#39600=CARTESIAN_POINT('',(-85.,2.73550713331128E-11,-47.4999999999866));
#39601=CARTESIAN_POINT('',(-84.9999999999973,-29.7296559353338,-47.4999999999832));
#39602=CARTESIAN_POINT('',(-85.,2.70220044257252E-11,-47.4999999999866));
#39603=CARTESIAN_POINT('',(-85.,2.70220044257252E-11,-47.4999999999866));
#39604=CARTESIAN_POINT('',(-84.9999999999919,-90.999999999973,-47.4999999999761));
#39605=CARTESIAN_POINT('',(-84.9999999999919,-90.999999999969,-12.4999999999761));
#39606=CARTESIAN_POINT('',(-84.9999999999973,-29.7296559353338,-47.4999999999832));
#39607=CARTESIAN_POINT('',(-84.9999999999973,-29.7296559353338,-47.4999999999832));
#39608=CARTESIAN_POINT('Origin',(-81.0000000000025,29.7500000000274,-47.49999999999));
#39609=CARTESIAN_POINT('',(-77.0000000000051,59.5000000000277,-47.4999999999935));
#39610=CARTESIAN_POINT('',(-85.,2.70220044257252E-11,-47.4999999999866));
#39611=CARTESIAN_POINT('',(-77.0000000000051,59.5000000000277,-47.4999999999935));
#39612=CARTESIAN_POINT('Origin',(-5.07927033766009E-12,59.5000000000344,
-47.4999999999935));
#39613=CARTESIAN_POINT('',(-5.07927033766009E-12,59.5000000000344,-47.4999999999935));
#39614=CARTESIAN_POINT('Origin',(-77.0000000000051,59.5000000000177,-137.259999999993));
#39615=CARTESIAN_POINT('',(-5.07927033766009E-12,59.5000000000344,-47.4999999999935));
#39616=CARTESIAN_POINT('Origin',(-5.07927033766009E-12,59.5000000000344,
-47.4999999999935));
#39617=CARTESIAN_POINT('',(76.9999999999949,59.5000000000411,-47.4999999999935));
#39618=CARTESIAN_POINT('',(-5.07927033766009E-12,59.5000000000344,-47.4999999999935));
#39619=CARTESIAN_POINT('',(76.9999999999949,59.5000000000411,-47.4999999999935));
#39620=CARTESIAN_POINT('Origin',(80.9999999999976,29.7500000000415,-47.49999999999));
#39621=CARTESIAN_POINT('',(85.,4.17602150776242E-11,-47.4999999999866));
#39622=CARTESIAN_POINT('',(76.9999999999949,59.5000000000411,-47.4999999999935));
#39623=CARTESIAN_POINT('',(85.,4.18434818044711E-11,-47.4999999999866));
#39624=CARTESIAN_POINT('Origin',(85.0000000000052,-57.4999999999582,-47.49999999998));
#39625=CARTESIAN_POINT('',(85.0000000000041,-45.5697141142131,-77.7499999999813));
#39626=CARTESIAN_POINT('',(85.000000000008,-90.9999999999582,-47.4999999999761));
#39627=CARTESIAN_POINT('',(85.0000000000027,-29.729655935319,-47.4999999999832));
#39628=CARTESIAN_POINT('',(85.000000000008,-90.9999999999541,-12.4999999999761));
#39629=CARTESIAN_POINT('',(85.0000000000026,-28.4302858857068,-47.4999999999833));
#39630=CARTESIAN_POINT('',(85.0000000000027,-29.729655935319,-47.4999999999832));
#39631=CARTESIAN_POINT('',(85.0000000000026,-28.4302858857103,-77.7499999999833));
#39632=CARTESIAN_POINT('Origin',(93.4000000000033,-36.9999999999609,-77.7499999999823));
#39633=CARTESIAN_POINT('Origin',(93.4000000000033,-36.9999999999574,-47.4999999999823));
#39634=CARTESIAN_POINT('Origin',(-49.,3.01583844702913E-11,-47.4999999999866));
#39635=CARTESIAN_POINT('',(47.1894200398715,47.1894200399139,-47.499999999992));
#39636=CARTESIAN_POINT('Ctrl Pts',(41.8306113344323,41.8306113344787,-6.99999999999148));
#39637=CARTESIAN_POINT('Ctrl Pts',(43.5801600662902,43.5801600663354,-20.1628904977639));
#39638=CARTESIAN_POINT('Ctrl Pts',(45.4545606962369,45.4545606962808,-34.3333927313629));
#39639=CARTESIAN_POINT('Ctrl Pts',(47.1894200398713,47.189420039914,-47.499999999992));
#39640=CARTESIAN_POINT('Origin',(-49.,3.01583844702913E-11,-47.4999999999866));
#39641=CARTESIAN_POINT('Origin',(4.38538094726937E-12,-48.9999999999656,
-47.499999999981));
#39642=CARTESIAN_POINT('',(-47.1894200398795,47.1894200399057,-47.499999999992));
#39643=CARTESIAN_POINT('Origin',(4.38538094726937E-12,-48.9999999999656,
-47.499999999981));
#39644=CARTESIAN_POINT('Ctrl Pts',(-41.8306113344396,41.8306113344712,-6.99999999999142));
#39645=CARTESIAN_POINT('Ctrl Pts',(-43.5801617860844,43.5801617861141,-20.1629034367356));
#39646=CARTESIAN_POINT('Ctrl Pts',(-45.4545647173523,45.4545647173802,-34.3334232493081));
#39647=CARTESIAN_POINT('Ctrl Pts',(-47.1894200398796,47.1894200399056,-47.499999999992));
#39648=CARTESIAN_POINT('Origin',(49.,3.8707101759905E-11,-47.4999999999866));
#39649=CARTESIAN_POINT('',(-47.1894200398712,-47.1894200398451,-47.4999999999812));
#39650=CARTESIAN_POINT('Ctrl Pts',(-41.8306113344323,-41.8306113344004,
-6.99999999998177));
#39651=CARTESIAN_POINT('Ctrl Pts',(-43.5801603135757,-43.5801603135456,
-20.1628923582288));
#39652=CARTESIAN_POINT('Ctrl Pts',(-45.4545609881339,-45.4545609881059,
-34.3333949466865));
#39653=CARTESIAN_POINT('Ctrl Pts',(-47.1894200398713,-47.1894200398451,
-47.4999999999812));
#39654=CARTESIAN_POINT('Origin',(49.,3.8707101759905E-11,-47.4999999999866));
#39655=CARTESIAN_POINT('Origin',(-4.16333634234434E-12,49.0000000000344,
-47.4999999999922));
#39656=CARTESIAN_POINT('Origin',(-4.16333634234434E-12,49.0000000000344,
-47.4999999999922));
#39657=CARTESIAN_POINT('Origin',(-67.4999999999919,-90.9999999999674,-12.4999999999761));
#39658=CARTESIAN_POINT('',(-90.6698729810919,-90.9999999999695,-12.4999999999761));
#39659=CARTESIAN_POINT('',(-44.330127018892,-90.9999999999654,-12.4999999999761));
#39660=CARTESIAN_POINT('',(-67.4999999999919,-90.9999999999674,-12.4999999999761));
#39661=CARTESIAN_POINT('',(-44.330127018892,-90.9999999999695,-47.4999999999761));
#39662=CARTESIAN_POINT('',(-44.330127018892,-90.9999999999654,-12.4999999999761));
#39663=CARTESIAN_POINT('',(8.07687250414801E-12,-90.9999999999656,-47.4999999999761));
#39664=CARTESIAN_POINT('',(-90.6698729810919,-90.9999999999695,-12.4999999999761));
#39665=CARTESIAN_POINT('Origin',(-42.1650635094416,-94.7499999999652,-12.4999999999757));
#39666=CARTESIAN_POINT('',(-39.9999999999913,-98.499999999965,-12.4999999999752));
#39667=CARTESIAN_POINT('',(-44.330127018892,-90.9999999999654,-12.4999999999761));
#39668=CARTESIAN_POINT('',(-39.9999999999913,-98.4999999999691,-47.4999999999753));
#39669=CARTESIAN_POINT('',(-39.9999999999913,-98.499999999965,-12.4999999999752));
#39670=CARTESIAN_POINT('',(-39.9999999999913,-98.4999999999691,-47.4999999999753));
#39671=CARTESIAN_POINT('Origin',(-92.8349364905416,-94.7499999999697,-12.4999999999757));
#39672=CARTESIAN_POINT('',(-94.9999999999913,-98.4999999999698,-12.4999999999752));
#39673=CARTESIAN_POINT('',(-94.9999999999913,-98.4999999999698,-12.4999999999752));
#39674=CARTESIAN_POINT('',(-94.9999999999913,-98.4999999999698,-12.4999999999752));
#39675=CARTESIAN_POINT('Origin',(-97.4999999999927,-81.8344999999848,-140.499999999977));
#39676=CARTESIAN_POINT('',(-94.9999999999913,-98.4999999999698,-12.4999999999752));
#39677=CARTESIAN_POINT('Origin',(-97.9999999999927,-81.8344999999852,-143.999999999977));
#39678=CARTESIAN_POINT('',(-94.9999999999913,-98.4999999999698,-12.4999999999752));
#39679=CARTESIAN_POINT('Origin',(-97.4999999999927,-81.8344999999848,-140.499999999977));
#39680=CARTESIAN_POINT('',(-94.9999999999913,-98.4999999999698,-12.4999999999752));
#39681=CARTESIAN_POINT('',(-94.9999999999913,-98.4999999999698,-12.4999999999752));
#39682=CARTESIAN_POINT('Origin',(-92.8349364905416,-94.7499999999697,-12.4999999999757));
#39683=CARTESIAN_POINT('',(-94.9999999999913,-98.4999999999929,-212.499999999975));
#39684=CARTESIAN_POINT('',(-90.6698729810919,-90.9999999999925,-212.499999999976));
#39685=CARTESIAN_POINT('',(-94.9999999999913,-98.4999999999929,-212.499999999975));
#39686=CARTESIAN_POINT('',(-94.9999999999913,-98.4999999999698,-12.4999999999752));
#39687=CARTESIAN_POINT('',(-90.6698729810919,-90.9999999999695,-12.4999999999761));
#39688=CARTESIAN_POINT('Origin',(-67.4999999999919,-90.9999999999674,-12.4999999999761));
#39689=CARTESIAN_POINT('',(-44.330127018892,-90.9999999999885,-212.499999999976));
#39690=CARTESIAN_POINT('',(-67.4999999999919,-90.9999999999905,-212.499999999976));
#39691=CARTESIAN_POINT('',(-44.330127018892,-90.9999999999654,-12.4999999999761));
#39692=CARTESIAN_POINT('Origin',(-42.1650635094416,-94.7499999999652,-12.4999999999757));
#39693=CARTESIAN_POINT('',(-39.9999999999913,-98.4999999999881,-212.499999999975));
#39694=CARTESIAN_POINT('',(-44.330127018892,-90.9999999999885,-212.499999999976));
#39695=CARTESIAN_POINT('',(-39.9999999999913,-98.499999999965,-12.4999999999752));
#39696=CARTESIAN_POINT('Origin',(8.71525074330748E-12,-98.4999999999763,
-140.499999999975));
#39697=CARTESIAN_POINT('',(40.0000000000088,-98.4999999999728,-140.499999999975));
#39698=CARTESIAN_POINT('',(40.0000000000088,-98.4999999999581,-12.4999999999752));
#39699=CARTESIAN_POINT('',(-39.9999999999913,-98.4999999999798,-140.499999999975));
#39700=CARTESIAN_POINT('',(8.71525074330748E-12,-98.4999999999763,-140.499999999975));
#39701=CARTESIAN_POINT('',(-39.9999999999913,-98.499999999965,-12.4999999999752));
#39702=CARTESIAN_POINT('Origin',(42.1650635094584,-94.7499999999579,-12.4999999999757));
#39703=CARTESIAN_POINT('',(40.0000000000088,-98.4999999999811,-212.499999999975));
#39704=CARTESIAN_POINT('',(44.330127018908,-90.9999999999807,-212.499999999976));
#39705=CARTESIAN_POINT('',(40.0000000000088,-98.4999999999811,-212.499999999975));
#39706=CARTESIAN_POINT('',(40.0000000000088,-98.4999999999581,-12.4999999999752));
#39707=CARTESIAN_POINT('',(44.330127018908,-90.9999999999577,-12.4999999999761));
#39708=CARTESIAN_POINT('Origin',(67.5000000000081,-90.9999999999557,-12.4999999999761));
#39709=CARTESIAN_POINT('',(90.669872981108,-90.9999999999767,-212.499999999976));
#39710=CARTESIAN_POINT('',(67.5000000000081,-90.9999999999787,-212.499999999976));
#39711=CARTESIAN_POINT('',(90.669872981108,-90.9999999999536,-12.4999999999761));
#39712=CARTESIAN_POINT('Origin',(92.8349364905584,-94.7499999999534,-12.4999999999757));
#39713=CARTESIAN_POINT('',(95.0000000000087,-98.4999999999763,-212.499999999975));
#39714=CARTESIAN_POINT('',(90.669872981108,-90.9999999999767,-212.499999999976));
#39715=CARTESIAN_POINT('',(95.0000000000087,-98.4999999999533,-12.4999999999752));
#39716=CARTESIAN_POINT('Origin',(97.5000000000073,-81.8344999999678,-140.499999999977));
#39717=CARTESIAN_POINT('',(95.0000000000087,-98.4999999999533,-12.4999999999752));
#39718=CARTESIAN_POINT('Origin',(98.0000000000073,-81.8344999999681,-143.999999999977));
#39719=CARTESIAN_POINT('',(95.0000000000087,-98.4999999999533,-12.4999999999752));
#39720=CARTESIAN_POINT('Origin',(97.5000000000073,-81.8344999999678,-140.499999999977));
#39721=CARTESIAN_POINT('',(95.0000000000087,-98.4999999999533,-12.4999999999752));
#39722=CARTESIAN_POINT('Origin',(67.5000000000081,-90.9999999999557,-12.4999999999761));
#39723=CARTESIAN_POINT('',(44.330127018908,-90.9999999999577,-12.4999999999761));
#39724=CARTESIAN_POINT('',(90.669872981108,-90.9999999999536,-12.4999999999761));
#39725=CARTESIAN_POINT('',(67.5000000000081,-90.9999999999557,-12.4999999999761));
#39726=CARTESIAN_POINT('',(90.669872981108,-90.9999999999536,-12.4999999999761));
#39727=CARTESIAN_POINT('',(44.330127018908,-90.9999999999617,-47.4999999999761));
#39728=CARTESIAN_POINT('',(8.07687250414801E-12,-90.9999999999656,-47.4999999999761));
#39729=CARTESIAN_POINT('',(44.330127018908,-90.9999999999577,-12.4999999999761));
#39730=CARTESIAN_POINT('Origin',(92.8349364905584,-94.7499999999534,-12.4999999999757));
#39731=CARTESIAN_POINT('',(95.0000000000087,-98.4999999999533,-12.4999999999752));
#39732=CARTESIAN_POINT('',(90.669872981108,-90.9999999999536,-12.4999999999761));
#39733=CARTESIAN_POINT('',(95.0000000000087,-98.4999999999533,-12.4999999999752));
#39734=CARTESIAN_POINT('Origin',(42.1650635094584,-94.7499999999579,-12.4999999999757));
#39735=CARTESIAN_POINT('',(40.0000000000088,-98.4999999999581,-12.4999999999752));
#39736=CARTESIAN_POINT('',(40.0000000000088,-98.4999999999581,-12.4999999999752));
#39737=CARTESIAN_POINT('',(40.0000000000088,-98.4999999999621,-47.4999999999753));
#39738=CARTESIAN_POINT('',(44.330127018908,-90.9999999999617,-47.4999999999761));
#39739=CARTESIAN_POINT('',(40.0000000000088,-98.4999999999581,-12.4999999999752));
#39740=CARTESIAN_POINT('Origin',(2.72004641033164E-12,-29.7296559353265,
-47.4999999999832));
#39741=CARTESIAN_POINT('',(-39.9999999999898,-114.999999999969,-47.4999999999733));
#39742=CARTESIAN_POINT('',(-39.9999999999905,-106.749999999969,-47.4999999999743));
#39743=CARTESIAN_POINT('',(40.0000000000102,-114.999999999962,-47.4999999999733));
#39744=CARTESIAN_POINT('',(1.01585406753202E-11,-114.999999999966,-47.4999999999733));
#39745=CARTESIAN_POINT('',(40.0000000000095,-106.749999999962,-47.4999999999743));
#39746=CARTESIAN_POINT('Origin',(-39.9999999999905,-106.749999999965,-12.4999999999743));
#39747=CARTESIAN_POINT('',(-39.9999999999898,-114.999999999965,-12.4999999999733));
#39748=CARTESIAN_POINT('',(-39.9999999999908,-103.559005108899,-12.4999999999747));
#39749=CARTESIAN_POINT('',(-39.9999999999898,-114.999999999969,-47.4999999999733));
#39750=CARTESIAN_POINT('Origin',(-67.4999999999909,-103.559005108901,-12.4999999999747));
#39751=CARTESIAN_POINT('',(-94.9999999999898,-114.99999999997,-12.4999999999733));
#39752=CARTESIAN_POINT('',(-94.9999999999906,-106.74999999997,-12.4999999999743));
#39753=CARTESIAN_POINT('',(1.01585406753202E-11,-114.999999999962,-12.4999999999733));
#39754=CARTESIAN_POINT('Origin',(-94.9999999999906,-106.74999999997,-12.4999999999743));
#39755=CARTESIAN_POINT('',(-94.9999999999898,-114.999999999993,-212.499999999974));
#39756=CARTESIAN_POINT('',(-94.9999999999908,-103.559005108927,-212.499999999974));
#39757=CARTESIAN_POINT('',(-94.9999999999898,-114.999999999974,-47.4999999999733));
#39758=CARTESIAN_POINT('Origin',(-67.4999999999909,-103.559005108924,-212.499999999974));
#39759=CARTESIAN_POINT('',(-39.9999999999898,-114.999999999988,-212.499999999974));
#39760=CARTESIAN_POINT('',(-39.9999999999905,-106.749999999988,-212.499999999974));
#39761=CARTESIAN_POINT('',(1.01585406753202E-11,-114.999999999985,-212.499999999974));
#39762=CARTESIAN_POINT('Origin',(-39.9999999999905,-106.749999999965,-12.4999999999743));
#39763=CARTESIAN_POINT('',(-39.9999999999898,-114.99999999998,-140.499999999973));
#39764=CARTESIAN_POINT('',(-39.9999999999973,-29.7296559353406,-140.499999999983));
#39765=CARTESIAN_POINT('',(-39.9999999999898,-114.999999999969,-47.4999999999733));
#39766=CARTESIAN_POINT('Origin',(2.72004641033164E-12,-29.7296559353372,
-140.499999999983));
#39767=CARTESIAN_POINT('',(40.0000000000102,-114.999999999973,-140.499999999973));
#39768=CARTESIAN_POINT('',(40.0000000000095,-106.749999999973,-140.499999999974));
#39769=CARTESIAN_POINT('',(1.01585406753202E-11,-114.999999999976,-140.499999999973));
#39770=CARTESIAN_POINT('Origin',(40.0000000000095,-106.749999999958,-12.4999999999743));
#39771=CARTESIAN_POINT('',(40.0000000000102,-114.999999999981,-212.499999999974));
#39772=CARTESIAN_POINT('',(40.0000000000092,-103.559005108915,-212.499999999974));
#39773=CARTESIAN_POINT('',(40.0000000000102,-114.999999999962,-47.4999999999733));
#39774=CARTESIAN_POINT('Origin',(67.5000000000092,-103.559005108913,-212.499999999974));
#39775=CARTESIAN_POINT('',(95.0000000000102,-114.999999999976,-212.499999999974));
#39776=CARTESIAN_POINT('',(95.0000000000094,-106.749999999976,-212.499999999974));
#39777=CARTESIAN_POINT('',(1.01585406753202E-11,-114.999999999985,-212.499999999974));
#39778=CARTESIAN_POINT('Origin',(95.0000000000094,-106.749999999953,-12.4999999999743));
#39779=CARTESIAN_POINT('',(95.0000000000102,-114.999999999953,-12.4999999999733));
#39780=CARTESIAN_POINT('',(95.0000000000092,-103.559005108887,-12.4999999999747));
#39781=CARTESIAN_POINT('',(95.0000000000102,-114.999999999957,-47.4999999999733));
#39782=CARTESIAN_POINT('Origin',(67.5000000000092,-103.55900510889,-12.4999999999747));
#39783=CARTESIAN_POINT('',(40.0000000000102,-114.999999999958,-12.4999999999733));
#39784=CARTESIAN_POINT('',(40.0000000000095,-106.749999999958,-12.4999999999743));
#39785=CARTESIAN_POINT('',(1.01585406753202E-11,-114.999999999962,-12.4999999999733));
#39786=CARTESIAN_POINT('Origin',(40.0000000000095,-106.749999999958,-12.4999999999743));
#39787=CARTESIAN_POINT('',(40.0000000000102,-114.999999999962,-47.4999999999733));
#39788=CARTESIAN_POINT('Origin',(1.01585406753202E-11,-114.999999999966,
-47.4999999999733));
#39948=UNCERTAINTY_MEASURE_WITH_UNIT(LENGTH_MEASURE(0.01),#39960,
'DISTANCE_ACCURACY_VALUE',
'Maximum model space distance between geometric entities at asserted c
onnectivities');
#39950=UNCERTAINTY_MEASURE_WITH_UNIT(LENGTH_MEASURE(0.01),#39960,
'DISTANCE_ACCURACY_VALUE',
'Maximum model space distance between geometric entities at asserted c
onnectivities');
#39957=(
GEOMETRIC_REPRESENTATION_CONTEXT(3)
GLOBAL_UNCERTAINTY_ASSIGNED_CONTEXT((#39948))
GLOBAL_UNIT_ASSIGNED_CONTEXT((#39960,#39962,#39963))
REPRESENTATION_CONTEXT('','3D')
);
#39959=(
GEOMETRIC_REPRESENTATION_CONTEXT(3)
GLOBAL_UNCERTAINTY_ASSIGNED_CONTEXT((#39950))
GLOBAL_UNIT_ASSIGNED_CONTEXT((#39960,#39962,#39963))
REPRESENTATION_CONTEXT('','3D')
);
#39960=(
LENGTH_UNIT()
NAMED_UNIT(*)
SI_UNIT(.MILLI.,.METRE.)
);
#39962=(
NAMED_UNIT(*)
PLANE_ANGLE_UNIT()
SI_UNIT($,.RADIAN.)
);
#39963=(
NAMED_UNIT(*)
SI_UNIT($,.STERADIAN.)
SOLID_ANGLE_UNIT()
);
#39970=SHAPE_DEFINITION_REPRESENTATION(#39978,#40007);
#39978=PRODUCT_DEFINITION_SHAPE('',$,#40016);
#40007=SHAPE_REPRESENTATION('',(#18852),#39957);
#40009=PRODUCT_DEFINITION_CONTEXT('part definition',#40035,'design');
#40016=PRODUCT_DEFINITION('Reference_Motor_Envelope',
'Reference_Motor_Envelope',#40024,#40009);
#40024=PRODUCT_DEFINITION_FORMATION('',$,#40043);
#40035=APPLICATION_CONTEXT(
'Core Data for Automotive Mechanical Design Process');
#40036=PRODUCT_CONTEXT('part definition',#40035,'mechanical');
#40043=PRODUCT('Reference_Motor_Envelope','Reference_Motor_Envelope',$,
(#40036));
#40046=PRESENTATION_STYLE_ASSIGNMENT((#40048));
#40048=SURFACE_STYLE_USAGE(.BOTH.,#40050);
#40050=SURFACE_SIDE_STYLE('',(#40052));
#40052=SURFACE_STYLE_FILL_AREA(#40054);
#40054=FILL_AREA_STYLE('Opaque(202,209,238)',(#40056));
#40056=FILL_AREA_STYLE_COLOUR('Opaque(202,209,238)',#40058);
#40058=COLOUR_RGB('Opaque(202,209,238)', 0.66274510, 0.83137255, 0.94901961);
ENDSEC;
END-ISO-10303-21;
